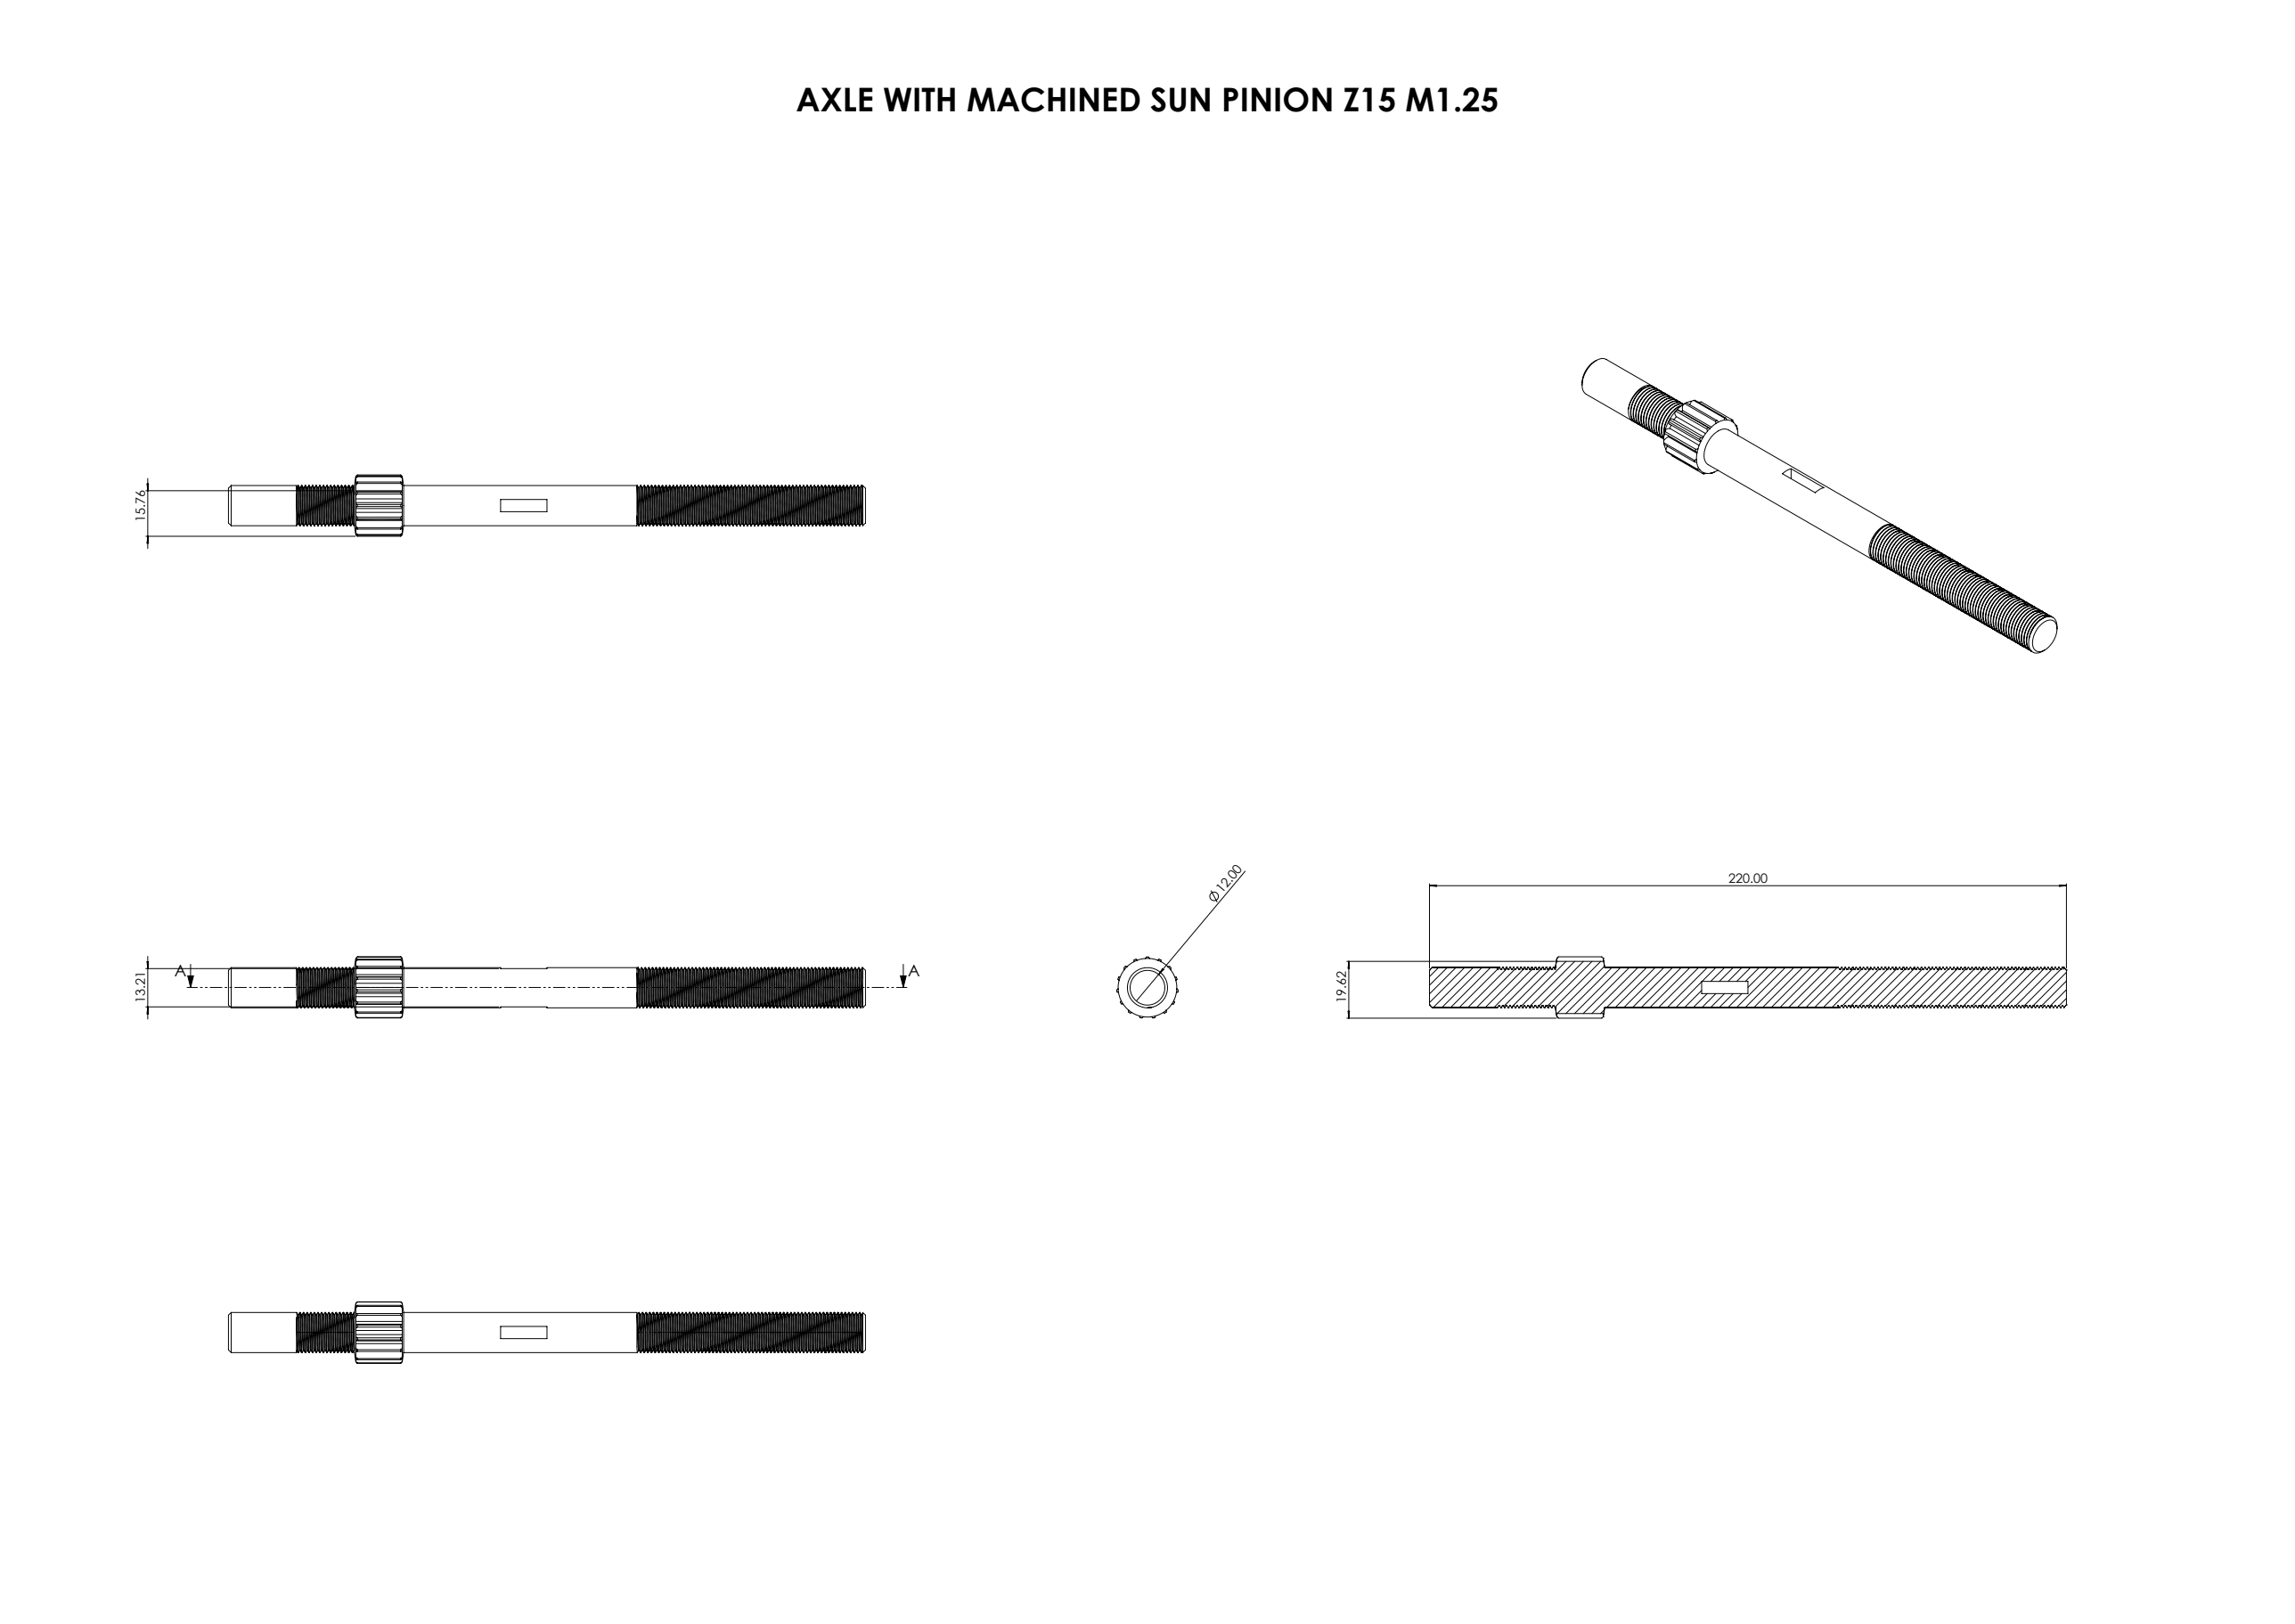
ISO-10303-21;
HEADER;
/* Generated by software containing ST-Developer
 * from STEP Tools, Inc. (www.steptools.com) 
 */

FILE_DESCRIPTION(
/* description */ (''),
/* implementation_level */ '2;1');

FILE_NAME(
/* name */ '01_Axle_with_Machined_Sun_Pinion_Z15_M1.25.step',
/* time_stamp */ '2026-10-11T13:00:10-07:00',
/* author */ (''),
/* organization */ (''),
/* preprocessor_version */ 'ST-DEVELOPER v20.2',
/* originating_system */ 'Autodesk Translation Framework v15.15.0.0',
/* authorisation */ '');

FILE_SCHEMA (('AUTOMOTIVE_DESIGN { 1 0 10303 214 3 1 1 }'));
ENDSEC;

DATA;
#10=MECHANICAL_DESIGN_GEOMETRIC_PRESENTATION_REPRESENTATION('',(#358),#65563);
#336=SHAPE_REPRESENTATION_RELATIONSHIP('SRR','None',#65614,#347);
#347=ADVANCED_BREP_SHAPE_REPRESENTATION('',(#369),#65552);
#358=STYLED_ITEM('',(#65788),#369);
#369=MANIFOLD_SOLID_BREP('Body1',#20008);
#380=CONICAL_SURFACE('',#20340,10.375,0.785398163397451);
#381=CONICAL_SURFACE('',#20343,10.375,0.785398163397451);
#382=CONICAL_SURFACE('',#20348,10.375,0.785398163397451);
#383=CONICAL_SURFACE('',#20357,10.375,0.785398163397451);
#384=CONICAL_SURFACE('',#20362,10.375,0.785398163397451);
#385=CONICAL_SURFACE('',#20371,10.375,0.785398163397451);
#386=CONICAL_SURFACE('',#20376,10.375,0.785398163397451);
#387=CONICAL_SURFACE('',#20385,10.375,0.785398163397451);
#388=CONICAL_SURFACE('',#20390,10.375,0.785398163397451);
#389=CONICAL_SURFACE('',#20399,10.375,0.785398163397451);
#390=CONICAL_SURFACE('',#20404,10.375,0.785398163397451);
#391=CONICAL_SURFACE('',#20413,10.375,0.785398163397451);
#392=CONICAL_SURFACE('',#20418,10.375,0.785398163397451);
#393=CONICAL_SURFACE('',#20427,10.375,0.785398163397451);
#394=CONICAL_SURFACE('',#20432,10.375,0.785398163397451);
#395=CONICAL_SURFACE('',#20443,10.375,0.785398163397451);
#396=CONICAL_SURFACE('',#20448,10.375,0.785398163397451);
#397=CONICAL_SURFACE('',#20457,10.375,0.785398163397451);
#398=CONICAL_SURFACE('',#20462,10.375,0.785398163397451);
#399=CONICAL_SURFACE('',#20471,10.375,0.785398163397451);
#400=CONICAL_SURFACE('',#20476,10.375,0.785398163397451);
#401=CONICAL_SURFACE('',#20485,10.375,0.785398163397451);
#402=CONICAL_SURFACE('',#20490,10.375,0.785398163397451);
#403=CONICAL_SURFACE('',#20499,10.375,0.785398163397451);
#404=CONICAL_SURFACE('',#20504,10.375,0.785398163397451);
#405=CONICAL_SURFACE('',#20513,10.375,0.785398163397451);
#406=CONICAL_SURFACE('',#20518,10.375,0.785398163397451);
#407=CONICAL_SURFACE('',#20527,10.375,0.785398163397451);
#408=CONICAL_SURFACE('',#20532,10.375,0.785398163397451);
#409=CONICAL_SURFACE('',#20541,10.375,0.785398163397451);
#410=CONICAL_SURFACE('',#20547,6.5,0.78539816339745);
#411=CONICAL_SURFACE('',#20548,8.5625,1.41214106460849);
#412=CONICAL_SURFACE('',#20549,8.5625,1.4121410646085);
#413=CONICAL_SURFACE('',#20552,6.5,0.78539816339745);
#500=(
BOUNDED_SURFACE()
B_SPLINE_SURFACE(5,1,((#42423,#42424),(#42425,#42426),(#42427,#42428),(#42429,
#42430),(#42431,#42432),(#42433,#42434),(#42435,#42436),(#42437,#42438),
(#42439,#42440),(#42441,#42442),(#42443,#42444),(#42445,#42446),(#42447,
#42448),(#42449,#42450),(#42451,#42452),(#42453,#42454),(#42455,#42456),
(#42457,#42458),(#42459,#42460),(#42461,#42462),(#42463,#42464),(#42465,
#42466),(#42467,#42468),(#42469,#42470),(#42471,#42472),(#42473,#42474),
(#42475,#42476),(#42477,#42478),(#42479,#42480),(#42481,#42482),(#42483,
#42484),(#42485,#42486),(#42487,#42488),(#42489,#42490),(#42491,#42492),
(#42493,#42494),(#42495,#42496),(#42497,#42498),(#42499,#42500),(#42501,
#42502)),.UNSPECIFIED.,.F.,.F.,.F.)
B_SPLINE_SURFACE_WITH_KNOTS((6,1,1,1,1,1,1,1,1,1,1,1,1,1,1,1,1,1,1,1,1,
1,1,1,1,1,1,1,1,1,1,1,1,1,1,6),(2,2),(-1.,-0.971428571428572,-0.942857142857143,
-0.914285714285714,-0.885714285714286,-0.857142857142857,-0.828571428571429,
-0.8,-0.771428571428572,-0.742857142857143,-0.714285714285714,-0.685714285714286,
-0.657142857142857,-0.628571428571429,-0.6,-0.571428571428572,-0.542857142857143,
-0.514285714285714,-0.485714285714286,-0.457142857142857,-0.428571428571429,
-0.4,-0.371428571428571,-0.342857142857143,-0.314285714285714,-0.285714285714286,
-0.257142857142857,-0.228571428571429,-0.2,-0.171428571428571,-0.142857142857143,
-0.114285714285714,-0.0857142857142857,-0.0571428571428571,-0.0285714285714286,
0.),(0.,1.6),.UNSPECIFIED.)
GEOMETRIC_REPRESENTATION_ITEM()
RATIONAL_B_SPLINE_SURFACE(((1.,1.),(1.,1.),(1.,1.),(1.,1.),(1.,1.),(1.,
1.),(1.,1.),(1.,1.),(1.,1.),(1.,1.),(1.,1.),(1.,1.),(1.,1.),(1.,1.),(1.,
1.),(1.,1.),(1.,1.),(1.,1.),(1.,1.),(1.,1.),(1.,1.),(1.,1.),(1.,1.),(1.,
1.),(1.,1.),(1.,1.),(1.,1.),(1.,1.),(1.,1.),(1.,1.),(1.,1.),(1.,1.),(1.,
1.),(1.,1.),(1.,1.),(1.,1.),(1.,1.),(1.,1.),(1.,1.),(1.,1.)))
REPRESENTATION_ITEM('')
SURFACE()
);
#501=(
BOUNDED_SURFACE()
B_SPLINE_SURFACE(5,1,((#42551,#42552),(#42553,#42554),(#42555,#42556),(#42557,
#42558),(#42559,#42560),(#42561,#42562),(#42563,#42564),(#42565,#42566),
(#42567,#42568),(#42569,#42570),(#42571,#42572),(#42573,#42574),(#42575,
#42576),(#42577,#42578),(#42579,#42580),(#42581,#42582),(#42583,#42584),
(#42585,#42586),(#42587,#42588),(#42589,#42590),(#42591,#42592),(#42593,
#42594),(#42595,#42596),(#42597,#42598),(#42599,#42600),(#42601,#42602),
(#42603,#42604),(#42605,#42606),(#42607,#42608),(#42609,#42610),(#42611,
#42612),(#42613,#42614),(#42615,#42616),(#42617,#42618),(#42619,#42620),
(#42621,#42622),(#42623,#42624),(#42625,#42626),(#42627,#42628),(#42629,
#42630)),.UNSPECIFIED.,.F.,.F.,.F.)
B_SPLINE_SURFACE_WITH_KNOTS((6,1,1,1,1,1,1,1,1,1,1,1,1,1,1,1,1,1,1,1,1,
1,1,1,1,1,1,1,1,1,1,1,1,1,1,6),(2,2),(-1.,-0.971428571428572,-0.942857142857143,
-0.914285714285714,-0.885714285714286,-0.857142857142857,-0.828571428571429,
-0.8,-0.771428571428572,-0.742857142857143,-0.714285714285714,-0.685714285714286,
-0.657142857142857,-0.628571428571429,-0.6,-0.571428571428572,-0.542857142857143,
-0.514285714285714,-0.485714285714286,-0.457142857142857,-0.428571428571429,
-0.4,-0.371428571428571,-0.342857142857143,-0.314285714285714,-0.285714285714286,
-0.257142857142857,-0.228571428571429,-0.2,-0.171428571428571,-0.142857142857143,
-0.114285714285714,-0.0857142857142857,-0.0571428571428571,-0.0285714285714286,
0.),(0.,1.6),.UNSPECIFIED.)
GEOMETRIC_REPRESENTATION_ITEM()
RATIONAL_B_SPLINE_SURFACE(((1.,1.),(1.,1.),(1.,1.),(1.,1.),(1.,1.),(1.,
1.),(1.,1.),(1.,1.),(1.,1.),(1.,1.),(1.,1.),(1.,1.),(1.,1.),(1.,1.),(1.,
1.),(1.,1.),(1.,1.),(1.,1.),(1.,1.),(1.,1.),(1.,1.),(1.,1.),(1.,1.),(1.,
1.),(1.,1.),(1.,1.),(1.,1.),(1.,1.),(1.,1.),(1.,1.),(1.,1.),(1.,1.),(1.,
1.),(1.,1.),(1.,1.),(1.,1.),(1.,1.),(1.,1.),(1.,1.),(1.,1.)))
REPRESENTATION_ITEM('')
SURFACE()
);
#502=(
BOUNDED_SURFACE()
B_SPLINE_SURFACE(5,1,((#42775,#42776),(#42777,#42778),(#42779,#42780),(#42781,
#42782),(#42783,#42784),(#42785,#42786),(#42787,#42788),(#42789,#42790),
(#42791,#42792),(#42793,#42794),(#42795,#42796),(#42797,#42798),(#42799,
#42800),(#42801,#42802),(#42803,#42804),(#42805,#42806),(#42807,#42808),
(#42809,#42810),(#42811,#42812),(#42813,#42814),(#42815,#42816),(#42817,
#42818),(#42819,#42820),(#42821,#42822),(#42823,#42824),(#42825,#42826),
(#42827,#42828),(#42829,#42830),(#42831,#42832),(#42833,#42834),(#42835,
#42836),(#42837,#42838),(#42839,#42840),(#42841,#42842),(#42843,#42844),
(#42845,#42846),(#42847,#42848),(#42849,#42850),(#42851,#42852),(#42853,
#42854)),.UNSPECIFIED.,.F.,.F.,.F.)
B_SPLINE_SURFACE_WITH_KNOTS((6,1,1,1,1,1,1,1,1,1,1,1,1,1,1,1,1,1,1,1,1,
1,1,1,1,1,1,1,1,1,1,1,1,1,1,6),(2,2),(-1.,-0.971428571428572,-0.942857142857143,
-0.914285714285714,-0.885714285714286,-0.857142857142857,-0.828571428571429,
-0.8,-0.771428571428572,-0.742857142857143,-0.714285714285714,-0.685714285714286,
-0.657142857142857,-0.628571428571429,-0.6,-0.571428571428572,-0.542857142857143,
-0.514285714285714,-0.485714285714286,-0.457142857142857,-0.428571428571429,
-0.4,-0.371428571428571,-0.342857142857143,-0.314285714285714,-0.285714285714286,
-0.257142857142857,-0.228571428571429,-0.2,-0.171428571428571,-0.142857142857143,
-0.114285714285714,-0.0857142857142857,-0.0571428571428571,-0.0285714285714286,
0.),(0.,1.6),.UNSPECIFIED.)
GEOMETRIC_REPRESENTATION_ITEM()
RATIONAL_B_SPLINE_SURFACE(((1.,1.),(1.,1.),(1.,1.),(1.,1.),(1.,1.),(1.,
1.),(1.,1.),(1.,1.),(1.,1.),(1.,1.),(1.,1.),(1.,1.),(1.,1.),(1.,1.),(1.,
1.),(1.,1.),(1.,1.),(1.,1.),(1.,1.),(1.,1.),(1.,1.),(1.,1.),(1.,1.),(1.,
1.),(1.,1.),(1.,1.),(1.,1.),(1.,1.),(1.,1.),(1.,1.),(1.,1.),(1.,1.),(1.,
1.),(1.,1.),(1.,1.),(1.,1.),(1.,1.),(1.,1.),(1.,1.),(1.,1.)))
REPRESENTATION_ITEM('')
SURFACE()
);
#503=(
BOUNDED_SURFACE()
B_SPLINE_SURFACE(5,1,((#42903,#42904),(#42905,#42906),(#42907,#42908),(#42909,
#42910),(#42911,#42912),(#42913,#42914),(#42915,#42916),(#42917,#42918),
(#42919,#42920),(#42921,#42922),(#42923,#42924),(#42925,#42926),(#42927,
#42928),(#42929,#42930),(#42931,#42932),(#42933,#42934),(#42935,#42936),
(#42937,#42938),(#42939,#42940),(#42941,#42942),(#42943,#42944),(#42945,
#42946),(#42947,#42948),(#42949,#42950),(#42951,#42952),(#42953,#42954),
(#42955,#42956),(#42957,#42958),(#42959,#42960),(#42961,#42962),(#42963,
#42964),(#42965,#42966),(#42967,#42968),(#42969,#42970),(#42971,#42972),
(#42973,#42974),(#42975,#42976),(#42977,#42978),(#42979,#42980),(#42981,
#42982)),.UNSPECIFIED.,.F.,.F.,.F.)
B_SPLINE_SURFACE_WITH_KNOTS((6,1,1,1,1,1,1,1,1,1,1,1,1,1,1,1,1,1,1,1,1,
1,1,1,1,1,1,1,1,1,1,1,1,1,1,6),(2,2),(-1.,-0.971428571428572,-0.942857142857143,
-0.914285714285714,-0.885714285714286,-0.857142857142857,-0.828571428571429,
-0.8,-0.771428571428572,-0.742857142857143,-0.714285714285714,-0.685714285714286,
-0.657142857142857,-0.628571428571429,-0.6,-0.571428571428572,-0.542857142857143,
-0.514285714285714,-0.485714285714286,-0.457142857142857,-0.428571428571429,
-0.4,-0.371428571428571,-0.342857142857143,-0.314285714285714,-0.285714285714286,
-0.257142857142857,-0.228571428571429,-0.2,-0.171428571428571,-0.142857142857143,
-0.114285714285714,-0.0857142857142857,-0.0571428571428571,-0.0285714285714286,
0.),(0.,1.6),.UNSPECIFIED.)
GEOMETRIC_REPRESENTATION_ITEM()
RATIONAL_B_SPLINE_SURFACE(((1.,1.),(1.,1.),(1.,1.),(1.,1.),(1.,1.),(1.,
1.),(1.,1.),(1.,1.),(1.,1.),(1.,1.),(1.,1.),(1.,1.),(1.,1.),(1.,1.),(1.,
1.),(1.,1.),(1.,1.),(1.,1.),(1.,1.),(1.,1.),(1.,1.),(1.,1.),(1.,1.),(1.,
1.),(1.,1.),(1.,1.),(1.,1.),(1.,1.),(1.,1.),(1.,1.),(1.,1.),(1.,1.),(1.,
1.),(1.,1.),(1.,1.),(1.,1.),(1.,1.),(1.,1.),(1.,1.),(1.,1.)))
REPRESENTATION_ITEM('')
SURFACE()
);
#504=(
BOUNDED_SURFACE()
B_SPLINE_SURFACE(5,1,((#43097,#43098),(#43099,#43100),(#43101,#43102),(#43103,
#43104),(#43105,#43106),(#43107,#43108),(#43109,#43110),(#43111,#43112),
(#43113,#43114),(#43115,#43116),(#43117,#43118),(#43119,#43120),(#43121,
#43122),(#43123,#43124),(#43125,#43126),(#43127,#43128),(#43129,#43130),
(#43131,#43132),(#43133,#43134),(#43135,#43136),(#43137,#43138),(#43139,
#43140),(#43141,#43142),(#43143,#43144),(#43145,#43146),(#43147,#43148),
(#43149,#43150),(#43151,#43152),(#43153,#43154),(#43155,#43156),(#43157,
#43158),(#43159,#43160),(#43161,#43162),(#43163,#43164),(#43165,#43166),
(#43167,#43168),(#43169,#43170),(#43171,#43172),(#43173,#43174),(#43175,
#43176)),.UNSPECIFIED.,.F.,.F.,.F.)
B_SPLINE_SURFACE_WITH_KNOTS((6,1,1,1,1,1,1,1,1,1,1,1,1,1,1,1,1,1,1,1,1,
1,1,1,1,1,1,1,1,1,1,1,1,1,1,6),(2,2),(-1.,-0.971428571428572,-0.942857142857143,
-0.914285714285714,-0.885714285714286,-0.857142857142857,-0.828571428571429,
-0.8,-0.771428571428572,-0.742857142857143,-0.714285714285714,-0.685714285714286,
-0.657142857142857,-0.628571428571429,-0.6,-0.571428571428572,-0.542857142857143,
-0.514285714285714,-0.485714285714286,-0.457142857142857,-0.428571428571429,
-0.4,-0.371428571428571,-0.342857142857143,-0.314285714285714,-0.285714285714286,
-0.257142857142857,-0.228571428571429,-0.2,-0.171428571428571,-0.142857142857143,
-0.114285714285714,-0.0857142857142857,-0.0571428571428571,-0.0285714285714286,
0.),(0.,1.6),.UNSPECIFIED.)
GEOMETRIC_REPRESENTATION_ITEM()
RATIONAL_B_SPLINE_SURFACE(((1.,1.),(1.,1.),(1.,1.),(1.,1.),(1.,1.),(1.,
1.),(1.,1.),(1.,1.),(1.,1.),(1.,1.),(1.,1.),(1.,1.),(1.,1.),(1.,1.),(1.,
1.),(1.,1.),(1.,1.),(1.,1.),(1.,1.),(1.,1.),(1.,1.),(1.,1.),(1.,1.),(1.,
1.),(1.,1.),(1.,1.),(1.,1.),(1.,1.),(1.,1.),(1.,1.),(1.,1.),(1.,1.),(1.,
1.),(1.,1.),(1.,1.),(1.,1.),(1.,1.),(1.,1.),(1.,1.),(1.,1.)))
REPRESENTATION_ITEM('')
SURFACE()
);
#505=(
BOUNDED_SURFACE()
B_SPLINE_SURFACE(5,1,((#43225,#43226),(#43227,#43228),(#43229,#43230),(#43231,
#43232),(#43233,#43234),(#43235,#43236),(#43237,#43238),(#43239,#43240),
(#43241,#43242),(#43243,#43244),(#43245,#43246),(#43247,#43248),(#43249,
#43250),(#43251,#43252),(#43253,#43254),(#43255,#43256),(#43257,#43258),
(#43259,#43260),(#43261,#43262),(#43263,#43264),(#43265,#43266),(#43267,
#43268),(#43269,#43270),(#43271,#43272),(#43273,#43274),(#43275,#43276),
(#43277,#43278),(#43279,#43280),(#43281,#43282),(#43283,#43284),(#43285,
#43286),(#43287,#43288),(#43289,#43290),(#43291,#43292),(#43293,#43294),
(#43295,#43296),(#43297,#43298),(#43299,#43300),(#43301,#43302),(#43303,
#43304)),.UNSPECIFIED.,.F.,.F.,.F.)
B_SPLINE_SURFACE_WITH_KNOTS((6,1,1,1,1,1,1,1,1,1,1,1,1,1,1,1,1,1,1,1,1,
1,1,1,1,1,1,1,1,1,1,1,1,1,1,6),(2,2),(-1.,-0.971428571428572,-0.942857142857143,
-0.914285714285714,-0.885714285714286,-0.857142857142857,-0.828571428571429,
-0.8,-0.771428571428572,-0.742857142857143,-0.714285714285714,-0.685714285714286,
-0.657142857142857,-0.628571428571429,-0.6,-0.571428571428572,-0.542857142857143,
-0.514285714285714,-0.485714285714286,-0.457142857142857,-0.428571428571429,
-0.4,-0.371428571428571,-0.342857142857143,-0.314285714285714,-0.285714285714286,
-0.257142857142857,-0.228571428571429,-0.2,-0.171428571428571,-0.142857142857143,
-0.114285714285714,-0.0857142857142857,-0.0571428571428571,-0.0285714285714286,
0.),(0.,1.6),.UNSPECIFIED.)
GEOMETRIC_REPRESENTATION_ITEM()
RATIONAL_B_SPLINE_SURFACE(((1.,1.),(1.,1.),(1.,1.),(1.,1.),(1.,1.),(1.,
1.),(1.,1.),(1.,1.),(1.,1.),(1.,1.),(1.,1.),(1.,1.),(1.,1.),(1.,1.),(1.,
1.),(1.,1.),(1.,1.),(1.,1.),(1.,1.),(1.,1.),(1.,1.),(1.,1.),(1.,1.),(1.,
1.),(1.,1.),(1.,1.),(1.,1.),(1.,1.),(1.,1.),(1.,1.),(1.,1.),(1.,1.),(1.,
1.),(1.,1.),(1.,1.),(1.,1.),(1.,1.),(1.,1.),(1.,1.),(1.,1.)))
REPRESENTATION_ITEM('')
SURFACE()
);
#506=(
BOUNDED_SURFACE()
B_SPLINE_SURFACE(5,1,((#43419,#43420),(#43421,#43422),(#43423,#43424),(#43425,
#43426),(#43427,#43428),(#43429,#43430),(#43431,#43432),(#43433,#43434),
(#43435,#43436),(#43437,#43438),(#43439,#43440),(#43441,#43442),(#43443,
#43444),(#43445,#43446),(#43447,#43448),(#43449,#43450),(#43451,#43452),
(#43453,#43454),(#43455,#43456),(#43457,#43458),(#43459,#43460),(#43461,
#43462),(#43463,#43464),(#43465,#43466),(#43467,#43468),(#43469,#43470),
(#43471,#43472),(#43473,#43474),(#43475,#43476),(#43477,#43478),(#43479,
#43480),(#43481,#43482),(#43483,#43484),(#43485,#43486),(#43487,#43488),
(#43489,#43490),(#43491,#43492),(#43493,#43494),(#43495,#43496),(#43497,
#43498)),.UNSPECIFIED.,.F.,.F.,.F.)
B_SPLINE_SURFACE_WITH_KNOTS((6,1,1,1,1,1,1,1,1,1,1,1,1,1,1,1,1,1,1,1,1,
1,1,1,1,1,1,1,1,1,1,1,1,1,1,6),(2,2),(-1.,-0.971428571428572,-0.942857142857143,
-0.914285714285714,-0.885714285714286,-0.857142857142857,-0.828571428571429,
-0.8,-0.771428571428572,-0.742857142857143,-0.714285714285714,-0.685714285714286,
-0.657142857142857,-0.628571428571429,-0.6,-0.571428571428572,-0.542857142857143,
-0.514285714285714,-0.485714285714286,-0.457142857142857,-0.428571428571429,
-0.4,-0.371428571428571,-0.342857142857143,-0.314285714285714,-0.285714285714286,
-0.257142857142857,-0.228571428571429,-0.2,-0.171428571428571,-0.142857142857143,
-0.114285714285714,-0.0857142857142857,-0.0571428571428571,-0.0285714285714286,
0.),(0.,1.6),.UNSPECIFIED.)
GEOMETRIC_REPRESENTATION_ITEM()
RATIONAL_B_SPLINE_SURFACE(((1.,1.),(1.,1.),(1.,1.),(1.,1.),(1.,1.),(1.,
1.),(1.,1.),(1.,1.),(1.,1.),(1.,1.),(1.,1.),(1.,1.),(1.,1.),(1.,1.),(1.,
1.),(1.,1.),(1.,1.),(1.,1.),(1.,1.),(1.,1.),(1.,1.),(1.,1.),(1.,1.),(1.,
1.),(1.,1.),(1.,1.),(1.,1.),(1.,1.),(1.,1.),(1.,1.),(1.,1.),(1.,1.),(1.,
1.),(1.,1.),(1.,1.),(1.,1.),(1.,1.),(1.,1.),(1.,1.),(1.,1.)))
REPRESENTATION_ITEM('')
SURFACE()
);
#507=(
BOUNDED_SURFACE()
B_SPLINE_SURFACE(5,1,((#43547,#43548),(#43549,#43550),(#43551,#43552),(#43553,
#43554),(#43555,#43556),(#43557,#43558),(#43559,#43560),(#43561,#43562),
(#43563,#43564),(#43565,#43566),(#43567,#43568),(#43569,#43570),(#43571,
#43572),(#43573,#43574),(#43575,#43576),(#43577,#43578),(#43579,#43580),
(#43581,#43582),(#43583,#43584),(#43585,#43586),(#43587,#43588),(#43589,
#43590),(#43591,#43592),(#43593,#43594),(#43595,#43596),(#43597,#43598),
(#43599,#43600),(#43601,#43602),(#43603,#43604),(#43605,#43606),(#43607,
#43608),(#43609,#43610),(#43611,#43612),(#43613,#43614),(#43615,#43616),
(#43617,#43618),(#43619,#43620),(#43621,#43622),(#43623,#43624),(#43625,
#43626)),.UNSPECIFIED.,.F.,.F.,.F.)
B_SPLINE_SURFACE_WITH_KNOTS((6,1,1,1,1,1,1,1,1,1,1,1,1,1,1,1,1,1,1,1,1,
1,1,1,1,1,1,1,1,1,1,1,1,1,1,6),(2,2),(-1.,-0.971428571428572,-0.942857142857143,
-0.914285714285714,-0.885714285714286,-0.857142857142857,-0.828571428571429,
-0.8,-0.771428571428572,-0.742857142857143,-0.714285714285714,-0.685714285714286,
-0.657142857142857,-0.628571428571429,-0.6,-0.571428571428572,-0.542857142857143,
-0.514285714285714,-0.485714285714286,-0.457142857142857,-0.428571428571429,
-0.4,-0.371428571428571,-0.342857142857143,-0.314285714285714,-0.285714285714286,
-0.257142857142857,-0.228571428571429,-0.2,-0.171428571428571,-0.142857142857143,
-0.114285714285714,-0.0857142857142857,-0.0571428571428571,-0.0285714285714286,
0.),(0.,1.6),.UNSPECIFIED.)
GEOMETRIC_REPRESENTATION_ITEM()
RATIONAL_B_SPLINE_SURFACE(((1.,1.),(1.,1.),(1.,1.),(1.,1.),(1.,1.),(1.,
1.),(1.,1.),(1.,1.),(1.,1.),(1.,1.),(1.,1.),(1.,1.),(1.,1.),(1.,1.),(1.,
1.),(1.,1.),(1.,1.),(1.,1.),(1.,1.),(1.,1.),(1.,1.),(1.,1.),(1.,1.),(1.,
1.),(1.,1.),(1.,1.),(1.,1.),(1.,1.),(1.,1.),(1.,1.),(1.,1.),(1.,1.),(1.,
1.),(1.,1.),(1.,1.),(1.,1.),(1.,1.),(1.,1.),(1.,1.),(1.,1.)))
REPRESENTATION_ITEM('')
SURFACE()
);
#508=(
BOUNDED_SURFACE()
B_SPLINE_SURFACE(5,1,((#43741,#43742),(#43743,#43744),(#43745,#43746),(#43747,
#43748),(#43749,#43750),(#43751,#43752),(#43753,#43754),(#43755,#43756),
(#43757,#43758),(#43759,#43760),(#43761,#43762),(#43763,#43764),(#43765,
#43766),(#43767,#43768),(#43769,#43770),(#43771,#43772),(#43773,#43774),
(#43775,#43776),(#43777,#43778),(#43779,#43780),(#43781,#43782),(#43783,
#43784),(#43785,#43786),(#43787,#43788),(#43789,#43790),(#43791,#43792),
(#43793,#43794),(#43795,#43796),(#43797,#43798),(#43799,#43800),(#43801,
#43802),(#43803,#43804),(#43805,#43806),(#43807,#43808),(#43809,#43810),
(#43811,#43812),(#43813,#43814),(#43815,#43816),(#43817,#43818),(#43819,
#43820)),.UNSPECIFIED.,.F.,.F.,.F.)
B_SPLINE_SURFACE_WITH_KNOTS((6,1,1,1,1,1,1,1,1,1,1,1,1,1,1,1,1,1,1,1,1,
1,1,1,1,1,1,1,1,1,1,1,1,1,1,6),(2,2),(-1.,-0.971428571428572,-0.942857142857143,
-0.914285714285714,-0.885714285714286,-0.857142857142857,-0.828571428571429,
-0.8,-0.771428571428572,-0.742857142857143,-0.714285714285714,-0.685714285714286,
-0.657142857142857,-0.628571428571429,-0.6,-0.571428571428572,-0.542857142857143,
-0.514285714285714,-0.485714285714286,-0.457142857142857,-0.428571428571429,
-0.4,-0.371428571428571,-0.342857142857143,-0.314285714285714,-0.285714285714286,
-0.257142857142857,-0.228571428571429,-0.2,-0.171428571428571,-0.142857142857143,
-0.114285714285714,-0.0857142857142857,-0.0571428571428571,-0.0285714285714286,
0.),(0.,1.6),.UNSPECIFIED.)
GEOMETRIC_REPRESENTATION_ITEM()
RATIONAL_B_SPLINE_SURFACE(((1.,1.),(1.,1.),(1.,1.),(1.,1.),(1.,1.),(1.,
1.),(1.,1.),(1.,1.),(1.,1.),(1.,1.),(1.,1.),(1.,1.),(1.,1.),(1.,1.),(1.,
1.),(1.,1.),(1.,1.),(1.,1.),(1.,1.),(1.,1.),(1.,1.),(1.,1.),(1.,1.),(1.,
1.),(1.,1.),(1.,1.),(1.,1.),(1.,1.),(1.,1.),(1.,1.),(1.,1.),(1.,1.),(1.,
1.),(1.,1.),(1.,1.),(1.,1.),(1.,1.),(1.,1.),(1.,1.),(1.,1.)))
REPRESENTATION_ITEM('')
SURFACE()
);
#509=(
BOUNDED_SURFACE()
B_SPLINE_SURFACE(5,1,((#43882,#43883),(#43884,#43885),(#43886,#43887),(#43888,
#43889),(#43890,#43891),(#43892,#43893),(#43894,#43895),(#43896,#43897),
(#43898,#43899),(#43900,#43901),(#43902,#43903),(#43904,#43905),(#43906,
#43907),(#43908,#43909),(#43910,#43911),(#43912,#43913),(#43914,#43915),
(#43916,#43917),(#43918,#43919),(#43920,#43921),(#43922,#43923),(#43924,
#43925),(#43926,#43927),(#43928,#43929),(#43930,#43931),(#43932,#43933),
(#43934,#43935),(#43936,#43937),(#43938,#43939),(#43940,#43941),(#43942,
#43943),(#43944,#43945),(#43946,#43947),(#43948,#43949),(#43950,#43951),
(#43952,#43953),(#43954,#43955),(#43956,#43957),(#43958,#43959),(#43960,
#43961)),.UNSPECIFIED.,.F.,.F.,.F.)
B_SPLINE_SURFACE_WITH_KNOTS((6,1,1,1,1,1,1,1,1,1,1,1,1,1,1,1,1,1,1,1,1,
1,1,1,1,1,1,1,1,1,1,1,1,1,1,6),(2,2),(-1.,-0.971428571428572,-0.942857142857143,
-0.914285714285714,-0.885714285714286,-0.857142857142857,-0.828571428571429,
-0.8,-0.771428571428572,-0.742857142857143,-0.714285714285714,-0.685714285714286,
-0.657142857142857,-0.628571428571429,-0.6,-0.571428571428572,-0.542857142857143,
-0.514285714285714,-0.485714285714286,-0.457142857142857,-0.428571428571429,
-0.4,-0.371428571428571,-0.342857142857143,-0.314285714285714,-0.285714285714286,
-0.257142857142857,-0.228571428571429,-0.2,-0.171428571428571,-0.142857142857143,
-0.114285714285714,-0.0857142857142857,-0.0571428571428571,-0.0285714285714286,
0.),(0.,1.6),.UNSPECIFIED.)
GEOMETRIC_REPRESENTATION_ITEM()
RATIONAL_B_SPLINE_SURFACE(((1.,1.),(1.,1.),(1.,1.),(1.,1.),(1.,1.),(1.,
1.),(1.,1.),(1.,1.),(1.,1.),(1.,1.),(1.,1.),(1.,1.),(1.,1.),(1.,1.),(1.,
1.),(1.,1.),(1.,1.),(1.,1.),(1.,1.),(1.,1.),(1.,1.),(1.,1.),(1.,1.),(1.,
1.),(1.,1.),(1.,1.),(1.,1.),(1.,1.),(1.,1.),(1.,1.),(1.,1.),(1.,1.),(1.,
1.),(1.,1.),(1.,1.),(1.,1.),(1.,1.),(1.,1.),(1.,1.),(1.,1.)))
REPRESENTATION_ITEM('')
SURFACE()
);
#510=(
BOUNDED_SURFACE()
B_SPLINE_SURFACE(5,1,((#44076,#44077),(#44078,#44079),(#44080,#44081),(#44082,
#44083),(#44084,#44085),(#44086,#44087),(#44088,#44089),(#44090,#44091),
(#44092,#44093),(#44094,#44095),(#44096,#44097),(#44098,#44099),(#44100,
#44101),(#44102,#44103),(#44104,#44105),(#44106,#44107),(#44108,#44109),
(#44110,#44111),(#44112,#44113),(#44114,#44115),(#44116,#44117),(#44118,
#44119),(#44120,#44121),(#44122,#44123),(#44124,#44125),(#44126,#44127),
(#44128,#44129),(#44130,#44131),(#44132,#44133),(#44134,#44135),(#44136,
#44137),(#44138,#44139),(#44140,#44141),(#44142,#44143),(#44144,#44145),
(#44146,#44147),(#44148,#44149),(#44150,#44151),(#44152,#44153),(#44154,
#44155)),.UNSPECIFIED.,.F.,.F.,.F.)
B_SPLINE_SURFACE_WITH_KNOTS((6,1,1,1,1,1,1,1,1,1,1,1,1,1,1,1,1,1,1,1,1,
1,1,1,1,1,1,1,1,1,1,1,1,1,1,6),(2,2),(-1.,-0.971428571428572,-0.942857142857143,
-0.914285714285714,-0.885714285714286,-0.857142857142857,-0.828571428571429,
-0.8,-0.771428571428572,-0.742857142857143,-0.714285714285714,-0.685714285714286,
-0.657142857142857,-0.628571428571429,-0.6,-0.571428571428572,-0.542857142857143,
-0.514285714285714,-0.485714285714286,-0.457142857142857,-0.428571428571429,
-0.4,-0.371428571428571,-0.342857142857143,-0.314285714285714,-0.285714285714286,
-0.257142857142857,-0.228571428571429,-0.2,-0.171428571428571,-0.142857142857143,
-0.114285714285714,-0.0857142857142857,-0.0571428571428571,-0.0285714285714286,
0.),(0.,1.6),.UNSPECIFIED.)
GEOMETRIC_REPRESENTATION_ITEM()
RATIONAL_B_SPLINE_SURFACE(((1.,1.),(1.,1.),(1.,1.),(1.,1.),(1.,1.),(1.,
1.),(1.,1.),(1.,1.),(1.,1.),(1.,1.),(1.,1.),(1.,1.),(1.,1.),(1.,1.),(1.,
1.),(1.,1.),(1.,1.),(1.,1.),(1.,1.),(1.,1.),(1.,1.),(1.,1.),(1.,1.),(1.,
1.),(1.,1.),(1.,1.),(1.,1.),(1.,1.),(1.,1.),(1.,1.),(1.,1.),(1.,1.),(1.,
1.),(1.,1.),(1.,1.),(1.,1.),(1.,1.),(1.,1.),(1.,1.),(1.,1.)))
REPRESENTATION_ITEM('')
SURFACE()
);
#511=(
BOUNDED_SURFACE()
B_SPLINE_SURFACE(5,1,((#44204,#44205),(#44206,#44207),(#44208,#44209),(#44210,
#44211),(#44212,#44213),(#44214,#44215),(#44216,#44217),(#44218,#44219),
(#44220,#44221),(#44222,#44223),(#44224,#44225),(#44226,#44227),(#44228,
#44229),(#44230,#44231),(#44232,#44233),(#44234,#44235),(#44236,#44237),
(#44238,#44239),(#44240,#44241),(#44242,#44243),(#44244,#44245),(#44246,
#44247),(#44248,#44249),(#44250,#44251),(#44252,#44253),(#44254,#44255),
(#44256,#44257),(#44258,#44259),(#44260,#44261),(#44262,#44263),(#44264,
#44265),(#44266,#44267),(#44268,#44269),(#44270,#44271),(#44272,#44273),
(#44274,#44275),(#44276,#44277),(#44278,#44279),(#44280,#44281),(#44282,
#44283)),.UNSPECIFIED.,.F.,.F.,.F.)
B_SPLINE_SURFACE_WITH_KNOTS((6,1,1,1,1,1,1,1,1,1,1,1,1,1,1,1,1,1,1,1,1,
1,1,1,1,1,1,1,1,1,1,1,1,1,1,6),(2,2),(-1.,-0.971428571428572,-0.942857142857143,
-0.914285714285714,-0.885714285714286,-0.857142857142857,-0.828571428571429,
-0.8,-0.771428571428572,-0.742857142857143,-0.714285714285714,-0.685714285714286,
-0.657142857142857,-0.628571428571429,-0.6,-0.571428571428572,-0.542857142857143,
-0.514285714285714,-0.485714285714286,-0.457142857142857,-0.428571428571429,
-0.4,-0.371428571428571,-0.342857142857143,-0.314285714285714,-0.285714285714286,
-0.257142857142857,-0.228571428571429,-0.2,-0.171428571428571,-0.142857142857143,
-0.114285714285714,-0.0857142857142857,-0.0571428571428571,-0.0285714285714286,
0.),(0.,1.6),.UNSPECIFIED.)
GEOMETRIC_REPRESENTATION_ITEM()
RATIONAL_B_SPLINE_SURFACE(((1.,1.),(1.,1.),(1.,1.),(1.,1.),(1.,1.),(1.,
1.),(1.,1.),(1.,1.),(1.,1.),(1.,1.),(1.,1.),(1.,1.),(1.,1.),(1.,1.),(1.,
1.),(1.,1.),(1.,1.),(1.,1.),(1.,1.),(1.,1.),(1.,1.),(1.,1.),(1.,1.),(1.,
1.),(1.,1.),(1.,1.),(1.,1.),(1.,1.),(1.,1.),(1.,1.),(1.,1.),(1.,1.),(1.,
1.),(1.,1.),(1.,1.),(1.,1.),(1.,1.),(1.,1.),(1.,1.),(1.,1.)))
REPRESENTATION_ITEM('')
SURFACE()
);
#512=(
BOUNDED_SURFACE()
B_SPLINE_SURFACE(5,1,((#44398,#44399),(#44400,#44401),(#44402,#44403),(#44404,
#44405),(#44406,#44407),(#44408,#44409),(#44410,#44411),(#44412,#44413),
(#44414,#44415),(#44416,#44417),(#44418,#44419),(#44420,#44421),(#44422,
#44423),(#44424,#44425),(#44426,#44427),(#44428,#44429),(#44430,#44431),
(#44432,#44433),(#44434,#44435),(#44436,#44437),(#44438,#44439),(#44440,
#44441),(#44442,#44443),(#44444,#44445),(#44446,#44447),(#44448,#44449),
(#44450,#44451),(#44452,#44453),(#44454,#44455),(#44456,#44457),(#44458,
#44459),(#44460,#44461),(#44462,#44463),(#44464,#44465),(#44466,#44467),
(#44468,#44469),(#44470,#44471),(#44472,#44473),(#44474,#44475),(#44476,
#44477)),.UNSPECIFIED.,.F.,.F.,.F.)
B_SPLINE_SURFACE_WITH_KNOTS((6,1,1,1,1,1,1,1,1,1,1,1,1,1,1,1,1,1,1,1,1,
1,1,1,1,1,1,1,1,1,1,1,1,1,1,6),(2,2),(-1.,-0.971428571428572,-0.942857142857143,
-0.914285714285714,-0.885714285714286,-0.857142857142857,-0.828571428571429,
-0.8,-0.771428571428572,-0.742857142857143,-0.714285714285714,-0.685714285714286,
-0.657142857142857,-0.628571428571429,-0.6,-0.571428571428572,-0.542857142857143,
-0.514285714285714,-0.485714285714286,-0.457142857142857,-0.428571428571429,
-0.4,-0.371428571428571,-0.342857142857143,-0.314285714285714,-0.285714285714286,
-0.257142857142857,-0.228571428571429,-0.2,-0.171428571428571,-0.142857142857143,
-0.114285714285714,-0.0857142857142857,-0.0571428571428571,-0.0285714285714286,
0.),(0.,1.6),.UNSPECIFIED.)
GEOMETRIC_REPRESENTATION_ITEM()
RATIONAL_B_SPLINE_SURFACE(((1.,1.),(1.,1.),(1.,1.),(1.,1.),(1.,1.),(1.,
1.),(1.,1.),(1.,1.),(1.,1.),(1.,1.),(1.,1.),(1.,1.),(1.,1.),(1.,1.),(1.,
1.),(1.,1.),(1.,1.),(1.,1.),(1.,1.),(1.,1.),(1.,1.),(1.,1.),(1.,1.),(1.,
1.),(1.,1.),(1.,1.),(1.,1.),(1.,1.),(1.,1.),(1.,1.),(1.,1.),(1.,1.),(1.,
1.),(1.,1.),(1.,1.),(1.,1.),(1.,1.),(1.,1.),(1.,1.),(1.,1.)))
REPRESENTATION_ITEM('')
SURFACE()
);
#513=(
BOUNDED_SURFACE()
B_SPLINE_SURFACE(5,1,((#44526,#44527),(#44528,#44529),(#44530,#44531),(#44532,
#44533),(#44534,#44535),(#44536,#44537),(#44538,#44539),(#44540,#44541),
(#44542,#44543),(#44544,#44545),(#44546,#44547),(#44548,#44549),(#44550,
#44551),(#44552,#44553),(#44554,#44555),(#44556,#44557),(#44558,#44559),
(#44560,#44561),(#44562,#44563),(#44564,#44565),(#44566,#44567),(#44568,
#44569),(#44570,#44571),(#44572,#44573),(#44574,#44575),(#44576,#44577),
(#44578,#44579),(#44580,#44581),(#44582,#44583),(#44584,#44585),(#44586,
#44587),(#44588,#44589),(#44590,#44591),(#44592,#44593),(#44594,#44595),
(#44596,#44597),(#44598,#44599),(#44600,#44601),(#44602,#44603),(#44604,
#44605)),.UNSPECIFIED.,.F.,.F.,.F.)
B_SPLINE_SURFACE_WITH_KNOTS((6,1,1,1,1,1,1,1,1,1,1,1,1,1,1,1,1,1,1,1,1,
1,1,1,1,1,1,1,1,1,1,1,1,1,1,6),(2,2),(-1.,-0.971428571428572,-0.942857142857143,
-0.914285714285714,-0.885714285714286,-0.857142857142857,-0.828571428571429,
-0.8,-0.771428571428572,-0.742857142857143,-0.714285714285714,-0.685714285714286,
-0.657142857142857,-0.628571428571429,-0.6,-0.571428571428572,-0.542857142857143,
-0.514285714285714,-0.485714285714286,-0.457142857142857,-0.428571428571429,
-0.4,-0.371428571428571,-0.342857142857143,-0.314285714285714,-0.285714285714286,
-0.257142857142857,-0.228571428571429,-0.2,-0.171428571428571,-0.142857142857143,
-0.114285714285714,-0.0857142857142857,-0.0571428571428571,-0.0285714285714286,
0.),(0.,1.6),.UNSPECIFIED.)
GEOMETRIC_REPRESENTATION_ITEM()
RATIONAL_B_SPLINE_SURFACE(((1.,1.),(1.,1.),(1.,1.),(1.,1.),(1.,1.),(1.,
1.),(1.,1.),(1.,1.),(1.,1.),(1.,1.),(1.,1.),(1.,1.),(1.,1.),(1.,1.),(1.,
1.),(1.,1.),(1.,1.),(1.,1.),(1.,1.),(1.,1.),(1.,1.),(1.,1.),(1.,1.),(1.,
1.),(1.,1.),(1.,1.),(1.,1.),(1.,1.),(1.,1.),(1.,1.),(1.,1.),(1.,1.),(1.,
1.),(1.,1.),(1.,1.),(1.,1.),(1.,1.),(1.,1.),(1.,1.),(1.,1.)))
REPRESENTATION_ITEM('')
SURFACE()
);
#514=(
BOUNDED_SURFACE()
B_SPLINE_SURFACE(5,1,((#44722,#44723),(#44724,#44725),(#44726,#44727),(#44728,
#44729),(#44730,#44731),(#44732,#44733),(#44734,#44735),(#44736,#44737),
(#44738,#44739),(#44740,#44741),(#44742,#44743),(#44744,#44745),(#44746,
#44747),(#44748,#44749),(#44750,#44751),(#44752,#44753),(#44754,#44755),
(#44756,#44757),(#44758,#44759),(#44760,#44761),(#44762,#44763),(#44764,
#44765),(#44766,#44767),(#44768,#44769),(#44770,#44771),(#44772,#44773),
(#44774,#44775),(#44776,#44777),(#44778,#44779),(#44780,#44781),(#44782,
#44783),(#44784,#44785),(#44786,#44787),(#44788,#44789),(#44790,#44791),
(#44792,#44793),(#44794,#44795),(#44796,#44797),(#44798,#44799),(#44800,
#44801)),.UNSPECIFIED.,.F.,.F.,.F.)
B_SPLINE_SURFACE_WITH_KNOTS((6,1,1,1,1,1,1,1,1,1,1,1,1,1,1,1,1,1,1,1,1,
1,1,1,1,1,1,1,1,1,1,1,1,1,1,6),(2,2),(-1.,-0.971428571428572,-0.942857142857143,
-0.914285714285714,-0.885714285714286,-0.857142857142857,-0.828571428571429,
-0.8,-0.771428571428572,-0.742857142857143,-0.714285714285714,-0.685714285714286,
-0.657142857142857,-0.628571428571429,-0.6,-0.571428571428572,-0.542857142857143,
-0.514285714285714,-0.485714285714286,-0.457142857142857,-0.428571428571429,
-0.4,-0.371428571428571,-0.342857142857143,-0.314285714285714,-0.285714285714286,
-0.257142857142857,-0.228571428571429,-0.2,-0.171428571428571,-0.142857142857143,
-0.114285714285714,-0.0857142857142857,-0.0571428571428571,-0.0285714285714286,
0.),(0.,1.6),.UNSPECIFIED.)
GEOMETRIC_REPRESENTATION_ITEM()
RATIONAL_B_SPLINE_SURFACE(((1.,1.),(1.,1.),(1.,1.),(1.,1.),(1.,1.),(1.,
1.),(1.,1.),(1.,1.),(1.,1.),(1.,1.),(1.,1.),(1.,1.),(1.,1.),(1.,1.),(1.,
1.),(1.,1.),(1.,1.),(1.,1.),(1.,1.),(1.,1.),(1.,1.),(1.,1.),(1.,1.),(1.,
1.),(1.,1.),(1.,1.),(1.,1.),(1.,1.),(1.,1.),(1.,1.),(1.,1.),(1.,1.),(1.,
1.),(1.,1.),(1.,1.),(1.,1.),(1.,1.),(1.,1.),(1.,1.),(1.,1.)))
REPRESENTATION_ITEM('')
SURFACE()
);
#515=(
BOUNDED_SURFACE()
B_SPLINE_SURFACE(5,1,((#44852,#44853),(#44854,#44855),(#44856,#44857),(#44858,
#44859),(#44860,#44861),(#44862,#44863),(#44864,#44865),(#44866,#44867),
(#44868,#44869),(#44870,#44871),(#44872,#44873),(#44874,#44875),(#44876,
#44877),(#44878,#44879),(#44880,#44881),(#44882,#44883),(#44884,#44885),
(#44886,#44887),(#44888,#44889),(#44890,#44891),(#44892,#44893),(#44894,
#44895),(#44896,#44897),(#44898,#44899),(#44900,#44901),(#44902,#44903),
(#44904,#44905),(#44906,#44907),(#44908,#44909),(#44910,#44911),(#44912,
#44913),(#44914,#44915),(#44916,#44917),(#44918,#44919),(#44920,#44921),
(#44922,#44923),(#44924,#44925),(#44926,#44927),(#44928,#44929),(#44930,
#44931)),.UNSPECIFIED.,.F.,.F.,.F.)
B_SPLINE_SURFACE_WITH_KNOTS((6,1,1,1,1,1,1,1,1,1,1,1,1,1,1,1,1,1,1,1,1,
1,1,1,1,1,1,1,1,1,1,1,1,1,1,6),(2,2),(-1.,-0.971428571428572,-0.942857142857143,
-0.914285714285714,-0.885714285714286,-0.857142857142857,-0.828571428571429,
-0.8,-0.771428571428572,-0.742857142857143,-0.714285714285714,-0.685714285714286,
-0.657142857142857,-0.628571428571429,-0.6,-0.571428571428572,-0.542857142857143,
-0.514285714285714,-0.485714285714286,-0.457142857142857,-0.428571428571429,
-0.4,-0.371428571428571,-0.342857142857143,-0.314285714285714,-0.285714285714286,
-0.257142857142857,-0.228571428571429,-0.2,-0.171428571428571,-0.142857142857143,
-0.114285714285714,-0.0857142857142857,-0.0571428571428571,-0.0285714285714286,
0.),(0.,1.6),.UNSPECIFIED.)
GEOMETRIC_REPRESENTATION_ITEM()
RATIONAL_B_SPLINE_SURFACE(((1.,1.),(1.,1.),(1.,1.),(1.,1.),(1.,1.),(1.,
1.),(1.,1.),(1.,1.),(1.,1.),(1.,1.),(1.,1.),(1.,1.),(1.,1.),(1.,1.),(1.,
1.),(1.,1.),(1.,1.),(1.,1.),(1.,1.),(1.,1.),(1.,1.),(1.,1.),(1.,1.),(1.,
1.),(1.,1.),(1.,1.),(1.,1.),(1.,1.),(1.,1.),(1.,1.),(1.,1.),(1.,1.),(1.,
1.),(1.,1.),(1.,1.),(1.,1.),(1.,1.),(1.,1.),(1.,1.),(1.,1.)))
REPRESENTATION_ITEM('')
SURFACE()
);
#516=(
BOUNDED_SURFACE()
B_SPLINE_SURFACE(5,1,((#45048,#45049),(#45050,#45051),(#45052,#45053),(#45054,
#45055),(#45056,#45057),(#45058,#45059),(#45060,#45061),(#45062,#45063),
(#45064,#45065),(#45066,#45067),(#45068,#45069),(#45070,#45071),(#45072,
#45073),(#45074,#45075),(#45076,#45077),(#45078,#45079),(#45080,#45081),
(#45082,#45083),(#45084,#45085),(#45086,#45087),(#45088,#45089),(#45090,
#45091),(#45092,#45093),(#45094,#45095),(#45096,#45097),(#45098,#45099),
(#45100,#45101),(#45102,#45103),(#45104,#45105),(#45106,#45107),(#45108,
#45109),(#45110,#45111),(#45112,#45113),(#45114,#45115),(#45116,#45117),
(#45118,#45119),(#45120,#45121),(#45122,#45123),(#45124,#45125),(#45126,
#45127)),.UNSPECIFIED.,.F.,.F.,.F.)
B_SPLINE_SURFACE_WITH_KNOTS((6,1,1,1,1,1,1,1,1,1,1,1,1,1,1,1,1,1,1,1,1,
1,1,1,1,1,1,1,1,1,1,1,1,1,1,6),(2,2),(-1.,-0.971428571428572,-0.942857142857143,
-0.914285714285714,-0.885714285714286,-0.857142857142857,-0.828571428571429,
-0.8,-0.771428571428572,-0.742857142857143,-0.714285714285714,-0.685714285714286,
-0.657142857142857,-0.628571428571429,-0.6,-0.571428571428572,-0.542857142857143,
-0.514285714285714,-0.485714285714286,-0.457142857142857,-0.428571428571429,
-0.4,-0.371428571428571,-0.342857142857143,-0.314285714285714,-0.285714285714286,
-0.257142857142857,-0.228571428571429,-0.2,-0.171428571428571,-0.142857142857143,
-0.114285714285714,-0.0857142857142857,-0.0571428571428571,-0.0285714285714286,
0.),(0.,1.6),.UNSPECIFIED.)
GEOMETRIC_REPRESENTATION_ITEM()
RATIONAL_B_SPLINE_SURFACE(((1.,1.),(1.,1.),(1.,1.),(1.,1.),(1.,1.),(1.,
1.),(1.,1.),(1.,1.),(1.,1.),(1.,1.),(1.,1.),(1.,1.),(1.,1.),(1.,1.),(1.,
1.),(1.,1.),(1.,1.),(1.,1.),(1.,1.),(1.,1.),(1.,1.),(1.,1.),(1.,1.),(1.,
1.),(1.,1.),(1.,1.),(1.,1.),(1.,1.),(1.,1.),(1.,1.),(1.,1.),(1.,1.),(1.,
1.),(1.,1.),(1.,1.),(1.,1.),(1.,1.),(1.,1.),(1.,1.),(1.,1.)))
REPRESENTATION_ITEM('')
SURFACE()
);
#517=(
BOUNDED_SURFACE()
B_SPLINE_SURFACE(5,1,((#45176,#45177),(#45178,#45179),(#45180,#45181),(#45182,
#45183),(#45184,#45185),(#45186,#45187),(#45188,#45189),(#45190,#45191),
(#45192,#45193),(#45194,#45195),(#45196,#45197),(#45198,#45199),(#45200,
#45201),(#45202,#45203),(#45204,#45205),(#45206,#45207),(#45208,#45209),
(#45210,#45211),(#45212,#45213),(#45214,#45215),(#45216,#45217),(#45218,
#45219),(#45220,#45221),(#45222,#45223),(#45224,#45225),(#45226,#45227),
(#45228,#45229),(#45230,#45231),(#45232,#45233),(#45234,#45235),(#45236,
#45237),(#45238,#45239),(#45240,#45241),(#45242,#45243),(#45244,#45245),
(#45246,#45247),(#45248,#45249),(#45250,#45251),(#45252,#45253),(#45254,
#45255)),.UNSPECIFIED.,.F.,.F.,.F.)
B_SPLINE_SURFACE_WITH_KNOTS((6,1,1,1,1,1,1,1,1,1,1,1,1,1,1,1,1,1,1,1,1,
1,1,1,1,1,1,1,1,1,1,1,1,1,1,6),(2,2),(-1.,-0.971428571428572,-0.942857142857143,
-0.914285714285714,-0.885714285714286,-0.857142857142857,-0.828571428571429,
-0.8,-0.771428571428572,-0.742857142857143,-0.714285714285714,-0.685714285714286,
-0.657142857142857,-0.628571428571429,-0.6,-0.571428571428572,-0.542857142857143,
-0.514285714285714,-0.485714285714286,-0.457142857142857,-0.428571428571429,
-0.4,-0.371428571428571,-0.342857142857143,-0.314285714285714,-0.285714285714286,
-0.257142857142857,-0.228571428571429,-0.2,-0.171428571428571,-0.142857142857143,
-0.114285714285714,-0.0857142857142857,-0.0571428571428571,-0.0285714285714286,
0.),(0.,1.6),.UNSPECIFIED.)
GEOMETRIC_REPRESENTATION_ITEM()
RATIONAL_B_SPLINE_SURFACE(((1.,1.),(1.,1.),(1.,1.),(1.,1.),(1.,1.),(1.,
1.),(1.,1.),(1.,1.),(1.,1.),(1.,1.),(1.,1.),(1.,1.),(1.,1.),(1.,1.),(1.,
1.),(1.,1.),(1.,1.),(1.,1.),(1.,1.),(1.,1.),(1.,1.),(1.,1.),(1.,1.),(1.,
1.),(1.,1.),(1.,1.),(1.,1.),(1.,1.),(1.,1.),(1.,1.),(1.,1.),(1.,1.),(1.,
1.),(1.,1.),(1.,1.),(1.,1.),(1.,1.),(1.,1.),(1.,1.),(1.,1.)))
REPRESENTATION_ITEM('')
SURFACE()
);
#518=(
BOUNDED_SURFACE()
B_SPLINE_SURFACE(5,1,((#45370,#45371),(#45372,#45373),(#45374,#45375),(#45376,
#45377),(#45378,#45379),(#45380,#45381),(#45382,#45383),(#45384,#45385),
(#45386,#45387),(#45388,#45389),(#45390,#45391),(#45392,#45393),(#45394,
#45395),(#45396,#45397),(#45398,#45399),(#45400,#45401),(#45402,#45403),
(#45404,#45405),(#45406,#45407),(#45408,#45409),(#45410,#45411),(#45412,
#45413),(#45414,#45415),(#45416,#45417),(#45418,#45419),(#45420,#45421),
(#45422,#45423),(#45424,#45425),(#45426,#45427),(#45428,#45429),(#45430,
#45431),(#45432,#45433),(#45434,#45435),(#45436,#45437),(#45438,#45439),
(#45440,#45441),(#45442,#45443),(#45444,#45445),(#45446,#45447),(#45448,
#45449)),.UNSPECIFIED.,.F.,.F.,.F.)
B_SPLINE_SURFACE_WITH_KNOTS((6,1,1,1,1,1,1,1,1,1,1,1,1,1,1,1,1,1,1,1,1,
1,1,1,1,1,1,1,1,1,1,1,1,1,1,6),(2,2),(-1.,-0.971428571428572,-0.942857142857143,
-0.914285714285714,-0.885714285714286,-0.857142857142857,-0.828571428571429,
-0.8,-0.771428571428572,-0.742857142857143,-0.714285714285714,-0.685714285714286,
-0.657142857142857,-0.628571428571429,-0.6,-0.571428571428572,-0.542857142857143,
-0.514285714285714,-0.485714285714286,-0.457142857142857,-0.428571428571429,
-0.4,-0.371428571428571,-0.342857142857143,-0.314285714285714,-0.285714285714286,
-0.257142857142857,-0.228571428571429,-0.2,-0.171428571428571,-0.142857142857143,
-0.114285714285714,-0.0857142857142857,-0.0571428571428571,-0.0285714285714286,
0.),(0.,1.6),.UNSPECIFIED.)
GEOMETRIC_REPRESENTATION_ITEM()
RATIONAL_B_SPLINE_SURFACE(((1.,1.),(1.,1.),(1.,1.),(1.,1.),(1.,1.),(1.,
1.),(1.,1.),(1.,1.),(1.,1.),(1.,1.),(1.,1.),(1.,1.),(1.,1.),(1.,1.),(1.,
1.),(1.,1.),(1.,1.),(1.,1.),(1.,1.),(1.,1.),(1.,1.),(1.,1.),(1.,1.),(1.,
1.),(1.,1.),(1.,1.),(1.,1.),(1.,1.),(1.,1.),(1.,1.),(1.,1.),(1.,1.),(1.,
1.),(1.,1.),(1.,1.),(1.,1.),(1.,1.),(1.,1.),(1.,1.),(1.,1.)))
REPRESENTATION_ITEM('')
SURFACE()
);
#519=(
BOUNDED_SURFACE()
B_SPLINE_SURFACE(5,1,((#45498,#45499),(#45500,#45501),(#45502,#45503),(#45504,
#45505),(#45506,#45507),(#45508,#45509),(#45510,#45511),(#45512,#45513),
(#45514,#45515),(#45516,#45517),(#45518,#45519),(#45520,#45521),(#45522,
#45523),(#45524,#45525),(#45526,#45527),(#45528,#45529),(#45530,#45531),
(#45532,#45533),(#45534,#45535),(#45536,#45537),(#45538,#45539),(#45540,
#45541),(#45542,#45543),(#45544,#45545),(#45546,#45547),(#45548,#45549),
(#45550,#45551),(#45552,#45553),(#45554,#45555),(#45556,#45557),(#45558,
#45559),(#45560,#45561),(#45562,#45563),(#45564,#45565),(#45566,#45567),
(#45568,#45569),(#45570,#45571),(#45572,#45573),(#45574,#45575),(#45576,
#45577)),.UNSPECIFIED.,.F.,.F.,.F.)
B_SPLINE_SURFACE_WITH_KNOTS((6,1,1,1,1,1,1,1,1,1,1,1,1,1,1,1,1,1,1,1,1,
1,1,1,1,1,1,1,1,1,1,1,1,1,1,6),(2,2),(-1.,-0.971428571428572,-0.942857142857143,
-0.914285714285714,-0.885714285714286,-0.857142857142857,-0.828571428571429,
-0.8,-0.771428571428572,-0.742857142857143,-0.714285714285714,-0.685714285714286,
-0.657142857142857,-0.628571428571429,-0.6,-0.571428571428572,-0.542857142857143,
-0.514285714285714,-0.485714285714286,-0.457142857142857,-0.428571428571429,
-0.4,-0.371428571428571,-0.342857142857143,-0.314285714285714,-0.285714285714286,
-0.257142857142857,-0.228571428571429,-0.2,-0.171428571428571,-0.142857142857143,
-0.114285714285714,-0.0857142857142857,-0.0571428571428571,-0.0285714285714286,
0.),(0.,1.6),.UNSPECIFIED.)
GEOMETRIC_REPRESENTATION_ITEM()
RATIONAL_B_SPLINE_SURFACE(((1.,1.),(1.,1.),(1.,1.),(1.,1.),(1.,1.),(1.,
1.),(1.,1.),(1.,1.),(1.,1.),(1.,1.),(1.,1.),(1.,1.),(1.,1.),(1.,1.),(1.,
1.),(1.,1.),(1.,1.),(1.,1.),(1.,1.),(1.,1.),(1.,1.),(1.,1.),(1.,1.),(1.,
1.),(1.,1.),(1.,1.),(1.,1.),(1.,1.),(1.,1.),(1.,1.),(1.,1.),(1.,1.),(1.,
1.),(1.,1.),(1.,1.),(1.,1.),(1.,1.),(1.,1.),(1.,1.),(1.,1.)))
REPRESENTATION_ITEM('')
SURFACE()
);
#520=(
BOUNDED_SURFACE()
B_SPLINE_SURFACE(5,1,((#45692,#45693),(#45694,#45695),(#45696,#45697),(#45698,
#45699),(#45700,#45701),(#45702,#45703),(#45704,#45705),(#45706,#45707),
(#45708,#45709),(#45710,#45711),(#45712,#45713),(#45714,#45715),(#45716,
#45717),(#45718,#45719),(#45720,#45721),(#45722,#45723),(#45724,#45725),
(#45726,#45727),(#45728,#45729),(#45730,#45731),(#45732,#45733),(#45734,
#45735),(#45736,#45737),(#45738,#45739),(#45740,#45741),(#45742,#45743),
(#45744,#45745),(#45746,#45747),(#45748,#45749),(#45750,#45751),(#45752,
#45753),(#45754,#45755),(#45756,#45757),(#45758,#45759),(#45760,#45761),
(#45762,#45763),(#45764,#45765),(#45766,#45767),(#45768,#45769),(#45770,
#45771)),.UNSPECIFIED.,.F.,.F.,.F.)
B_SPLINE_SURFACE_WITH_KNOTS((6,1,1,1,1,1,1,1,1,1,1,1,1,1,1,1,1,1,1,1,1,
1,1,1,1,1,1,1,1,1,1,1,1,1,1,6),(2,2),(-1.,-0.971428571428572,-0.942857142857143,
-0.914285714285714,-0.885714285714286,-0.857142857142857,-0.828571428571429,
-0.8,-0.771428571428572,-0.742857142857143,-0.714285714285714,-0.685714285714286,
-0.657142857142857,-0.628571428571429,-0.6,-0.571428571428572,-0.542857142857143,
-0.514285714285714,-0.485714285714286,-0.457142857142857,-0.428571428571429,
-0.4,-0.371428571428571,-0.342857142857143,-0.314285714285714,-0.285714285714286,
-0.257142857142857,-0.228571428571429,-0.2,-0.171428571428571,-0.142857142857143,
-0.114285714285714,-0.0857142857142857,-0.0571428571428571,-0.0285714285714286,
0.),(0.,1.6),.UNSPECIFIED.)
GEOMETRIC_REPRESENTATION_ITEM()
RATIONAL_B_SPLINE_SURFACE(((1.,1.),(1.,1.),(1.,1.),(1.,1.),(1.,1.),(1.,
1.),(1.,1.),(1.,1.),(1.,1.),(1.,1.),(1.,1.),(1.,1.),(1.,1.),(1.,1.),(1.,
1.),(1.,1.),(1.,1.),(1.,1.),(1.,1.),(1.,1.),(1.,1.),(1.,1.),(1.,1.),(1.,
1.),(1.,1.),(1.,1.),(1.,1.),(1.,1.),(1.,1.),(1.,1.),(1.,1.),(1.,1.),(1.,
1.),(1.,1.),(1.,1.),(1.,1.),(1.,1.),(1.,1.),(1.,1.),(1.,1.)))
REPRESENTATION_ITEM('')
SURFACE()
);
#521=(
BOUNDED_SURFACE()
B_SPLINE_SURFACE(5,1,((#45820,#45821),(#45822,#45823),(#45824,#45825),(#45826,
#45827),(#45828,#45829),(#45830,#45831),(#45832,#45833),(#45834,#45835),
(#45836,#45837),(#45838,#45839),(#45840,#45841),(#45842,#45843),(#45844,
#45845),(#45846,#45847),(#45848,#45849),(#45850,#45851),(#45852,#45853),
(#45854,#45855),(#45856,#45857),(#45858,#45859),(#45860,#45861),(#45862,
#45863),(#45864,#45865),(#45866,#45867),(#45868,#45869),(#45870,#45871),
(#45872,#45873),(#45874,#45875),(#45876,#45877),(#45878,#45879),(#45880,
#45881),(#45882,#45883),(#45884,#45885),(#45886,#45887),(#45888,#45889),
(#45890,#45891),(#45892,#45893),(#45894,#45895),(#45896,#45897),(#45898,
#45899)),.UNSPECIFIED.,.F.,.F.,.F.)
B_SPLINE_SURFACE_WITH_KNOTS((6,1,1,1,1,1,1,1,1,1,1,1,1,1,1,1,1,1,1,1,1,
1,1,1,1,1,1,1,1,1,1,1,1,1,1,6),(2,2),(-1.,-0.971428571428572,-0.942857142857143,
-0.914285714285714,-0.885714285714286,-0.857142857142857,-0.828571428571429,
-0.8,-0.771428571428572,-0.742857142857143,-0.714285714285714,-0.685714285714286,
-0.657142857142857,-0.628571428571429,-0.6,-0.571428571428572,-0.542857142857143,
-0.514285714285714,-0.485714285714286,-0.457142857142857,-0.428571428571429,
-0.4,-0.371428571428571,-0.342857142857143,-0.314285714285714,-0.285714285714286,
-0.257142857142857,-0.228571428571429,-0.2,-0.171428571428571,-0.142857142857143,
-0.114285714285714,-0.0857142857142857,-0.0571428571428571,-0.0285714285714286,
0.),(0.,1.6),.UNSPECIFIED.)
GEOMETRIC_REPRESENTATION_ITEM()
RATIONAL_B_SPLINE_SURFACE(((1.,1.),(1.,1.),(1.,1.),(1.,1.),(1.,1.),(1.,
1.),(1.,1.),(1.,1.),(1.,1.),(1.,1.),(1.,1.),(1.,1.),(1.,1.),(1.,1.),(1.,
1.),(1.,1.),(1.,1.),(1.,1.),(1.,1.),(1.,1.),(1.,1.),(1.,1.),(1.,1.),(1.,
1.),(1.,1.),(1.,1.),(1.,1.),(1.,1.),(1.,1.),(1.,1.),(1.,1.),(1.,1.),(1.,
1.),(1.,1.),(1.,1.),(1.,1.),(1.,1.),(1.,1.),(1.,1.),(1.,1.)))
REPRESENTATION_ITEM('')
SURFACE()
);
#522=(
BOUNDED_SURFACE()
B_SPLINE_SURFACE(5,1,((#46020,#46021),(#46022,#46023),(#46024,#46025),(#46026,
#46027),(#46028,#46029),(#46030,#46031),(#46032,#46033),(#46034,#46035),
(#46036,#46037),(#46038,#46039),(#46040,#46041),(#46042,#46043),(#46044,
#46045),(#46046,#46047),(#46048,#46049),(#46050,#46051),(#46052,#46053),
(#46054,#46055),(#46056,#46057),(#46058,#46059),(#46060,#46061),(#46062,
#46063),(#46064,#46065),(#46066,#46067),(#46068,#46069),(#46070,#46071),
(#46072,#46073),(#46074,#46075),(#46076,#46077),(#46078,#46079),(#46080,
#46081),(#46082,#46083),(#46084,#46085),(#46086,#46087),(#46088,#46089),
(#46090,#46091),(#46092,#46093),(#46094,#46095),(#46096,#46097),(#46098,
#46099)),.UNSPECIFIED.,.F.,.F.,.F.)
B_SPLINE_SURFACE_WITH_KNOTS((6,1,1,1,1,1,1,1,1,1,1,1,1,1,1,1,1,1,1,1,1,
1,1,1,1,1,1,1,1,1,1,1,1,1,1,6),(2,2),(-1.,-0.971428571428572,-0.942857142857143,
-0.914285714285714,-0.885714285714286,-0.857142857142857,-0.828571428571429,
-0.8,-0.771428571428572,-0.742857142857143,-0.714285714285714,-0.685714285714286,
-0.657142857142857,-0.628571428571429,-0.6,-0.571428571428572,-0.542857142857143,
-0.514285714285714,-0.485714285714286,-0.457142857142857,-0.428571428571429,
-0.4,-0.371428571428571,-0.342857142857143,-0.314285714285714,-0.285714285714286,
-0.257142857142857,-0.228571428571429,-0.2,-0.171428571428571,-0.142857142857143,
-0.114285714285714,-0.0857142857142857,-0.0571428571428571,-0.0285714285714286,
0.),(0.,1.6),.UNSPECIFIED.)
GEOMETRIC_REPRESENTATION_ITEM()
RATIONAL_B_SPLINE_SURFACE(((1.,1.),(1.,1.),(1.,1.),(1.,1.),(1.,1.),(1.,
1.),(1.,1.),(1.,1.),(1.,1.),(1.,1.),(1.,1.),(1.,1.),(1.,1.),(1.,1.),(1.,
1.),(1.,1.),(1.,1.),(1.,1.),(1.,1.),(1.,1.),(1.,1.),(1.,1.),(1.,1.),(1.,
1.),(1.,1.),(1.,1.),(1.,1.),(1.,1.),(1.,1.),(1.,1.),(1.,1.),(1.,1.),(1.,
1.),(1.,1.),(1.,1.),(1.,1.),(1.,1.),(1.,1.),(1.,1.),(1.,1.)))
REPRESENTATION_ITEM('')
SURFACE()
);
#523=(
BOUNDED_SURFACE()
B_SPLINE_SURFACE(5,1,((#46148,#46149),(#46150,#46151),(#46152,#46153),(#46154,
#46155),(#46156,#46157),(#46158,#46159),(#46160,#46161),(#46162,#46163),
(#46164,#46165),(#46166,#46167),(#46168,#46169),(#46170,#46171),(#46172,
#46173),(#46174,#46175),(#46176,#46177),(#46178,#46179),(#46180,#46181),
(#46182,#46183),(#46184,#46185),(#46186,#46187),(#46188,#46189),(#46190,
#46191),(#46192,#46193),(#46194,#46195),(#46196,#46197),(#46198,#46199),
(#46200,#46201),(#46202,#46203),(#46204,#46205),(#46206,#46207),(#46208,
#46209),(#46210,#46211),(#46212,#46213),(#46214,#46215),(#46216,#46217),
(#46218,#46219),(#46220,#46221),(#46222,#46223),(#46224,#46225),(#46226,
#46227)),.UNSPECIFIED.,.F.,.F.,.F.)
B_SPLINE_SURFACE_WITH_KNOTS((6,1,1,1,1,1,1,1,1,1,1,1,1,1,1,1,1,1,1,1,1,
1,1,1,1,1,1,1,1,1,1,1,1,1,1,6),(2,2),(-1.,-0.971428571428572,-0.942857142857143,
-0.914285714285714,-0.885714285714286,-0.857142857142857,-0.828571428571429,
-0.8,-0.771428571428572,-0.742857142857143,-0.714285714285714,-0.685714285714286,
-0.657142857142857,-0.628571428571429,-0.6,-0.571428571428572,-0.542857142857143,
-0.514285714285714,-0.485714285714286,-0.457142857142857,-0.428571428571429,
-0.4,-0.371428571428571,-0.342857142857143,-0.314285714285714,-0.285714285714286,
-0.257142857142857,-0.228571428571429,-0.2,-0.171428571428571,-0.142857142857143,
-0.114285714285714,-0.0857142857142857,-0.0571428571428571,-0.0285714285714286,
0.),(0.,1.6),.UNSPECIFIED.)
GEOMETRIC_REPRESENTATION_ITEM()
RATIONAL_B_SPLINE_SURFACE(((1.,1.),(1.,1.),(1.,1.),(1.,1.),(1.,1.),(1.,
1.),(1.,1.),(1.,1.),(1.,1.),(1.,1.),(1.,1.),(1.,1.),(1.,1.),(1.,1.),(1.,
1.),(1.,1.),(1.,1.),(1.,1.),(1.,1.),(1.,1.),(1.,1.),(1.,1.),(1.,1.),(1.,
1.),(1.,1.),(1.,1.),(1.,1.),(1.,1.),(1.,1.),(1.,1.),(1.,1.),(1.,1.),(1.,
1.),(1.,1.),(1.,1.),(1.,1.),(1.,1.),(1.,1.),(1.,1.),(1.,1.)))
REPRESENTATION_ITEM('')
SURFACE()
);
#524=(
BOUNDED_SURFACE()
B_SPLINE_SURFACE(5,1,((#46342,#46343),(#46344,#46345),(#46346,#46347),(#46348,
#46349),(#46350,#46351),(#46352,#46353),(#46354,#46355),(#46356,#46357),
(#46358,#46359),(#46360,#46361),(#46362,#46363),(#46364,#46365),(#46366,
#46367),(#46368,#46369),(#46370,#46371),(#46372,#46373),(#46374,#46375),
(#46376,#46377),(#46378,#46379),(#46380,#46381),(#46382,#46383),(#46384,
#46385),(#46386,#46387),(#46388,#46389),(#46390,#46391),(#46392,#46393),
(#46394,#46395),(#46396,#46397),(#46398,#46399),(#46400,#46401),(#46402,
#46403),(#46404,#46405),(#46406,#46407),(#46408,#46409),(#46410,#46411),
(#46412,#46413),(#46414,#46415),(#46416,#46417),(#46418,#46419),(#46420,
#46421)),.UNSPECIFIED.,.F.,.F.,.F.)
B_SPLINE_SURFACE_WITH_KNOTS((6,1,1,1,1,1,1,1,1,1,1,1,1,1,1,1,1,1,1,1,1,
1,1,1,1,1,1,1,1,1,1,1,1,1,1,6),(2,2),(-1.,-0.971428571428572,-0.942857142857143,
-0.914285714285714,-0.885714285714286,-0.857142857142857,-0.828571428571429,
-0.8,-0.771428571428572,-0.742857142857143,-0.714285714285714,-0.685714285714286,
-0.657142857142857,-0.628571428571429,-0.6,-0.571428571428572,-0.542857142857143,
-0.514285714285714,-0.485714285714286,-0.457142857142857,-0.428571428571429,
-0.4,-0.371428571428571,-0.342857142857143,-0.314285714285714,-0.285714285714286,
-0.257142857142857,-0.228571428571429,-0.2,-0.171428571428571,-0.142857142857143,
-0.114285714285714,-0.0857142857142857,-0.0571428571428571,-0.0285714285714286,
0.),(0.,1.6),.UNSPECIFIED.)
GEOMETRIC_REPRESENTATION_ITEM()
RATIONAL_B_SPLINE_SURFACE(((1.,1.),(1.,1.),(1.,1.),(1.,1.),(1.,1.),(1.,
1.),(1.,1.),(1.,1.),(1.,1.),(1.,1.),(1.,1.),(1.,1.),(1.,1.),(1.,1.),(1.,
1.),(1.,1.),(1.,1.),(1.,1.),(1.,1.),(1.,1.),(1.,1.),(1.,1.),(1.,1.),(1.,
1.),(1.,1.),(1.,1.),(1.,1.),(1.,1.),(1.,1.),(1.,1.),(1.,1.),(1.,1.),(1.,
1.),(1.,1.),(1.,1.),(1.,1.),(1.,1.),(1.,1.),(1.,1.),(1.,1.)))
REPRESENTATION_ITEM('')
SURFACE()
);
#525=(
BOUNDED_SURFACE()
B_SPLINE_SURFACE(5,1,((#46470,#46471),(#46472,#46473),(#46474,#46475),(#46476,
#46477),(#46478,#46479),(#46480,#46481),(#46482,#46483),(#46484,#46485),
(#46486,#46487),(#46488,#46489),(#46490,#46491),(#46492,#46493),(#46494,
#46495),(#46496,#46497),(#46498,#46499),(#46500,#46501),(#46502,#46503),
(#46504,#46505),(#46506,#46507),(#46508,#46509),(#46510,#46511),(#46512,
#46513),(#46514,#46515),(#46516,#46517),(#46518,#46519),(#46520,#46521),
(#46522,#46523),(#46524,#46525),(#46526,#46527),(#46528,#46529),(#46530,
#46531),(#46532,#46533),(#46534,#46535),(#46536,#46537),(#46538,#46539),
(#46540,#46541),(#46542,#46543),(#46544,#46545),(#46546,#46547),(#46548,
#46549)),.UNSPECIFIED.,.F.,.F.,.F.)
B_SPLINE_SURFACE_WITH_KNOTS((6,1,1,1,1,1,1,1,1,1,1,1,1,1,1,1,1,1,1,1,1,
1,1,1,1,1,1,1,1,1,1,1,1,1,1,6),(2,2),(-1.,-0.971428571428572,-0.942857142857143,
-0.914285714285714,-0.885714285714286,-0.857142857142857,-0.828571428571429,
-0.8,-0.771428571428572,-0.742857142857143,-0.714285714285714,-0.685714285714286,
-0.657142857142857,-0.628571428571429,-0.6,-0.571428571428572,-0.542857142857143,
-0.514285714285714,-0.485714285714286,-0.457142857142857,-0.428571428571429,
-0.4,-0.371428571428571,-0.342857142857143,-0.314285714285714,-0.285714285714286,
-0.257142857142857,-0.228571428571429,-0.2,-0.171428571428571,-0.142857142857143,
-0.114285714285714,-0.0857142857142857,-0.0571428571428571,-0.0285714285714286,
0.),(0.,1.6),.UNSPECIFIED.)
GEOMETRIC_REPRESENTATION_ITEM()
RATIONAL_B_SPLINE_SURFACE(((1.,1.),(1.,1.),(1.,1.),(1.,1.),(1.,1.),(1.,
1.),(1.,1.),(1.,1.),(1.,1.),(1.,1.),(1.,1.),(1.,1.),(1.,1.),(1.,1.),(1.,
1.),(1.,1.),(1.,1.),(1.,1.),(1.,1.),(1.,1.),(1.,1.),(1.,1.),(1.,1.),(1.,
1.),(1.,1.),(1.,1.),(1.,1.),(1.,1.),(1.,1.),(1.,1.),(1.,1.),(1.,1.),(1.,
1.),(1.,1.),(1.,1.),(1.,1.),(1.,1.),(1.,1.),(1.,1.),(1.,1.)))
REPRESENTATION_ITEM('')
SURFACE()
);
#526=(
BOUNDED_SURFACE()
B_SPLINE_SURFACE(5,1,((#46664,#46665),(#46666,#46667),(#46668,#46669),(#46670,
#46671),(#46672,#46673),(#46674,#46675),(#46676,#46677),(#46678,#46679),
(#46680,#46681),(#46682,#46683),(#46684,#46685),(#46686,#46687),(#46688,
#46689),(#46690,#46691),(#46692,#46693),(#46694,#46695),(#46696,#46697),
(#46698,#46699),(#46700,#46701),(#46702,#46703),(#46704,#46705),(#46706,
#46707),(#46708,#46709),(#46710,#46711),(#46712,#46713),(#46714,#46715),
(#46716,#46717),(#46718,#46719),(#46720,#46721),(#46722,#46723),(#46724,
#46725),(#46726,#46727),(#46728,#46729),(#46730,#46731),(#46732,#46733),
(#46734,#46735),(#46736,#46737),(#46738,#46739),(#46740,#46741),(#46742,
#46743)),.UNSPECIFIED.,.F.,.F.,.F.)
B_SPLINE_SURFACE_WITH_KNOTS((6,1,1,1,1,1,1,1,1,1,1,1,1,1,1,1,1,1,1,1,1,
1,1,1,1,1,1,1,1,1,1,1,1,1,1,6),(2,2),(-1.,-0.971428571428572,-0.942857142857143,
-0.914285714285714,-0.885714285714286,-0.857142857142857,-0.828571428571429,
-0.8,-0.771428571428572,-0.742857142857143,-0.714285714285714,-0.685714285714286,
-0.657142857142857,-0.628571428571429,-0.6,-0.571428571428572,-0.542857142857143,
-0.514285714285714,-0.485714285714286,-0.457142857142857,-0.428571428571429,
-0.4,-0.371428571428571,-0.342857142857143,-0.314285714285714,-0.285714285714286,
-0.257142857142857,-0.228571428571429,-0.2,-0.171428571428571,-0.142857142857143,
-0.114285714285714,-0.0857142857142857,-0.0571428571428571,-0.0285714285714286,
0.),(0.,1.6),.UNSPECIFIED.)
GEOMETRIC_REPRESENTATION_ITEM()
RATIONAL_B_SPLINE_SURFACE(((1.,1.),(1.,1.),(1.,1.),(1.,1.),(1.,1.),(1.,
1.),(1.,1.),(1.,1.),(1.,1.),(1.,1.),(1.,1.),(1.,1.),(1.,1.),(1.,1.),(1.,
1.),(1.,1.),(1.,1.),(1.,1.),(1.,1.),(1.,1.),(1.,1.),(1.,1.),(1.,1.),(1.,
1.),(1.,1.),(1.,1.),(1.,1.),(1.,1.),(1.,1.),(1.,1.),(1.,1.),(1.,1.),(1.,
1.),(1.,1.),(1.,1.),(1.,1.),(1.,1.),(1.,1.),(1.,1.),(1.,1.)))
REPRESENTATION_ITEM('')
SURFACE()
);
#527=(
BOUNDED_SURFACE()
B_SPLINE_SURFACE(5,1,((#46792,#46793),(#46794,#46795),(#46796,#46797),(#46798,
#46799),(#46800,#46801),(#46802,#46803),(#46804,#46805),(#46806,#46807),
(#46808,#46809),(#46810,#46811),(#46812,#46813),(#46814,#46815),(#46816,
#46817),(#46818,#46819),(#46820,#46821),(#46822,#46823),(#46824,#46825),
(#46826,#46827),(#46828,#46829),(#46830,#46831),(#46832,#46833),(#46834,
#46835),(#46836,#46837),(#46838,#46839),(#46840,#46841),(#46842,#46843),
(#46844,#46845),(#46846,#46847),(#46848,#46849),(#46850,#46851),(#46852,
#46853),(#46854,#46855),(#46856,#46857),(#46858,#46859),(#46860,#46861),
(#46862,#46863),(#46864,#46865),(#46866,#46867),(#46868,#46869),(#46870,
#46871)),.UNSPECIFIED.,.F.,.F.,.F.)
B_SPLINE_SURFACE_WITH_KNOTS((6,1,1,1,1,1,1,1,1,1,1,1,1,1,1,1,1,1,1,1,1,
1,1,1,1,1,1,1,1,1,1,1,1,1,1,6),(2,2),(-1.,-0.971428571428572,-0.942857142857143,
-0.914285714285714,-0.885714285714286,-0.857142857142857,-0.828571428571429,
-0.8,-0.771428571428572,-0.742857142857143,-0.714285714285714,-0.685714285714286,
-0.657142857142857,-0.628571428571429,-0.6,-0.571428571428572,-0.542857142857143,
-0.514285714285714,-0.485714285714286,-0.457142857142857,-0.428571428571429,
-0.4,-0.371428571428571,-0.342857142857143,-0.314285714285714,-0.285714285714286,
-0.257142857142857,-0.228571428571429,-0.2,-0.171428571428571,-0.142857142857143,
-0.114285714285714,-0.0857142857142857,-0.0571428571428571,-0.0285714285714286,
0.),(0.,1.6),.UNSPECIFIED.)
GEOMETRIC_REPRESENTATION_ITEM()
RATIONAL_B_SPLINE_SURFACE(((1.,1.),(1.,1.),(1.,1.),(1.,1.),(1.,1.),(1.,
1.),(1.,1.),(1.,1.),(1.,1.),(1.,1.),(1.,1.),(1.,1.),(1.,1.),(1.,1.),(1.,
1.),(1.,1.),(1.,1.),(1.,1.),(1.,1.),(1.,1.),(1.,1.),(1.,1.),(1.,1.),(1.,
1.),(1.,1.),(1.,1.),(1.,1.),(1.,1.),(1.,1.),(1.,1.),(1.,1.),(1.,1.),(1.,
1.),(1.,1.),(1.,1.),(1.,1.),(1.,1.),(1.,1.),(1.,1.),(1.,1.)))
REPRESENTATION_ITEM('')
SURFACE()
);
#528=(
BOUNDED_SURFACE()
B_SPLINE_SURFACE(5,1,((#46926,#46927),(#46928,#46929),(#46930,#46931),(#46932,
#46933),(#46934,#46935),(#46936,#46937),(#46938,#46939),(#46940,#46941),
(#46942,#46943),(#46944,#46945),(#46946,#46947),(#46948,#46949),(#46950,
#46951),(#46952,#46953),(#46954,#46955),(#46956,#46957),(#46958,#46959),
(#46960,#46961),(#46962,#46963),(#46964,#46965),(#46966,#46967),(#46968,
#46969),(#46970,#46971),(#46972,#46973),(#46974,#46975),(#46976,#46977),
(#46978,#46979),(#46980,#46981),(#46982,#46983),(#46984,#46985),(#46986,
#46987),(#46988,#46989),(#46990,#46991),(#46992,#46993),(#46994,#46995),
(#46996,#46997),(#46998,#46999),(#47000,#47001),(#47002,#47003),(#47004,
#47005)),.UNSPECIFIED.,.F.,.F.,.F.)
B_SPLINE_SURFACE_WITH_KNOTS((6,1,1,1,1,1,1,1,1,1,1,1,1,1,1,1,1,1,1,1,1,
1,1,1,1,1,1,1,1,1,1,1,1,1,1,6),(2,2),(-1.,-0.971428571428572,-0.942857142857143,
-0.914285714285714,-0.885714285714286,-0.857142857142857,-0.828571428571429,
-0.8,-0.771428571428572,-0.742857142857143,-0.714285714285714,-0.685714285714286,
-0.657142857142857,-0.628571428571429,-0.6,-0.571428571428572,-0.542857142857143,
-0.514285714285714,-0.485714285714286,-0.457142857142857,-0.428571428571429,
-0.4,-0.371428571428571,-0.342857142857143,-0.314285714285714,-0.285714285714286,
-0.257142857142857,-0.228571428571429,-0.2,-0.171428571428571,-0.142857142857143,
-0.114285714285714,-0.0857142857142857,-0.0571428571428571,-0.0285714285714286,
0.),(0.,1.6),.UNSPECIFIED.)
GEOMETRIC_REPRESENTATION_ITEM()
RATIONAL_B_SPLINE_SURFACE(((1.,1.),(1.,1.),(1.,1.),(1.,1.),(1.,1.),(1.,
1.),(1.,1.),(1.,1.),(1.,1.),(1.,1.),(1.,1.),(1.,1.),(1.,1.),(1.,1.),(1.,
1.),(1.,1.),(1.,1.),(1.,1.),(1.,1.),(1.,1.),(1.,1.),(1.,1.),(1.,1.),(1.,
1.),(1.,1.),(1.,1.),(1.,1.),(1.,1.),(1.,1.),(1.,1.),(1.,1.),(1.,1.),(1.,
1.),(1.,1.),(1.,1.),(1.,1.),(1.,1.),(1.,1.),(1.,1.),(1.,1.)))
REPRESENTATION_ITEM('')
SURFACE()
);
#529=(
BOUNDED_SURFACE()
B_SPLINE_SURFACE(5,1,((#47100,#47101),(#47102,#47103),(#47104,#47105),(#47106,
#47107),(#47108,#47109),(#47110,#47111),(#47112,#47113),(#47114,#47115),
(#47116,#47117),(#47118,#47119),(#47120,#47121),(#47122,#47123),(#47124,
#47125),(#47126,#47127),(#47128,#47129),(#47130,#47131),(#47132,#47133),
(#47134,#47135),(#47136,#47137),(#47138,#47139),(#47140,#47141),(#47142,
#47143),(#47144,#47145),(#47146,#47147),(#47148,#47149),(#47150,#47151),
(#47152,#47153),(#47154,#47155),(#47156,#47157),(#47158,#47159),(#47160,
#47161),(#47162,#47163),(#47164,#47165),(#47166,#47167),(#47168,#47169),
(#47170,#47171),(#47172,#47173),(#47174,#47175),(#47176,#47177),(#47178,
#47179)),.UNSPECIFIED.,.F.,.F.,.F.)
B_SPLINE_SURFACE_WITH_KNOTS((6,1,1,1,1,1,1,1,1,1,1,1,1,1,1,1,1,1,1,1,1,
1,1,1,1,1,1,1,1,1,1,1,1,1,1,6),(2,2),(-1.,-0.971428571428572,-0.942857142857143,
-0.914285714285714,-0.885714285714286,-0.857142857142857,-0.828571428571429,
-0.8,-0.771428571428572,-0.742857142857143,-0.714285714285714,-0.685714285714286,
-0.657142857142857,-0.628571428571429,-0.6,-0.571428571428572,-0.542857142857143,
-0.514285714285714,-0.485714285714286,-0.457142857142857,-0.428571428571429,
-0.4,-0.371428571428571,-0.342857142857143,-0.314285714285714,-0.285714285714286,
-0.257142857142857,-0.228571428571429,-0.2,-0.171428571428571,-0.142857142857143,
-0.114285714285714,-0.0857142857142857,-0.0571428571428571,-0.0285714285714286,
0.),(0.,1.6),.UNSPECIFIED.)
GEOMETRIC_REPRESENTATION_ITEM()
RATIONAL_B_SPLINE_SURFACE(((1.,1.),(1.,1.),(1.,1.),(1.,1.),(1.,1.),(1.,
1.),(1.,1.),(1.,1.),(1.,1.),(1.,1.),(1.,1.),(1.,1.),(1.,1.),(1.,1.),(1.,
1.),(1.,1.),(1.,1.),(1.,1.),(1.,1.),(1.,1.),(1.,1.),(1.,1.),(1.,1.),(1.,
1.),(1.,1.),(1.,1.),(1.,1.),(1.,1.),(1.,1.),(1.,1.),(1.,1.),(1.,1.),(1.,
1.),(1.,1.),(1.,1.),(1.,1.),(1.,1.),(1.,1.),(1.,1.),(1.,1.)))
REPRESENTATION_ITEM('')
SURFACE()
);
#608=(
BOUNDED_CURVE()
B_SPLINE_CURVE(5,(#42367,#42368,#42369,#42370,#42371,#42372,#42373,#42374,
#42375,#42376,#42377,#42378,#42379,#42380,#42381,#42382,#42383,#42384,#42385,
#42386,#42387,#42388,#42389,#42390,#42391,#42392,#42393,#42394,#42395),
 .UNSPECIFIED.,.F.,.F.)
B_SPLINE_CURVE_WITH_KNOTS((6,1,1,1,1,1,1,1,1,1,1,1,1,1,1,1,1,1,1,1,1,1,
1,1,6),(0.,0.0285714285714286,0.0571428571428571,0.0857142857142857,0.114285714285714,
0.142857142857143,0.171428571428571,0.2,0.228571428571429,0.257142857142857,
0.285714285714286,0.314285714285714,0.342857142857143,0.371428571428571,
0.4,0.428571428571429,0.457142857142857,0.485714285714286,0.514285714285714,
0.542857142857143,0.571428571428572,0.6,0.628571428571429,0.657142857142857,
0.667078900656917),.UNSPECIFIED.)
CURVE()
GEOMETRIC_REPRESENTATION_ITEM()
RATIONAL_B_SPLINE_CURVE((1.,1.,1.,1.,1.,1.,1.,1.,1.,1.,1.,1.,1.,1.,1.,1.,
1.,1.,1.,1.,1.,1.,1.,1.,1.,1.,1.,1.,1.))
REPRESENTATION_ITEM('')
);
#609=(
BOUNDED_CURVE()
B_SPLINE_CURVE(5,(#42398,#42399,#42400,#42401,#42402,#42403,#42404,#42405,
#42406,#42407,#42408,#42409,#42410,#42411,#42412,#42413,#42414,#42415,#42416,
#42417,#42418,#42419,#42420,#42421,#42422),.UNSPECIFIED.,.F.,.F.)
B_SPLINE_CURVE_WITH_KNOTS((6,1,1,1,1,1,1,1,1,1,1,1,1,1,1,1,1,1,1,1,6),(0.436331539942223,
0.457142857142857,0.485714285714286,0.514285714285714,0.542857142857143,
0.571428571428572,0.6,0.628571428571429,0.657142857142857,0.685714285714286,
0.714285714285714,0.742857142857143,0.771428571428572,0.8,0.828571428571429,
0.857142857142857,0.885714285714286,0.914285714285714,0.942857142857143,
0.971428571428572,1.),.UNSPECIFIED.)
CURVE()
GEOMETRIC_REPRESENTATION_ITEM()
RATIONAL_B_SPLINE_CURVE((1.,1.,1.,1.,1.,1.,1.,1.,1.,1.,1.,1.,1.,1.,1.,1.,
1.,1.,1.,1.,1.,1.,1.,1.,1.))
REPRESENTATION_ITEM('')
);
#610=(
BOUNDED_CURVE()
B_SPLINE_CURVE(5,(#42511,#42512,#42513,#42514,#42515,#42516,#42517,#42518,
#42519,#42520,#42521,#42522,#42523,#42524,#42525,#42526,#42527,#42528,#42529,
#42530,#42531,#42532,#42533,#42534,#42535),.UNSPECIFIED.,.F.,.F.)
B_SPLINE_CURVE_WITH_KNOTS((6,1,1,1,1,1,1,1,1,1,1,1,1,1,1,1,1,1,1,1,6),(-1.,
-0.971428571428572,-0.942857142857143,-0.914285714285714,-0.885714285714286,
-0.857142857142857,-0.828571428571429,-0.8,-0.771428571428572,-0.742857142857143,
-0.714285714285714,-0.685714285714286,-0.657142857142857,-0.628571428571429,
-0.6,-0.571428571428572,-0.542857142857143,-0.514285714285714,-0.485714285714286,
-0.457142857142857,-0.436331539942219),.UNSPECIFIED.)
CURVE()
GEOMETRIC_REPRESENTATION_ITEM()
RATIONAL_B_SPLINE_CURVE((1.,1.,1.,1.,1.,1.,1.,1.,1.,1.,1.,1.,1.,1.,1.,1.,
1.,1.,1.,1.,1.,1.,1.,1.,1.))
REPRESENTATION_ITEM('')
);
#611=(
BOUNDED_CURVE()
B_SPLINE_CURVE(5,(#42652,#42653,#42654,#42655,#42656,#42657,#42658,#42659,
#42660,#42661,#42662,#42663,#42664,#42665,#42666,#42667,#42668,#42669,#42670,
#42671,#42672,#42673,#42674,#42675,#42676,#42677,#42678,#42679,#42680),
 .UNSPECIFIED.,.F.,.F.)
B_SPLINE_CURVE_WITH_KNOTS((6,1,1,1,1,1,1,1,1,1,1,1,1,1,1,1,1,1,1,1,1,1,
1,1,6),(-0.667078900656922,-0.657142857142857,-0.628571428571429,-0.6,-0.571428571428572,
-0.542857142857143,-0.514285714285714,-0.485714285714286,-0.457142857142857,
-0.428571428571429,-0.4,-0.371428571428571,-0.342857142857143,-0.314285714285714,
-0.285714285714286,-0.257142857142857,-0.228571428571429,-0.2,-0.171428571428571,
-0.142857142857143,-0.114285714285714,-0.0857142857142857,-0.0571428571428571,
-0.0285714285714286,0.),.UNSPECIFIED.)
CURVE()
GEOMETRIC_REPRESENTATION_ITEM()
RATIONAL_B_SPLINE_CURVE((1.,1.,1.,1.,1.,1.,1.,1.,1.,1.,1.,1.,1.,1.,1.,1.,
1.,1.,1.,1.,1.,1.,1.,1.,1.,1.,1.,1.,1.))
REPRESENTATION_ITEM('')
);
#612=(
BOUNDED_CURVE()
B_SPLINE_CURVE(5,(#42719,#42720,#42721,#42722,#42723,#42724,#42725,#42726,
#42727,#42728,#42729,#42730,#42731,#42732,#42733,#42734,#42735,#42736,#42737,
#42738,#42739,#42740,#42741,#42742,#42743,#42744,#42745,#42746,#42747),
 .UNSPECIFIED.,.F.,.F.)
B_SPLINE_CURVE_WITH_KNOTS((6,1,1,1,1,1,1,1,1,1,1,1,1,1,1,1,1,1,1,1,1,1,
1,1,6),(0.,0.0285714285714286,0.0571428571428571,0.0857142857142857,0.114285714285714,
0.142857142857143,0.171428571428571,0.2,0.228571428571429,0.257142857142857,
0.285714285714286,0.314285714285714,0.342857142857143,0.371428571428571,
0.4,0.428571428571429,0.457142857142857,0.485714285714286,0.514285714285714,
0.542857142857143,0.571428571428572,0.6,0.628571428571429,0.657142857142857,
0.667078900656917),.UNSPECIFIED.)
CURVE()
GEOMETRIC_REPRESENTATION_ITEM()
RATIONAL_B_SPLINE_CURVE((1.,1.,1.,1.,1.,1.,1.,1.,1.,1.,1.,1.,1.,1.,1.,1.,
1.,1.,1.,1.,1.,1.,1.,1.,1.,1.,1.,1.,1.))
REPRESENTATION_ITEM('')
);
#613=(
BOUNDED_CURVE()
B_SPLINE_CURVE(5,(#42750,#42751,#42752,#42753,#42754,#42755,#42756,#42757,
#42758,#42759,#42760,#42761,#42762,#42763,#42764,#42765,#42766,#42767,#42768,
#42769,#42770,#42771,#42772,#42773,#42774),.UNSPECIFIED.,.F.,.F.)
B_SPLINE_CURVE_WITH_KNOTS((6,1,1,1,1,1,1,1,1,1,1,1,1,1,1,1,1,1,1,1,6),(0.436331539942223,
0.457142857142857,0.485714285714286,0.514285714285714,0.542857142857143,
0.571428571428572,0.6,0.628571428571429,0.657142857142857,0.685714285714286,
0.714285714285714,0.742857142857143,0.771428571428572,0.8,0.828571428571429,
0.857142857142857,0.885714285714286,0.914285714285714,0.942857142857143,
0.971428571428572,1.),.UNSPECIFIED.)
CURVE()
GEOMETRIC_REPRESENTATION_ITEM()
RATIONAL_B_SPLINE_CURVE((1.,1.,1.,1.,1.,1.,1.,1.,1.,1.,1.,1.,1.,1.,1.,1.,
1.,1.,1.,1.,1.,1.,1.,1.,1.))
REPRESENTATION_ITEM('')
);
#614=(
BOUNDED_CURVE()
B_SPLINE_CURVE(5,(#42863,#42864,#42865,#42866,#42867,#42868,#42869,#42870,
#42871,#42872,#42873,#42874,#42875,#42876,#42877,#42878,#42879,#42880,#42881,
#42882,#42883,#42884,#42885,#42886,#42887),.UNSPECIFIED.,.F.,.F.)
B_SPLINE_CURVE_WITH_KNOTS((6,1,1,1,1,1,1,1,1,1,1,1,1,1,1,1,1,1,1,1,6),(-1.,
-0.971428571428572,-0.942857142857143,-0.914285714285714,-0.885714285714286,
-0.857142857142857,-0.828571428571429,-0.8,-0.771428571428572,-0.742857142857143,
-0.714285714285714,-0.685714285714286,-0.657142857142857,-0.628571428571429,
-0.6,-0.571428571428572,-0.542857142857143,-0.514285714285714,-0.485714285714286,
-0.457142857142857,-0.436331539942219),.UNSPECIFIED.)
CURVE()
GEOMETRIC_REPRESENTATION_ITEM()
RATIONAL_B_SPLINE_CURVE((1.,1.,1.,1.,1.,1.,1.,1.,1.,1.,1.,1.,1.,1.,1.,1.,
1.,1.,1.,1.,1.,1.,1.,1.,1.))
REPRESENTATION_ITEM('')
);
#615=(
BOUNDED_CURVE()
B_SPLINE_CURVE(5,(#42983,#42984,#42985,#42986,#42987,#42988,#42989,#42990,
#42991,#42992,#42993,#42994,#42995,#42996,#42997,#42998,#42999,#43000,#43001,
#43002,#43003,#43004,#43005,#43006,#43007,#43008,#43009,#43010,#43011),
 .UNSPECIFIED.,.F.,.F.)
B_SPLINE_CURVE_WITH_KNOTS((6,1,1,1,1,1,1,1,1,1,1,1,1,1,1,1,1,1,1,1,1,1,
1,1,6),(-0.667078900656922,-0.657142857142857,-0.628571428571429,-0.6,-0.571428571428572,
-0.542857142857143,-0.514285714285714,-0.485714285714286,-0.457142857142857,
-0.428571428571429,-0.4,-0.371428571428571,-0.342857142857143,-0.314285714285714,
-0.285714285714286,-0.257142857142857,-0.228571428571429,-0.2,-0.171428571428571,
-0.142857142857143,-0.114285714285714,-0.0857142857142857,-0.0571428571428571,
-0.0285714285714286,0.),.UNSPECIFIED.)
CURVE()
GEOMETRIC_REPRESENTATION_ITEM()
RATIONAL_B_SPLINE_CURVE((1.,1.,1.,1.,1.,1.,1.,1.,1.,1.,1.,1.,1.,1.,1.,1.,
1.,1.,1.,1.,1.,1.,1.,1.,1.,1.,1.,1.,1.))
REPRESENTATION_ITEM('')
);
#616=(
BOUNDED_CURVE()
B_SPLINE_CURVE(5,(#43041,#43042,#43043,#43044,#43045,#43046,#43047,#43048,
#43049,#43050,#43051,#43052,#43053,#43054,#43055,#43056,#43057,#43058,#43059,
#43060,#43061,#43062,#43063,#43064,#43065,#43066,#43067,#43068,#43069),
 .UNSPECIFIED.,.F.,.F.)
B_SPLINE_CURVE_WITH_KNOTS((6,1,1,1,1,1,1,1,1,1,1,1,1,1,1,1,1,1,1,1,1,1,
1,1,6),(0.,0.0285714285714286,0.0571428571428571,0.0857142857142857,0.114285714285714,
0.142857142857143,0.171428571428571,0.2,0.228571428571429,0.257142857142857,
0.285714285714286,0.314285714285714,0.342857142857143,0.371428571428571,
0.4,0.428571428571429,0.457142857142857,0.485714285714286,0.514285714285714,
0.542857142857143,0.571428571428572,0.6,0.628571428571429,0.657142857142857,
0.667078900656917),.UNSPECIFIED.)
CURVE()
GEOMETRIC_REPRESENTATION_ITEM()
RATIONAL_B_SPLINE_CURVE((1.,1.,1.,1.,1.,1.,1.,1.,1.,1.,1.,1.,1.,1.,1.,1.,
1.,1.,1.,1.,1.,1.,1.,1.,1.,1.,1.,1.,1.))
REPRESENTATION_ITEM('')
);
#617=(
BOUNDED_CURVE()
B_SPLINE_CURVE(5,(#43072,#43073,#43074,#43075,#43076,#43077,#43078,#43079,
#43080,#43081,#43082,#43083,#43084,#43085,#43086,#43087,#43088,#43089,#43090,
#43091,#43092,#43093,#43094,#43095,#43096),.UNSPECIFIED.,.F.,.F.)
B_SPLINE_CURVE_WITH_KNOTS((6,1,1,1,1,1,1,1,1,1,1,1,1,1,1,1,1,1,1,1,6),(0.436331539942223,
0.457142857142857,0.485714285714286,0.514285714285714,0.542857142857143,
0.571428571428572,0.6,0.628571428571429,0.657142857142857,0.685714285714286,
0.714285714285714,0.742857142857143,0.771428571428572,0.8,0.828571428571429,
0.857142857142857,0.885714285714286,0.914285714285714,0.942857142857143,
0.971428571428572,1.),.UNSPECIFIED.)
CURVE()
GEOMETRIC_REPRESENTATION_ITEM()
RATIONAL_B_SPLINE_CURVE((1.,1.,1.,1.,1.,1.,1.,1.,1.,1.,1.,1.,1.,1.,1.,1.,
1.,1.,1.,1.,1.,1.,1.,1.,1.))
REPRESENTATION_ITEM('')
);
#618=(
BOUNDED_CURVE()
B_SPLINE_CURVE(5,(#43185,#43186,#43187,#43188,#43189,#43190,#43191,#43192,
#43193,#43194,#43195,#43196,#43197,#43198,#43199,#43200,#43201,#43202,#43203,
#43204,#43205,#43206,#43207,#43208,#43209),.UNSPECIFIED.,.F.,.F.)
B_SPLINE_CURVE_WITH_KNOTS((6,1,1,1,1,1,1,1,1,1,1,1,1,1,1,1,1,1,1,1,6),(-1.,
-0.971428571428572,-0.942857142857143,-0.914285714285714,-0.885714285714286,
-0.857142857142857,-0.828571428571429,-0.8,-0.771428571428572,-0.742857142857143,
-0.714285714285714,-0.685714285714286,-0.657142857142857,-0.628571428571429,
-0.6,-0.571428571428572,-0.542857142857143,-0.514285714285714,-0.485714285714286,
-0.457142857142857,-0.436331539942219),.UNSPECIFIED.)
CURVE()
GEOMETRIC_REPRESENTATION_ITEM()
RATIONAL_B_SPLINE_CURVE((1.,1.,1.,1.,1.,1.,1.,1.,1.,1.,1.,1.,1.,1.,1.,1.,
1.,1.,1.,1.,1.,1.,1.,1.,1.))
REPRESENTATION_ITEM('')
);
#619=(
BOUNDED_CURVE()
B_SPLINE_CURVE(5,(#43305,#43306,#43307,#43308,#43309,#43310,#43311,#43312,
#43313,#43314,#43315,#43316,#43317,#43318,#43319,#43320,#43321,#43322,#43323,
#43324,#43325,#43326,#43327,#43328,#43329,#43330,#43331,#43332,#43333),
 .UNSPECIFIED.,.F.,.F.)
B_SPLINE_CURVE_WITH_KNOTS((6,1,1,1,1,1,1,1,1,1,1,1,1,1,1,1,1,1,1,1,1,1,
1,1,6),(-0.667078900656922,-0.657142857142857,-0.628571428571429,-0.6,-0.571428571428572,
-0.542857142857143,-0.514285714285714,-0.485714285714286,-0.457142857142857,
-0.428571428571429,-0.4,-0.371428571428571,-0.342857142857143,-0.314285714285714,
-0.285714285714286,-0.257142857142857,-0.228571428571429,-0.2,-0.171428571428571,
-0.142857142857143,-0.114285714285714,-0.0857142857142857,-0.0571428571428571,
-0.0285714285714286,0.),.UNSPECIFIED.)
CURVE()
GEOMETRIC_REPRESENTATION_ITEM()
RATIONAL_B_SPLINE_CURVE((1.,1.,1.,1.,1.,1.,1.,1.,1.,1.,1.,1.,1.,1.,1.,1.,
1.,1.,1.,1.,1.,1.,1.,1.,1.,1.,1.,1.,1.))
REPRESENTATION_ITEM('')
);
#620=(
BOUNDED_CURVE()
B_SPLINE_CURVE(5,(#43363,#43364,#43365,#43366,#43367,#43368,#43369,#43370,
#43371,#43372,#43373,#43374,#43375,#43376,#43377,#43378,#43379,#43380,#43381,
#43382,#43383,#43384,#43385,#43386,#43387,#43388,#43389,#43390,#43391),
 .UNSPECIFIED.,.F.,.F.)
B_SPLINE_CURVE_WITH_KNOTS((6,1,1,1,1,1,1,1,1,1,1,1,1,1,1,1,1,1,1,1,1,1,
1,1,6),(0.,0.0285714285714286,0.0571428571428571,0.0857142857142857,0.114285714285714,
0.142857142857143,0.171428571428571,0.2,0.228571428571429,0.257142857142857,
0.285714285714286,0.314285714285714,0.342857142857143,0.371428571428571,
0.4,0.428571428571429,0.457142857142857,0.485714285714286,0.514285714285714,
0.542857142857143,0.571428571428572,0.6,0.628571428571429,0.657142857142857,
0.667078900656917),.UNSPECIFIED.)
CURVE()
GEOMETRIC_REPRESENTATION_ITEM()
RATIONAL_B_SPLINE_CURVE((1.,1.,1.,1.,1.,1.,1.,1.,1.,1.,1.,1.,1.,1.,1.,1.,
1.,1.,1.,1.,1.,1.,1.,1.,1.,1.,1.,1.,1.))
REPRESENTATION_ITEM('')
);
#621=(
BOUNDED_CURVE()
B_SPLINE_CURVE(5,(#43394,#43395,#43396,#43397,#43398,#43399,#43400,#43401,
#43402,#43403,#43404,#43405,#43406,#43407,#43408,#43409,#43410,#43411,#43412,
#43413,#43414,#43415,#43416,#43417,#43418),.UNSPECIFIED.,.F.,.F.)
B_SPLINE_CURVE_WITH_KNOTS((6,1,1,1,1,1,1,1,1,1,1,1,1,1,1,1,1,1,1,1,6),(0.436331539942223,
0.457142857142857,0.485714285714286,0.514285714285714,0.542857142857143,
0.571428571428572,0.6,0.628571428571429,0.657142857142857,0.685714285714286,
0.714285714285714,0.742857142857143,0.771428571428572,0.8,0.828571428571429,
0.857142857142857,0.885714285714286,0.914285714285714,0.942857142857143,
0.971428571428572,1.),.UNSPECIFIED.)
CURVE()
GEOMETRIC_REPRESENTATION_ITEM()
RATIONAL_B_SPLINE_CURVE((1.,1.,1.,1.,1.,1.,1.,1.,1.,1.,1.,1.,1.,1.,1.,1.,
1.,1.,1.,1.,1.,1.,1.,1.,1.))
REPRESENTATION_ITEM('')
);
#622=(
BOUNDED_CURVE()
B_SPLINE_CURVE(5,(#43507,#43508,#43509,#43510,#43511,#43512,#43513,#43514,
#43515,#43516,#43517,#43518,#43519,#43520,#43521,#43522,#43523,#43524,#43525,
#43526,#43527,#43528,#43529,#43530,#43531),.UNSPECIFIED.,.F.,.F.)
B_SPLINE_CURVE_WITH_KNOTS((6,1,1,1,1,1,1,1,1,1,1,1,1,1,1,1,1,1,1,1,6),(-1.,
-0.971428571428572,-0.942857142857143,-0.914285714285714,-0.885714285714286,
-0.857142857142857,-0.828571428571429,-0.8,-0.771428571428572,-0.742857142857143,
-0.714285714285714,-0.685714285714286,-0.657142857142857,-0.628571428571429,
-0.6,-0.571428571428572,-0.542857142857143,-0.514285714285714,-0.485714285714286,
-0.457142857142857,-0.436331539942219),.UNSPECIFIED.)
CURVE()
GEOMETRIC_REPRESENTATION_ITEM()
RATIONAL_B_SPLINE_CURVE((1.,1.,1.,1.,1.,1.,1.,1.,1.,1.,1.,1.,1.,1.,1.,1.,
1.,1.,1.,1.,1.,1.,1.,1.,1.))
REPRESENTATION_ITEM('')
);
#623=(
BOUNDED_CURVE()
B_SPLINE_CURVE(5,(#43627,#43628,#43629,#43630,#43631,#43632,#43633,#43634,
#43635,#43636,#43637,#43638,#43639,#43640,#43641,#43642,#43643,#43644,#43645,
#43646,#43647,#43648,#43649,#43650,#43651,#43652,#43653,#43654,#43655),
 .UNSPECIFIED.,.F.,.F.)
B_SPLINE_CURVE_WITH_KNOTS((6,1,1,1,1,1,1,1,1,1,1,1,1,1,1,1,1,1,1,1,1,1,
1,1,6),(-0.667078900656922,-0.657142857142857,-0.628571428571429,-0.6,-0.571428571428572,
-0.542857142857143,-0.514285714285714,-0.485714285714286,-0.457142857142857,
-0.428571428571429,-0.4,-0.371428571428571,-0.342857142857143,-0.314285714285714,
-0.285714285714286,-0.257142857142857,-0.228571428571429,-0.2,-0.171428571428571,
-0.142857142857143,-0.114285714285714,-0.0857142857142857,-0.0571428571428571,
-0.0285714285714286,0.),.UNSPECIFIED.)
CURVE()
GEOMETRIC_REPRESENTATION_ITEM()
RATIONAL_B_SPLINE_CURVE((1.,1.,1.,1.,1.,1.,1.,1.,1.,1.,1.,1.,1.,1.,1.,1.,
1.,1.,1.,1.,1.,1.,1.,1.,1.,1.,1.,1.,1.))
REPRESENTATION_ITEM('')
);
#624=(
BOUNDED_CURVE()
B_SPLINE_CURVE(5,(#43685,#43686,#43687,#43688,#43689,#43690,#43691,#43692,
#43693,#43694,#43695,#43696,#43697,#43698,#43699,#43700,#43701,#43702,#43703,
#43704,#43705,#43706,#43707,#43708,#43709,#43710,#43711,#43712,#43713),
 .UNSPECIFIED.,.F.,.F.)
B_SPLINE_CURVE_WITH_KNOTS((6,1,1,1,1,1,1,1,1,1,1,1,1,1,1,1,1,1,1,1,1,1,
1,1,6),(0.,0.0285714285714286,0.0571428571428571,0.0857142857142857,0.114285714285714,
0.142857142857143,0.171428571428571,0.2,0.228571428571429,0.257142857142857,
0.285714285714286,0.314285714285714,0.342857142857143,0.371428571428571,
0.4,0.428571428571429,0.457142857142857,0.485714285714286,0.514285714285714,
0.542857142857143,0.571428571428572,0.6,0.628571428571429,0.657142857142857,
0.667078900656917),.UNSPECIFIED.)
CURVE()
GEOMETRIC_REPRESENTATION_ITEM()
RATIONAL_B_SPLINE_CURVE((1.,1.,1.,1.,1.,1.,1.,1.,1.,1.,1.,1.,1.,1.,1.,1.,
1.,1.,1.,1.,1.,1.,1.,1.,1.,1.,1.,1.,1.))
REPRESENTATION_ITEM('')
);
#625=(
BOUNDED_CURVE()
B_SPLINE_CURVE(5,(#43716,#43717,#43718,#43719,#43720,#43721,#43722,#43723,
#43724,#43725,#43726,#43727,#43728,#43729,#43730,#43731,#43732,#43733,#43734,
#43735,#43736,#43737,#43738,#43739,#43740),.UNSPECIFIED.,.F.,.F.)
B_SPLINE_CURVE_WITH_KNOTS((6,1,1,1,1,1,1,1,1,1,1,1,1,1,1,1,1,1,1,1,6),(0.436331539942223,
0.457142857142857,0.485714285714286,0.514285714285714,0.542857142857143,
0.571428571428572,0.6,0.628571428571429,0.657142857142857,0.685714285714286,
0.714285714285714,0.742857142857143,0.771428571428572,0.8,0.828571428571429,
0.857142857142857,0.885714285714286,0.914285714285714,0.942857142857143,
0.971428571428572,1.),.UNSPECIFIED.)
CURVE()
GEOMETRIC_REPRESENTATION_ITEM()
RATIONAL_B_SPLINE_CURVE((1.,1.,1.,1.,1.,1.,1.,1.,1.,1.,1.,1.,1.,1.,1.,1.,
1.,1.,1.,1.,1.,1.,1.,1.,1.))
REPRESENTATION_ITEM('')
);
#626=(
BOUNDED_CURVE()
B_SPLINE_CURVE(5,(#43829,#43830,#43831,#43832,#43833,#43834,#43835,#43836,
#43837,#43838,#43839,#43840,#43841,#43842,#43843,#43844,#43845,#43846,#43847,
#43848,#43849,#43850,#43851,#43852,#43853),.UNSPECIFIED.,.F.,.F.)
B_SPLINE_CURVE_WITH_KNOTS((6,1,1,1,1,1,1,1,1,1,1,1,1,1,1,1,1,1,1,1,6),(-1.,
-0.971428571428572,-0.942857142857143,-0.914285714285714,-0.885714285714286,
-0.857142857142857,-0.828571428571429,-0.8,-0.771428571428572,-0.742857142857143,
-0.714285714285714,-0.685714285714286,-0.657142857142857,-0.628571428571429,
-0.6,-0.571428571428572,-0.542857142857143,-0.514285714285714,-0.485714285714286,
-0.457142857142857,-0.436331539942219),.UNSPECIFIED.)
CURVE()
GEOMETRIC_REPRESENTATION_ITEM()
RATIONAL_B_SPLINE_CURVE((1.,1.,1.,1.,1.,1.,1.,1.,1.,1.,1.,1.,1.,1.,1.,1.,
1.,1.,1.,1.,1.,1.,1.,1.,1.))
REPRESENTATION_ITEM('')
);
#627=(
BOUNDED_CURVE()
B_SPLINE_CURVE(5,(#43962,#43963,#43964,#43965,#43966,#43967,#43968,#43969,
#43970,#43971,#43972,#43973,#43974,#43975,#43976,#43977,#43978,#43979,#43980,
#43981,#43982,#43983,#43984,#43985,#43986,#43987,#43988,#43989,#43990),
 .UNSPECIFIED.,.F.,.F.)
B_SPLINE_CURVE_WITH_KNOTS((6,1,1,1,1,1,1,1,1,1,1,1,1,1,1,1,1,1,1,1,1,1,
1,1,6),(-0.667078900656922,-0.657142857142857,-0.628571428571429,-0.6,-0.571428571428572,
-0.542857142857143,-0.514285714285714,-0.485714285714286,-0.457142857142857,
-0.428571428571429,-0.4,-0.371428571428571,-0.342857142857143,-0.314285714285714,
-0.285714285714286,-0.257142857142857,-0.228571428571429,-0.2,-0.171428571428571,
-0.142857142857143,-0.114285714285714,-0.0857142857142857,-0.0571428571428571,
-0.0285714285714286,0.),.UNSPECIFIED.)
CURVE()
GEOMETRIC_REPRESENTATION_ITEM()
RATIONAL_B_SPLINE_CURVE((1.,1.,1.,1.,1.,1.,1.,1.,1.,1.,1.,1.,1.,1.,1.,1.,
1.,1.,1.,1.,1.,1.,1.,1.,1.,1.,1.,1.,1.))
REPRESENTATION_ITEM('')
);
#628=(
BOUNDED_CURVE()
B_SPLINE_CURVE(5,(#44020,#44021,#44022,#44023,#44024,#44025,#44026,#44027,
#44028,#44029,#44030,#44031,#44032,#44033,#44034,#44035,#44036,#44037,#44038,
#44039,#44040,#44041,#44042,#44043,#44044,#44045,#44046,#44047,#44048),
 .UNSPECIFIED.,.F.,.F.)
B_SPLINE_CURVE_WITH_KNOTS((6,1,1,1,1,1,1,1,1,1,1,1,1,1,1,1,1,1,1,1,1,1,
1,1,6),(0.,0.0285714285714286,0.0571428571428571,0.0857142857142857,0.114285714285714,
0.142857142857143,0.171428571428571,0.2,0.228571428571429,0.257142857142857,
0.285714285714286,0.314285714285714,0.342857142857143,0.371428571428571,
0.4,0.428571428571429,0.457142857142857,0.485714285714286,0.514285714285714,
0.542857142857143,0.571428571428572,0.6,0.628571428571429,0.657142857142857,
0.667078900656916),.UNSPECIFIED.)
CURVE()
GEOMETRIC_REPRESENTATION_ITEM()
RATIONAL_B_SPLINE_CURVE((1.,1.,1.,1.,1.,1.,1.,1.,1.,1.,1.,1.,1.,1.,1.,1.,
1.,1.,1.,1.,1.,1.,1.,1.,1.,1.,1.,1.,1.))
REPRESENTATION_ITEM('')
);
#629=(
BOUNDED_CURVE()
B_SPLINE_CURVE(5,(#44051,#44052,#44053,#44054,#44055,#44056,#44057,#44058,
#44059,#44060,#44061,#44062,#44063,#44064,#44065,#44066,#44067,#44068,#44069,
#44070,#44071,#44072,#44073,#44074,#44075),.UNSPECIFIED.,.F.,.F.)
B_SPLINE_CURVE_WITH_KNOTS((6,1,1,1,1,1,1,1,1,1,1,1,1,1,1,1,1,1,1,1,6),(0.436331539942223,
0.457142857142857,0.485714285714286,0.514285714285714,0.542857142857143,
0.571428571428572,0.6,0.628571428571429,0.657142857142857,0.685714285714286,
0.714285714285714,0.742857142857143,0.771428571428572,0.8,0.828571428571429,
0.857142857142857,0.885714285714286,0.914285714285714,0.942857142857143,
0.971428571428572,1.),.UNSPECIFIED.)
CURVE()
GEOMETRIC_REPRESENTATION_ITEM()
RATIONAL_B_SPLINE_CURVE((1.,1.,1.,1.,1.,1.,1.,1.,1.,1.,1.,1.,1.,1.,1.,1.,
1.,1.,1.,1.,1.,1.,1.,1.,1.))
REPRESENTATION_ITEM('')
);
#630=(
BOUNDED_CURVE()
B_SPLINE_CURVE(5,(#44164,#44165,#44166,#44167,#44168,#44169,#44170,#44171,
#44172,#44173,#44174,#44175,#44176,#44177,#44178,#44179,#44180,#44181,#44182,
#44183,#44184,#44185,#44186,#44187,#44188),.UNSPECIFIED.,.F.,.F.)
B_SPLINE_CURVE_WITH_KNOTS((6,1,1,1,1,1,1,1,1,1,1,1,1,1,1,1,1,1,1,1,6),(-1.,
-0.971428571428572,-0.942857142857143,-0.914285714285714,-0.885714285714286,
-0.857142857142857,-0.828571428571429,-0.8,-0.771428571428572,-0.742857142857143,
-0.714285714285714,-0.685714285714286,-0.657142857142857,-0.628571428571429,
-0.6,-0.571428571428572,-0.542857142857143,-0.514285714285714,-0.485714285714286,
-0.457142857142857,-0.436331539942219),.UNSPECIFIED.)
CURVE()
GEOMETRIC_REPRESENTATION_ITEM()
RATIONAL_B_SPLINE_CURVE((1.,1.,1.,1.,1.,1.,1.,1.,1.,1.,1.,1.,1.,1.,1.,1.,
1.,1.,1.,1.,1.,1.,1.,1.,1.))
REPRESENTATION_ITEM('')
);
#631=(
BOUNDED_CURVE()
B_SPLINE_CURVE(5,(#44284,#44285,#44286,#44287,#44288,#44289,#44290,#44291,
#44292,#44293,#44294,#44295,#44296,#44297,#44298,#44299,#44300,#44301,#44302,
#44303,#44304,#44305,#44306,#44307,#44308,#44309,#44310,#44311,#44312),
 .UNSPECIFIED.,.F.,.F.)
B_SPLINE_CURVE_WITH_KNOTS((6,1,1,1,1,1,1,1,1,1,1,1,1,1,1,1,1,1,1,1,1,1,
1,1,6),(-0.667078900656921,-0.657142857142857,-0.628571428571429,-0.6,-0.571428571428572,
-0.542857142857143,-0.514285714285714,-0.485714285714286,-0.457142857142857,
-0.428571428571429,-0.4,-0.371428571428571,-0.342857142857143,-0.314285714285714,
-0.285714285714286,-0.257142857142857,-0.228571428571429,-0.2,-0.171428571428571,
-0.142857142857143,-0.114285714285714,-0.0857142857142857,-0.0571428571428571,
-0.0285714285714286,0.),.UNSPECIFIED.)
CURVE()
GEOMETRIC_REPRESENTATION_ITEM()
RATIONAL_B_SPLINE_CURVE((1.,1.,1.,1.,1.,1.,1.,1.,1.,1.,1.,1.,1.,1.,1.,1.,
1.,1.,1.,1.,1.,1.,1.,1.,1.,1.,1.,1.,1.))
REPRESENTATION_ITEM('')
);
#632=(
BOUNDED_CURVE()
B_SPLINE_CURVE(5,(#44342,#44343,#44344,#44345,#44346,#44347,#44348,#44349,
#44350,#44351,#44352,#44353,#44354,#44355,#44356,#44357,#44358,#44359,#44360,
#44361,#44362,#44363,#44364,#44365,#44366,#44367,#44368,#44369,#44370),
 .UNSPECIFIED.,.F.,.F.)
B_SPLINE_CURVE_WITH_KNOTS((6,1,1,1,1,1,1,1,1,1,1,1,1,1,1,1,1,1,1,1,1,1,
1,1,6),(0.,0.0285714285714286,0.0571428571428571,0.0857142857142857,0.114285714285714,
0.142857142857143,0.171428571428571,0.2,0.228571428571429,0.257142857142857,
0.285714285714286,0.314285714285714,0.342857142857143,0.371428571428571,
0.4,0.428571428571429,0.457142857142857,0.485714285714286,0.514285714285714,
0.542857142857143,0.571428571428572,0.6,0.628571428571429,0.657142857142857,
0.667078900656917),.UNSPECIFIED.)
CURVE()
GEOMETRIC_REPRESENTATION_ITEM()
RATIONAL_B_SPLINE_CURVE((1.,1.,1.,1.,1.,1.,1.,1.,1.,1.,1.,1.,1.,1.,1.,1.,
1.,1.,1.,1.,1.,1.,1.,1.,1.,1.,1.,1.,1.))
REPRESENTATION_ITEM('')
);
#633=(
BOUNDED_CURVE()
B_SPLINE_CURVE(5,(#44373,#44374,#44375,#44376,#44377,#44378,#44379,#44380,
#44381,#44382,#44383,#44384,#44385,#44386,#44387,#44388,#44389,#44390,#44391,
#44392,#44393,#44394,#44395,#44396,#44397),.UNSPECIFIED.,.F.,.F.)
B_SPLINE_CURVE_WITH_KNOTS((6,1,1,1,1,1,1,1,1,1,1,1,1,1,1,1,1,1,1,1,6),(0.436331539942223,
0.457142857142857,0.485714285714286,0.514285714285714,0.542857142857143,
0.571428571428572,0.6,0.628571428571429,0.657142857142857,0.685714285714286,
0.714285714285714,0.742857142857143,0.771428571428572,0.8,0.828571428571429,
0.857142857142857,0.885714285714286,0.914285714285714,0.942857142857143,
0.971428571428572,1.),.UNSPECIFIED.)
CURVE()
GEOMETRIC_REPRESENTATION_ITEM()
RATIONAL_B_SPLINE_CURVE((1.,1.,1.,1.,1.,1.,1.,1.,1.,1.,1.,1.,1.,1.,1.,1.,
1.,1.,1.,1.,1.,1.,1.,1.,1.))
REPRESENTATION_ITEM('')
);
#634=(
BOUNDED_CURVE()
B_SPLINE_CURVE(5,(#44486,#44487,#44488,#44489,#44490,#44491,#44492,#44493,
#44494,#44495,#44496,#44497,#44498,#44499,#44500,#44501,#44502,#44503,#44504,
#44505,#44506,#44507,#44508,#44509,#44510),.UNSPECIFIED.,.F.,.F.)
B_SPLINE_CURVE_WITH_KNOTS((6,1,1,1,1,1,1,1,1,1,1,1,1,1,1,1,1,1,1,1,6),(-1.,
-0.971428571428572,-0.942857142857143,-0.914285714285714,-0.885714285714286,
-0.857142857142857,-0.828571428571429,-0.8,-0.771428571428572,-0.742857142857143,
-0.714285714285714,-0.685714285714286,-0.657142857142857,-0.628571428571429,
-0.6,-0.571428571428572,-0.542857142857143,-0.514285714285714,-0.485714285714286,
-0.457142857142857,-0.436331539942219),.UNSPECIFIED.)
CURVE()
GEOMETRIC_REPRESENTATION_ITEM()
RATIONAL_B_SPLINE_CURVE((1.,1.,1.,1.,1.,1.,1.,1.,1.,1.,1.,1.,1.,1.,1.,1.,
1.,1.,1.,1.,1.,1.,1.,1.,1.))
REPRESENTATION_ITEM('')
);
#635=(
BOUNDED_CURVE()
B_SPLINE_CURVE(5,(#44606,#44607,#44608,#44609,#44610,#44611,#44612,#44613,
#44614,#44615,#44616,#44617,#44618,#44619,#44620,#44621,#44622,#44623,#44624,
#44625,#44626,#44627,#44628,#44629,#44630,#44631,#44632,#44633,#44634),
 .UNSPECIFIED.,.F.,.F.)
B_SPLINE_CURVE_WITH_KNOTS((6,1,1,1,1,1,1,1,1,1,1,1,1,1,1,1,1,1,1,1,1,1,
1,1,6),(-0.667078900656922,-0.657142857142857,-0.628571428571429,-0.6,-0.571428571428572,
-0.542857142857143,-0.514285714285714,-0.485714285714286,-0.457142857142857,
-0.428571428571429,-0.4,-0.371428571428571,-0.342857142857143,-0.314285714285714,
-0.285714285714286,-0.257142857142857,-0.228571428571429,-0.2,-0.171428571428571,
-0.142857142857143,-0.114285714285714,-0.0857142857142857,-0.0571428571428571,
-0.0285714285714286,0.),.UNSPECIFIED.)
CURVE()
GEOMETRIC_REPRESENTATION_ITEM()
RATIONAL_B_SPLINE_CURVE((1.,1.,1.,1.,1.,1.,1.,1.,1.,1.,1.,1.,1.,1.,1.,1.,
1.,1.,1.,1.,1.,1.,1.,1.,1.,1.,1.,1.,1.))
REPRESENTATION_ITEM('')
);
#636=(
BOUNDED_CURVE()
B_SPLINE_CURVE(5,(#44666,#44667,#44668,#44669,#44670,#44671,#44672,#44673,
#44674,#44675,#44676,#44677,#44678,#44679,#44680,#44681,#44682,#44683,#44684,
#44685,#44686,#44687,#44688,#44689,#44690,#44691,#44692,#44693,#44694),
 .UNSPECIFIED.,.F.,.F.)
B_SPLINE_CURVE_WITH_KNOTS((6,1,1,1,1,1,1,1,1,1,1,1,1,1,1,1,1,1,1,1,1,1,
1,1,6),(0.,0.0285714285714286,0.0571428571428571,0.0857142857142857,0.114285714285714,
0.142857142857143,0.171428571428571,0.2,0.228571428571429,0.257142857142857,
0.285714285714286,0.314285714285714,0.342857142857143,0.371428571428571,
0.4,0.428571428571429,0.457142857142857,0.485714285714286,0.514285714285714,
0.542857142857143,0.571428571428572,0.6,0.628571428571429,0.657142857142857,
0.667078900656917),.UNSPECIFIED.)
CURVE()
GEOMETRIC_REPRESENTATION_ITEM()
RATIONAL_B_SPLINE_CURVE((1.,1.,1.,1.,1.,1.,1.,1.,1.,1.,1.,1.,1.,1.,1.,1.,
1.,1.,1.,1.,1.,1.,1.,1.,1.,1.,1.,1.,1.))
REPRESENTATION_ITEM('')
);
#637=(
BOUNDED_CURVE()
B_SPLINE_CURVE(5,(#44697,#44698,#44699,#44700,#44701,#44702,#44703,#44704,
#44705,#44706,#44707,#44708,#44709,#44710,#44711,#44712,#44713,#44714,#44715,
#44716,#44717,#44718,#44719,#44720,#44721),.UNSPECIFIED.,.F.,.F.)
B_SPLINE_CURVE_WITH_KNOTS((6,1,1,1,1,1,1,1,1,1,1,1,1,1,1,1,1,1,1,1,6),(0.436331539942224,
0.457142857142857,0.485714285714286,0.514285714285714,0.542857142857143,
0.571428571428572,0.6,0.628571428571429,0.657142857142857,0.685714285714286,
0.714285714285714,0.742857142857143,0.771428571428572,0.8,0.828571428571429,
0.857142857142857,0.885714285714286,0.914285714285714,0.942857142857143,
0.971428571428572,1.),.UNSPECIFIED.)
CURVE()
GEOMETRIC_REPRESENTATION_ITEM()
RATIONAL_B_SPLINE_CURVE((1.,1.,1.,1.,1.,1.,1.,1.,1.,1.,1.,1.,1.,1.,1.,1.,
1.,1.,1.,1.,1.,1.,1.,1.,1.))
REPRESENTATION_ITEM('')
);
#638=(
BOUNDED_CURVE()
B_SPLINE_CURVE(5,(#44812,#44813,#44814,#44815,#44816,#44817,#44818,#44819,
#44820,#44821,#44822,#44823,#44824,#44825,#44826,#44827,#44828,#44829,#44830,
#44831,#44832,#44833,#44834,#44835,#44836),.UNSPECIFIED.,.F.,.F.)
B_SPLINE_CURVE_WITH_KNOTS((6,1,1,1,1,1,1,1,1,1,1,1,1,1,1,1,1,1,1,1,6),(-1.,
-0.971428571428572,-0.942857142857143,-0.914285714285714,-0.885714285714286,
-0.857142857142857,-0.828571428571429,-0.8,-0.771428571428572,-0.742857142857143,
-0.714285714285714,-0.685714285714286,-0.657142857142857,-0.628571428571429,
-0.6,-0.571428571428572,-0.542857142857143,-0.514285714285714,-0.485714285714286,
-0.457142857142857,-0.43633153994222),.UNSPECIFIED.)
CURVE()
GEOMETRIC_REPRESENTATION_ITEM()
RATIONAL_B_SPLINE_CURVE((1.,1.,1.,1.,1.,1.,1.,1.,1.,1.,1.,1.,1.,1.,1.,1.,
1.,1.,1.,1.,1.,1.,1.,1.,1.))
REPRESENTATION_ITEM('')
);
#639=(
BOUNDED_CURVE()
B_SPLINE_CURVE(5,(#44932,#44933,#44934,#44935,#44936,#44937,#44938,#44939,
#44940,#44941,#44942,#44943,#44944,#44945,#44946,#44947,#44948,#44949,#44950,
#44951,#44952,#44953,#44954,#44955,#44956,#44957,#44958,#44959,#44960),
 .UNSPECIFIED.,.F.,.F.)
B_SPLINE_CURVE_WITH_KNOTS((6,1,1,1,1,1,1,1,1,1,1,1,1,1,1,1,1,1,1,1,1,1,
1,1,6),(-0.667078900656922,-0.657142857142857,-0.628571428571429,-0.6,-0.571428571428572,
-0.542857142857143,-0.514285714285714,-0.485714285714286,-0.457142857142857,
-0.428571428571429,-0.4,-0.371428571428571,-0.342857142857143,-0.314285714285714,
-0.285714285714286,-0.257142857142857,-0.228571428571429,-0.2,-0.171428571428571,
-0.142857142857143,-0.114285714285714,-0.0857142857142857,-0.0571428571428571,
-0.0285714285714286,0.),.UNSPECIFIED.)
CURVE()
GEOMETRIC_REPRESENTATION_ITEM()
RATIONAL_B_SPLINE_CURVE((1.,1.,1.,1.,1.,1.,1.,1.,1.,1.,1.,1.,1.,1.,1.,1.,
1.,1.,1.,1.,1.,1.,1.,1.,1.,1.,1.,1.,1.))
REPRESENTATION_ITEM('')
);
#640=(
BOUNDED_CURVE()
B_SPLINE_CURVE(5,(#44992,#44993,#44994,#44995,#44996,#44997,#44998,#44999,
#45000,#45001,#45002,#45003,#45004,#45005,#45006,#45007,#45008,#45009,#45010,
#45011,#45012,#45013,#45014,#45015,#45016,#45017,#45018,#45019,#45020),
 .UNSPECIFIED.,.F.,.F.)
B_SPLINE_CURVE_WITH_KNOTS((6,1,1,1,1,1,1,1,1,1,1,1,1,1,1,1,1,1,1,1,1,1,
1,1,6),(0.,0.0285714285714286,0.0571428571428571,0.0857142857142857,0.114285714285714,
0.142857142857143,0.171428571428571,0.2,0.228571428571429,0.257142857142857,
0.285714285714286,0.314285714285714,0.342857142857143,0.371428571428571,
0.4,0.428571428571429,0.457142857142857,0.485714285714286,0.514285714285714,
0.542857142857143,0.571428571428572,0.6,0.628571428571429,0.657142857142857,
0.667078900656917),.UNSPECIFIED.)
CURVE()
GEOMETRIC_REPRESENTATION_ITEM()
RATIONAL_B_SPLINE_CURVE((1.,1.,1.,1.,1.,1.,1.,1.,1.,1.,1.,1.,1.,1.,1.,1.,
1.,1.,1.,1.,1.,1.,1.,1.,1.,1.,1.,1.,1.))
REPRESENTATION_ITEM('')
);
#641=(
BOUNDED_CURVE()
B_SPLINE_CURVE(5,(#45023,#45024,#45025,#45026,#45027,#45028,#45029,#45030,
#45031,#45032,#45033,#45034,#45035,#45036,#45037,#45038,#45039,#45040,#45041,
#45042,#45043,#45044,#45045,#45046,#45047),.UNSPECIFIED.,.F.,.F.)
B_SPLINE_CURVE_WITH_KNOTS((6,1,1,1,1,1,1,1,1,1,1,1,1,1,1,1,1,1,1,1,6),(0.436331539942223,
0.457142857142857,0.485714285714286,0.514285714285714,0.542857142857143,
0.571428571428572,0.6,0.628571428571429,0.657142857142857,0.685714285714286,
0.714285714285714,0.742857142857143,0.771428571428572,0.8,0.828571428571429,
0.857142857142857,0.885714285714286,0.914285714285714,0.942857142857143,
0.971428571428572,1.),.UNSPECIFIED.)
CURVE()
GEOMETRIC_REPRESENTATION_ITEM()
RATIONAL_B_SPLINE_CURVE((1.,1.,1.,1.,1.,1.,1.,1.,1.,1.,1.,1.,1.,1.,1.,1.,
1.,1.,1.,1.,1.,1.,1.,1.,1.))
REPRESENTATION_ITEM('')
);
#642=(
BOUNDED_CURVE()
B_SPLINE_CURVE(5,(#45136,#45137,#45138,#45139,#45140,#45141,#45142,#45143,
#45144,#45145,#45146,#45147,#45148,#45149,#45150,#45151,#45152,#45153,#45154,
#45155,#45156,#45157,#45158,#45159,#45160),.UNSPECIFIED.,.F.,.F.)
B_SPLINE_CURVE_WITH_KNOTS((6,1,1,1,1,1,1,1,1,1,1,1,1,1,1,1,1,1,1,1,6),(-1.,
-0.971428571428572,-0.942857142857143,-0.914285714285714,-0.885714285714286,
-0.857142857142857,-0.828571428571429,-0.8,-0.771428571428572,-0.742857142857143,
-0.714285714285714,-0.685714285714286,-0.657142857142857,-0.628571428571429,
-0.6,-0.571428571428572,-0.542857142857143,-0.514285714285714,-0.485714285714286,
-0.457142857142857,-0.436331539942219),.UNSPECIFIED.)
CURVE()
GEOMETRIC_REPRESENTATION_ITEM()
RATIONAL_B_SPLINE_CURVE((1.,1.,1.,1.,1.,1.,1.,1.,1.,1.,1.,1.,1.,1.,1.,1.,
1.,1.,1.,1.,1.,1.,1.,1.,1.))
REPRESENTATION_ITEM('')
);
#643=(
BOUNDED_CURVE()
B_SPLINE_CURVE(5,(#45256,#45257,#45258,#45259,#45260,#45261,#45262,#45263,
#45264,#45265,#45266,#45267,#45268,#45269,#45270,#45271,#45272,#45273,#45274,
#45275,#45276,#45277,#45278,#45279,#45280,#45281,#45282,#45283,#45284),
 .UNSPECIFIED.,.F.,.F.)
B_SPLINE_CURVE_WITH_KNOTS((6,1,1,1,1,1,1,1,1,1,1,1,1,1,1,1,1,1,1,1,1,1,
1,1,6),(-0.667078900656922,-0.657142857142857,-0.628571428571429,-0.6,-0.571428571428572,
-0.542857142857143,-0.514285714285714,-0.485714285714286,-0.457142857142857,
-0.428571428571429,-0.4,-0.371428571428571,-0.342857142857143,-0.314285714285714,
-0.285714285714286,-0.257142857142857,-0.228571428571429,-0.2,-0.171428571428571,
-0.142857142857143,-0.114285714285714,-0.0857142857142857,-0.0571428571428571,
-0.0285714285714286,0.),.UNSPECIFIED.)
CURVE()
GEOMETRIC_REPRESENTATION_ITEM()
RATIONAL_B_SPLINE_CURVE((1.,1.,1.,1.,1.,1.,1.,1.,1.,1.,1.,1.,1.,1.,1.,1.,
1.,1.,1.,1.,1.,1.,1.,1.,1.,1.,1.,1.,1.))
REPRESENTATION_ITEM('')
);
#644=(
BOUNDED_CURVE()
B_SPLINE_CURVE(5,(#45314,#45315,#45316,#45317,#45318,#45319,#45320,#45321,
#45322,#45323,#45324,#45325,#45326,#45327,#45328,#45329,#45330,#45331,#45332,
#45333,#45334,#45335,#45336,#45337,#45338,#45339,#45340,#45341,#45342),
 .UNSPECIFIED.,.F.,.F.)
B_SPLINE_CURVE_WITH_KNOTS((6,1,1,1,1,1,1,1,1,1,1,1,1,1,1,1,1,1,1,1,1,1,
1,1,6),(0.,0.0285714285714286,0.0571428571428571,0.0857142857142857,0.114285714285714,
0.142857142857143,0.171428571428571,0.2,0.228571428571429,0.257142857142857,
0.285714285714286,0.314285714285714,0.342857142857143,0.371428571428571,
0.4,0.428571428571429,0.457142857142857,0.485714285714286,0.514285714285714,
0.542857142857143,0.571428571428572,0.6,0.628571428571429,0.657142857142857,
0.667078900656917),.UNSPECIFIED.)
CURVE()
GEOMETRIC_REPRESENTATION_ITEM()
RATIONAL_B_SPLINE_CURVE((1.,1.,1.,1.,1.,1.,1.,1.,1.,1.,1.,1.,1.,1.,1.,1.,
1.,1.,1.,1.,1.,1.,1.,1.,1.,1.,1.,1.,1.))
REPRESENTATION_ITEM('')
);
#645=(
BOUNDED_CURVE()
B_SPLINE_CURVE(5,(#45345,#45346,#45347,#45348,#45349,#45350,#45351,#45352,
#45353,#45354,#45355,#45356,#45357,#45358,#45359,#45360,#45361,#45362,#45363,
#45364,#45365,#45366,#45367,#45368,#45369),.UNSPECIFIED.,.F.,.F.)
B_SPLINE_CURVE_WITH_KNOTS((6,1,1,1,1,1,1,1,1,1,1,1,1,1,1,1,1,1,1,1,6),(0.436331539942223,
0.457142857142857,0.485714285714286,0.514285714285714,0.542857142857143,
0.571428571428572,0.6,0.628571428571429,0.657142857142857,0.685714285714286,
0.714285714285714,0.742857142857143,0.771428571428572,0.8,0.828571428571429,
0.857142857142857,0.885714285714286,0.914285714285714,0.942857142857143,
0.971428571428572,1.),.UNSPECIFIED.)
CURVE()
GEOMETRIC_REPRESENTATION_ITEM()
RATIONAL_B_SPLINE_CURVE((1.,1.,1.,1.,1.,1.,1.,1.,1.,1.,1.,1.,1.,1.,1.,1.,
1.,1.,1.,1.,1.,1.,1.,1.,1.))
REPRESENTATION_ITEM('')
);
#646=(
BOUNDED_CURVE()
B_SPLINE_CURVE(5,(#45458,#45459,#45460,#45461,#45462,#45463,#45464,#45465,
#45466,#45467,#45468,#45469,#45470,#45471,#45472,#45473,#45474,#45475,#45476,
#45477,#45478,#45479,#45480,#45481,#45482),.UNSPECIFIED.,.F.,.F.)
B_SPLINE_CURVE_WITH_KNOTS((6,1,1,1,1,1,1,1,1,1,1,1,1,1,1,1,1,1,1,1,6),(-1.,
-0.971428571428572,-0.942857142857143,-0.914285714285714,-0.885714285714286,
-0.857142857142857,-0.828571428571429,-0.8,-0.771428571428572,-0.742857142857143,
-0.714285714285714,-0.685714285714286,-0.657142857142857,-0.628571428571429,
-0.6,-0.571428571428572,-0.542857142857143,-0.514285714285714,-0.485714285714286,
-0.457142857142857,-0.436331539942219),.UNSPECIFIED.)
CURVE()
GEOMETRIC_REPRESENTATION_ITEM()
RATIONAL_B_SPLINE_CURVE((1.,1.,1.,1.,1.,1.,1.,1.,1.,1.,1.,1.,1.,1.,1.,1.,
1.,1.,1.,1.,1.,1.,1.,1.,1.))
REPRESENTATION_ITEM('')
);
#647=(
BOUNDED_CURVE()
B_SPLINE_CURVE(5,(#45578,#45579,#45580,#45581,#45582,#45583,#45584,#45585,
#45586,#45587,#45588,#45589,#45590,#45591,#45592,#45593,#45594,#45595,#45596,
#45597,#45598,#45599,#45600,#45601,#45602,#45603,#45604,#45605,#45606),
 .UNSPECIFIED.,.F.,.F.)
B_SPLINE_CURVE_WITH_KNOTS((6,1,1,1,1,1,1,1,1,1,1,1,1,1,1,1,1,1,1,1,1,1,
1,1,6),(-0.667078900656922,-0.657142857142857,-0.628571428571429,-0.6,-0.571428571428572,
-0.542857142857143,-0.514285714285714,-0.485714285714286,-0.457142857142857,
-0.428571428571429,-0.4,-0.371428571428571,-0.342857142857143,-0.314285714285714,
-0.285714285714286,-0.257142857142857,-0.228571428571429,-0.2,-0.171428571428571,
-0.142857142857143,-0.114285714285714,-0.0857142857142857,-0.0571428571428571,
-0.0285714285714286,0.),.UNSPECIFIED.)
CURVE()
GEOMETRIC_REPRESENTATION_ITEM()
RATIONAL_B_SPLINE_CURVE((1.,1.,1.,1.,1.,1.,1.,1.,1.,1.,1.,1.,1.,1.,1.,1.,
1.,1.,1.,1.,1.,1.,1.,1.,1.,1.,1.,1.,1.))
REPRESENTATION_ITEM('')
);
#648=(
BOUNDED_CURVE()
B_SPLINE_CURVE(5,(#45636,#45637,#45638,#45639,#45640,#45641,#45642,#45643,
#45644,#45645,#45646,#45647,#45648,#45649,#45650,#45651,#45652,#45653,#45654,
#45655,#45656,#45657,#45658,#45659,#45660,#45661,#45662,#45663,#45664),
 .UNSPECIFIED.,.F.,.F.)
B_SPLINE_CURVE_WITH_KNOTS((6,1,1,1,1,1,1,1,1,1,1,1,1,1,1,1,1,1,1,1,1,1,
1,1,6),(0.,0.0285714285714286,0.0571428571428571,0.0857142857142857,0.114285714285714,
0.142857142857143,0.171428571428571,0.2,0.228571428571429,0.257142857142857,
0.285714285714286,0.314285714285714,0.342857142857143,0.371428571428571,
0.4,0.428571428571429,0.457142857142857,0.485714285714286,0.514285714285714,
0.542857142857143,0.571428571428572,0.6,0.628571428571429,0.657142857142857,
0.667078900656917),.UNSPECIFIED.)
CURVE()
GEOMETRIC_REPRESENTATION_ITEM()
RATIONAL_B_SPLINE_CURVE((1.,1.,1.,1.,1.,1.,1.,1.,1.,1.,1.,1.,1.,1.,1.,1.,
1.,1.,1.,1.,1.,1.,1.,1.,1.,1.,1.,1.,1.))
REPRESENTATION_ITEM('')
);
#649=(
BOUNDED_CURVE()
B_SPLINE_CURVE(5,(#45667,#45668,#45669,#45670,#45671,#45672,#45673,#45674,
#45675,#45676,#45677,#45678,#45679,#45680,#45681,#45682,#45683,#45684,#45685,
#45686,#45687,#45688,#45689,#45690,#45691),.UNSPECIFIED.,.F.,.F.)
B_SPLINE_CURVE_WITH_KNOTS((6,1,1,1,1,1,1,1,1,1,1,1,1,1,1,1,1,1,1,1,6),(0.436331539942223,
0.457142857142857,0.485714285714286,0.514285714285714,0.542857142857143,
0.571428571428572,0.6,0.628571428571429,0.657142857142857,0.685714285714286,
0.714285714285714,0.742857142857143,0.771428571428572,0.8,0.828571428571429,
0.857142857142857,0.885714285714286,0.914285714285714,0.942857142857143,
0.971428571428572,1.),.UNSPECIFIED.)
CURVE()
GEOMETRIC_REPRESENTATION_ITEM()
RATIONAL_B_SPLINE_CURVE((1.,1.,1.,1.,1.,1.,1.,1.,1.,1.,1.,1.,1.,1.,1.,1.,
1.,1.,1.,1.,1.,1.,1.,1.,1.))
REPRESENTATION_ITEM('')
);
#650=(
BOUNDED_CURVE()
B_SPLINE_CURVE(5,(#45780,#45781,#45782,#45783,#45784,#45785,#45786,#45787,
#45788,#45789,#45790,#45791,#45792,#45793,#45794,#45795,#45796,#45797,#45798,
#45799,#45800,#45801,#45802,#45803,#45804),.UNSPECIFIED.,.F.,.F.)
B_SPLINE_CURVE_WITH_KNOTS((6,1,1,1,1,1,1,1,1,1,1,1,1,1,1,1,1,1,1,1,6),(-1.,
-0.971428571428572,-0.942857142857143,-0.914285714285714,-0.885714285714286,
-0.857142857142857,-0.828571428571429,-0.8,-0.771428571428572,-0.742857142857143,
-0.714285714285714,-0.685714285714286,-0.657142857142857,-0.628571428571429,
-0.6,-0.571428571428572,-0.542857142857143,-0.514285714285714,-0.485714285714286,
-0.457142857142857,-0.436331539942219),.UNSPECIFIED.)
CURVE()
GEOMETRIC_REPRESENTATION_ITEM()
RATIONAL_B_SPLINE_CURVE((1.,1.,1.,1.,1.,1.,1.,1.,1.,1.,1.,1.,1.,1.,1.,1.,
1.,1.,1.,1.,1.,1.,1.,1.,1.))
REPRESENTATION_ITEM('')
);
#651=(
BOUNDED_CURVE()
B_SPLINE_CURVE(5,(#45900,#45901,#45902,#45903,#45904,#45905,#45906,#45907,
#45908,#45909,#45910,#45911,#45912,#45913,#45914,#45915,#45916,#45917,#45918,
#45919,#45920,#45921,#45922,#45923,#45924,#45925,#45926,#45927,#45928),
 .UNSPECIFIED.,.F.,.F.)
B_SPLINE_CURVE_WITH_KNOTS((6,1,1,1,1,1,1,1,1,1,1,1,1,1,1,1,1,1,1,1,1,1,
1,1,6),(-0.667078900656922,-0.657142857142857,-0.628571428571429,-0.6,-0.571428571428572,
-0.542857142857143,-0.514285714285714,-0.485714285714286,-0.457142857142857,
-0.428571428571429,-0.4,-0.371428571428571,-0.342857142857143,-0.314285714285714,
-0.285714285714286,-0.257142857142857,-0.228571428571429,-0.2,-0.171428571428571,
-0.142857142857143,-0.114285714285714,-0.0857142857142857,-0.0571428571428571,
-0.0285714285714286,0.),.UNSPECIFIED.)
CURVE()
GEOMETRIC_REPRESENTATION_ITEM()
RATIONAL_B_SPLINE_CURVE((1.,1.,1.,1.,1.,1.,1.,1.,1.,1.,1.,1.,1.,1.,1.,1.,
1.,1.,1.,1.,1.,1.,1.,1.,1.,1.,1.,1.,1.))
REPRESENTATION_ITEM('')
);
#652=(
BOUNDED_CURVE()
B_SPLINE_CURVE(5,(#45964,#45965,#45966,#45967,#45968,#45969,#45970,#45971,
#45972,#45973,#45974,#45975,#45976,#45977,#45978,#45979,#45980,#45981,#45982,
#45983,#45984,#45985,#45986,#45987,#45988,#45989,#45990,#45991,#45992),
 .UNSPECIFIED.,.F.,.F.)
B_SPLINE_CURVE_WITH_KNOTS((6,1,1,1,1,1,1,1,1,1,1,1,1,1,1,1,1,1,1,1,1,1,
1,1,6),(0.,0.0285714285714286,0.0571428571428571,0.0857142857142857,0.114285714285714,
0.142857142857143,0.171428571428571,0.2,0.228571428571429,0.257142857142857,
0.285714285714286,0.314285714285714,0.342857142857143,0.371428571428571,
0.4,0.428571428571429,0.457142857142857,0.485714285714286,0.514285714285714,
0.542857142857143,0.571428571428572,0.6,0.628571428571429,0.657142857142857,
0.667078900656916),.UNSPECIFIED.)
CURVE()
GEOMETRIC_REPRESENTATION_ITEM()
RATIONAL_B_SPLINE_CURVE((1.,1.,1.,1.,1.,1.,1.,1.,1.,1.,1.,1.,1.,1.,1.,1.,
1.,1.,1.,1.,1.,1.,1.,1.,1.,1.,1.,1.,1.))
REPRESENTATION_ITEM('')
);
#653=(
BOUNDED_CURVE()
B_SPLINE_CURVE(5,(#45995,#45996,#45997,#45998,#45999,#46000,#46001,#46002,
#46003,#46004,#46005,#46006,#46007,#46008,#46009,#46010,#46011,#46012,#46013,
#46014,#46015,#46016,#46017,#46018,#46019),.UNSPECIFIED.,.F.,.F.)
B_SPLINE_CURVE_WITH_KNOTS((6,1,1,1,1,1,1,1,1,1,1,1,1,1,1,1,1,1,1,1,6),(0.436331539942224,
0.457142857142857,0.485714285714286,0.514285714285714,0.542857142857143,
0.571428571428572,0.6,0.628571428571429,0.657142857142857,0.685714285714286,
0.714285714285714,0.742857142857143,0.771428571428572,0.8,0.828571428571429,
0.857142857142857,0.885714285714286,0.914285714285714,0.942857142857143,
0.971428571428572,1.),.UNSPECIFIED.)
CURVE()
GEOMETRIC_REPRESENTATION_ITEM()
RATIONAL_B_SPLINE_CURVE((1.,1.,1.,1.,1.,1.,1.,1.,1.,1.,1.,1.,1.,1.,1.,1.,
1.,1.,1.,1.,1.,1.,1.,1.,1.))
REPRESENTATION_ITEM('')
);
#654=(
BOUNDED_CURVE()
B_SPLINE_CURVE(5,(#46108,#46109,#46110,#46111,#46112,#46113,#46114,#46115,
#46116,#46117,#46118,#46119,#46120,#46121,#46122,#46123,#46124,#46125,#46126,
#46127,#46128,#46129,#46130,#46131,#46132),.UNSPECIFIED.,.F.,.F.)
B_SPLINE_CURVE_WITH_KNOTS((6,1,1,1,1,1,1,1,1,1,1,1,1,1,1,1,1,1,1,1,6),(-1.,
-0.971428571428572,-0.942857142857143,-0.914285714285714,-0.885714285714286,
-0.857142857142857,-0.828571428571429,-0.8,-0.771428571428572,-0.742857142857143,
-0.714285714285714,-0.685714285714286,-0.657142857142857,-0.628571428571429,
-0.6,-0.571428571428572,-0.542857142857143,-0.514285714285714,-0.485714285714286,
-0.457142857142857,-0.43633153994222),.UNSPECIFIED.)
CURVE()
GEOMETRIC_REPRESENTATION_ITEM()
RATIONAL_B_SPLINE_CURVE((1.,1.,1.,1.,1.,1.,1.,1.,1.,1.,1.,1.,1.,1.,1.,1.,
1.,1.,1.,1.,1.,1.,1.,1.,1.))
REPRESENTATION_ITEM('')
);
#655=(
BOUNDED_CURVE()
B_SPLINE_CURVE(5,(#46228,#46229,#46230,#46231,#46232,#46233,#46234,#46235,
#46236,#46237,#46238,#46239,#46240,#46241,#46242,#46243,#46244,#46245,#46246,
#46247,#46248,#46249,#46250,#46251,#46252,#46253,#46254,#46255,#46256),
 .UNSPECIFIED.,.F.,.F.)
B_SPLINE_CURVE_WITH_KNOTS((6,1,1,1,1,1,1,1,1,1,1,1,1,1,1,1,1,1,1,1,1,1,
1,1,6),(-0.667078900656921,-0.657142857142857,-0.628571428571429,-0.6,-0.571428571428572,
-0.542857142857143,-0.514285714285714,-0.485714285714286,-0.457142857142857,
-0.428571428571429,-0.4,-0.371428571428571,-0.342857142857143,-0.314285714285714,
-0.285714285714286,-0.257142857142857,-0.228571428571429,-0.2,-0.171428571428571,
-0.142857142857143,-0.114285714285714,-0.0857142857142857,-0.0571428571428571,
-0.0285714285714286,0.),.UNSPECIFIED.)
CURVE()
GEOMETRIC_REPRESENTATION_ITEM()
RATIONAL_B_SPLINE_CURVE((1.,1.,1.,1.,1.,1.,1.,1.,1.,1.,1.,1.,1.,1.,1.,1.,
1.,1.,1.,1.,1.,1.,1.,1.,1.,1.,1.,1.,1.))
REPRESENTATION_ITEM('')
);
#656=(
BOUNDED_CURVE()
B_SPLINE_CURVE(5,(#46286,#46287,#46288,#46289,#46290,#46291,#46292,#46293,
#46294,#46295,#46296,#46297,#46298,#46299,#46300,#46301,#46302,#46303,#46304,
#46305,#46306,#46307,#46308,#46309,#46310,#46311,#46312,#46313,#46314),
 .UNSPECIFIED.,.F.,.F.)
B_SPLINE_CURVE_WITH_KNOTS((6,1,1,1,1,1,1,1,1,1,1,1,1,1,1,1,1,1,1,1,1,1,
1,1,6),(0.,0.0285714285714286,0.0571428571428571,0.0857142857142857,0.114285714285714,
0.142857142857143,0.171428571428571,0.2,0.228571428571429,0.257142857142857,
0.285714285714286,0.314285714285714,0.342857142857143,0.371428571428571,
0.4,0.428571428571429,0.457142857142857,0.485714285714286,0.514285714285714,
0.542857142857143,0.571428571428572,0.6,0.628571428571429,0.657142857142857,
0.667078900656917),.UNSPECIFIED.)
CURVE()
GEOMETRIC_REPRESENTATION_ITEM()
RATIONAL_B_SPLINE_CURVE((1.,1.,1.,1.,1.,1.,1.,1.,1.,1.,1.,1.,1.,1.,1.,1.,
1.,1.,1.,1.,1.,1.,1.,1.,1.,1.,1.,1.,1.))
REPRESENTATION_ITEM('')
);
#657=(
BOUNDED_CURVE()
B_SPLINE_CURVE(5,(#46317,#46318,#46319,#46320,#46321,#46322,#46323,#46324,
#46325,#46326,#46327,#46328,#46329,#46330,#46331,#46332,#46333,#46334,#46335,
#46336,#46337,#46338,#46339,#46340,#46341),.UNSPECIFIED.,.F.,.F.)
B_SPLINE_CURVE_WITH_KNOTS((6,1,1,1,1,1,1,1,1,1,1,1,1,1,1,1,1,1,1,1,6),(0.436331539942224,
0.457142857142857,0.485714285714286,0.514285714285714,0.542857142857143,
0.571428571428572,0.6,0.628571428571429,0.657142857142857,0.685714285714286,
0.714285714285714,0.742857142857143,0.771428571428572,0.8,0.828571428571429,
0.857142857142857,0.885714285714286,0.914285714285714,0.942857142857143,
0.971428571428572,1.),.UNSPECIFIED.)
CURVE()
GEOMETRIC_REPRESENTATION_ITEM()
RATIONAL_B_SPLINE_CURVE((1.,1.,1.,1.,1.,1.,1.,1.,1.,1.,1.,1.,1.,1.,1.,1.,
1.,1.,1.,1.,1.,1.,1.,1.,1.))
REPRESENTATION_ITEM('')
);
#658=(
BOUNDED_CURVE()
B_SPLINE_CURVE(5,(#46430,#46431,#46432,#46433,#46434,#46435,#46436,#46437,
#46438,#46439,#46440,#46441,#46442,#46443,#46444,#46445,#46446,#46447,#46448,
#46449,#46450,#46451,#46452,#46453,#46454),.UNSPECIFIED.,.F.,.F.)
B_SPLINE_CURVE_WITH_KNOTS((6,1,1,1,1,1,1,1,1,1,1,1,1,1,1,1,1,1,1,1,6),(-1.,
-0.971428571428572,-0.942857142857143,-0.914285714285714,-0.885714285714286,
-0.857142857142857,-0.828571428571429,-0.8,-0.771428571428572,-0.742857142857143,
-0.714285714285714,-0.685714285714286,-0.657142857142857,-0.628571428571429,
-0.6,-0.571428571428572,-0.542857142857143,-0.514285714285714,-0.485714285714286,
-0.457142857142857,-0.43633153994222),.UNSPECIFIED.)
CURVE()
GEOMETRIC_REPRESENTATION_ITEM()
RATIONAL_B_SPLINE_CURVE((1.,1.,1.,1.,1.,1.,1.,1.,1.,1.,1.,1.,1.,1.,1.,1.,
1.,1.,1.,1.,1.,1.,1.,1.,1.))
REPRESENTATION_ITEM('')
);
#659=(
BOUNDED_CURVE()
B_SPLINE_CURVE(5,(#46550,#46551,#46552,#46553,#46554,#46555,#46556,#46557,
#46558,#46559,#46560,#46561,#46562,#46563,#46564,#46565,#46566,#46567,#46568,
#46569,#46570,#46571,#46572,#46573,#46574,#46575,#46576,#46577,#46578),
 .UNSPECIFIED.,.F.,.F.)
B_SPLINE_CURVE_WITH_KNOTS((6,1,1,1,1,1,1,1,1,1,1,1,1,1,1,1,1,1,1,1,1,1,
1,1,6),(-0.667078900656921,-0.657142857142857,-0.628571428571429,-0.6,-0.571428571428572,
-0.542857142857143,-0.514285714285714,-0.485714285714286,-0.457142857142857,
-0.428571428571429,-0.4,-0.371428571428571,-0.342857142857143,-0.314285714285714,
-0.285714285714286,-0.257142857142857,-0.228571428571429,-0.2,-0.171428571428571,
-0.142857142857143,-0.114285714285714,-0.0857142857142857,-0.0571428571428571,
-0.0285714285714286,0.),.UNSPECIFIED.)
CURVE()
GEOMETRIC_REPRESENTATION_ITEM()
RATIONAL_B_SPLINE_CURVE((1.,1.,1.,1.,1.,1.,1.,1.,1.,1.,1.,1.,1.,1.,1.,1.,
1.,1.,1.,1.,1.,1.,1.,1.,1.,1.,1.,1.,1.))
REPRESENTATION_ITEM('')
);
#660=(
BOUNDED_CURVE()
B_SPLINE_CURVE(5,(#46608,#46609,#46610,#46611,#46612,#46613,#46614,#46615,
#46616,#46617,#46618,#46619,#46620,#46621,#46622,#46623,#46624,#46625,#46626,
#46627,#46628,#46629,#46630,#46631,#46632,#46633,#46634,#46635,#46636),
 .UNSPECIFIED.,.F.,.F.)
B_SPLINE_CURVE_WITH_KNOTS((6,1,1,1,1,1,1,1,1,1,1,1,1,1,1,1,1,1,1,1,1,1,
1,1,6),(0.,0.0285714285714286,0.0571428571428571,0.0857142857142857,0.114285714285714,
0.142857142857143,0.171428571428571,0.2,0.228571428571429,0.257142857142857,
0.285714285714286,0.314285714285714,0.342857142857143,0.371428571428571,
0.4,0.428571428571429,0.457142857142857,0.485714285714286,0.514285714285714,
0.542857142857143,0.571428571428572,0.6,0.628571428571429,0.657142857142857,
0.667078900656917),.UNSPECIFIED.)
CURVE()
GEOMETRIC_REPRESENTATION_ITEM()
RATIONAL_B_SPLINE_CURVE((1.,1.,1.,1.,1.,1.,1.,1.,1.,1.,1.,1.,1.,1.,1.,1.,
1.,1.,1.,1.,1.,1.,1.,1.,1.,1.,1.,1.,1.))
REPRESENTATION_ITEM('')
);
#661=(
BOUNDED_CURVE()
B_SPLINE_CURVE(5,(#46639,#46640,#46641,#46642,#46643,#46644,#46645,#46646,
#46647,#46648,#46649,#46650,#46651,#46652,#46653,#46654,#46655,#46656,#46657,
#46658,#46659,#46660,#46661,#46662,#46663),.UNSPECIFIED.,.F.,.F.)
B_SPLINE_CURVE_WITH_KNOTS((6,1,1,1,1,1,1,1,1,1,1,1,1,1,1,1,1,1,1,1,6),(0.436331539942223,
0.457142857142857,0.485714285714286,0.514285714285714,0.542857142857143,
0.571428571428572,0.6,0.628571428571429,0.657142857142857,0.685714285714286,
0.714285714285714,0.742857142857143,0.771428571428572,0.8,0.828571428571429,
0.857142857142857,0.885714285714286,0.914285714285714,0.942857142857143,
0.971428571428572,1.),.UNSPECIFIED.)
CURVE()
GEOMETRIC_REPRESENTATION_ITEM()
RATIONAL_B_SPLINE_CURVE((1.,1.,1.,1.,1.,1.,1.,1.,1.,1.,1.,1.,1.,1.,1.,1.,
1.,1.,1.,1.,1.,1.,1.,1.,1.))
REPRESENTATION_ITEM('')
);
#662=(
BOUNDED_CURVE()
B_SPLINE_CURVE(5,(#46752,#46753,#46754,#46755,#46756,#46757,#46758,#46759,
#46760,#46761,#46762,#46763,#46764,#46765,#46766,#46767,#46768,#46769,#46770,
#46771,#46772,#46773,#46774,#46775,#46776),.UNSPECIFIED.,.F.,.F.)
B_SPLINE_CURVE_WITH_KNOTS((6,1,1,1,1,1,1,1,1,1,1,1,1,1,1,1,1,1,1,1,6),(-1.,
-0.971428571428572,-0.942857142857143,-0.914285714285714,-0.885714285714286,
-0.857142857142857,-0.828571428571429,-0.8,-0.771428571428572,-0.742857142857143,
-0.714285714285714,-0.685714285714286,-0.657142857142857,-0.628571428571429,
-0.6,-0.571428571428572,-0.542857142857143,-0.514285714285714,-0.485714285714286,
-0.457142857142857,-0.436331539942219),.UNSPECIFIED.)
CURVE()
GEOMETRIC_REPRESENTATION_ITEM()
RATIONAL_B_SPLINE_CURVE((1.,1.,1.,1.,1.,1.,1.,1.,1.,1.,1.,1.,1.,1.,1.,1.,
1.,1.,1.,1.,1.,1.,1.,1.,1.))
REPRESENTATION_ITEM('')
);
#663=(
BOUNDED_CURVE()
B_SPLINE_CURVE(5,(#46872,#46873,#46874,#46875,#46876,#46877,#46878,#46879,
#46880,#46881,#46882,#46883,#46884,#46885,#46886,#46887,#46888,#46889,#46890,
#46891,#46892,#46893,#46894,#46895,#46896,#46897,#46898,#46899,#46900),
 .UNSPECIFIED.,.F.,.F.)
B_SPLINE_CURVE_WITH_KNOTS((6,1,1,1,1,1,1,1,1,1,1,1,1,1,1,1,1,1,1,1,1,1,
1,1,6),(-0.667078900656922,-0.657142857142857,-0.628571428571429,-0.6,-0.571428571428572,
-0.542857142857143,-0.514285714285714,-0.485714285714286,-0.457142857142857,
-0.428571428571429,-0.4,-0.371428571428571,-0.342857142857143,-0.314285714285714,
-0.285714285714286,-0.257142857142857,-0.228571428571429,-0.2,-0.171428571428571,
-0.142857142857143,-0.114285714285714,-0.0857142857142857,-0.0571428571428571,
-0.0285714285714286,0.),.UNSPECIFIED.)
CURVE()
GEOMETRIC_REPRESENTATION_ITEM()
RATIONAL_B_SPLINE_CURVE((1.,1.,1.,1.,1.,1.,1.,1.,1.,1.,1.,1.,1.,1.,1.,1.,
1.,1.,1.,1.,1.,1.,1.,1.,1.,1.,1.,1.,1.))
REPRESENTATION_ITEM('')
);
#664=(
BOUNDED_CURVE()
B_SPLINE_CURVE(5,(#47007,#47008,#47009,#47010,#47011,#47012,#47013,#47014,
#47015,#47016,#47017,#47018,#47019,#47020,#47021,#47022,#47023,#47024,#47025,
#47026,#47027,#47028,#47029,#47030,#47031,#47032,#47033,#47034,#47035),
 .UNSPECIFIED.,.F.,.F.)
B_SPLINE_CURVE_WITH_KNOTS((6,1,1,1,1,1,1,1,1,1,1,1,1,1,1,1,1,1,1,1,1,1,
1,1,6),(-0.667078900656922,-0.657142857142857,-0.628571428571429,-0.6,-0.571428571428572,
-0.542857142857143,-0.514285714285714,-0.485714285714286,-0.457142857142857,
-0.428571428571429,-0.4,-0.371428571428571,-0.342857142857143,-0.314285714285714,
-0.285714285714286,-0.257142857142857,-0.228571428571429,-0.2,-0.171428571428571,
-0.142857142857143,-0.114285714285714,-0.0857142857142857,-0.0571428571428571,
-0.0285714285714286,0.),.UNSPECIFIED.)
CURVE()
GEOMETRIC_REPRESENTATION_ITEM()
RATIONAL_B_SPLINE_CURVE((1.,1.,1.,1.,1.,1.,1.,1.,1.,1.,1.,1.,1.,1.,1.,1.,
1.,1.,1.,1.,1.,1.,1.,1.,1.,1.,1.,1.,1.))
REPRESENTATION_ITEM('')
);
#665=(
BOUNDED_CURVE()
B_SPLINE_CURVE(5,(#47038,#47039,#47040,#47041,#47042,#47043,#47044,#47045,
#47046,#47047,#47048,#47049,#47050,#47051,#47052,#47053,#47054,#47055,#47056,
#47057,#47058,#47059,#47060,#47061,#47062,#47063,#47064,#47065,#47066),
 .UNSPECIFIED.,.F.,.F.)
B_SPLINE_CURVE_WITH_KNOTS((6,1,1,1,1,1,1,1,1,1,1,1,1,1,1,1,1,1,1,1,1,1,
1,1,6),(0.,0.0285714285714286,0.0571428571428571,0.0857142857142857,0.114285714285714,
0.142857142857143,0.171428571428571,0.2,0.228571428571429,0.257142857142857,
0.285714285714286,0.314285714285714,0.342857142857143,0.371428571428571,
0.4,0.428571428571429,0.457142857142857,0.485714285714286,0.514285714285714,
0.542857142857143,0.571428571428572,0.6,0.628571428571429,0.657142857142857,
0.667078900656918),.UNSPECIFIED.)
CURVE()
GEOMETRIC_REPRESENTATION_ITEM()
RATIONAL_B_SPLINE_CURVE((1.,1.,1.,1.,1.,1.,1.,1.,1.,1.,1.,1.,1.,1.,1.,1.,
1.,1.,1.,1.,1.,1.,1.,1.,1.,1.,1.,1.,1.))
REPRESENTATION_ITEM('')
);
#666=(
BOUNDED_CURVE()
B_SPLINE_CURVE(5,(#47071,#47072,#47073,#47074,#47075,#47076,#47077,#47078,
#47079,#47080,#47081,#47082,#47083,#47084,#47085,#47086,#47087,#47088,#47089,
#47090,#47091,#47092,#47093,#47094,#47095),.UNSPECIFIED.,.F.,.F.)
B_SPLINE_CURVE_WITH_KNOTS((6,1,1,1,1,1,1,1,1,1,1,1,1,1,1,1,1,1,1,1,6),(0.436331539942222,
0.457142857142857,0.485714285714286,0.514285714285714,0.542857142857143,
0.571428571428572,0.6,0.628571428571429,0.657142857142857,0.685714285714286,
0.714285714285714,0.742857142857143,0.771428571428572,0.8,0.828571428571429,
0.857142857142857,0.885714285714286,0.914285714285714,0.942857142857143,
0.971428571428572,1.),.UNSPECIFIED.)
CURVE()
GEOMETRIC_REPRESENTATION_ITEM()
RATIONAL_B_SPLINE_CURVE((1.,1.,1.,1.,1.,1.,1.,1.,1.,1.,1.,1.,1.,1.,1.,1.,
1.,1.,1.,1.,1.,1.,1.,1.,1.))
REPRESENTATION_ITEM('')
);
#667=(
BOUNDED_CURVE()
B_SPLINE_CURVE(5,(#47192,#47193,#47194,#47195,#47196,#47197,#47198,#47199,
#47200,#47201,#47202,#47203,#47204,#47205,#47206,#47207,#47208,#47209,#47210,
#47211,#47212,#47213,#47214,#47215,#47216),.UNSPECIFIED.,.F.,.F.)
B_SPLINE_CURVE_WITH_KNOTS((6,1,1,1,1,1,1,1,1,1,1,1,1,1,1,1,1,1,1,1,6),(-1.,
-0.971428571428572,-0.942857142857143,-0.914285714285714,-0.885714285714286,
-0.857142857142857,-0.828571428571429,-0.8,-0.771428571428572,-0.742857142857143,
-0.714285714285714,-0.685714285714286,-0.657142857142857,-0.628571428571429,
-0.6,-0.571428571428572,-0.542857142857143,-0.514285714285714,-0.485714285714286,
-0.457142857142857,-0.436331539942219),.UNSPECIFIED.)
CURVE()
GEOMETRIC_REPRESENTATION_ITEM()
RATIONAL_B_SPLINE_CURVE((1.,1.,1.,1.,1.,1.,1.,1.,1.,1.,1.,1.,1.,1.,1.,1.,
1.,1.,1.,1.,1.,1.,1.,1.,1.))
REPRESENTATION_ITEM('')
);
#834=B_SPLINE_SURFACE_WITH_KNOTS('',3,3,((#35741,#35742,#35743,#35744,#35745,
#35746,#35747,#35748,#35749,#35750,#35751,#35752,#35753,#35754,#35755,#35756,
#35757,#35758,#35759,#35760,#35761,#35762,#35763,#35764,#35765,#35766,#35767,
#35768,#35769,#35770,#35771,#35772,#35773,#35774,#35775,#35776,#35777,#35778,
#35779,#35780,#35781,#35782,#35783,#35784,#35785,#35786,#35787,#35788,#35789,
#35790,#35791,#35792,#35793,#35794,#35795,#35796,#35797,#35798,#35799,#35800,
#35801,#35802,#35803,#35804,#35805,#35806,#35807,#35808,#35809,#35810,#35811,
#35812,#35813,#35814,#35815,#35816,#35817,#35818,#35819,#35820,#35821,#35822,
#35823,#35824,#35825,#35826,#35827,#35828,#35829,#35830,#35831,#35832,#35833,
#35834,#35835,#35836,#35837,#35838,#35839,#35840,#35841,#35842,#35843,#35844,
#35845,#35846,#35847,#35848,#35849,#35850,#35851,#35852,#35853,#35854,#35855,
#35856,#35857,#35858,#35859,#35860,#35861,#35862,#35863,#35864,#35865,#35866,
#35867,#35868,#35869,#35870,#35871,#35872,#35873,#35874,#35875,#35876,#35877,
#35878,#35879,#35880,#35881,#35882,#35883,#35884,#35885,#35886,#35887,#35888,
#35889,#35890,#35891,#35892,#35893,#35894,#35895,#35896,#35897,#35898,#35899,
#35900,#35901,#35902,#35903,#35904,#35905,#35906,#35907,#35908,#35909,#35910,
#35911,#35912,#35913,#35914,#35915,#35916,#35917,#35918,#35919,#35920,#35921,
#35922,#35923,#35924,#35925,#35926,#35927,#35928,#35929,#35930,#35931,#35932,
#35933,#35934,#35935,#35936,#35937,#35938,#35939,#35940,#35941,#35942,#35943,
#35944,#35945,#35946,#35947,#35948,#35949,#35950,#35951,#35952,#35953,#35954,
#35955,#35956,#35957,#35958,#35959,#35960,#35961,#35962,#35963,#35964,#35965,
#35966,#35967,#35968,#35969,#35970,#35971,#35972,#35973,#35974,#35975,#35976,
#35977,#35978,#35979,#35980,#35981,#35982,#35983,#35984,#35985,#35986,#35987,
#35988,#35989,#35990,#35991,#35992,#35993,#35994,#35995,#35996,#35997,#35998,
#35999,#36000,#36001,#36002,#36003,#36004,#36005,#36006,#36007,#36008,#36009,
#36010,#36011,#36012,#36013,#36014,#36015,#36016,#36017,#36018,#36019,#36020,
#36021,#36022,#36023,#36024,#36025,#36026,#36027,#36028,#36029,#36030,#36031,
#36032,#36033,#36034,#36035,#36036,#36037,#36038,#36039,#36040,#36041,#36042,
#36043,#36044,#36045,#36046,#36047,#36048,#36049,#36050,#36051,#36052,#36053,
#36054,#36055,#36056,#36057,#36058,#36059,#36060,#36061,#36062,#36063,#36064,
#36065,#36066,#36067,#36068,#36069,#36070,#36071,#36072,#36073,#36074,#36075,
#36076,#36077,#36078,#36079,#36080,#36081,#36082,#36083,#36084,#36085,#36086,
#36087,#36088,#36089,#36090,#36091,#36092,#36093,#36094,#36095,#36096,#36097,
#36098,#36099,#36100,#36101,#36102,#36103,#36104,#36105,#36106,#36107,#36108,
#36109,#36110,#36111,#36112,#36113,#36114,#36115,#36116,#36117,#36118,#36119,
#36120,#36121,#36122,#36123,#36124,#36125,#36126,#36127,#36128,#36129,#36130,
#36131,#36132,#36133,#36134,#36135,#36136,#36137,#36138,#36139,#36140,#36141,
#36142,#36143,#36144,#36145,#36146,#36147,#36148,#36149,#36150,#36151,#36152,
#36153,#36154,#36155,#36156,#36157,#36158,#36159,#36160,#36161,#36162,#36163,
#36164,#36165,#36166,#36167,#36168,#36169,#36170,#36171,#36172,#36173,#36174,
#36175,#36176,#36177,#36178,#36179,#36180,#36181,#36182,#36183,#36184,#36185,
#36186,#36187,#36188,#36189,#36190,#36191,#36192,#36193,#36194,#36195,#36196,
#36197,#36198,#36199,#36200,#36201,#36202,#36203,#36204,#36205,#36206,#36207,
#36208,#36209,#36210,#36211,#36212,#36213,#36214,#36215,#36216,#36217,#36218,
#36219,#36220,#36221,#36222,#36223,#36224,#36225,#36226,#36227,#36228,#36229,
#36230,#36231,#36232,#36233,#36234,#36235,#36236,#36237,#36238,#36239,#36240,
#36241,#36242,#36243,#36244,#36245,#36246,#36247,#36248,#36249,#36250,#36251,
#36252,#36253),(#36254,#36255,#36256,#36257,#36258,#36259,#36260,#36261,
#36262,#36263,#36264,#36265,#36266,#36267,#36268,#36269,#36270,#36271,#36272,
#36273,#36274,#36275,#36276,#36277,#36278,#36279,#36280,#36281,#36282,#36283,
#36284,#36285,#36286,#36287,#36288,#36289,#36290,#36291,#36292,#36293,#36294,
#36295,#36296,#36297,#36298,#36299,#36300,#36301,#36302,#36303,#36304,#36305,
#36306,#36307,#36308,#36309,#36310,#36311,#36312,#36313,#36314,#36315,#36316,
#36317,#36318,#36319,#36320,#36321,#36322,#36323,#36324,#36325,#36326,#36327,
#36328,#36329,#36330,#36331,#36332,#36333,#36334,#36335,#36336,#36337,#36338,
#36339,#36340,#36341,#36342,#36343,#36344,#36345,#36346,#36347,#36348,#36349,
#36350,#36351,#36352,#36353,#36354,#36355,#36356,#36357,#36358,#36359,#36360,
#36361,#36362,#36363,#36364,#36365,#36366,#36367,#36368,#36369,#36370,#36371,
#36372,#36373,#36374,#36375,#36376,#36377,#36378,#36379,#36380,#36381,#36382,
#36383,#36384,#36385,#36386,#36387,#36388,#36389,#36390,#36391,#36392,#36393,
#36394,#36395,#36396,#36397,#36398,#36399,#36400,#36401,#36402,#36403,#36404,
#36405,#36406,#36407,#36408,#36409,#36410,#36411,#36412,#36413,#36414,#36415,
#36416,#36417,#36418,#36419,#36420,#36421,#36422,#36423,#36424,#36425,#36426,
#36427,#36428,#36429,#36430,#36431,#36432,#36433,#36434,#36435,#36436,#36437,
#36438,#36439,#36440,#36441,#36442,#36443,#36444,#36445,#36446,#36447,#36448,
#36449,#36450,#36451,#36452,#36453,#36454,#36455,#36456,#36457,#36458,#36459,
#36460,#36461,#36462,#36463,#36464,#36465,#36466,#36467,#36468,#36469,#36470,
#36471,#36472,#36473,#36474,#36475,#36476,#36477,#36478,#36479,#36480,#36481,
#36482,#36483,#36484,#36485,#36486,#36487,#36488,#36489,#36490,#36491,#36492,
#36493,#36494,#36495,#36496,#36497,#36498,#36499,#36500,#36501,#36502,#36503,
#36504,#36505,#36506,#36507,#36508,#36509,#36510,#36511,#36512,#36513,#36514,
#36515,#36516,#36517,#36518,#36519,#36520,#36521,#36522,#36523,#36524,#36525,
#36526,#36527,#36528,#36529,#36530,#36531,#36532,#36533,#36534,#36535,#36536,
#36537,#36538,#36539,#36540,#36541,#36542,#36543,#36544,#36545,#36546,#36547,
#36548,#36549,#36550,#36551,#36552,#36553,#36554,#36555,#36556,#36557,#36558,
#36559,#36560,#36561,#36562,#36563,#36564,#36565,#36566,#36567,#36568,#36569,
#36570,#36571,#36572,#36573,#36574,#36575,#36576,#36577,#36578,#36579,#36580,
#36581,#36582,#36583,#36584,#36585,#36586,#36587,#36588,#36589,#36590,#36591,
#36592,#36593,#36594,#36595,#36596,#36597,#36598,#36599,#36600,#36601,#36602,
#36603,#36604,#36605,#36606,#36607,#36608,#36609,#36610,#36611,#36612,#36613,
#36614,#36615,#36616,#36617,#36618,#36619,#36620,#36621,#36622,#36623,#36624,
#36625,#36626,#36627,#36628,#36629,#36630,#36631,#36632,#36633,#36634,#36635,
#36636,#36637,#36638,#36639,#36640,#36641,#36642,#36643,#36644,#36645,#36646,
#36647,#36648,#36649,#36650,#36651,#36652,#36653,#36654,#36655,#36656,#36657,
#36658,#36659,#36660,#36661,#36662,#36663,#36664,#36665,#36666,#36667,#36668,
#36669,#36670,#36671,#36672,#36673,#36674,#36675,#36676,#36677,#36678,#36679,
#36680,#36681,#36682,#36683,#36684,#36685,#36686,#36687,#36688,#36689,#36690,
#36691,#36692,#36693,#36694,#36695,#36696,#36697,#36698,#36699,#36700,#36701,
#36702,#36703,#36704,#36705,#36706,#36707,#36708,#36709,#36710,#36711,#36712,
#36713,#36714,#36715,#36716,#36717,#36718,#36719,#36720,#36721,#36722,#36723,
#36724,#36725,#36726,#36727,#36728,#36729,#36730,#36731,#36732,#36733,#36734,
#36735,#36736,#36737,#36738,#36739,#36740,#36741,#36742,#36743,#36744,#36745,
#36746,#36747,#36748,#36749,#36750,#36751,#36752,#36753,#36754,#36755,#36756,
#36757,#36758,#36759,#36760,#36761,#36762,#36763,#36764,#36765,#36766),
(#36767,#36768,#36769,#36770,#36771,#36772,#36773,#36774,#36775,#36776,
#36777,#36778,#36779,#36780,#36781,#36782,#36783,#36784,#36785,#36786,#36787,
#36788,#36789,#36790,#36791,#36792,#36793,#36794,#36795,#36796,#36797,#36798,
#36799,#36800,#36801,#36802,#36803,#36804,#36805,#36806,#36807,#36808,#36809,
#36810,#36811,#36812,#36813,#36814,#36815,#36816,#36817,#36818,#36819,#36820,
#36821,#36822,#36823,#36824,#36825,#36826,#36827,#36828,#36829,#36830,#36831,
#36832,#36833,#36834,#36835,#36836,#36837,#36838,#36839,#36840,#36841,#36842,
#36843,#36844,#36845,#36846,#36847,#36848,#36849,#36850,#36851,#36852,#36853,
#36854,#36855,#36856,#36857,#36858,#36859,#36860,#36861,#36862,#36863,#36864,
#36865,#36866,#36867,#36868,#36869,#36870,#36871,#36872,#36873,#36874,#36875,
#36876,#36877,#36878,#36879,#36880,#36881,#36882,#36883,#36884,#36885,#36886,
#36887,#36888,#36889,#36890,#36891,#36892,#36893,#36894,#36895,#36896,#36897,
#36898,#36899,#36900,#36901,#36902,#36903,#36904,#36905,#36906,#36907,#36908,
#36909,#36910,#36911,#36912,#36913,#36914,#36915,#36916,#36917,#36918,#36919,
#36920,#36921,#36922,#36923,#36924,#36925,#36926,#36927,#36928,#36929,#36930,
#36931,#36932,#36933,#36934,#36935,#36936,#36937,#36938,#36939,#36940,#36941,
#36942,#36943,#36944,#36945,#36946,#36947,#36948,#36949,#36950,#36951,#36952,
#36953,#36954,#36955,#36956,#36957,#36958,#36959,#36960,#36961,#36962,#36963,
#36964,#36965,#36966,#36967,#36968,#36969,#36970,#36971,#36972,#36973,#36974,
#36975,#36976,#36977,#36978,#36979,#36980,#36981,#36982,#36983,#36984,#36985,
#36986,#36987,#36988,#36989,#36990,#36991,#36992,#36993,#36994,#36995,#36996,
#36997,#36998,#36999,#37000,#37001,#37002,#37003,#37004,#37005,#37006,#37007,
#37008,#37009,#37010,#37011,#37012,#37013,#37014,#37015,#37016,#37017,#37018,
#37019,#37020,#37021,#37022,#37023,#37024,#37025,#37026,#37027,#37028,#37029,
#37030,#37031,#37032,#37033,#37034,#37035,#37036,#37037,#37038,#37039,#37040,
#37041,#37042,#37043,#37044,#37045,#37046,#37047,#37048,#37049,#37050,#37051,
#37052,#37053,#37054,#37055,#37056,#37057,#37058,#37059,#37060,#37061,#37062,
#37063,#37064,#37065,#37066,#37067,#37068,#37069,#37070,#37071,#37072,#37073,
#37074,#37075,#37076,#37077,#37078,#37079,#37080,#37081,#37082,#37083,#37084,
#37085,#37086,#37087,#37088,#37089,#37090,#37091,#37092,#37093,#37094,#37095,
#37096,#37097,#37098,#37099,#37100,#37101,#37102,#37103,#37104,#37105,#37106,
#37107,#37108,#37109,#37110,#37111,#37112,#37113,#37114,#37115,#37116,#37117,
#37118,#37119,#37120,#37121,#37122,#37123,#37124,#37125,#37126,#37127,#37128,
#37129,#37130,#37131,#37132,#37133,#37134,#37135,#37136,#37137,#37138,#37139,
#37140,#37141,#37142,#37143,#37144,#37145,#37146,#37147,#37148,#37149,#37150,
#37151,#37152,#37153,#37154,#37155,#37156,#37157,#37158,#37159,#37160,#37161,
#37162,#37163,#37164,#37165,#37166,#37167,#37168,#37169,#37170,#37171,#37172,
#37173,#37174,#37175,#37176,#37177,#37178,#37179,#37180,#37181,#37182,#37183,
#37184,#37185,#37186,#37187,#37188,#37189,#37190,#37191,#37192,#37193,#37194,
#37195,#37196,#37197,#37198,#37199,#37200,#37201,#37202,#37203,#37204,#37205,
#37206,#37207,#37208,#37209,#37210,#37211,#37212,#37213,#37214,#37215,#37216,
#37217,#37218,#37219,#37220,#37221,#37222,#37223,#37224,#37225,#37226,#37227,
#37228,#37229,#37230,#37231,#37232,#37233,#37234,#37235,#37236,#37237,#37238,
#37239,#37240,#37241,#37242,#37243,#37244,#37245,#37246,#37247,#37248,#37249,
#37250,#37251,#37252,#37253,#37254,#37255,#37256,#37257,#37258,#37259,#37260,
#37261,#37262,#37263,#37264,#37265,#37266,#37267,#37268,#37269,#37270,#37271,
#37272,#37273,#37274,#37275,#37276,#37277,#37278,#37279),(#37280,#37281,
#37282,#37283,#37284,#37285,#37286,#37287,#37288,#37289,#37290,#37291,#37292,
#37293,#37294,#37295,#37296,#37297,#37298,#37299,#37300,#37301,#37302,#37303,
#37304,#37305,#37306,#37307,#37308,#37309,#37310,#37311,#37312,#37313,#37314,
#37315,#37316,#37317,#37318,#37319,#37320,#37321,#37322,#37323,#37324,#37325,
#37326,#37327,#37328,#37329,#37330,#37331,#37332,#37333,#37334,#37335,#37336,
#37337,#37338,#37339,#37340,#37341,#37342,#37343,#37344,#37345,#37346,#37347,
#37348,#37349,#37350,#37351,#37352,#37353,#37354,#37355,#37356,#37357,#37358,
#37359,#37360,#37361,#37362,#37363,#37364,#37365,#37366,#37367,#37368,#37369,
#37370,#37371,#37372,#37373,#37374,#37375,#37376,#37377,#37378,#37379,#37380,
#37381,#37382,#37383,#37384,#37385,#37386,#37387,#37388,#37389,#37390,#37391,
#37392,#37393,#37394,#37395,#37396,#37397,#37398,#37399,#37400,#37401,#37402,
#37403,#37404,#37405,#37406,#37407,#37408,#37409,#37410,#37411,#37412,#37413,
#37414,#37415,#37416,#37417,#37418,#37419,#37420,#37421,#37422,#37423,#37424,
#37425,#37426,#37427,#37428,#37429,#37430,#37431,#37432,#37433,#37434,#37435,
#37436,#37437,#37438,#37439,#37440,#37441,#37442,#37443,#37444,#37445,#37446,
#37447,#37448,#37449,#37450,#37451,#37452,#37453,#37454,#37455,#37456,#37457,
#37458,#37459,#37460,#37461,#37462,#37463,#37464,#37465,#37466,#37467,#37468,
#37469,#37470,#37471,#37472,#37473,#37474,#37475,#37476,#37477,#37478,#37479,
#37480,#37481,#37482,#37483,#37484,#37485,#37486,#37487,#37488,#37489,#37490,
#37491,#37492,#37493,#37494,#37495,#37496,#37497,#37498,#37499,#37500,#37501,
#37502,#37503,#37504,#37505,#37506,#37507,#37508,#37509,#37510,#37511,#37512,
#37513,#37514,#37515,#37516,#37517,#37518,#37519,#37520,#37521,#37522,#37523,
#37524,#37525,#37526,#37527,#37528,#37529,#37530,#37531,#37532,#37533,#37534,
#37535,#37536,#37537,#37538,#37539,#37540,#37541,#37542,#37543,#37544,#37545,
#37546,#37547,#37548,#37549,#37550,#37551,#37552,#37553,#37554,#37555,#37556,
#37557,#37558,#37559,#37560,#37561,#37562,#37563,#37564,#37565,#37566,#37567,
#37568,#37569,#37570,#37571,#37572,#37573,#37574,#37575,#37576,#37577,#37578,
#37579,#37580,#37581,#37582,#37583,#37584,#37585,#37586,#37587,#37588,#37589,
#37590,#37591,#37592,#37593,#37594,#37595,#37596,#37597,#37598,#37599,#37600,
#37601,#37602,#37603,#37604,#37605,#37606,#37607,#37608,#37609,#37610,#37611,
#37612,#37613,#37614,#37615,#37616,#37617,#37618,#37619,#37620,#37621,#37622,
#37623,#37624,#37625,#37626,#37627,#37628,#37629,#37630,#37631,#37632,#37633,
#37634,#37635,#37636,#37637,#37638,#37639,#37640,#37641,#37642,#37643,#37644,
#37645,#37646,#37647,#37648,#37649,#37650,#37651,#37652,#37653,#37654,#37655,
#37656,#37657,#37658,#37659,#37660,#37661,#37662,#37663,#37664,#37665,#37666,
#37667,#37668,#37669,#37670,#37671,#37672,#37673,#37674,#37675,#37676,#37677,
#37678,#37679,#37680,#37681,#37682,#37683,#37684,#37685,#37686,#37687,#37688,
#37689,#37690,#37691,#37692,#37693,#37694,#37695,#37696,#37697,#37698,#37699,
#37700,#37701,#37702,#37703,#37704,#37705,#37706,#37707,#37708,#37709,#37710,
#37711,#37712,#37713,#37714,#37715,#37716,#37717,#37718,#37719,#37720,#37721,
#37722,#37723,#37724,#37725,#37726,#37727,#37728,#37729,#37730,#37731,#37732,
#37733,#37734,#37735,#37736,#37737,#37738,#37739,#37740,#37741,#37742,#37743,
#37744,#37745,#37746,#37747,#37748,#37749,#37750,#37751,#37752,#37753,#37754,
#37755,#37756,#37757,#37758,#37759,#37760,#37761,#37762,#37763,#37764,#37765,
#37766,#37767,#37768,#37769,#37770,#37771,#37772,#37773,#37774,#37775,#37776,
#37777,#37778,#37779,#37780,#37781,#37782,#37783,#37784,#37785,#37786,#37787,
#37788,#37789,#37790,#37791,#37792)),.UNSPECIFIED.,.F.,.F.,.F.,(4,4),(4,
1,1,1,1,1,1,1,1,1,1,1,1,1,1,1,1,1,1,1,1,1,1,1,1,1,1,1,1,1,1,1,1,1,1,1,1,
1,1,1,1,1,1,1,1,1,1,1,1,1,1,1,1,1,1,1,1,1,1,1,1,1,1,1,1,1,1,1,1,1,1,1,1,
1,1,1,1,1,1,1,1,1,1,1,1,1,1,1,1,1,1,1,1,1,1,1,1,1,1,1,1,1,1,1,1,1,1,1,1,
1,1,1,1,1,1,1,1,1,1,1,1,1,1,1,1,1,1,1,1,1,1,1,1,1,1,1,1,1,1,1,1,1,1,1,1,
1,1,1,1,1,1,1,1,1,1,1,1,1,1,1,1,1,1,1,1,1,1,1,1,1,1,1,1,1,1,1,1,1,1,1,1,
1,1,1,1,1,1,1,1,1,1,1,1,1,1,1,1,1,1,1,1,1,1,1,1,1,1,1,1,1,1,1,1,1,1,1,1,
1,1,1,1,1,1,1,1,1,1,1,1,1,1,1,1,1,1,1,1,1,1,1,1,1,1,1,1,1,1,1,1,1,1,1,1,
1,1,1,1,1,1,1,1,1,1,1,1,1,1,1,1,1,1,1,1,1,1,1,1,1,1,1,1,1,1,1,1,1,1,1,1,
1,1,1,1,1,1,1,1,1,1,1,1,1,1,1,1,1,1,1,1,1,1,1,1,1,1,1,1,1,1,1,1,1,1,1,1,
1,1,1,1,1,1,1,1,1,1,1,1,1,1,1,1,1,1,1,1,1,1,1,1,1,1,1,1,1,1,1,1,1,1,1,1,
1,1,1,1,1,1,1,1,1,1,1,1,1,1,1,1,1,1,1,1,1,1,1,1,1,1,1,1,1,1,1,1,1,1,1,1,
1,1,1,1,1,1,1,1,1,1,1,1,1,1,1,1,1,1,1,1,1,1,1,1,1,1,1,1,1,1,1,1,1,1,1,1,
1,1,1,1,1,1,1,1,1,1,1,1,1,1,1,1,1,1,1,1,1,1,1,1,1,1,1,1,1,1,1,1,1,1,1,1,
1,1,1,1,1,1,1,1,1,1,1,1,1,1,1,1,1,1,1,1,1,1,1,1,1,1,1,1,1,1,1,1,1,1,1,1,
1,1,1,1,1,4),(0.,0.082416750926819),(11.1008888355104,11.5998029140446,
12.0987169925787,12.5976310711128,13.096545149647,14.0943733067152,15.0922014637835,
16.0900296208517,16.5889436993859,17.08785777792,17.5867718564541,18.0856859349882,
19.0835140920565,20.0813422491248,21.079170406193,22.0769985632613,23.0748267203295,
23.5737407988637,24.0726548773978,24.5715689559319,25.070483034466,26.0683111915343,
27.0661393486026,28.0639675056708,29.0617956627391,30.0596238198073,30.5585378983415,
31.0574519768756,31.5563660554097,32.0552801339438,33.0531082910121,34.0509364480804,
35.0487646051486,36.0465927622169,37.0444209192851,37.5433349978193,38.0422490763534,
38.5411631548875,39.0400772334217,40.0379053904899,41.0357335475582,42.0335617046264,
43.0313898616947,44.0292180187629,44.5281320972971,45.0270461758312,45.5259602543653,
46.0248743328995,47.0227024899677,48.020530647036,49.0183588041042,50.0161869611725,
51.0140151182407,51.5129291967749,52.011843275309,52.5107573538431,53.0096714323773,
54.0074995894455,55.0053277465138,56.003155903582,57.0009840606503,57.9988122177186,
58.4977262962527,58.9966403747868,59.4955544533209,59.9944685318551,60.9922966889233,
61.9901248459916,62.9879530030598,63.9857811601281,64.9836093171964,65.4825233957305,
65.9814374742646,66.4803515527987,66.9792656313329,67.9770937884011,68.9749219454694,
69.9727501025376,70.9705782596059,71.9684064166742,72.4673204952083,72.9662345737424,
73.4651486522765,73.9640627308107,74.9618908878789,75.9597190449472,76.9575472020154,
77.9553753590837,78.953203516152,79.4521175946861,79.9510316732202,80.4499457517543,
80.9488598302885,81.9466879873567,82.944516144425,83.9423443014932,84.9401724585615,
85.9380006156298,86.4369146941639,86.935828772698,87.4347428512321,87.9336569297663,
88.9314850868345,89.9293132439028,90.927141400971,91.9249695580393,92.9227977151076,
93.4217117936417,93.9206258721758,94.4195399507099,94.9184540292441,95.9162821863123,
96.9141103433806,97.9119385004489,98.9097666575171,99.9075948145854,100.406508893119,
100.905422971654,101.404337050188,101.903251128722,102.90107928579,103.898907442858,
104.896735599927,105.894563756995,106.892391914063,107.391305992597,107.890220071131,
108.389134149666,108.8880482282,109.885876385268,110.883704542336,111.881532699404,
112.879360856473,113.877189013541,114.376103092075,114.875017170609,115.373931249143,
115.872845327677,116.870673484746,117.868501641814,118.866329798882,119.864157955951,
120.861986113019,121.360900191553,121.859814270087,122.358728348621,122.857642427155,
123.855470584224,124.853298741292,125.85112689836,126.848955055428,127.846783212497,
128.345697291031,128.844611369565,129.343525448099,129.842439526633,130.840267683701,
131.83809584077,132.835923997838,133.833752154906,134.831580311974,135.330494390509,
135.829408469043,136.328322547577,136.827236626111,137.825064783179,138.822892940247,
139.820721097316,140.818549254384,141.816377411452,142.315291489986,142.81420556852,
143.313119647055,143.812033725589,144.809861882657,145.807690039725,146.805518196793,
147.803346353862,148.80117451093,149.300088589464,149.799002667998,150.297916746532,
150.796830825067,151.794658982135,152.792487139203,153.790315296271,154.78814345334,
155.785971610408,156.284885688942,156.783799767476,157.28271384601,157.781627924544,
158.779456081613,159.777284238681,160.775112395749,161.772940552817,162.770768709886,
163.26968278842,163.768596866954,164.267510945488,164.766425024022,165.76425318109,
166.762081338159,167.759909495227,168.757737652295,169.755565809363,170.254479887898,
170.753393966432,171.252308044966,171.7512221235,172.749050280568,173.746878437636,
174.744706594705,175.742534751773,176.740362908841,177.239276987375,177.738191065909,
178.237105144444,178.736019222978,179.733847380046,180.731675537114,181.729503694182,
182.727331851251,183.725160008319,184.224074086853,184.722988165387,185.221902243921,
185.720816322456,186.718644479524,187.716472636592,188.71430079366,189.712128950729,
190.709957107797,191.208871186331,191.707785264865,192.206699343399,192.705613421933,
193.703441579002,194.70126973607,195.699097893138,196.696926050206,197.694754207275,
198.193668285809,198.692582364343,199.191496442877,199.690410521411,200.688238678479,
201.686066835548,202.683894992616,203.681723149684,204.679551306752,205.178465385287,
205.677379463821,206.176293542355,206.675207620889,207.673035777957,208.670863935025,
209.668692092094,210.666520249162,211.66434840623,212.662176563298,213.161090641833,
213.660004720367,214.657832877435,215.655661034503,216.653489191572,217.152403270106,
217.65131734864,218.150231427174,218.649145505708,219.646973662776,220.644801819845,
221.642629976913,222.640458133981,223.638286291049,224.137200369583,224.636114448118,
225.135028526652,225.633942605186,226.631770762254,227.629598919322,228.627427076391,
229.625255233459,230.623083390527,231.121997469061,231.620911547595,232.11982562613,
232.618739704664,233.616567861732,234.6143960188,235.612224175868,236.610052332937,
237.607880490005,238.106794568539,238.605708647073,239.104622725607,239.603536804141,
240.60136496121,241.599193118278,242.597021275346,243.594849432414,244.592677589483,
245.091591668017,245.590505746551,246.089419825085,246.588333903619,247.586162060688,
248.583990217756,249.581818374824,250.579646531892,251.577474688961,252.076388767495,
252.575302846029,253.074216924563,253.573131003097,254.570959160165,255.568787317234,
256.566615474302,257.56444363137,258.562271788438,259.061185866972,259.560099945507,
260.059014024041,260.557928102575,261.555756259643,262.553584416711,263.55141257378,
264.549240730848,265.547068887916,266.04598296645,266.544897044984,267.043811123519,
267.542725202053,268.540553359121,269.538381516189,270.536209673257,271.534037830326,
272.531865987394,273.030780065928,273.529694144462,274.028608222996,274.52752230153,
275.525350458599,276.523178615667,277.521006772735,278.518834929803,279.516663086872,
280.015577165406,280.51449124394,281.013405322474,281.512319401008,282.510147558077,
283.507975715145,284.505803872213,285.503632029281,286.50146018635,287.000374264884,
287.499288343418,287.998202421952,288.497116500486,289.494944657554,290.492772814623,
291.490600971691,292.488429128759,293.486257285827,293.985171364361,294.484085442896,
294.98299952143,295.481913599964,296.479741757032,297.4775699141,298.475398071169,
299.473226228237,300.471054385305,300.969968463839,301.468882542373,301.967796620908,
302.466710699442,303.46453885651,304.462367013578,305.460195170646,306.458023327715,
307.455851484783,307.954765563317,308.453679641851,308.952593720385,309.451507798919,
310.449335955988,311.447164113056,312.444992270124,313.442820427192,314.440648584261,
314.939562662795,315.438476741329,315.937390819863,316.436304898397,317.434133055466,
318.431961212534,319.429789369602,320.42761752667,321.425445683739,321.924359762273,
322.423273840807,322.922187919341,323.421101997875,324.418930154943,325.416758312012,
326.41458646908,327.412414626148,328.410242783216,328.90915686175,329.408070940285,
329.906985018819,330.405899097353,331.403727254421,332.401555411489,333.399383568558,
334.397211725626,335.395039882694,335.893953961228,336.392868039762,336.891782118297,
337.390696196831,338.388524353899,339.386352510967,340.384180668035,341.382008825104,
342.379836982172,342.878751060706,343.37766513924,343.876579217774,344.375493296308,
345.373321453377,346.371149610445,347.368977767513,348.366805924582,349.36463408165,
349.863548160184,350.362462238718,350.861376317252,351.360290395786,352.358118552855,
353.355946709923,354.353774866991,355.351603024059,356.349431181128,356.848345259662,
357.347259338196,357.84617341673,358.345087495264,359.342915652332,360.340743809401,
361.338571966469,362.336400123537,363.334228280605,363.83314235914,364.332056437674,
364.830970516208,365.329884594742,366.32771275181,367.325540908878,368.323369065947,
369.321197223015,370.319025380083,370.817939458617,371.316853537151,371.815767615686,
372.31468169422,373.312509851288,374.310338008356,375.308166165424,376.305994322493,
377.303822479561,377.802736558095,378.301650636629,378.800564715163,379.299478793698,
380.297306950766,381.295135107834,382.292963264902,383.290791421971,384.288619579039,
384.787533657573,385.286447736107,385.785361814641,386.284275893175,387.282104050244,
388.279932207312,389.27776036438,390.275588521448,391.273416678517,391.772330757051,
392.271244835585,392.770158914119,393.269072992653,394.266901149721,395.26472930679,
396.262557463858,397.260385620926,398.258213777994,398.757127856529,399.256041935063,
399.754956013597,400.253870092131,401.251698249199,402.249526406267,403.247354563336,
403.74626864187,404.245182720404,404.744096798938,405.243010877472),
 .UNSPECIFIED.);
#835=B_SPLINE_SURFACE_WITH_KNOTS('',3,3,((#38059,#38060,#38061,#38062,#38063,
#38064,#38065,#38066,#38067,#38068,#38069,#38070,#38071,#38072,#38073,#38074,
#38075,#38076,#38077,#38078,#38079,#38080,#38081,#38082,#38083,#38084,#38085,
#38086,#38087,#38088,#38089,#38090,#38091,#38092,#38093,#38094,#38095,#38096,
#38097,#38098,#38099,#38100,#38101,#38102,#38103,#38104,#38105,#38106,#38107,
#38108,#38109,#38110,#38111,#38112,#38113,#38114,#38115,#38116,#38117,#38118,
#38119,#38120,#38121,#38122,#38123,#38124,#38125,#38126,#38127,#38128,#38129,
#38130,#38131,#38132,#38133,#38134,#38135,#38136,#38137,#38138,#38139,#38140,
#38141,#38142,#38143,#38144,#38145,#38146,#38147,#38148,#38149,#38150,#38151,
#38152,#38153,#38154,#38155,#38156,#38157,#38158,#38159,#38160,#38161,#38162,
#38163,#38164,#38165,#38166,#38167,#38168,#38169,#38170,#38171,#38172,#38173,
#38174,#38175,#38176,#38177,#38178,#38179,#38180,#38181,#38182,#38183,#38184,
#38185,#38186,#38187,#38188,#38189,#38190,#38191,#38192,#38193,#38194,#38195,
#38196,#38197,#38198,#38199,#38200,#38201,#38202,#38203,#38204,#38205,#38206,
#38207,#38208,#38209,#38210,#38211,#38212,#38213,#38214,#38215,#38216,#38217,
#38218,#38219,#38220,#38221,#38222,#38223,#38224,#38225,#38226,#38227,#38228,
#38229,#38230,#38231,#38232,#38233,#38234,#38235,#38236,#38237,#38238,#38239,
#38240,#38241,#38242,#38243,#38244,#38245,#38246,#38247,#38248,#38249,#38250,
#38251,#38252,#38253,#38254,#38255,#38256,#38257,#38258,#38259,#38260,#38261,
#38262,#38263,#38264,#38265,#38266,#38267,#38268,#38269,#38270,#38271,#38272,
#38273,#38274,#38275,#38276,#38277,#38278,#38279,#38280,#38281,#38282,#38283,
#38284,#38285,#38286,#38287,#38288,#38289,#38290,#38291,#38292,#38293,#38294,
#38295,#38296,#38297,#38298,#38299,#38300,#38301,#38302,#38303,#38304,#38305,
#38306,#38307,#38308,#38309,#38310,#38311,#38312,#38313,#38314,#38315,#38316,
#38317,#38318,#38319,#38320,#38321,#38322,#38323,#38324,#38325,#38326,#38327,
#38328,#38329,#38330,#38331,#38332,#38333,#38334,#38335,#38336,#38337,#38338,
#38339,#38340,#38341,#38342,#38343,#38344,#38345,#38346,#38347,#38348,#38349,
#38350,#38351,#38352,#38353,#38354,#38355,#38356,#38357,#38358,#38359,#38360,
#38361,#38362,#38363,#38364,#38365,#38366,#38367,#38368,#38369,#38370,#38371,
#38372,#38373,#38374,#38375,#38376,#38377,#38378,#38379,#38380,#38381,#38382,
#38383,#38384,#38385,#38386,#38387,#38388,#38389,#38390,#38391,#38392,#38393,
#38394,#38395,#38396,#38397,#38398,#38399,#38400,#38401,#38402,#38403,#38404,
#38405,#38406,#38407,#38408,#38409,#38410,#38411,#38412,#38413,#38414,#38415,
#38416,#38417,#38418,#38419,#38420,#38421,#38422,#38423,#38424,#38425,#38426,
#38427,#38428,#38429,#38430,#38431,#38432,#38433,#38434,#38435,#38436,#38437,
#38438,#38439,#38440,#38441,#38442,#38443,#38444,#38445,#38446,#38447,#38448,
#38449,#38450,#38451,#38452,#38453,#38454,#38455,#38456,#38457,#38458,#38459,
#38460,#38461,#38462,#38463,#38464,#38465,#38466,#38467,#38468,#38469,#38470,
#38471,#38472,#38473,#38474,#38475,#38476,#38477,#38478,#38479,#38480,#38481,
#38482,#38483,#38484,#38485,#38486,#38487,#38488,#38489,#38490,#38491,#38492,
#38493,#38494,#38495,#38496,#38497,#38498,#38499,#38500,#38501,#38502,#38503,
#38504,#38505,#38506,#38507,#38508,#38509,#38510,#38511,#38512,#38513,#38514,
#38515,#38516,#38517,#38518,#38519,#38520,#38521,#38522,#38523,#38524,#38525,
#38526,#38527,#38528,#38529,#38530,#38531,#38532,#38533,#38534,#38535,#38536,
#38537,#38538,#38539,#38540,#38541,#38542,#38543,#38544,#38545,#38546,#38547,
#38548,#38549,#38550,#38551,#38552,#38553,#38554,#38555,#38556,#38557,#38558,
#38559,#38560,#38561,#38562,#38563,#38564,#38565,#38566,#38567,#38568,#38569,
#38570,#38571),(#38572,#38573,#38574,#38575,#38576,#38577,#38578,#38579,
#38580,#38581,#38582,#38583,#38584,#38585,#38586,#38587,#38588,#38589,#38590,
#38591,#38592,#38593,#38594,#38595,#38596,#38597,#38598,#38599,#38600,#38601,
#38602,#38603,#38604,#38605,#38606,#38607,#38608,#38609,#38610,#38611,#38612,
#38613,#38614,#38615,#38616,#38617,#38618,#38619,#38620,#38621,#38622,#38623,
#38624,#38625,#38626,#38627,#38628,#38629,#38630,#38631,#38632,#38633,#38634,
#38635,#38636,#38637,#38638,#38639,#38640,#38641,#38642,#38643,#38644,#38645,
#38646,#38647,#38648,#38649,#38650,#38651,#38652,#38653,#38654,#38655,#38656,
#38657,#38658,#38659,#38660,#38661,#38662,#38663,#38664,#38665,#38666,#38667,
#38668,#38669,#38670,#38671,#38672,#38673,#38674,#38675,#38676,#38677,#38678,
#38679,#38680,#38681,#38682,#38683,#38684,#38685,#38686,#38687,#38688,#38689,
#38690,#38691,#38692,#38693,#38694,#38695,#38696,#38697,#38698,#38699,#38700,
#38701,#38702,#38703,#38704,#38705,#38706,#38707,#38708,#38709,#38710,#38711,
#38712,#38713,#38714,#38715,#38716,#38717,#38718,#38719,#38720,#38721,#38722,
#38723,#38724,#38725,#38726,#38727,#38728,#38729,#38730,#38731,#38732,#38733,
#38734,#38735,#38736,#38737,#38738,#38739,#38740,#38741,#38742,#38743,#38744,
#38745,#38746,#38747,#38748,#38749,#38750,#38751,#38752,#38753,#38754,#38755,
#38756,#38757,#38758,#38759,#38760,#38761,#38762,#38763,#38764,#38765,#38766,
#38767,#38768,#38769,#38770,#38771,#38772,#38773,#38774,#38775,#38776,#38777,
#38778,#38779,#38780,#38781,#38782,#38783,#38784,#38785,#38786,#38787,#38788,
#38789,#38790,#38791,#38792,#38793,#38794,#38795,#38796,#38797,#38798,#38799,
#38800,#38801,#38802,#38803,#38804,#38805,#38806,#38807,#38808,#38809,#38810,
#38811,#38812,#38813,#38814,#38815,#38816,#38817,#38818,#38819,#38820,#38821,
#38822,#38823,#38824,#38825,#38826,#38827,#38828,#38829,#38830,#38831,#38832,
#38833,#38834,#38835,#38836,#38837,#38838,#38839,#38840,#38841,#38842,#38843,
#38844,#38845,#38846,#38847,#38848,#38849,#38850,#38851,#38852,#38853,#38854,
#38855,#38856,#38857,#38858,#38859,#38860,#38861,#38862,#38863,#38864,#38865,
#38866,#38867,#38868,#38869,#38870,#38871,#38872,#38873,#38874,#38875,#38876,
#38877,#38878,#38879,#38880,#38881,#38882,#38883,#38884,#38885,#38886,#38887,
#38888,#38889,#38890,#38891,#38892,#38893,#38894,#38895,#38896,#38897,#38898,
#38899,#38900,#38901,#38902,#38903,#38904,#38905,#38906,#38907,#38908,#38909,
#38910,#38911,#38912,#38913,#38914,#38915,#38916,#38917,#38918,#38919,#38920,
#38921,#38922,#38923,#38924,#38925,#38926,#38927,#38928,#38929,#38930,#38931,
#38932,#38933,#38934,#38935,#38936,#38937,#38938,#38939,#38940,#38941,#38942,
#38943,#38944,#38945,#38946,#38947,#38948,#38949,#38950,#38951,#38952,#38953,
#38954,#38955,#38956,#38957,#38958,#38959,#38960,#38961,#38962,#38963,#38964,
#38965,#38966,#38967,#38968,#38969,#38970,#38971,#38972,#38973,#38974,#38975,
#38976,#38977,#38978,#38979,#38980,#38981,#38982,#38983,#38984,#38985,#38986,
#38987,#38988,#38989,#38990,#38991,#38992,#38993,#38994,#38995,#38996,#38997,
#38998,#38999,#39000,#39001,#39002,#39003,#39004,#39005,#39006,#39007,#39008,
#39009,#39010,#39011,#39012,#39013,#39014,#39015,#39016,#39017,#39018,#39019,
#39020,#39021,#39022,#39023,#39024,#39025,#39026,#39027,#39028,#39029,#39030,
#39031,#39032,#39033,#39034,#39035,#39036,#39037,#39038,#39039,#39040,#39041,
#39042,#39043,#39044,#39045,#39046,#39047,#39048,#39049,#39050,#39051,#39052,
#39053,#39054,#39055,#39056,#39057,#39058,#39059,#39060,#39061,#39062,#39063,
#39064,#39065,#39066,#39067,#39068,#39069,#39070,#39071,#39072,#39073,#39074,
#39075,#39076,#39077,#39078,#39079,#39080,#39081,#39082,#39083,#39084),
(#39085,#39086,#39087,#39088,#39089,#39090,#39091,#39092,#39093,#39094,
#39095,#39096,#39097,#39098,#39099,#39100,#39101,#39102,#39103,#39104,#39105,
#39106,#39107,#39108,#39109,#39110,#39111,#39112,#39113,#39114,#39115,#39116,
#39117,#39118,#39119,#39120,#39121,#39122,#39123,#39124,#39125,#39126,#39127,
#39128,#39129,#39130,#39131,#39132,#39133,#39134,#39135,#39136,#39137,#39138,
#39139,#39140,#39141,#39142,#39143,#39144,#39145,#39146,#39147,#39148,#39149,
#39150,#39151,#39152,#39153,#39154,#39155,#39156,#39157,#39158,#39159,#39160,
#39161,#39162,#39163,#39164,#39165,#39166,#39167,#39168,#39169,#39170,#39171,
#39172,#39173,#39174,#39175,#39176,#39177,#39178,#39179,#39180,#39181,#39182,
#39183,#39184,#39185,#39186,#39187,#39188,#39189,#39190,#39191,#39192,#39193,
#39194,#39195,#39196,#39197,#39198,#39199,#39200,#39201,#39202,#39203,#39204,
#39205,#39206,#39207,#39208,#39209,#39210,#39211,#39212,#39213,#39214,#39215,
#39216,#39217,#39218,#39219,#39220,#39221,#39222,#39223,#39224,#39225,#39226,
#39227,#39228,#39229,#39230,#39231,#39232,#39233,#39234,#39235,#39236,#39237,
#39238,#39239,#39240,#39241,#39242,#39243,#39244,#39245,#39246,#39247,#39248,
#39249,#39250,#39251,#39252,#39253,#39254,#39255,#39256,#39257,#39258,#39259,
#39260,#39261,#39262,#39263,#39264,#39265,#39266,#39267,#39268,#39269,#39270,
#39271,#39272,#39273,#39274,#39275,#39276,#39277,#39278,#39279,#39280,#39281,
#39282,#39283,#39284,#39285,#39286,#39287,#39288,#39289,#39290,#39291,#39292,
#39293,#39294,#39295,#39296,#39297,#39298,#39299,#39300,#39301,#39302,#39303,
#39304,#39305,#39306,#39307,#39308,#39309,#39310,#39311,#39312,#39313,#39314,
#39315,#39316,#39317,#39318,#39319,#39320,#39321,#39322,#39323,#39324,#39325,
#39326,#39327,#39328,#39329,#39330,#39331,#39332,#39333,#39334,#39335,#39336,
#39337,#39338,#39339,#39340,#39341,#39342,#39343,#39344,#39345,#39346,#39347,
#39348,#39349,#39350,#39351,#39352,#39353,#39354,#39355,#39356,#39357,#39358,
#39359,#39360,#39361,#39362,#39363,#39364,#39365,#39366,#39367,#39368,#39369,
#39370,#39371,#39372,#39373,#39374,#39375,#39376,#39377,#39378,#39379,#39380,
#39381,#39382,#39383,#39384,#39385,#39386,#39387,#39388,#39389,#39390,#39391,
#39392,#39393,#39394,#39395,#39396,#39397,#39398,#39399,#39400,#39401,#39402,
#39403,#39404,#39405,#39406,#39407,#39408,#39409,#39410,#39411,#39412,#39413,
#39414,#39415,#39416,#39417,#39418,#39419,#39420,#39421,#39422,#39423,#39424,
#39425,#39426,#39427,#39428,#39429,#39430,#39431,#39432,#39433,#39434,#39435,
#39436,#39437,#39438,#39439,#39440,#39441,#39442,#39443,#39444,#39445,#39446,
#39447,#39448,#39449,#39450,#39451,#39452,#39453,#39454,#39455,#39456,#39457,
#39458,#39459,#39460,#39461,#39462,#39463,#39464,#39465,#39466,#39467,#39468,
#39469,#39470,#39471,#39472,#39473,#39474,#39475,#39476,#39477,#39478,#39479,
#39480,#39481,#39482,#39483,#39484,#39485,#39486,#39487,#39488,#39489,#39490,
#39491,#39492,#39493,#39494,#39495,#39496,#39497,#39498,#39499,#39500,#39501,
#39502,#39503,#39504,#39505,#39506,#39507,#39508,#39509,#39510,#39511,#39512,
#39513,#39514,#39515,#39516,#39517,#39518,#39519,#39520,#39521,#39522,#39523,
#39524,#39525,#39526,#39527,#39528,#39529,#39530,#39531,#39532,#39533,#39534,
#39535,#39536,#39537,#39538,#39539,#39540,#39541,#39542,#39543,#39544,#39545,
#39546,#39547,#39548,#39549,#39550,#39551,#39552,#39553,#39554,#39555,#39556,
#39557,#39558,#39559,#39560,#39561,#39562,#39563,#39564,#39565,#39566,#39567,
#39568,#39569,#39570,#39571,#39572,#39573,#39574,#39575,#39576,#39577,#39578,
#39579,#39580,#39581,#39582,#39583,#39584,#39585,#39586,#39587,#39588,#39589,
#39590,#39591,#39592,#39593,#39594,#39595,#39596,#39597),(#39598,#39599,
#39600,#39601,#39602,#39603,#39604,#39605,#39606,#39607,#39608,#39609,#39610,
#39611,#39612,#39613,#39614,#39615,#39616,#39617,#39618,#39619,#39620,#39621,
#39622,#39623,#39624,#39625,#39626,#39627,#39628,#39629,#39630,#39631,#39632,
#39633,#39634,#39635,#39636,#39637,#39638,#39639,#39640,#39641,#39642,#39643,
#39644,#39645,#39646,#39647,#39648,#39649,#39650,#39651,#39652,#39653,#39654,
#39655,#39656,#39657,#39658,#39659,#39660,#39661,#39662,#39663,#39664,#39665,
#39666,#39667,#39668,#39669,#39670,#39671,#39672,#39673,#39674,#39675,#39676,
#39677,#39678,#39679,#39680,#39681,#39682,#39683,#39684,#39685,#39686,#39687,
#39688,#39689,#39690,#39691,#39692,#39693,#39694,#39695,#39696,#39697,#39698,
#39699,#39700,#39701,#39702,#39703,#39704,#39705,#39706,#39707,#39708,#39709,
#39710,#39711,#39712,#39713,#39714,#39715,#39716,#39717,#39718,#39719,#39720,
#39721,#39722,#39723,#39724,#39725,#39726,#39727,#39728,#39729,#39730,#39731,
#39732,#39733,#39734,#39735,#39736,#39737,#39738,#39739,#39740,#39741,#39742,
#39743,#39744,#39745,#39746,#39747,#39748,#39749,#39750,#39751,#39752,#39753,
#39754,#39755,#39756,#39757,#39758,#39759,#39760,#39761,#39762,#39763,#39764,
#39765,#39766,#39767,#39768,#39769,#39770,#39771,#39772,#39773,#39774,#39775,
#39776,#39777,#39778,#39779,#39780,#39781,#39782,#39783,#39784,#39785,#39786,
#39787,#39788,#39789,#39790,#39791,#39792,#39793,#39794,#39795,#39796,#39797,
#39798,#39799,#39800,#39801,#39802,#39803,#39804,#39805,#39806,#39807,#39808,
#39809,#39810,#39811,#39812,#39813,#39814,#39815,#39816,#39817,#39818,#39819,
#39820,#39821,#39822,#39823,#39824,#39825,#39826,#39827,#39828,#39829,#39830,
#39831,#39832,#39833,#39834,#39835,#39836,#39837,#39838,#39839,#39840,#39841,
#39842,#39843,#39844,#39845,#39846,#39847,#39848,#39849,#39850,#39851,#39852,
#39853,#39854,#39855,#39856,#39857,#39858,#39859,#39860,#39861,#39862,#39863,
#39864,#39865,#39866,#39867,#39868,#39869,#39870,#39871,#39872,#39873,#39874,
#39875,#39876,#39877,#39878,#39879,#39880,#39881,#39882,#39883,#39884,#39885,
#39886,#39887,#39888,#39889,#39890,#39891,#39892,#39893,#39894,#39895,#39896,
#39897,#39898,#39899,#39900,#39901,#39902,#39903,#39904,#39905,#39906,#39907,
#39908,#39909,#39910,#39911,#39912,#39913,#39914,#39915,#39916,#39917,#39918,
#39919,#39920,#39921,#39922,#39923,#39924,#39925,#39926,#39927,#39928,#39929,
#39930,#39931,#39932,#39933,#39934,#39935,#39936,#39937,#39938,#39939,#39940,
#39941,#39942,#39943,#39944,#39945,#39946,#39947,#39948,#39949,#39950,#39951,
#39952,#39953,#39954,#39955,#39956,#39957,#39958,#39959,#39960,#39961,#39962,
#39963,#39964,#39965,#39966,#39967,#39968,#39969,#39970,#39971,#39972,#39973,
#39974,#39975,#39976,#39977,#39978,#39979,#39980,#39981,#39982,#39983,#39984,
#39985,#39986,#39987,#39988,#39989,#39990,#39991,#39992,#39993,#39994,#39995,
#39996,#39997,#39998,#39999,#40000,#40001,#40002,#40003,#40004,#40005,#40006,
#40007,#40008,#40009,#40010,#40011,#40012,#40013,#40014,#40015,#40016,#40017,
#40018,#40019,#40020,#40021,#40022,#40023,#40024,#40025,#40026,#40027,#40028,
#40029,#40030,#40031,#40032,#40033,#40034,#40035,#40036,#40037,#40038,#40039,
#40040,#40041,#40042,#40043,#40044,#40045,#40046,#40047,#40048,#40049,#40050,
#40051,#40052,#40053,#40054,#40055,#40056,#40057,#40058,#40059,#40060,#40061,
#40062,#40063,#40064,#40065,#40066,#40067,#40068,#40069,#40070,#40071,#40072,
#40073,#40074,#40075,#40076,#40077,#40078,#40079,#40080,#40081,#40082,#40083,
#40084,#40085,#40086,#40087,#40088,#40089,#40090,#40091,#40092,#40093,#40094,
#40095,#40096,#40097,#40098,#40099,#40100,#40101,#40102,#40103,#40104,#40105,
#40106,#40107,#40108,#40109,#40110)),.UNSPECIFIED.,.F.,.F.,.F.,(4,4),(4,
1,1,1,1,1,1,1,1,1,1,1,1,1,1,1,1,1,1,1,1,1,1,1,1,1,1,1,1,1,1,1,1,1,1,1,1,
1,1,1,1,1,1,1,1,1,1,1,1,1,1,1,1,1,1,1,1,1,1,1,1,1,1,1,1,1,1,1,1,1,1,1,1,
1,1,1,1,1,1,1,1,1,1,1,1,1,1,1,1,1,1,1,1,1,1,1,1,1,1,1,1,1,1,1,1,1,1,1,1,
1,1,1,1,1,1,1,1,1,1,1,1,1,1,1,1,1,1,1,1,1,1,1,1,1,1,1,1,1,1,1,1,1,1,1,1,
1,1,1,1,1,1,1,1,1,1,1,1,1,1,1,1,1,1,1,1,1,1,1,1,1,1,1,1,1,1,1,1,1,1,1,1,
1,1,1,1,1,1,1,1,1,1,1,1,1,1,1,1,1,1,1,1,1,1,1,1,1,1,1,1,1,1,1,1,1,1,1,1,
1,1,1,1,1,1,1,1,1,1,1,1,1,1,1,1,1,1,1,1,1,1,1,1,1,1,1,1,1,1,1,1,1,1,1,1,
1,1,1,1,1,1,1,1,1,1,1,1,1,1,1,1,1,1,1,1,1,1,1,1,1,1,1,1,1,1,1,1,1,1,1,1,
1,1,1,1,1,1,1,1,1,1,1,1,1,1,1,1,1,1,1,1,1,1,1,1,1,1,1,1,1,1,1,1,1,1,1,1,
1,1,1,1,1,1,1,1,1,1,1,1,1,1,1,1,1,1,1,1,1,1,1,1,1,1,1,1,1,1,1,1,1,1,1,1,
1,1,1,1,1,1,1,1,1,1,1,1,1,1,1,1,1,1,1,1,1,1,1,1,1,1,1,1,1,1,1,1,1,1,1,1,
1,1,1,1,1,1,1,1,1,1,1,1,1,1,1,1,1,1,1,1,1,1,1,1,1,1,1,1,1,1,1,1,1,1,1,1,
1,1,1,1,1,1,1,1,1,1,1,1,1,1,1,1,1,1,1,1,1,1,1,1,1,1,1,1,1,1,1,1,1,1,1,1,
1,1,1,1,1,1,1,1,1,1,1,1,1,1,1,1,1,1,1,1,1,1,1,1,1,1,1,1,1,1,1,1,1,1,1,1,
1,1,1,1,1,4),(0.,0.082416750926819),(14.4112373819487,14.9101514604828,
15.4090655390169,15.9079796175511,16.4068936960852,17.4047218531535,18.4025500102217,
19.40037816729,19.8992922458241,20.3982063243582,20.8971204028924,21.3960344814265,
22.3938626384947,23.391690795563,24.3895189526313,25.3873471096995,26.3851752667678,
26.8840893453019,27.383003423836,27.8819175023702,28.3808315809043,29.3786597379725,
30.3764878950408,31.3743160521091,32.3721442091773,33.3699723662456,33.8688864447797,
34.3678005233138,34.866714601848,35.3656286803821,36.3634568374504,37.3612849945186,
38.3591131515869,39.3569413086551,40.3547694657234,40.8536835442575,41.3525976227916,
41.8515117013258,42.3504257798599,43.3482539369282,44.3460820939964,45.3439102510647,
46.3417384081329,47.3395665652012,47.8384806437353,48.3373947222694,48.8363088008036,
49.3352228793377,50.333051036406,51.3308791934742,52.3287073505425,53.3265355076107,
54.324363664679,54.8232777432131,55.3221918217472,55.8211059002814,56.3200199788155,
57.3178481358838,58.315676292952,59.3135044500203,60.3113326070885,61.3091607641568,
61.8080748426909,62.306988921225,62.8059029997592,63.3048170782933,64.3026452353616,
65.3004733924298,66.2983015494981,67.2961297065663,68.2939578636346,68.7928719421687,
69.2917860207028,69.790700099237,70.2896141777711,71.2874423348394,72.2852704919076,
73.2830986489759,74.2809268060441,75.2787549631124,75.7776690416465,76.2765831201806,
76.7754971987148,77.2744112772489,78.2722394343172,79.2700675913854,80.2678957484537,
81.2657239055219,82.2635520625902,82.7624661411243,83.2613802196584,83.7602942981926,
84.2592083767267,85.257036533795,86.2548646908632,87.2526928479315,88.2505210049997,
89.248349162068,89.7472632406021,90.2461773191363,90.7450913976704,91.2440054762045,
92.2418336332728,93.239661790341,94.2374899474093,95.2353181044775,96.2331462615458,
96.7320603400799,97.2309744186141,97.7298884971482,98.2288025756823,99.2266307327506,
100.224458889819,101.222287046887,102.220115203955,103.217943361024,103.716857439558,
104.215771518092,104.714685596626,105.21359967516,106.211427832228,107.209255989297,
108.207084146365,109.204912303433,110.202740460501,110.701654539036,111.20056861757,
111.699482696104,112.198396774638,113.196224931706,114.194053088774,115.191881245843,
116.189709402911,117.187537559979,117.686451638513,118.185365717047,118.684279795582,
119.183193874116,120.181022031184,121.178850188252,122.17667834532,123.174506502389,
124.172334659457,124.671248737991,125.170162816525,125.669076895059,126.167990973594,
127.165819130662,128.16364728773,129.161475444798,130.159303601867,131.157131758935,
131.656045837469,132.154959916003,132.653873994537,133.152788073071,134.15061623014,
135.148444387208,136.146272544276,137.144100701344,138.141928858413,138.640842936947,
139.139757015481,139.638671094015,140.137585172549,141.135413329617,142.133241486686,
143.131069643754,144.128897800822,145.12672595789,145.625640036425,146.124554114959,
146.623468193493,147.122382272027,148.120210429095,149.118038586163,150.115866743232,
151.1136949003,152.111523057368,152.610437135902,153.109351214436,153.608265292971,
154.107179371505,155.105007528573,156.102835685641,157.100663842709,158.098491999778,
159.096320156846,159.59523423538,160.094148313914,160.593062392448,161.091976470983,
162.089804628051,163.087632785119,164.085460942187,165.083289099256,166.081117256324,
166.580031334858,167.078945413392,167.577859491926,168.07677357046,169.074601727529,
170.072429884597,171.070258041665,172.068086198733,173.065914355802,173.564828434336,
174.06374251287,174.562656591404,175.061570669938,176.059398827006,177.057226984075,
178.055055141143,179.052883298211,180.050711455279,180.549625533814,181.048539612348,
181.547453690882,182.046367769416,183.044195926484,184.042024083552,185.039852240621,
186.037680397689,187.035508554757,187.534422633291,188.033336711825,188.53225079036,
189.031164868894,190.028993025962,191.02682118303,192.024649340099,193.022477497167,
194.020305654235,194.519219732769,195.018133811303,195.517047889837,196.015961968372,
197.01379012544,198.011618282508,199.009446439576,200.007274596645,201.005102753713,
201.504016832247,202.002930910781,202.501844989315,203.000759067849,203.998587224918,
204.996415381986,205.994243539054,206.992071696122,207.989899853191,208.488813931725,
208.987728010259,209.486642088793,209.985556167327,210.983384324395,211.981212481464,
212.979040638532,213.9768687956,214.974696952668,215.972525109737,216.471439188271,
216.970353266805,217.968181423873,218.966009580941,219.96383773801,220.462751816544,
220.961665895078,221.460579973612,221.959494052146,222.957322209214,223.955150366283,
224.952978523351,225.950806680419,226.948634837488,227.447548916022,227.946462994556,
228.44537707309,228.944291151624,229.942119308692,230.939947465761,231.937775622829,
232.935603779897,233.933431936965,234.432346015499,234.931260094034,235.430174172568,
235.929088251102,236.92691640817,237.924744565238,238.922572722307,239.920400879375,
240.918229036443,241.417143114977,241.916057193511,242.414971272045,242.91388535058,
243.911713507648,244.909541664716,245.907369821784,246.905197978853,247.903026135921,
248.401940214455,248.900854292989,249.399768371523,249.898682450057,250.896510607126,
251.894338764194,252.892166921262,253.88999507833,254.887823235399,255.386737313933,
255.885651392467,256.384565471001,256.883479549535,257.881307706603,258.879135863672,
259.87696402074,260.874792177808,261.872620334877,262.371534413411,262.870448491945,
263.369362570479,263.868276649013,264.866104806081,265.86393296315,266.861761120218,
267.859589277286,268.857417434354,269.356331512888,269.855245591423,270.354159669957,
270.853073748491,271.850901905559,272.848730062627,273.846558219696,274.844386376764,
275.842214533832,276.341128612366,276.8400426909,277.338956769435,277.837870847969,
278.835699005037,279.833527162105,280.831355319173,281.829183476242,282.82701163331,
283.325925711844,283.824839790378,284.323753868912,284.822667947446,285.820496104515,
286.818324261583,287.816152418651,288.813980575719,289.811808732788,290.310722811322,
290.809636889856,291.30855096839,291.807465046924,292.805293203993,293.803121361061,
294.800949518129,295.798777675197,296.796605832266,297.2955199108,297.794433989334,
298.293348067868,298.792262146402,299.79009030347,300.787918460539,301.785746617607,
302.783574774675,303.781402931743,304.280317010277,304.779231088812,305.278145167346,
305.77705924588,306.774887402948,307.772715560016,308.770543717085,309.768371874153,
310.766200031221,311.265114109755,311.764028188289,312.262942266824,312.761856345358,
313.759684502426,314.757512659494,315.755340816562,316.753168973631,317.750997130699,
318.249911209233,318.748825287767,319.247739366301,319.746653444835,320.744481601904,
321.742309758972,322.74013791604,323.737966073108,324.735794230177,325.234708308711,
325.733622387245,326.232536465779,326.731450544313,327.729278701381,328.72710685845,
329.724935015518,330.722763172586,331.720591329655,332.219505408189,332.718419486723,
333.217333565257,333.716247643791,334.714075800859,335.711903957928,336.709732114996,
337.707560272064,338.705388429132,339.204302507666,339.703216586201,340.202130664735,
340.701044743269,341.698872900337,342.696701057405,343.694529214474,344.692357371542,
345.69018552861,346.189099607144,346.688013685678,347.186927764213,347.685841842747,
348.683669999815,349.681498156883,350.679326313951,351.67715447102,352.674982628088,
353.173896706622,353.672810785156,354.17172486369,354.670638942224,355.668467099293,
356.666295256361,357.664123413429,358.661951570497,359.659779727566,360.1586938061,
360.657607884634,361.156521963168,361.655436041702,362.653264198771,363.651092355839,
364.648920512907,365.646748669975,366.644576827044,367.143490905578,367.642404984112,
368.141319062646,368.64023314118,369.638061298248,370.635889455317,371.633717612385,
372.631545769453,373.629373926521,374.128288005055,374.62720208359,375.126116162124,
375.625030240658,376.622858397726,377.620686554794,378.618514711863,379.616342868931,
380.614171025999,381.113085104533,381.611999183067,382.110913261602,382.609827340136,
383.607655497204,384.605483654272,385.60331181134,386.601139968409,387.598968125477,
388.097882204011,388.596796282545,389.095710361079,389.594624439613,390.592452596682,
391.59028075375,392.588108910818,393.585937067887,394.583765224955,395.082679303489,
395.581593382023,396.080507460557,396.579421539091,397.57724969616,398.575077853228,
399.572906010296,400.570734167364,401.568562324433,402.067476402967,402.566390481501,
403.065304560035,403.564218638569,404.562046795637,405.559874952706,406.557703109774,
407.056617188308,407.555531266842,408.054445345376,408.55335942391),
 .UNSPECIFIED.);
#836=B_SPLINE_SURFACE_WITH_KNOTS('',3,3,((#40363,#40364,#40365,#40366,#40367,
#40368,#40369,#40370,#40371,#40372,#40373,#40374,#40375,#40376,#40377,#40378,
#40379,#40380,#40381,#40382,#40383,#40384,#40385,#40386,#40387,#40388,#40389,
#40390,#40391,#40392,#40393,#40394,#40395,#40396,#40397,#40398,#40399,#40400,
#40401,#40402,#40403,#40404,#40405,#40406,#40407,#40408,#40409,#40410,#40411,
#40412,#40413,#40414,#40415,#40416,#40417,#40418,#40419,#40420,#40421,#40422,
#40423,#40424,#40425,#40426,#40427,#40428,#40429,#40430,#40431,#40432,#40433,
#40434,#40435,#40436,#40437,#40438,#40439,#40440,#40441,#40442,#40443,#40444,
#40445,#40446,#40447,#40448,#40449,#40450,#40451,#40452,#40453,#40454,#40455,
#40456,#40457,#40458,#40459,#40460,#40461,#40462,#40463,#40464,#40465,#40466,
#40467,#40468,#40469,#40470,#40471,#40472,#40473,#40474,#40475,#40476,#40477,
#40478,#40479,#40480,#40481,#40482,#40483,#40484,#40485,#40486,#40487,#40488,
#40489,#40490,#40491,#40492,#40493,#40494,#40495,#40496,#40497,#40498,#40499,
#40500,#40501,#40502,#40503,#40504,#40505,#40506,#40507,#40508,#40509,#40510,
#40511,#40512,#40513,#40514,#40515,#40516,#40517,#40518,#40519,#40520,#40521,
#40522,#40523,#40524,#40525,#40526,#40527,#40528,#40529,#40530,#40531,#40532,
#40533,#40534,#40535,#40536,#40537,#40538,#40539,#40540,#40541,#40542,#40543,
#40544,#40545,#40546,#40547,#40548,#40549,#40550,#40551,#40552,#40553,#40554,
#40555,#40556,#40557,#40558,#40559,#40560,#40561,#40562,#40563,#40564,#40565,
#40566,#40567,#40568,#40569,#40570,#40571),(#40572,#40573,#40574,#40575,
#40576,#40577,#40578,#40579,#40580,#40581,#40582,#40583,#40584,#40585,#40586,
#40587,#40588,#40589,#40590,#40591,#40592,#40593,#40594,#40595,#40596,#40597,
#40598,#40599,#40600,#40601,#40602,#40603,#40604,#40605,#40606,#40607,#40608,
#40609,#40610,#40611,#40612,#40613,#40614,#40615,#40616,#40617,#40618,#40619,
#40620,#40621,#40622,#40623,#40624,#40625,#40626,#40627,#40628,#40629,#40630,
#40631,#40632,#40633,#40634,#40635,#40636,#40637,#40638,#40639,#40640,#40641,
#40642,#40643,#40644,#40645,#40646,#40647,#40648,#40649,#40650,#40651,#40652,
#40653,#40654,#40655,#40656,#40657,#40658,#40659,#40660,#40661,#40662,#40663,
#40664,#40665,#40666,#40667,#40668,#40669,#40670,#40671,#40672,#40673,#40674,
#40675,#40676,#40677,#40678,#40679,#40680,#40681,#40682,#40683,#40684,#40685,
#40686,#40687,#40688,#40689,#40690,#40691,#40692,#40693,#40694,#40695,#40696,
#40697,#40698,#40699,#40700,#40701,#40702,#40703,#40704,#40705,#40706,#40707,
#40708,#40709,#40710,#40711,#40712,#40713,#40714,#40715,#40716,#40717,#40718,
#40719,#40720,#40721,#40722,#40723,#40724,#40725,#40726,#40727,#40728,#40729,
#40730,#40731,#40732,#40733,#40734,#40735,#40736,#40737,#40738,#40739,#40740,
#40741,#40742,#40743,#40744,#40745,#40746,#40747,#40748,#40749,#40750,#40751,
#40752,#40753,#40754,#40755,#40756,#40757,#40758,#40759,#40760,#40761,#40762,
#40763,#40764,#40765,#40766,#40767,#40768,#40769,#40770,#40771,#40772,#40773,
#40774,#40775,#40776,#40777,#40778,#40779,#40780),(#40781,#40782,#40783,
#40784,#40785,#40786,#40787,#40788,#40789,#40790,#40791,#40792,#40793,#40794,
#40795,#40796,#40797,#40798,#40799,#40800,#40801,#40802,#40803,#40804,#40805,
#40806,#40807,#40808,#40809,#40810,#40811,#40812,#40813,#40814,#40815,#40816,
#40817,#40818,#40819,#40820,#40821,#40822,#40823,#40824,#40825,#40826,#40827,
#40828,#40829,#40830,#40831,#40832,#40833,#40834,#40835,#40836,#40837,#40838,
#40839,#40840,#40841,#40842,#40843,#40844,#40845,#40846,#40847,#40848,#40849,
#40850,#40851,#40852,#40853,#40854,#40855,#40856,#40857,#40858,#40859,#40860,
#40861,#40862,#40863,#40864,#40865,#40866,#40867,#40868,#40869,#40870,#40871,
#40872,#40873,#40874,#40875,#40876,#40877,#40878,#40879,#40880,#40881,#40882,
#40883,#40884,#40885,#40886,#40887,#40888,#40889,#40890,#40891,#40892,#40893,
#40894,#40895,#40896,#40897,#40898,#40899,#40900,#40901,#40902,#40903,#40904,
#40905,#40906,#40907,#40908,#40909,#40910,#40911,#40912,#40913,#40914,#40915,
#40916,#40917,#40918,#40919,#40920,#40921,#40922,#40923,#40924,#40925,#40926,
#40927,#40928,#40929,#40930,#40931,#40932,#40933,#40934,#40935,#40936,#40937,
#40938,#40939,#40940,#40941,#40942,#40943,#40944,#40945,#40946,#40947,#40948,
#40949,#40950,#40951,#40952,#40953,#40954,#40955,#40956,#40957,#40958,#40959,
#40960,#40961,#40962,#40963,#40964,#40965,#40966,#40967,#40968,#40969,#40970,
#40971,#40972,#40973,#40974,#40975,#40976,#40977,#40978,#40979,#40980,#40981,
#40982,#40983,#40984,#40985,#40986,#40987,#40988,#40989),(#40990,#40991,
#40992,#40993,#40994,#40995,#40996,#40997,#40998,#40999,#41000,#41001,#41002,
#41003,#41004,#41005,#41006,#41007,#41008,#41009,#41010,#41011,#41012,#41013,
#41014,#41015,#41016,#41017,#41018,#41019,#41020,#41021,#41022,#41023,#41024,
#41025,#41026,#41027,#41028,#41029,#41030,#41031,#41032,#41033,#41034,#41035,
#41036,#41037,#41038,#41039,#41040,#41041,#41042,#41043,#41044,#41045,#41046,
#41047,#41048,#41049,#41050,#41051,#41052,#41053,#41054,#41055,#41056,#41057,
#41058,#41059,#41060,#41061,#41062,#41063,#41064,#41065,#41066,#41067,#41068,
#41069,#41070,#41071,#41072,#41073,#41074,#41075,#41076,#41077,#41078,#41079,
#41080,#41081,#41082,#41083,#41084,#41085,#41086,#41087,#41088,#41089,#41090,
#41091,#41092,#41093,#41094,#41095,#41096,#41097,#41098,#41099,#41100,#41101,
#41102,#41103,#41104,#41105,#41106,#41107,#41108,#41109,#41110,#41111,#41112,
#41113,#41114,#41115,#41116,#41117,#41118,#41119,#41120,#41121,#41122,#41123,
#41124,#41125,#41126,#41127,#41128,#41129,#41130,#41131,#41132,#41133,#41134,
#41135,#41136,#41137,#41138,#41139,#41140,#41141,#41142,#41143,#41144,#41145,
#41146,#41147,#41148,#41149,#41150,#41151,#41152,#41153,#41154,#41155,#41156,
#41157,#41158,#41159,#41160,#41161,#41162,#41163,#41164,#41165,#41166,#41167,
#41168,#41169,#41170,#41171,#41172,#41173,#41174,#41175,#41176,#41177,#41178,
#41179,#41180,#41181,#41182,#41183,#41184,#41185,#41186,#41187,#41188,#41189,
#41190,#41191,#41192,#41193,#41194,#41195,#41196,#41197,#41198)),
 .UNSPECIFIED.,.F.,.F.,.F.,(4,4),(4,1,1,1,1,1,1,1,1,1,1,1,1,1,1,1,1,1,1,
1,1,1,1,1,1,1,1,1,1,1,1,1,1,1,1,1,1,1,1,1,1,1,1,1,1,1,1,1,1,1,1,1,1,1,1,
1,1,1,1,1,1,1,1,1,1,1,1,1,1,1,1,1,1,1,1,1,1,1,1,1,1,1,1,1,1,1,1,1,1,1,1,
1,1,1,1,1,1,1,1,1,1,1,1,1,1,1,1,1,1,1,1,1,1,1,1,1,1,1,1,1,1,1,1,1,1,1,1,
1,1,1,1,1,1,1,1,1,1,1,1,1,1,1,1,1,1,1,1,1,1,1,1,1,1,1,1,1,1,1,1,1,1,1,1,
1,1,1,1,1,1,1,1,1,1,1,1,1,1,1,1,1,1,1,1,1,1,1,1,1,1,1,1,1,1,1,1,1,1,1,1,
1,1,1,1,1,1,1,4),(0.,0.0824167509268187),(8.58761471263784,9.08568424559332,
9.58375377854879,10.0818233115043,10.5798928444598,11.0779623774152,11.5760319103707,
12.0741014433262,12.5721709762817,13.0702405092372,13.5683100421926,14.0663795751481,
14.5644491081036,15.0625186410591,15.5605881740146,16.05865770697,16.5567272399255,
17.054796772881,17.5528663058365,18.0509358387919,18.5490053717474,19.0470749047029,
19.5451444376584,20.0432139706139,20.5412835035693,21.0393530365248,21.5374225694803,
22.0354921024358,22.5335616353913,23.0316311683467,23.5297007013022,24.0277702342577,
24.5258397672132,25.0239093001687,25.5219788331241,26.0200483660796,26.5181178990351,
27.0161874319906,27.5142569649461,28.0123264979015,28.510396030857,29.0084655638125,
29.506535096768,30.0046046297235,30.5026741626789,31.0007436956344,31.4988132285899,
31.9968827615454,32.4949522945009,32.9930218274563,33.4910913604118,33.9891608933673,
34.4872304263228,34.9852999592783,35.4833694922337,35.9814390251892,36.4795085581447,
36.9775780911002,37.4756476240557,37.9737171570111,38.4717866899666,38.9698562229221,
39.4679257558776,39.9659952888331,40.4640648217885,40.962134354744,41.4602038876995,
41.958273420655,42.4563429536105,42.9544124865659,43.4524820195214,43.9505515524769,
44.4486210854324,44.9466906183878,45.4447601513433,45.9428296842988,46.4408992172543,
46.9389687502098,47.4370382831653,47.9351078161207,48.4331773490762,48.9312468820317,
49.4293164149872,49.9273859479427,50.4254554808981,50.9235250138536,51.4215945468091,
51.9196640797646,52.41773361272,52.9158031456755,53.413872678631,53.9119422115865,
54.410011744542,54.9080812774974,55.4061508104529,55.9042203434084,56.4022898763639,
56.9003594093194,57.3984289422748,57.8964984752303,58.3945680081858,58.8926375411413,
59.3907070740968,59.8887766070523,60.3868461400077,60.8849156729632,61.3829852059187,
61.8810547388742,62.3791242718296,62.8771938047851,63.3752633377406,63.8733328706961,
64.3714024036516,64.869471936607,65.3675414695625,65.865611002518,66.3636805354735,
66.861750068429,67.3598196013844,67.8578891343399,68.3559586672954,68.8540282002509,
69.3520977332063,69.8501672661618,70.3482367991173,70.8463063320728,71.3443758650283,
71.8424453979838,72.3405149309392,72.8385844638947,73.3366539968502,73.8347235298057,
74.3327930627611,74.8308625957166,75.3289321286721,75.8270016616276,76.3250711945831,
76.8231407275385,77.321210260494,77.8192797934495,78.317349326405,78.8154188593605,
79.3134883923159,79.8115579252714,80.3096274582269,80.8076969911824,81.3057665241379,
81.8038360570933,82.3019055900488,82.7999751230043,83.2980446559598,83.7961141889153,
84.2941837218707,84.7922532548262,85.2903227877817,85.7883923207372,86.2864618536927,
86.7845313866481,87.2826009196036,87.7806704525591,88.2787399855146,88.7768095184701,
89.2748790514255,89.772948584381,90.2710181173365,90.769087650292,91.2671571832475,
91.7652267162029,92.2632962491584,92.7613657821139,93.2594353150694,93.7575048480249,
94.2555743809803,94.7536439139358,95.2517134468913,95.7497829798468,96.2478525128023,
96.7459220457577,97.2439915787132,97.7420611116687,98.2401306446242,98.7382001775796,
99.2362697105351,99.7343392434906,100.232408776446,100.730478309402,101.228547842357,
101.726617375313,102.224686908268,102.722756441223,103.220825974179,103.718895507134,
104.21696504009,104.715034573045,105.213104106001,105.711173638956,106.209243171912,
106.707312704867,107.205382237823,107.703451770778,108.201521303734,108.699590836689,
109.197660369645,109.6957299026,110.193799435556,110.691868968511,111.189938501467),
 .UNSPECIFIED.);
#837=B_SPLINE_SURFACE_WITH_KNOTS('',3,3,((#41493,#41494,#41495,#41496,#41497,
#41498,#41499,#41500,#41501,#41502,#41503,#41504,#41505,#41506,#41507,#41508,
#41509,#41510,#41511,#41512,#41513,#41514,#41515,#41516,#41517,#41518,#41519,
#41520,#41521,#41522,#41523,#41524,#41525,#41526,#41527,#41528,#41529,#41530,
#41531,#41532,#41533,#41534,#41535,#41536,#41537,#41538,#41539,#41540,#41541,
#41542,#41543,#41544,#41545,#41546,#41547,#41548,#41549,#41550,#41551,#41552,
#41553,#41554,#41555,#41556,#41557,#41558,#41559,#41560,#41561,#41562,#41563,
#41564,#41565,#41566,#41567,#41568,#41569,#41570,#41571,#41572,#41573,#41574,
#41575,#41576,#41577,#41578,#41579,#41580,#41581,#41582,#41583,#41584,#41585,
#41586,#41587,#41588,#41589,#41590,#41591,#41592,#41593,#41594,#41595,#41596,
#41597,#41598,#41599,#41600,#41601,#41602,#41603,#41604,#41605,#41606,#41607,
#41608,#41609,#41610,#41611,#41612,#41613,#41614,#41615,#41616,#41617,#41618,
#41619,#41620,#41621,#41622,#41623,#41624,#41625,#41626,#41627,#41628,#41629,
#41630,#41631,#41632,#41633,#41634,#41635,#41636,#41637,#41638,#41639,#41640,
#41641,#41642,#41643,#41644,#41645,#41646,#41647,#41648,#41649,#41650,#41651,
#41652,#41653,#41654,#41655,#41656,#41657,#41658,#41659,#41660,#41661,#41662,
#41663,#41664,#41665,#41666,#41667,#41668,#41669,#41670,#41671,#41672,#41673,
#41674,#41675,#41676,#41677,#41678,#41679,#41680,#41681,#41682,#41683,#41684,
#41685,#41686,#41687,#41688,#41689,#41690,#41691,#41692,#41693,#41694,#41695,
#41696,#41697,#41698,#41699,#41700,#41701),(#41702,#41703,#41704,#41705,
#41706,#41707,#41708,#41709,#41710,#41711,#41712,#41713,#41714,#41715,#41716,
#41717,#41718,#41719,#41720,#41721,#41722,#41723,#41724,#41725,#41726,#41727,
#41728,#41729,#41730,#41731,#41732,#41733,#41734,#41735,#41736,#41737,#41738,
#41739,#41740,#41741,#41742,#41743,#41744,#41745,#41746,#41747,#41748,#41749,
#41750,#41751,#41752,#41753,#41754,#41755,#41756,#41757,#41758,#41759,#41760,
#41761,#41762,#41763,#41764,#41765,#41766,#41767,#41768,#41769,#41770,#41771,
#41772,#41773,#41774,#41775,#41776,#41777,#41778,#41779,#41780,#41781,#41782,
#41783,#41784,#41785,#41786,#41787,#41788,#41789,#41790,#41791,#41792,#41793,
#41794,#41795,#41796,#41797,#41798,#41799,#41800,#41801,#41802,#41803,#41804,
#41805,#41806,#41807,#41808,#41809,#41810,#41811,#41812,#41813,#41814,#41815,
#41816,#41817,#41818,#41819,#41820,#41821,#41822,#41823,#41824,#41825,#41826,
#41827,#41828,#41829,#41830,#41831,#41832,#41833,#41834,#41835,#41836,#41837,
#41838,#41839,#41840,#41841,#41842,#41843,#41844,#41845,#41846,#41847,#41848,
#41849,#41850,#41851,#41852,#41853,#41854,#41855,#41856,#41857,#41858,#41859,
#41860,#41861,#41862,#41863,#41864,#41865,#41866,#41867,#41868,#41869,#41870,
#41871,#41872,#41873,#41874,#41875,#41876,#41877,#41878,#41879,#41880,#41881,
#41882,#41883,#41884,#41885,#41886,#41887,#41888,#41889,#41890,#41891,#41892,
#41893,#41894,#41895,#41896,#41897,#41898,#41899,#41900,#41901,#41902,#41903,
#41904,#41905,#41906,#41907,#41908,#41909,#41910),(#41911,#41912,#41913,
#41914,#41915,#41916,#41917,#41918,#41919,#41920,#41921,#41922,#41923,#41924,
#41925,#41926,#41927,#41928,#41929,#41930,#41931,#41932,#41933,#41934,#41935,
#41936,#41937,#41938,#41939,#41940,#41941,#41942,#41943,#41944,#41945,#41946,
#41947,#41948,#41949,#41950,#41951,#41952,#41953,#41954,#41955,#41956,#41957,
#41958,#41959,#41960,#41961,#41962,#41963,#41964,#41965,#41966,#41967,#41968,
#41969,#41970,#41971,#41972,#41973,#41974,#41975,#41976,#41977,#41978,#41979,
#41980,#41981,#41982,#41983,#41984,#41985,#41986,#41987,#41988,#41989,#41990,
#41991,#41992,#41993,#41994,#41995,#41996,#41997,#41998,#41999,#42000,#42001,
#42002,#42003,#42004,#42005,#42006,#42007,#42008,#42009,#42010,#42011,#42012,
#42013,#42014,#42015,#42016,#42017,#42018,#42019,#42020,#42021,#42022,#42023,
#42024,#42025,#42026,#42027,#42028,#42029,#42030,#42031,#42032,#42033,#42034,
#42035,#42036,#42037,#42038,#42039,#42040,#42041,#42042,#42043,#42044,#42045,
#42046,#42047,#42048,#42049,#42050,#42051,#42052,#42053,#42054,#42055,#42056,
#42057,#42058,#42059,#42060,#42061,#42062,#42063,#42064,#42065,#42066,#42067,
#42068,#42069,#42070,#42071,#42072,#42073,#42074,#42075,#42076,#42077,#42078,
#42079,#42080,#42081,#42082,#42083,#42084,#42085,#42086,#42087,#42088,#42089,
#42090,#42091,#42092,#42093,#42094,#42095,#42096,#42097,#42098,#42099,#42100,
#42101,#42102,#42103,#42104,#42105,#42106,#42107,#42108,#42109,#42110,#42111,
#42112,#42113,#42114,#42115,#42116,#42117,#42118,#42119),(#42120,#42121,
#42122,#42123,#42124,#42125,#42126,#42127,#42128,#42129,#42130,#42131,#42132,
#42133,#42134,#42135,#42136,#42137,#42138,#42139,#42140,#42141,#42142,#42143,
#42144,#42145,#42146,#42147,#42148,#42149,#42150,#42151,#42152,#42153,#42154,
#42155,#42156,#42157,#42158,#42159,#42160,#42161,#42162,#42163,#42164,#42165,
#42166,#42167,#42168,#42169,#42170,#42171,#42172,#42173,#42174,#42175,#42176,
#42177,#42178,#42179,#42180,#42181,#42182,#42183,#42184,#42185,#42186,#42187,
#42188,#42189,#42190,#42191,#42192,#42193,#42194,#42195,#42196,#42197,#42198,
#42199,#42200,#42201,#42202,#42203,#42204,#42205,#42206,#42207,#42208,#42209,
#42210,#42211,#42212,#42213,#42214,#42215,#42216,#42217,#42218,#42219,#42220,
#42221,#42222,#42223,#42224,#42225,#42226,#42227,#42228,#42229,#42230,#42231,
#42232,#42233,#42234,#42235,#42236,#42237,#42238,#42239,#42240,#42241,#42242,
#42243,#42244,#42245,#42246,#42247,#42248,#42249,#42250,#42251,#42252,#42253,
#42254,#42255,#42256,#42257,#42258,#42259,#42260,#42261,#42262,#42263,#42264,
#42265,#42266,#42267,#42268,#42269,#42270,#42271,#42272,#42273,#42274,#42275,
#42276,#42277,#42278,#42279,#42280,#42281,#42282,#42283,#42284,#42285,#42286,
#42287,#42288,#42289,#42290,#42291,#42292,#42293,#42294,#42295,#42296,#42297,
#42298,#42299,#42300,#42301,#42302,#42303,#42304,#42305,#42306,#42307,#42308,
#42309,#42310,#42311,#42312,#42313,#42314,#42315,#42316,#42317,#42318,#42319,
#42320,#42321,#42322,#42323,#42324,#42325,#42326,#42327,#42328)),
 .UNSPECIFIED.,.F.,.F.,.F.,(4,4),(4,1,1,1,1,1,1,1,1,1,1,1,1,1,1,1,1,1,1,
1,1,1,1,1,1,1,1,1,1,1,1,1,1,1,1,1,1,1,1,1,1,1,1,1,1,1,1,1,1,1,1,1,1,1,1,
1,1,1,1,1,1,1,1,1,1,1,1,1,1,1,1,1,1,1,1,1,1,1,1,1,1,1,1,1,1,1,1,1,1,1,1,
1,1,1,1,1,1,1,1,1,1,1,1,1,1,1,1,1,1,1,1,1,1,1,1,1,1,1,1,1,1,1,1,1,1,1,1,
1,1,1,1,1,1,1,1,1,1,1,1,1,1,1,1,1,1,1,1,1,1,1,1,1,1,1,1,1,1,1,1,1,1,1,1,
1,1,1,1,1,1,1,1,1,1,1,1,1,1,1,1,1,1,1,1,1,1,1,1,1,1,1,1,1,1,1,1,1,1,1,1,
1,1,1,1,1,1,1,4),(0.,0.0824167509268187),(11.897963259076,12.3960327920314,
12.8941023249869,13.3921718579424,13.8902413908979,14.3883109238534,14.8863804568088,
15.3844499897643,15.8825195227198,16.3805890556753,16.8786585886308,17.3767281215862,
17.8747976545417,18.3728671874972,18.8709367204527,19.3690062534082,19.8670757863636,
20.3651453193191,20.8632148522746,21.3612843852301,21.8593539181856,22.357423451141,
22.8554929840965,23.353562517052,23.8516320500075,24.349701582963,24.8477711159184,
25.3458406488739,25.8439101818294,26.3419797147849,26.8400492477403,27.3381187806958,
27.8361883136513,28.3342578466068,28.8323273795623,29.3303969125177,29.8284664454732,
30.3265359784287,30.8246055113842,31.3226750443397,31.8207445772951,32.3188141102506,
32.8168836432061,33.3149531761616,33.8130227091171,34.3110922420725,34.809161775028,
35.3072313079835,35.805300840939,36.3033703738945,36.8014399068499,37.2995094398054,
37.7975789727609,38.2956485057164,38.7937180386719,39.2917875716273,39.7898571045828,
40.2879266375383,40.7859961704938,41.2840657034493,41.7821352364047,42.2802047693602,
42.7782743023157,43.2763438352712,43.7744133682266,44.2724829011821,44.7705524341376,
45.2686219670931,45.7666915000486,46.264761033004,46.7628305659595,47.260900098915,
47.7589696318705,48.257039164826,48.7551086977815,49.2531782307369,49.7512477636924,
50.2493172966479,50.7473868296034,51.2454563625588,51.7435258955143,52.2415954284698,
52.7396649614253,53.2377344943808,53.7358040273362,54.2338735602917,54.7319430932472,
55.2300126262027,55.7280821591582,56.2261516921136,56.7242212250691,57.2222907580246,
57.7203602909801,58.2184298239356,58.716499356891,59.2145688898465,59.712638422802,
60.2107079557575,60.708777488713,61.2068470216684,61.7049165546239,62.2029860875794,
62.7010556205349,63.1991251534903,63.6971946864458,64.1952642194013,64.6933337523568,
65.1914032853123,65.6894728182677,66.1875423512232,66.6856118841787,67.1836814171342,
67.6817509500897,68.1798204830451,68.6778900160006,69.1759595489561,69.6740290819116,
70.1720986148671,70.6701681478225,71.168237680778,71.6663072137335,72.164376746689,
72.6624462796445,73.1605158125999,73.6585853455554,74.1566548785109,74.6547244114664,
75.1527939444219,75.6508634773773,76.1489330103328,76.6470025432883,77.1450720762438,
77.6431416091993,78.1412111421547,78.6392806751102,79.1373502080657,79.6354197410212,
80.1334892739767,80.6315588069321,81.1296283398876,81.6276978728431,82.1257674057986,
82.6238369387541,83.1219064717095,83.619976004665,84.1180455376205,84.616115070576,
85.1141846035315,85.6122541364869,86.1103236694424,86.6083932023979,87.1064627353534,
87.6045322683088,88.1026018012643,88.6006713342198,89.0987408671753,89.5968104001308,
90.0948799330862,90.5929494660417,91.0910189989972,91.5890885319527,92.0871580649082,
92.5852275978636,93.0832971308191,93.5813666637746,94.0794361967301,94.5775057296856,
95.0755752626411,95.5736447955965,96.071714328552,96.5697838615075,97.067853394463,
97.5659229274184,98.0639924603739,98.5620619933294,99.0601315262849,99.5582010592404,
100.056270592196,100.554340125151,101.052409658107,101.550479191062,102.048548724018,
102.546618256973,103.044687789929,103.542757322884,104.04082685584,104.538896388795,
105.036965921751,105.535035454706,106.033104987662,106.531174520617,107.029244053573,
107.527313586528,108.025383119484,108.523452652439,109.021522185394,109.51959171835,
110.017661251305,110.515730784261,111.013800317216,111.511869850172,112.009939383127,
112.508008916083,113.006078449038,113.504147981994,114.002217514949,114.500287047905),
 .UNSPECIFIED.);
#853=PLANE('',#20315);
#854=PLANE('',#20316);
#855=PLANE('',#20317);
#856=PLANE('',#20318);
#857=PLANE('',#20319);
#858=PLANE('',#20322);
#859=PLANE('',#20325);
#860=PLANE('',#20328);
#861=PLANE('',#20333);
#862=PLANE('',#20338);
#863=PLANE('',#20350);
#864=PLANE('',#20355);
#865=PLANE('',#20364);
#866=PLANE('',#20369);
#867=PLANE('',#20378);
#868=PLANE('',#20383);
#869=PLANE('',#20392);
#870=PLANE('',#20397);
#871=PLANE('',#20406);
#872=PLANE('',#20411);
#873=PLANE('',#20420);
#874=PLANE('',#20425);
#875=PLANE('',#20434);
#876=PLANE('',#20440);
#877=PLANE('',#20450);
#878=PLANE('',#20455);
#879=PLANE('',#20464);
#880=PLANE('',#20469);
#881=PLANE('',#20478);
#882=PLANE('',#20483);
#883=PLANE('',#20492);
#884=PLANE('',#20497);
#885=PLANE('',#20506);
#886=PLANE('',#20511);
#887=PLANE('',#20520);
#888=PLANE('',#20525);
#889=PLANE('',#20534);
#890=PLANE('',#20539);
#891=PLANE('',#20545);
#892=PLANE('',#20554);
#1082=FACE_BOUND('',#2313,.T.);
#1126=FACE_OUTER_BOUND('',#2312,.T.);
#1127=FACE_OUTER_BOUND('',#2314,.T.);
#1128=FACE_OUTER_BOUND('',#2315,.T.);
#1129=FACE_OUTER_BOUND('',#2316,.T.);
#1130=FACE_OUTER_BOUND('',#2317,.T.);
#1131=FACE_OUTER_BOUND('',#2318,.T.);
#1132=FACE_OUTER_BOUND('',#2319,.T.);
#1133=FACE_OUTER_BOUND('',#2320,.T.);
#1134=FACE_OUTER_BOUND('',#2321,.T.);
#1135=FACE_OUTER_BOUND('',#2322,.T.);
#1136=FACE_OUTER_BOUND('',#2323,.T.);
#1137=FACE_OUTER_BOUND('',#2324,.T.);
#1138=FACE_OUTER_BOUND('',#2325,.T.);
#1139=FACE_OUTER_BOUND('',#2326,.T.);
#1140=FACE_OUTER_BOUND('',#2327,.T.);
#1141=FACE_OUTER_BOUND('',#2328,.T.);
#1142=FACE_OUTER_BOUND('',#2329,.T.);
#1143=FACE_OUTER_BOUND('',#2330,.T.);
#1144=FACE_OUTER_BOUND('',#2331,.T.);
#1145=FACE_OUTER_BOUND('',#2332,.T.);
#1146=FACE_OUTER_BOUND('',#2333,.T.);
#1147=FACE_OUTER_BOUND('',#2334,.T.);
#1148=FACE_OUTER_BOUND('',#2335,.T.);
#1149=FACE_OUTER_BOUND('',#2336,.T.);
#1150=FACE_OUTER_BOUND('',#2337,.T.);
#1151=FACE_OUTER_BOUND('',#2338,.T.);
#1152=FACE_OUTER_BOUND('',#2339,.T.);
#1153=FACE_OUTER_BOUND('',#2340,.T.);
#1154=FACE_OUTER_BOUND('',#2341,.T.);
#1155=FACE_OUTER_BOUND('',#2342,.T.);
#1156=FACE_OUTER_BOUND('',#2343,.T.);
#1157=FACE_OUTER_BOUND('',#2344,.T.);
#1158=FACE_OUTER_BOUND('',#2345,.T.);
#1159=FACE_OUTER_BOUND('',#2346,.T.);
#1160=FACE_OUTER_BOUND('',#2347,.T.);
#1161=FACE_OUTER_BOUND('',#2348,.T.);
#1162=FACE_OUTER_BOUND('',#2349,.T.);
#1163=FACE_OUTER_BOUND('',#2350,.T.);
#1164=FACE_OUTER_BOUND('',#2351,.T.);
#1165=FACE_OUTER_BOUND('',#2352,.T.);
#1166=FACE_OUTER_BOUND('',#2353,.T.);
#1167=FACE_OUTER_BOUND('',#2354,.T.);
#1168=FACE_OUTER_BOUND('',#2355,.T.);
#1169=FACE_OUTER_BOUND('',#2356,.T.);
#1170=FACE_OUTER_BOUND('',#2357,.T.);
#1171=FACE_OUTER_BOUND('',#2358,.T.);
#1172=FACE_OUTER_BOUND('',#2359,.T.);
#1173=FACE_OUTER_BOUND('',#2360,.T.);
#1174=FACE_OUTER_BOUND('',#2361,.T.);
#1175=FACE_OUTER_BOUND('',#2362,.T.);
#1176=FACE_OUTER_BOUND('',#2363,.T.);
#1177=FACE_OUTER_BOUND('',#2364,.T.);
#1178=FACE_OUTER_BOUND('',#2365,.T.);
#1179=FACE_OUTER_BOUND('',#2366,.T.);
#1180=FACE_OUTER_BOUND('',#2367,.T.);
#1181=FACE_OUTER_BOUND('',#2368,.T.);
#1182=FACE_OUTER_BOUND('',#2369,.T.);
#1183=FACE_OUTER_BOUND('',#2370,.T.);
#1184=FACE_OUTER_BOUND('',#2371,.T.);
#1185=FACE_OUTER_BOUND('',#2372,.T.);
#1186=FACE_OUTER_BOUND('',#2373,.T.);
#1187=FACE_OUTER_BOUND('',#2374,.T.);
#1188=FACE_OUTER_BOUND('',#2375,.T.);
#1189=FACE_OUTER_BOUND('',#2376,.T.);
#1190=FACE_OUTER_BOUND('',#2377,.T.);
#1191=FACE_OUTER_BOUND('',#2378,.T.);
#1192=FACE_OUTER_BOUND('',#2379,.T.);
#1193=FACE_OUTER_BOUND('',#2380,.T.);
#1194=FACE_OUTER_BOUND('',#2381,.T.);
#1195=FACE_OUTER_BOUND('',#2382,.T.);
#1196=FACE_OUTER_BOUND('',#2383,.T.);
#1197=FACE_OUTER_BOUND('',#2384,.T.);
#1198=FACE_OUTER_BOUND('',#2385,.T.);
#1199=FACE_OUTER_BOUND('',#2386,.T.);
#1200=FACE_OUTER_BOUND('',#2387,.T.);
#1201=FACE_OUTER_BOUND('',#2388,.T.);
#1202=FACE_OUTER_BOUND('',#2389,.T.);
#1203=FACE_OUTER_BOUND('',#2390,.T.);
#1204=FACE_OUTER_BOUND('',#2391,.T.);
#1205=FACE_OUTER_BOUND('',#2392,.T.);
#1206=FACE_OUTER_BOUND('',#2393,.T.);
#1207=FACE_OUTER_BOUND('',#2394,.T.);
#1208=FACE_OUTER_BOUND('',#2395,.T.);
#1209=FACE_OUTER_BOUND('',#2396,.T.);
#1210=FACE_OUTER_BOUND('',#2397,.T.);
#1211=FACE_OUTER_BOUND('',#2398,.T.);
#1212=FACE_OUTER_BOUND('',#2399,.T.);
#1213=FACE_OUTER_BOUND('',#2400,.T.);
#1214=FACE_OUTER_BOUND('',#2401,.T.);
#1215=FACE_OUTER_BOUND('',#2402,.T.);
#1216=FACE_OUTER_BOUND('',#2403,.T.);
#1217=FACE_OUTER_BOUND('',#2404,.T.);
#1218=FACE_OUTER_BOUND('',#2405,.T.);
#1219=FACE_OUTER_BOUND('',#2406,.T.);
#1220=FACE_OUTER_BOUND('',#2407,.T.);
#1221=FACE_OUTER_BOUND('',#2408,.T.);
#1222=FACE_OUTER_BOUND('',#2409,.T.);
#1223=FACE_OUTER_BOUND('',#2410,.T.);
#1224=FACE_OUTER_BOUND('',#2411,.T.);
#1225=FACE_OUTER_BOUND('',#2412,.T.);
#1226=FACE_OUTER_BOUND('',#2413,.T.);
#1227=FACE_OUTER_BOUND('',#2414,.T.);
#1228=FACE_OUTER_BOUND('',#2415,.T.);
#1229=FACE_OUTER_BOUND('',#2416,.T.);
#1230=FACE_OUTER_BOUND('',#2417,.T.);
#1231=FACE_OUTER_BOUND('',#2418,.T.);
#1232=FACE_OUTER_BOUND('',#2419,.T.);
#1233=FACE_OUTER_BOUND('',#2420,.T.);
#1234=FACE_OUTER_BOUND('',#2421,.T.);
#1235=FACE_OUTER_BOUND('',#2422,.T.);
#1236=FACE_OUTER_BOUND('',#2423,.T.);
#1237=FACE_OUTER_BOUND('',#2424,.T.);
#1238=FACE_OUTER_BOUND('',#2425,.T.);
#1239=FACE_OUTER_BOUND('',#2426,.T.);
#1240=FACE_OUTER_BOUND('',#2427,.T.);
#1241=FACE_OUTER_BOUND('',#2428,.T.);
#1242=FACE_OUTER_BOUND('',#2429,.T.);
#1243=FACE_OUTER_BOUND('',#2430,.T.);
#1244=FACE_OUTER_BOUND('',#2431,.T.);
#1245=FACE_OUTER_BOUND('',#2432,.T.);
#1246=FACE_OUTER_BOUND('',#2433,.T.);
#1247=FACE_OUTER_BOUND('',#2434,.T.);
#1248=FACE_OUTER_BOUND('',#2435,.T.);
#1249=FACE_OUTER_BOUND('',#2436,.T.);
#1250=FACE_OUTER_BOUND('',#2437,.T.);
#1251=FACE_OUTER_BOUND('',#2438,.T.);
#1252=FACE_OUTER_BOUND('',#2439,.T.);
#1253=FACE_OUTER_BOUND('',#2440,.T.);
#1254=FACE_OUTER_BOUND('',#2441,.T.);
#1255=FACE_OUTER_BOUND('',#2442,.T.);
#1256=FACE_OUTER_BOUND('',#2443,.T.);
#1257=FACE_OUTER_BOUND('',#2444,.T.);
#1258=FACE_OUTER_BOUND('',#2445,.T.);
#1259=FACE_OUTER_BOUND('',#2446,.T.);
#1260=FACE_OUTER_BOUND('',#2447,.T.);
#1261=FACE_OUTER_BOUND('',#2448,.T.);
#1262=FACE_OUTER_BOUND('',#2449,.T.);
#1263=FACE_OUTER_BOUND('',#2450,.T.);
#1264=FACE_OUTER_BOUND('',#2451,.T.);
#1265=FACE_OUTER_BOUND('',#2452,.T.);
#1266=FACE_OUTER_BOUND('',#2453,.T.);
#1267=FACE_OUTER_BOUND('',#2454,.T.);
#1268=FACE_OUTER_BOUND('',#2455,.T.);
#1269=FACE_OUTER_BOUND('',#2456,.T.);
#1270=FACE_OUTER_BOUND('',#2457,.T.);
#1271=FACE_OUTER_BOUND('',#2458,.T.);
#1272=FACE_OUTER_BOUND('',#2459,.T.);
#1273=FACE_OUTER_BOUND('',#2460,.T.);
#1274=FACE_OUTER_BOUND('',#2461,.T.);
#1275=FACE_OUTER_BOUND('',#2462,.T.);
#1276=FACE_OUTER_BOUND('',#2463,.T.);
#1277=FACE_OUTER_BOUND('',#2464,.T.);
#1278=FACE_OUTER_BOUND('',#2465,.T.);
#1279=FACE_OUTER_BOUND('',#2466,.T.);
#1280=FACE_OUTER_BOUND('',#2467,.T.);
#1281=FACE_OUTER_BOUND('',#2468,.T.);
#1282=FACE_OUTER_BOUND('',#2469,.T.);
#1283=FACE_OUTER_BOUND('',#2470,.T.);
#1284=FACE_OUTER_BOUND('',#2471,.T.);
#1285=FACE_OUTER_BOUND('',#2472,.T.);
#1286=FACE_OUTER_BOUND('',#2473,.T.);
#1287=FACE_OUTER_BOUND('',#2474,.T.);
#1288=FACE_OUTER_BOUND('',#2475,.T.);
#1289=FACE_OUTER_BOUND('',#2476,.T.);
#1290=FACE_OUTER_BOUND('',#2477,.T.);
#1291=FACE_OUTER_BOUND('',#2478,.T.);
#1292=FACE_OUTER_BOUND('',#2479,.T.);
#1293=FACE_OUTER_BOUND('',#2480,.T.);
#1294=FACE_OUTER_BOUND('',#2481,.T.);
#1295=FACE_OUTER_BOUND('',#2482,.T.);
#1296=FACE_OUTER_BOUND('',#2483,.T.);
#1297=FACE_OUTER_BOUND('',#2484,.T.);
#1298=FACE_OUTER_BOUND('',#2485,.T.);
#1299=FACE_OUTER_BOUND('',#2486,.T.);
#1300=FACE_OUTER_BOUND('',#2487,.T.);
#1301=FACE_OUTER_BOUND('',#2488,.T.);
#1302=FACE_OUTER_BOUND('',#2489,.T.);
#1303=FACE_OUTER_BOUND('',#2490,.T.);
#1304=FACE_OUTER_BOUND('',#2491,.T.);
#1305=FACE_OUTER_BOUND('',#2492,.T.);
#1306=FACE_OUTER_BOUND('',#2493,.T.);
#1307=FACE_OUTER_BOUND('',#2494,.T.);
#1308=FACE_OUTER_BOUND('',#2495,.T.);
#1309=FACE_OUTER_BOUND('',#2496,.T.);
#1310=FACE_OUTER_BOUND('',#2497,.T.);
#1311=FACE_OUTER_BOUND('',#2498,.T.);
#1312=FACE_OUTER_BOUND('',#2499,.T.);
#1313=FACE_OUTER_BOUND('',#2500,.T.);
#1314=FACE_OUTER_BOUND('',#2501,.T.);
#1315=FACE_OUTER_BOUND('',#2502,.T.);
#1316=FACE_OUTER_BOUND('',#2503,.T.);
#1317=FACE_OUTER_BOUND('',#2504,.T.);
#1318=FACE_OUTER_BOUND('',#2505,.T.);
#1319=FACE_OUTER_BOUND('',#2506,.T.);
#1320=FACE_OUTER_BOUND('',#2507,.T.);
#1321=FACE_OUTER_BOUND('',#2508,.T.);
#1322=FACE_OUTER_BOUND('',#2509,.T.);
#1323=FACE_OUTER_BOUND('',#2510,.T.);
#1324=FACE_OUTER_BOUND('',#2511,.T.);
#1325=FACE_OUTER_BOUND('',#2512,.T.);
#1326=FACE_OUTER_BOUND('',#2513,.T.);
#1327=FACE_OUTER_BOUND('',#2514,.T.);
#1328=FACE_OUTER_BOUND('',#2515,.T.);
#1329=FACE_OUTER_BOUND('',#2516,.T.);
#1330=FACE_OUTER_BOUND('',#2517,.T.);
#1331=FACE_OUTER_BOUND('',#2518,.T.);
#1332=FACE_OUTER_BOUND('',#2519,.T.);
#1333=FACE_OUTER_BOUND('',#2520,.T.);
#1334=FACE_OUTER_BOUND('',#2521,.T.);
#1335=FACE_OUTER_BOUND('',#2522,.T.);
#1336=FACE_OUTER_BOUND('',#2523,.T.);
#1337=FACE_OUTER_BOUND('',#2524,.T.);
#1338=FACE_OUTER_BOUND('',#2525,.T.);
#1339=FACE_OUTER_BOUND('',#2526,.T.);
#1340=FACE_OUTER_BOUND('',#2527,.T.);
#1341=FACE_OUTER_BOUND('',#2528,.T.);
#1342=FACE_OUTER_BOUND('',#2529,.T.);
#1343=FACE_OUTER_BOUND('',#2530,.T.);
#1344=FACE_OUTER_BOUND('',#2531,.T.);
#1345=FACE_OUTER_BOUND('',#2532,.T.);
#1346=FACE_OUTER_BOUND('',#2533,.T.);
#1347=FACE_OUTER_BOUND('',#2534,.T.);
#1348=FACE_OUTER_BOUND('',#2535,.T.);
#1349=FACE_OUTER_BOUND('',#2536,.T.);
#1350=FACE_OUTER_BOUND('',#2537,.T.);
#1351=FACE_OUTER_BOUND('',#2538,.T.);
#1352=FACE_OUTER_BOUND('',#2539,.T.);
#1353=FACE_OUTER_BOUND('',#2540,.T.);
#1354=FACE_OUTER_BOUND('',#2541,.T.);
#1355=FACE_OUTER_BOUND('',#2542,.T.);
#1356=FACE_OUTER_BOUND('',#2543,.T.);
#1357=FACE_OUTER_BOUND('',#2544,.T.);
#1358=FACE_OUTER_BOUND('',#2545,.T.);
#1359=FACE_OUTER_BOUND('',#2546,.T.);
#1360=FACE_OUTER_BOUND('',#2547,.T.);
#1361=FACE_OUTER_BOUND('',#2548,.T.);
#1362=FACE_OUTER_BOUND('',#2549,.T.);
#1363=FACE_OUTER_BOUND('',#2550,.T.);
#1364=FACE_OUTER_BOUND('',#2551,.T.);
#1365=FACE_OUTER_BOUND('',#2552,.T.);
#1366=FACE_OUTER_BOUND('',#2553,.T.);
#1367=FACE_OUTER_BOUND('',#2554,.T.);
#1368=FACE_OUTER_BOUND('',#2555,.T.);
#1369=FACE_OUTER_BOUND('',#2556,.T.);
#1370=FACE_OUTER_BOUND('',#2557,.T.);
#1371=FACE_OUTER_BOUND('',#2558,.T.);
#1372=FACE_OUTER_BOUND('',#2559,.T.);
#1373=FACE_OUTER_BOUND('',#2560,.T.);
#1374=FACE_OUTER_BOUND('',#2561,.T.);
#1375=FACE_OUTER_BOUND('',#2562,.T.);
#1376=FACE_OUTER_BOUND('',#2563,.T.);
#1377=FACE_OUTER_BOUND('',#2564,.T.);
#1378=FACE_OUTER_BOUND('',#2565,.T.);
#1379=FACE_OUTER_BOUND('',#2566,.T.);
#1380=FACE_OUTER_BOUND('',#2567,.T.);
#1381=FACE_OUTER_BOUND('',#2568,.T.);
#1382=FACE_OUTER_BOUND('',#2569,.T.);
#1383=FACE_OUTER_BOUND('',#2570,.T.);
#1384=FACE_OUTER_BOUND('',#2571,.T.);
#1385=FACE_OUTER_BOUND('',#2572,.T.);
#1386=FACE_OUTER_BOUND('',#2573,.T.);
#1387=FACE_OUTER_BOUND('',#2574,.T.);
#1388=FACE_OUTER_BOUND('',#2575,.T.);
#1389=FACE_OUTER_BOUND('',#2576,.T.);
#1390=FACE_OUTER_BOUND('',#2577,.T.);
#1391=FACE_OUTER_BOUND('',#2578,.T.);
#1392=FACE_OUTER_BOUND('',#2579,.T.);
#1393=FACE_OUTER_BOUND('',#2580,.T.);
#1394=FACE_OUTER_BOUND('',#2581,.T.);
#1395=FACE_OUTER_BOUND('',#2582,.T.);
#1396=FACE_OUTER_BOUND('',#2583,.T.);
#1397=FACE_OUTER_BOUND('',#2584,.T.);
#1398=FACE_OUTER_BOUND('',#2585,.T.);
#1399=FACE_OUTER_BOUND('',#2586,.T.);
#1400=FACE_OUTER_BOUND('',#2587,.T.);
#1401=FACE_OUTER_BOUND('',#2588,.T.);
#1402=FACE_OUTER_BOUND('',#2589,.T.);
#1403=FACE_OUTER_BOUND('',#2590,.T.);
#1404=FACE_OUTER_BOUND('',#2591,.T.);
#1405=FACE_OUTER_BOUND('',#2592,.T.);
#1406=FACE_OUTER_BOUND('',#2593,.T.);
#1407=FACE_OUTER_BOUND('',#2594,.T.);
#1408=FACE_OUTER_BOUND('',#2595,.T.);
#1409=FACE_OUTER_BOUND('',#2596,.T.);
#1410=FACE_OUTER_BOUND('',#2597,.T.);
#1411=FACE_OUTER_BOUND('',#2598,.T.);
#1412=FACE_OUTER_BOUND('',#2599,.T.);
#1413=FACE_OUTER_BOUND('',#2600,.T.);
#1414=FACE_OUTER_BOUND('',#2601,.T.);
#1415=FACE_OUTER_BOUND('',#2602,.T.);
#1416=FACE_OUTER_BOUND('',#2603,.T.);
#1417=FACE_OUTER_BOUND('',#2604,.T.);
#1418=FACE_OUTER_BOUND('',#2605,.T.);
#1419=FACE_OUTER_BOUND('',#2606,.T.);
#1420=FACE_OUTER_BOUND('',#2607,.T.);
#1421=FACE_OUTER_BOUND('',#2608,.T.);
#1422=FACE_OUTER_BOUND('',#2609,.T.);
#1423=FACE_OUTER_BOUND('',#2610,.T.);
#1424=FACE_OUTER_BOUND('',#2611,.T.);
#2312=EDGE_LOOP('',(#12188,#12189,#12190,#12191,#12192,#12193,#12194,#12195,
#12196,#12197,#12198,#12199,#12200,#12201,#12202,#12203));
#2313=EDGE_LOOP('',(#12204,#12205,#12206,#12207));
#2314=EDGE_LOOP('',(#12208,#12209,#12210,#12211));
#2315=EDGE_LOOP('',(#12212,#12213,#12214,#12215));
#2316=EDGE_LOOP('',(#12216,#12217,#12218,#12219));
#2317=EDGE_LOOP('',(#12220,#12221,#12222,#12223));
#2318=EDGE_LOOP('',(#12224,#12225,#12226,#12227));
#2319=EDGE_LOOP('',(#12228,#12229,#12230,#12231));
#2320=EDGE_LOOP('',(#12232,#12233,#12234,#12235));
#2321=EDGE_LOOP('',(#12236,#12237,#12238,#12239));
#2322=EDGE_LOOP('',(#12240,#12241,#12242,#12243));
#2323=EDGE_LOOP('',(#12244,#12245,#12246,#12247));
#2324=EDGE_LOOP('',(#12248,#12249,#12250,#12251));
#2325=EDGE_LOOP('',(#12252,#12253,#12254,#12255));
#2326=EDGE_LOOP('',(#12256,#12257,#12258,#12259));
#2327=EDGE_LOOP('',(#12260,#12261,#12262,#12263));
#2328=EDGE_LOOP('',(#12264,#12265,#12266,#12267));
#2329=EDGE_LOOP('',(#12268,#12269,#12270,#12271));
#2330=EDGE_LOOP('',(#12272,#12273,#12274,#12275));
#2331=EDGE_LOOP('',(#12276,#12277,#12278,#12279));
#2332=EDGE_LOOP('',(#12280,#12281,#12282,#12283));
#2333=EDGE_LOOP('',(#12284,#12285,#12286,#12287));
#2334=EDGE_LOOP('',(#12288,#12289,#12290,#12291));
#2335=EDGE_LOOP('',(#12292,#12293,#12294,#12295));
#2336=EDGE_LOOP('',(#12296,#12297,#12298,#12299));
#2337=EDGE_LOOP('',(#12300,#12301,#12302,#12303));
#2338=EDGE_LOOP('',(#12304,#12305,#12306,#12307));
#2339=EDGE_LOOP('',(#12308,#12309,#12310,#12311));
#2340=EDGE_LOOP('',(#12312,#12313,#12314,#12315));
#2341=EDGE_LOOP('',(#12316,#12317,#12318,#12319));
#2342=EDGE_LOOP('',(#12320,#12321,#12322,#12323));
#2343=EDGE_LOOP('',(#12324,#12325,#12326,#12327));
#2344=EDGE_LOOP('',(#12328,#12329,#12330,#12331));
#2345=EDGE_LOOP('',(#12332,#12333,#12334,#12335));
#2346=EDGE_LOOP('',(#12336,#12337,#12338,#12339));
#2347=EDGE_LOOP('',(#12340,#12341,#12342,#12343));
#2348=EDGE_LOOP('',(#12344,#12345,#12346,#12347));
#2349=EDGE_LOOP('',(#12348,#12349,#12350,#12351));
#2350=EDGE_LOOP('',(#12352,#12353,#12354,#12355));
#2351=EDGE_LOOP('',(#12356,#12357,#12358,#12359));
#2352=EDGE_LOOP('',(#12360,#12361,#12362,#12363));
#2353=EDGE_LOOP('',(#12364,#12365,#12366,#12367));
#2354=EDGE_LOOP('',(#12368,#12369,#12370,#12371));
#2355=EDGE_LOOP('',(#12372,#12373,#12374,#12375));
#2356=EDGE_LOOP('',(#12376,#12377,#12378,#12379));
#2357=EDGE_LOOP('',(#12380,#12381,#12382,#12383));
#2358=EDGE_LOOP('',(#12384,#12385,#12386,#12387));
#2359=EDGE_LOOP('',(#12388,#12389,#12390,#12391));
#2360=EDGE_LOOP('',(#12392,#12393,#12394,#12395));
#2361=EDGE_LOOP('',(#12396,#12397,#12398,#12399));
#2362=EDGE_LOOP('',(#12400,#12401,#12402,#12403));
#2363=EDGE_LOOP('',(#12404,#12405,#12406,#12407));
#2364=EDGE_LOOP('',(#12408,#12409,#12410,#12411));
#2365=EDGE_LOOP('',(#12412,#12413,#12414,#12415));
#2366=EDGE_LOOP('',(#12416,#12417,#12418,#12419));
#2367=EDGE_LOOP('',(#12420,#12421,#12422,#12423));
#2368=EDGE_LOOP('',(#12424,#12425,#12426,#12427));
#2369=EDGE_LOOP('',(#12428,#12429,#12430,#12431));
#2370=EDGE_LOOP('',(#12432,#12433,#12434,#12435));
#2371=EDGE_LOOP('',(#12436,#12437,#12438,#12439));
#2372=EDGE_LOOP('',(#12440,#12441,#12442,#12443));
#2373=EDGE_LOOP('',(#12444,#12445,#12446,#12447));
#2374=EDGE_LOOP('',(#12448,#12449,#12450,#12451));
#2375=EDGE_LOOP('',(#12452,#12453,#12454,#12455,#12456,#12457,#12458,#12459));
#2376=EDGE_LOOP('',(#12460,#12461,#12462,#12463));
#2377=EDGE_LOOP('',(#12464,#12465,#12466,#12467));
#2378=EDGE_LOOP('',(#12468,#12469,#12470,#12471));
#2379=EDGE_LOOP('',(#12472,#12473,#12474,#12475));
#2380=EDGE_LOOP('',(#12476,#12477,#12478,#12479));
#2381=EDGE_LOOP('',(#12480,#12481,#12482,#12483));
#2382=EDGE_LOOP('',(#12484,#12485,#12486,#12487));
#2383=EDGE_LOOP('',(#12488,#12489,#12490,#12491));
#2384=EDGE_LOOP('',(#12492,#12493,#12494,#12495));
#2385=EDGE_LOOP('',(#12496,#12497,#12498,#12499));
#2386=EDGE_LOOP('',(#12500,#12501,#12502,#12503));
#2387=EDGE_LOOP('',(#12504,#12505,#12506,#12507));
#2388=EDGE_LOOP('',(#12508,#12509,#12510,#12511));
#2389=EDGE_LOOP('',(#12512,#12513,#12514,#12515));
#2390=EDGE_LOOP('',(#12516,#12517,#12518,#12519));
#2391=EDGE_LOOP('',(#12520,#12521,#12522,#12523));
#2392=EDGE_LOOP('',(#12524,#12525,#12526,#12527));
#2393=EDGE_LOOP('',(#12528,#12529,#12530,#12531));
#2394=EDGE_LOOP('',(#12532,#12533,#12534,#12535));
#2395=EDGE_LOOP('',(#12536,#12537,#12538,#12539));
#2396=EDGE_LOOP('',(#12540,#12541,#12542,#12543));
#2397=EDGE_LOOP('',(#12544,#12545,#12546,#12547));
#2398=EDGE_LOOP('',(#12548,#12549,#12550,#12551));
#2399=EDGE_LOOP('',(#12552,#12553,#12554,#12555));
#2400=EDGE_LOOP('',(#12556,#12557,#12558,#12559));
#2401=EDGE_LOOP('',(#12560,#12561,#12562,#12563));
#2402=EDGE_LOOP('',(#12564,#12565,#12566,#12567));
#2403=EDGE_LOOP('',(#12568,#12569,#12570,#12571));
#2404=EDGE_LOOP('',(#12572,#12573,#12574,#12575));
#2405=EDGE_LOOP('',(#12576,#12577,#12578,#12579));
#2406=EDGE_LOOP('',(#12580,#12581,#12582,#12583));
#2407=EDGE_LOOP('',(#12584,#12585,#12586));
#2408=EDGE_LOOP('',(#12587,#12588,#12589,#12590,#12591));
#2409=EDGE_LOOP('',(#12592,#12593,#12594,#12595));
#2410=EDGE_LOOP('',(#12596,#12597,#12598,#12599));
#2411=EDGE_LOOP('',(#12600,#12601,#12602,#12603));
#2412=EDGE_LOOP('',(#12604,#12605,#12606,#12607));
#2413=EDGE_LOOP('',(#12608,#12609,#12610,#12611));
#2414=EDGE_LOOP('',(#12612,#12613,#12614,#12615));
#2415=EDGE_LOOP('',(#12616,#12617,#12618,#12619));
#2416=EDGE_LOOP('',(#12620,#12621,#12622,#12623));
#2417=EDGE_LOOP('',(#12624,#12625,#12626,#12627));
#2418=EDGE_LOOP('',(#12628,#12629,#12630,#12631));
#2419=EDGE_LOOP('',(#12632,#12633,#12634,#12635));
#2420=EDGE_LOOP('',(#12636,#12637,#12638,#12639));
#2421=EDGE_LOOP('',(#12640,#12641,#12642,#12643));
#2422=EDGE_LOOP('',(#12644,#12645,#12646,#12647));
#2423=EDGE_LOOP('',(#12648,#12649,#12650,#12651));
#2424=EDGE_LOOP('',(#12652,#12653,#12654,#12655));
#2425=EDGE_LOOP('',(#12656,#12657,#12658,#12659));
#2426=EDGE_LOOP('',(#12660,#12661,#12662,#12663));
#2427=EDGE_LOOP('',(#12664,#12665,#12666,#12667));
#2428=EDGE_LOOP('',(#12668,#12669,#12670,#12671));
#2429=EDGE_LOOP('',(#12672,#12673,#12674,#12675));
#2430=EDGE_LOOP('',(#12676,#12677,#12678,#12679));
#2431=EDGE_LOOP('',(#12680,#12681,#12682,#12683));
#2432=EDGE_LOOP('',(#12684,#12685,#12686,#12687));
#2433=EDGE_LOOP('',(#12688,#12689,#12690,#12691));
#2434=EDGE_LOOP('',(#12692,#12693,#12694,#12695));
#2435=EDGE_LOOP('',(#12696,#12697,#12698,#12699));
#2436=EDGE_LOOP('',(#12700,#12701,#12702,#12703));
#2437=EDGE_LOOP('',(#12704,#12705,#12706,#12707));
#2438=EDGE_LOOP('',(#12708,#12709,#12710,#12711));
#2439=EDGE_LOOP('',(#12712,#12713,#12714,#12715));
#2440=EDGE_LOOP('',(#12716,#12717,#12718,#12719));
#2441=EDGE_LOOP('',(#12720,#12721,#12722,#12723));
#2442=EDGE_LOOP('',(#12724,#12725,#12726,#12727));
#2443=EDGE_LOOP('',(#12728,#12729,#12730,#12731));
#2444=EDGE_LOOP('',(#12732,#12733,#12734,#12735));
#2445=EDGE_LOOP('',(#12736,#12737,#12738,#12739));
#2446=EDGE_LOOP('',(#12740,#12741,#12742,#12743));
#2447=EDGE_LOOP('',(#12744,#12745,#12746,#12747));
#2448=EDGE_LOOP('',(#12748,#12749,#12750,#12751));
#2449=EDGE_LOOP('',(#12752,#12753,#12754,#12755));
#2450=EDGE_LOOP('',(#12756,#12757,#12758,#12759));
#2451=EDGE_LOOP('',(#12760,#12761,#12762,#12763));
#2452=EDGE_LOOP('',(#12764,#12765,#12766,#12767));
#2453=EDGE_LOOP('',(#12768,#12769,#12770,#12771));
#2454=EDGE_LOOP('',(#12772,#12773,#12774,#12775));
#2455=EDGE_LOOP('',(#12776,#12777,#12778,#12779));
#2456=EDGE_LOOP('',(#12780,#12781,#12782,#12783));
#2457=EDGE_LOOP('',(#12784,#12785,#12786,#12787));
#2458=EDGE_LOOP('',(#12788,#12789,#12790,#12791));
#2459=EDGE_LOOP('',(#12792,#12793,#12794,#12795));
#2460=EDGE_LOOP('',(#12796,#12797,#12798,#12799));
#2461=EDGE_LOOP('',(#12800,#12801,#12802,#12803));
#2462=EDGE_LOOP('',(#12804,#12805,#12806,#12807));
#2463=EDGE_LOOP('',(#12808,#12809,#12810,#12811));
#2464=EDGE_LOOP('',(#12812,#12813,#12814,#12815));
#2465=EDGE_LOOP('',(#12816,#12817,#12818,#12819));
#2466=EDGE_LOOP('',(#12820,#12821,#12822,#12823));
#2467=EDGE_LOOP('',(#12824,#12825,#12826,#12827));
#2468=EDGE_LOOP('',(#12828,#12829,#12830,#12831));
#2469=EDGE_LOOP('',(#12832,#12833,#12834,#12835));
#2470=EDGE_LOOP('',(#12836,#12837,#12838,#12839));
#2471=EDGE_LOOP('',(#12840,#12841,#12842,#12843,#12844));
#2472=EDGE_LOOP('',(#12845,#12846,#12847,#12848));
#2473=EDGE_LOOP('',(#12849,#12850,#12851,#12852,#12853));
#2474=EDGE_LOOP('',(#12854,#12855,#12856,#12857,#12858,#12859));
#2475=EDGE_LOOP('',(#12860,#12861,#12862,#12863,#12864,#12865,#12866,#12867,
#12868,#12869,#12870,#12871,#12872,#12873,#12874,#12875,#12876,#12877,#12878,
#12879,#12880,#12881,#12882,#12883,#12884,#12885,#12886,#12887,#12888,#12889,
#12890,#12891,#12892,#12893,#12894,#12895,#12896,#12897,#12898,#12899,#12900,
#12901,#12902,#12903,#12904,#12905,#12906,#12907,#12908,#12909,#12910,#12911,
#12912,#12913,#12914,#12915,#12916,#12917,#12918,#12919,#12920,#12921,#12922,
#12923,#12924,#12925,#12926,#12927,#12928,#12929,#12930,#12931,#12932,#12933,
#12934,#12935,#12936,#12937,#12938,#12939,#12940,#12941,#12942,#12943,#12944,
#12945,#12946,#12947,#12948,#12949,#12950,#12951,#12952,#12953,#12954,#12955,
#12956,#12957,#12958,#12959,#12960,#12961,#12962,#12963,#12964,#12965,#12966,
#12967,#12968,#12969,#12970,#12971,#12972,#12973,#12974,#12975,#12976,#12977,
#12978,#12979,#12980,#12981,#12982,#12983,#12984,#12985,#12986,#12987));
#2476=EDGE_LOOP('',(#12988,#12989,#12990,#12991,#12992));
#2477=EDGE_LOOP('',(#12993,#12994,#12995,#12996));
#2478=EDGE_LOOP('',(#12997,#12998,#12999,#13000,#13001,#13002,#13003,#13004,
#13005,#13006,#13007,#13008,#13009,#13010,#13011,#13012,#13013,#13014,#13015,
#13016,#13017,#13018,#13019,#13020,#13021,#13022,#13023,#13024,#13025,#13026,
#13027,#13028,#13029,#13030,#13031,#13032,#13033,#13034,#13035,#13036,#13037,
#13038,#13039,#13040,#13041,#13042,#13043,#13044,#13045,#13046,#13047,#13048,
#13049,#13050,#13051,#13052,#13053,#13054,#13055,#13056,#13057,#13058,#13059,
#13060,#13061,#13062,#13063,#13064,#13065,#13066,#13067,#13068,#13069,#13070,
#13071,#13072,#13073,#13074,#13075,#13076,#13077,#13078,#13079,#13080,#13081,
#13082,#13083,#13084,#13085,#13086,#13087,#13088,#13089,#13090,#13091,#13092,
#13093,#13094,#13095,#13096,#13097,#13098,#13099,#13100,#13101,#13102,#13103,
#13104,#13105,#13106,#13107,#13108,#13109,#13110,#13111,#13112,#13113,#13114,
#13115,#13116,#13117,#13118,#13119,#13120,#13121,#13122,#13123,#13124,#13125));
#2479=EDGE_LOOP('',(#13126,#13127,#13128,#13129,#13130));
#2480=EDGE_LOOP('',(#13131,#13132,#13133,#13134,#13135,#13136,#13137,#13138,
#13139,#13140,#13141,#13142,#13143,#13144,#13145,#13146,#13147,#13148,#13149,
#13150,#13151,#13152,#13153,#13154,#13155,#13156,#13157,#13158,#13159,#13160,
#13161,#13162,#13163,#13164,#13165,#13166));
#2481=EDGE_LOOP('',(#13167,#13168,#13169,#13170,#13171));
#2482=EDGE_LOOP('',(#13172,#13173,#13174,#13175));
#2483=EDGE_LOOP('',(#13176,#13177,#13178,#13179,#13180,#13181,#13182,#13183,
#13184,#13185,#13186,#13187,#13188,#13189,#13190,#13191,#13192,#13193,#13194,
#13195,#13196,#13197,#13198,#13199,#13200,#13201,#13202,#13203,#13204,#13205,
#13206,#13207,#13208,#13209,#13210,#13211));
#2484=EDGE_LOOP('',(#13212,#13213,#13214,#13215));
#2485=EDGE_LOOP('',(#13216,#13217,#13218,#13219));
#2486=EDGE_LOOP('',(#13220,#13221,#13222,#13223,#13224,#13225));
#2487=EDGE_LOOP('',(#13226,#13227,#13228,#13229));
#2488=EDGE_LOOP('',(#13230,#13231,#13232,#13233,#13234,#13235));
#2489=EDGE_LOOP('',(#13236,#13237,#13238,#13239));
#2490=EDGE_LOOP('',(#13240,#13241,#13242,#13243));
#2491=EDGE_LOOP('',(#13244,#13245,#13246,#13247));
#2492=EDGE_LOOP('',(#13248,#13249,#13250,#13251));
#2493=EDGE_LOOP('',(#13252,#13253,#13254,#13255));
#2494=EDGE_LOOP('',(#13256,#13257,#13258,#13259));
#2495=EDGE_LOOP('',(#13260,#13261,#13262,#13263,#13264,#13265));
#2496=EDGE_LOOP('',(#13266,#13267,#13268,#13269));
#2497=EDGE_LOOP('',(#13270,#13271,#13272,#13273,#13274,#13275));
#2498=EDGE_LOOP('',(#13276,#13277,#13278,#13279));
#2499=EDGE_LOOP('',(#13280,#13281,#13282,#13283));
#2500=EDGE_LOOP('',(#13284,#13285,#13286,#13287));
#2501=EDGE_LOOP('',(#13288,#13289,#13290,#13291));
#2502=EDGE_LOOP('',(#13292,#13293,#13294,#13295));
#2503=EDGE_LOOP('',(#13296,#13297,#13298,#13299,#13300,#13301));
#2504=EDGE_LOOP('',(#13302,#13303,#13304,#13305));
#2505=EDGE_LOOP('',(#13306,#13307,#13308,#13309,#13310,#13311));
#2506=EDGE_LOOP('',(#13312,#13313,#13314,#13315));
#2507=EDGE_LOOP('',(#13316,#13317,#13318,#13319));
#2508=EDGE_LOOP('',(#13320,#13321,#13322,#13323));
#2509=EDGE_LOOP('',(#13324,#13325,#13326,#13327));
#2510=EDGE_LOOP('',(#13328,#13329,#13330,#13331));
#2511=EDGE_LOOP('',(#13332,#13333,#13334,#13335,#13336,#13337));
#2512=EDGE_LOOP('',(#13338,#13339,#13340,#13341));
#2513=EDGE_LOOP('',(#13342,#13343,#13344,#13345,#13346,#13347));
#2514=EDGE_LOOP('',(#13348,#13349,#13350,#13351));
#2515=EDGE_LOOP('',(#13352,#13353,#13354,#13355));
#2516=EDGE_LOOP('',(#13356,#13357,#13358,#13359));
#2517=EDGE_LOOP('',(#13360,#13361,#13362,#13363));
#2518=EDGE_LOOP('',(#13364,#13365,#13366,#13367));
#2519=EDGE_LOOP('',(#13368,#13369,#13370,#13371,#13372,#13373));
#2520=EDGE_LOOP('',(#13374,#13375,#13376,#13377));
#2521=EDGE_LOOP('',(#13378,#13379,#13380,#13381,#13382,#13383));
#2522=EDGE_LOOP('',(#13384,#13385,#13386,#13387));
#2523=EDGE_LOOP('',(#13388,#13389,#13390,#13391));
#2524=EDGE_LOOP('',(#13392,#13393,#13394,#13395));
#2525=EDGE_LOOP('',(#13396,#13397,#13398,#13399));
#2526=EDGE_LOOP('',(#13400,#13401,#13402,#13403));
#2527=EDGE_LOOP('',(#13404,#13405,#13406,#13407,#13408,#13409));
#2528=EDGE_LOOP('',(#13410,#13411,#13412,#13413));
#2529=EDGE_LOOP('',(#13414,#13415,#13416,#13417,#13418,#13419));
#2530=EDGE_LOOP('',(#13420,#13421,#13422,#13423));
#2531=EDGE_LOOP('',(#13424,#13425,#13426,#13427));
#2532=EDGE_LOOP('',(#13428,#13429,#13430,#13431));
#2533=EDGE_LOOP('',(#13432,#13433,#13434,#13435));
#2534=EDGE_LOOP('',(#13436,#13437,#13438,#13439));
#2535=EDGE_LOOP('',(#13440,#13441,#13442,#13443,#13444,#13445));
#2536=EDGE_LOOP('',(#13446,#13447,#13448,#13449));
#2537=EDGE_LOOP('',(#13450,#13451,#13452,#13453,#13454,#13455));
#2538=EDGE_LOOP('',(#13456,#13457,#13458,#13459));
#2539=EDGE_LOOP('',(#13460,#13461,#13462,#13463));
#2540=EDGE_LOOP('',(#13464,#13465,#13466,#13467));
#2541=EDGE_LOOP('',(#13468,#13469,#13470,#13471));
#2542=EDGE_LOOP('',(#13472,#13473,#13474,#13475,#13476));
#2543=EDGE_LOOP('',(#13477,#13478,#13479,#13480,#13481,#13482));
#2544=EDGE_LOOP('',(#13483,#13484,#13485,#13486));
#2545=EDGE_LOOP('',(#13487,#13488,#13489,#13490,#13491,#13492));
#2546=EDGE_LOOP('',(#13493,#13494,#13495,#13496,#13497));
#2547=EDGE_LOOP('',(#13498,#13499,#13500,#13501));
#2548=EDGE_LOOP('',(#13502,#13503,#13504,#13505));
#2549=EDGE_LOOP('',(#13506,#13507,#13508,#13509));
#2550=EDGE_LOOP('',(#13510,#13511,#13512,#13513));
#2551=EDGE_LOOP('',(#13514,#13515,#13516,#13517,#13518,#13519));
#2552=EDGE_LOOP('',(#13520,#13521,#13522,#13523));
#2553=EDGE_LOOP('',(#13524,#13525,#13526,#13527,#13528,#13529));
#2554=EDGE_LOOP('',(#13530,#13531,#13532,#13533));
#2555=EDGE_LOOP('',(#13534,#13535,#13536,#13537));
#2556=EDGE_LOOP('',(#13538,#13539,#13540,#13541));
#2557=EDGE_LOOP('',(#13542,#13543,#13544,#13545));
#2558=EDGE_LOOP('',(#13546,#13547,#13548,#13549));
#2559=EDGE_LOOP('',(#13550,#13551,#13552,#13553,#13554,#13555));
#2560=EDGE_LOOP('',(#13556,#13557,#13558,#13559));
#2561=EDGE_LOOP('',(#13560,#13561,#13562,#13563,#13564,#13565));
#2562=EDGE_LOOP('',(#13566,#13567,#13568,#13569));
#2563=EDGE_LOOP('',(#13570,#13571,#13572,#13573));
#2564=EDGE_LOOP('',(#13574,#13575,#13576,#13577));
#2565=EDGE_LOOP('',(#13578,#13579,#13580,#13581));
#2566=EDGE_LOOP('',(#13582,#13583,#13584,#13585));
#2567=EDGE_LOOP('',(#13586,#13587,#13588,#13589,#13590,#13591));
#2568=EDGE_LOOP('',(#13592,#13593,#13594,#13595));
#2569=EDGE_LOOP('',(#13596,#13597,#13598,#13599,#13600,#13601));
#2570=EDGE_LOOP('',(#13602,#13603,#13604,#13605));
#2571=EDGE_LOOP('',(#13606,#13607,#13608,#13609));
#2572=EDGE_LOOP('',(#13610,#13611,#13612,#13613));
#2573=EDGE_LOOP('',(#13614,#13615,#13616,#13617));
#2574=EDGE_LOOP('',(#13618,#13619,#13620,#13621));
#2575=EDGE_LOOP('',(#13622,#13623,#13624,#13625,#13626,#13627));
#2576=EDGE_LOOP('',(#13628,#13629,#13630,#13631));
#2577=EDGE_LOOP('',(#13632,#13633,#13634,#13635,#13636,#13637));
#2578=EDGE_LOOP('',(#13638,#13639,#13640,#13641));
#2579=EDGE_LOOP('',(#13642,#13643,#13644,#13645));
#2580=EDGE_LOOP('',(#13646,#13647,#13648,#13649));
#2581=EDGE_LOOP('',(#13650,#13651,#13652,#13653));
#2582=EDGE_LOOP('',(#13654,#13655,#13656,#13657));
#2583=EDGE_LOOP('',(#13658,#13659,#13660,#13661,#13662,#13663));
#2584=EDGE_LOOP('',(#13664,#13665,#13666,#13667));
#2585=EDGE_LOOP('',(#13668,#13669,#13670,#13671,#13672,#13673));
#2586=EDGE_LOOP('',(#13674,#13675,#13676,#13677));
#2587=EDGE_LOOP('',(#13678,#13679,#13680,#13681));
#2588=EDGE_LOOP('',(#13682,#13683,#13684,#13685));
#2589=EDGE_LOOP('',(#13686,#13687,#13688,#13689));
#2590=EDGE_LOOP('',(#13690,#13691,#13692,#13693));
#2591=EDGE_LOOP('',(#13694,#13695,#13696,#13697,#13698,#13699));
#2592=EDGE_LOOP('',(#13700,#13701,#13702,#13703));
#2593=EDGE_LOOP('',(#13704,#13705,#13706,#13707,#13708,#13709));
#2594=EDGE_LOOP('',(#13710,#13711,#13712,#13713));
#2595=EDGE_LOOP('',(#13714,#13715,#13716,#13717));
#2596=EDGE_LOOP('',(#13718,#13719,#13720,#13721));
#2597=EDGE_LOOP('',(#13722,#13723,#13724,#13725));
#2598=EDGE_LOOP('',(#13726,#13727,#13728,#13729,#13730,#13731));
#2599=EDGE_LOOP('',(#13732,#13733,#13734,#13735));
#2600=EDGE_LOOP('',(#13736,#13737,#13738,#13739));
#2601=EDGE_LOOP('',(#13740,#13741,#13742,#13743,#13744,#13745));
#2602=EDGE_LOOP('',(#13746,#13747,#13748,#13749));
#2603=EDGE_LOOP('',(#13750,#13751,#13752,#13753));
#2604=EDGE_LOOP('',(#13754,#13755,#13756,#13757));
#2605=EDGE_LOOP('',(#13758));
#2606=EDGE_LOOP('',(#13759,#13760,#13761,#13762));
#2607=EDGE_LOOP('',(#13763,#13764,#13765,#13766,#13767,#13768,#13769,#13770,
#13771,#13772,#13773,#13774,#13775,#13776,#13777,#13778,#13779,#13780,#13781,
#13782,#13783,#13784,#13785,#13786,#13787,#13788,#13789,#13790,#13791,#13792,
#13793,#13794,#13795,#13796,#13797,#13798));
#2608=EDGE_LOOP('',(#13799,#13800,#13801,#13802,#13803,#13804,#13805,#13806,
#13807,#13808,#13809,#13810,#13811,#13812,#13813,#13814,#13815,#13816,#13817,
#13818,#13819,#13820,#13821,#13822,#13823,#13824,#13825,#13826,#13827,#13828,
#13829,#13830,#13831,#13832));
#2609=EDGE_LOOP('',(#13833,#13834,#13835,#13836));
#2610=EDGE_LOOP('',(#13837,#13838,#13839,#13840,#13841,#13842));
#2611=EDGE_LOOP('',(#13843));
#3542=CIRCLE('',#20144,6.933);
#3543=CIRCLE('',#20145,6.933);
#3544=CIRCLE('',#20146,6.933);
#3545=CIRCLE('',#20147,6.933);
#3546=CIRCLE('',#20148,6.933);
#3547=CIRCLE('',#20149,6.933);
#3548=CIRCLE('',#20150,6.933);
#3549=CIRCLE('',#20151,6.933);
#3550=CIRCLE('',#20152,6.933);
#3551=CIRCLE('',#20215,6.933);
#3552=CIRCLE('',#20216,6.933);
#3553=CIRCLE('',#20217,6.933);
#3554=CIRCLE('',#20234,6.21925);
#3555=CIRCLE('',#20251,6.21925);
#3556=CIRCLE('',#20253,6.21925);
#3557=CIRCLE('',#20320,6.933);
#3558=CIRCLE('',#20321,6.933);
#3559=CIRCLE('',#20323,6.21925);
#3560=CIRCLE('',#20326,6.933);
#3561=CIRCLE('',#20327,6.933);
#3562=CIRCLE('',#20329,6.21925);
#3563=CIRCLE('',#20332,6.933);
#3564=CIRCLE('',#20334,10.125);
#3565=CIRCLE('',#20335,7.8125);
#3566=CIRCLE('',#20337,7.8125);
#3567=CIRCLE('',#20339,10.125);
#3568=CIRCLE('',#20341,10.625);
#3569=CIRCLE('',#20342,10.125);
#3570=CIRCLE('',#20344,10.125);
#3571=CIRCLE('',#20345,10.625);
#3572=CIRCLE('',#20347,10.625);
#3573=CIRCLE('',#20349,10.125);
#3574=CIRCLE('',#20351,10.125);
#3575=CIRCLE('',#20352,7.8125);
#3576=CIRCLE('',#20354,7.8125);
#3577=CIRCLE('',#20356,10.125);
#3578=CIRCLE('',#20358,10.625);
#3579=CIRCLE('',#20359,10.125);
#3580=CIRCLE('',#20361,10.625);
#3581=CIRCLE('',#20363,10.125);
#3582=CIRCLE('',#20365,10.125);
#3583=CIRCLE('',#20366,7.8125);
#3584=CIRCLE('',#20368,7.8125);
#3585=CIRCLE('',#20370,10.125);
#3586=CIRCLE('',#20372,10.625);
#3587=CIRCLE('',#20373,10.125);
#3588=CIRCLE('',#20375,10.625);
#3589=CIRCLE('',#20377,10.125);
#3590=CIRCLE('',#20379,10.125);
#3591=CIRCLE('',#20380,7.8125);
#3592=CIRCLE('',#20382,7.8125);
#3593=CIRCLE('',#20384,10.125);
#3594=CIRCLE('',#20386,10.625);
#3595=CIRCLE('',#20387,10.125);
#3596=CIRCLE('',#20389,10.625);
#3597=CIRCLE('',#20391,10.125);
#3598=CIRCLE('',#20393,10.125);
#3599=CIRCLE('',#20394,7.8125);
#3600=CIRCLE('',#20396,7.8125);
#3601=CIRCLE('',#20398,10.125);
#3602=CIRCLE('',#20400,10.625);
#3603=CIRCLE('',#20401,10.125);
#3604=CIRCLE('',#20403,10.625);
#3605=CIRCLE('',#20405,10.125);
#3606=CIRCLE('',#20407,10.125);
#3607=CIRCLE('',#20408,7.8125);
#3608=CIRCLE('',#20410,7.8125);
#3609=CIRCLE('',#20412,10.125);
#3610=CIRCLE('',#20414,10.625);
#3611=CIRCLE('',#20415,10.125);
#3612=CIRCLE('',#20417,10.625);
#3613=CIRCLE('',#20419,10.125);
#3614=CIRCLE('',#20421,10.125);
#3615=CIRCLE('',#20422,7.8125);
#3616=CIRCLE('',#20424,7.8125);
#3617=CIRCLE('',#20426,10.125);
#3618=CIRCLE('',#20428,10.625);
#3619=CIRCLE('',#20429,10.125);
#3620=CIRCLE('',#20431,10.625);
#3621=CIRCLE('',#20433,10.125);
#3622=CIRCLE('',#20435,10.125);
#3623=CIRCLE('',#20436,10.125);
#3624=CIRCLE('',#20437,7.8125);
#3625=CIRCLE('',#20439,7.8125);
#3626=CIRCLE('',#20441,10.125);
#3627=CIRCLE('',#20442,10.125);
#3628=CIRCLE('',#20444,10.625);
#3629=CIRCLE('',#20445,10.125);
#3630=CIRCLE('',#20447,10.625);
#3631=CIRCLE('',#20449,10.125);
#3632=CIRCLE('',#20451,10.125);
#3633=CIRCLE('',#20452,7.8125);
#3634=CIRCLE('',#20454,7.8125);
#3635=CIRCLE('',#20456,10.125);
#3636=CIRCLE('',#20458,10.625);
#3637=CIRCLE('',#20459,10.125);
#3638=CIRCLE('',#20461,10.625);
#3639=CIRCLE('',#20463,10.125);
#3640=CIRCLE('',#20465,10.125);
#3641=CIRCLE('',#20466,7.8125);
#3642=CIRCLE('',#20468,7.8125);
#3643=CIRCLE('',#20470,10.125);
#3644=CIRCLE('',#20472,10.625);
#3645=CIRCLE('',#20473,10.125);
#3646=CIRCLE('',#20475,10.625);
#3647=CIRCLE('',#20477,10.125);
#3648=CIRCLE('',#20479,10.125);
#3649=CIRCLE('',#20480,7.8125);
#3650=CIRCLE('',#20482,7.8125);
#3651=CIRCLE('',#20484,10.125);
#3652=CIRCLE('',#20486,10.625);
#3653=CIRCLE('',#20487,10.125);
#3654=CIRCLE('',#20489,10.625);
#3655=CIRCLE('',#20491,10.125);
#3656=CIRCLE('',#20493,10.125);
#3657=CIRCLE('',#20494,7.8125);
#3658=CIRCLE('',#20496,7.8125);
#3659=CIRCLE('',#20498,10.125);
#3660=CIRCLE('',#20500,10.625);
#3661=CIRCLE('',#20501,10.125);
#3662=CIRCLE('',#20503,10.625);
#3663=CIRCLE('',#20505,10.125);
#3664=CIRCLE('',#20507,10.125);
#3665=CIRCLE('',#20508,7.8125);
#3666=CIRCLE('',#20510,7.8125);
#3667=CIRCLE('',#20512,10.125);
#3668=CIRCLE('',#20514,10.625);
#3669=CIRCLE('',#20515,10.125);
#3670=CIRCLE('',#20517,10.625);
#3671=CIRCLE('',#20519,10.125);
#3672=CIRCLE('',#20521,10.125);
#3673=CIRCLE('',#20522,7.8125);
#3674=CIRCLE('',#20524,7.8125);
#3675=CIRCLE('',#20526,10.125);
#3676=CIRCLE('',#20528,10.625);
#3677=CIRCLE('',#20529,10.125);
#3678=CIRCLE('',#20531,10.625);
#3679=CIRCLE('',#20533,10.125);
#3680=CIRCLE('',#20535,10.125);
#3681=CIRCLE('',#20536,7.8125);
#3682=CIRCLE('',#20538,7.8125);
#3683=CIRCLE('',#20540,10.125);
#3684=CIRCLE('',#20542,10.625);
#3685=CIRCLE('',#20543,10.125);
#3686=CIRCLE('',#20546,6.);
#3687=CIRCLE('',#20551,6.933);
#3688=CIRCLE('',#20553,6.);
#4669=B_SPLINE_CURVE_WITH_KNOTS('',3,(#27826,#27827,#27828,#27829,#27830,
#27831,#27832,#27833,#27834,#27835,#27836,#27837,#27838,#27839,#27840,#27841,
#27842,#27843,#27844,#27845,#27846,#27847,#27848,#27849,#27850),
 .UNSPECIFIED.,.F.,.F.,(4,3,3,3,3,3,3,3,4),(-7.57991119318069,-6.9847970994778,
-6.48588302094367,-5.98696894240955,-5.48805486387542,-4.98914078534129,
-3.99131262827303,-2.99348447120477,-2.07135887395547),.UNSPECIFIED.);
#4670=B_SPLINE_CURVE_WITH_KNOTS('',3,(#27871,#27872,#27873,#27874,#27875,
#27876,#27877,#27878,#27879,#27880,#27881,#27882,#27883,#27884,#27885,#27886,
#27887,#27888,#27889,#27890,#27891,#27892),.UNSPECIFIED.,.F.,.F.,(4,3,3,
3,3,3,3,4),(0.,0.498914078534124,0.99782815706825,1.49674223560237,1.9956563141365,
2.99348447120475,3.991312628273,4.60707443244022),.UNSPECIFIED.);
#4671=B_SPLINE_CURVE_WITH_KNOTS('',3,(#27905,#27906,#27907,#27908,#27909,
#27910,#27911,#27912,#27913,#27914,#27915,#27916,#27917,#27918,#27919,#27920,
#27921,#27922,#27923,#27924,#27925,#27926,#27927,#27928,#27929,#27930,#27931,
#27932),.UNSPECIFIED.,.F.,.F.,(4,3,3,3,3,3,3,3,3,4),(-13.8630965003603,
-13.4706801204215,-12.9717660418873,-12.4728519633532,-11.9739378848191,
-10.9761097277508,-9.97828157068257,-8.98045341361432,-7.98262525654606,
-7.57991119318069),.UNSPECIFIED.);
#4672=B_SPLINE_CURVE_WITH_KNOTS('',3,(#27933,#27934,#27935,#27936,#27937,
#27938,#27939,#27940,#27941,#27942,#27943,#27944,#27945,#27946,#27947,#27948,
#27949,#27950,#27951,#27952,#27953,#27954,#27955,#27956,#27957,#27958,#27959,
#27960),.UNSPECIFIED.,.F.,.F.,(4,3,3,3,3,3,3,3,3,4),(4.60707443244022,4.98914078534126,
5.48805486387539,5.98696894240953,6.48588302094366,6.9847970994778,7.98262525654606,
8.98045341361433,9.9782815706826,10.8902597396198),.UNSPECIFIED.);
#4673=B_SPLINE_CURVE_WITH_KNOTS('',3,(#27965,#27966,#27967,#27968,#27969,
#27970,#27971,#27972,#27973,#27974,#27975,#27976,#27977,#27978,#27979,#27980,
#27981,#27982,#27983,#27984,#27985,#27986,#27987,#27988,#27989),
 .UNSPECIFIED.,.F.,.F.,(4,3,3,3,3,3,3,3,4),(-20.1462818075399,-19.2833612722667,
-18.4204407369935,-17.5575202017204,-16.6945996664472,-15.831679131174,
-14.9687585959009,-14.1058380606277,-13.8630965003603),.UNSPECIFIED.);
#4674=B_SPLINE_CURVE_WITH_KNOTS('',3,(#27990,#27991,#27992,#27993,#27994,
#27995,#27996,#27997,#27998,#27999,#28000,#28001,#28002,#28003,#28004,#28005,
#28006,#28007,#28008,#28009,#28010,#28011,#28012,#28013,#28014,#28015,#28016,
#28017,#28018,#28019,#28020),.UNSPECIFIED.,.F.,.F.,(4,3,3,3,3,3,3,3,3,3,
4),(10.8902597396198,10.9761097277509,11.9739378848191,12.4728519633533,
12.9717660418874,13.4706801204215,13.9695941989556,14.9674223560239,15.9652505130921,
16.9630786701604,17.1734450467994),.UNSPECIFIED.);
#4675=B_SPLINE_CURVE_WITH_KNOTS('',3,(#28025,#28026,#28027,#28028,#28029,
#28030,#28031,#28032,#28033,#28034,#28035,#28036,#28037,#28038,#28039,#28040,
#28041,#28042,#28043,#28044,#28045,#28046,#28047,#28048,#28049),
 .UNSPECIFIED.,.F.,.F.,(4,3,3,3,3,3,3,3,4),(-26.4294671147194,-25.9435320837747,
-24.9457039267064,-23.9478757696382,-22.9500476125699,-21.9522194555017,
-20.9543912984334,-20.4554772198993,-20.1462818075399),.UNSPECIFIED.);
#4676=B_SPLINE_CURVE_WITH_KNOTS('',3,(#28050,#28051,#28052,#28053,#28054,
#28055,#28056,#28057,#28058,#28059,#28060,#28061,#28062,#28063,#28064,#28065,
#28066,#28067,#28068,#28069,#28070,#28071,#28072,#28073,#28074,#28075,#28076,
#28077),.UNSPECIFIED.,.F.,.F.,(4,3,3,3,3,3,3,3,3,4),(17.1734450467994,17.9609068272287,
18.9587349842969,19.457649062831,19.9565631413651,20.4554772198993,20.9543912984334,
21.9522194555017,22.9500476125699,23.456630353979),.UNSPECIFIED.);
#4677=B_SPLINE_CURVE_WITH_KNOTS('',3,(#28082,#28083,#28084,#28085,#28086,
#28087,#28088,#28089,#28090,#28091,#28092,#28093,#28094,#28095,#28096,#28097,
#28098,#28099,#28100,#28101,#28102,#28103,#28104,#28105,#28106,#28107,#28108,
#28109),.UNSPECIFIED.,.F.,.F.,(4,3,3,3,3,3,3,3,3,4),(-32.712652421899,-31.9305010261842,
-30.932672869116,-29.9348447120477,-28.9370165549795,-27.9391883979112,
-27.4402743193771,-26.9413602408429,-26.4424461623088,-26.4294671147194),
 .UNSPECIFIED.);
#4678=B_SPLINE_CURVE_WITH_KNOTS('',3,(#28110,#28111,#28112,#28113,#28114,
#28115,#28116,#28117,#28118,#28119,#28120,#28121,#28122,#28123,#28124,#28125,
#28126,#28127,#28128,#28129,#28130,#28131,#28132,#28133,#28134,#28135,#28136,
#28137),.UNSPECIFIED.,.F.,.F.,(4,3,3,3,3,3,3,3,3,4),(23.456630353979,23.9478757696382,
24.9457039267064,25.9435320837747,26.4424461623088,26.941360240843,27.4402743193771,
27.9391883979112,28.9370165549795,29.7398156611586),.UNSPECIFIED.);
#4679=B_SPLINE_CURVE_WITH_KNOTS('',3,(#28142,#28143,#28144,#28145,#28146,
#28147,#28148,#28149,#28150,#28151,#28152,#28153,#28154,#28155,#28156,#28157,
#28158,#28159,#28160,#28161,#28162,#28163,#28164,#28165,#28166),
 .UNSPECIFIED.,.F.,.F.,(4,3,3,3,3,3,3,3,4),(-38.9958377290786,-38.1329171938055,
-37.2699966585323,-36.4070761232591,-35.544155587986,-34.6812350527128,
-33.8183145174396,-32.9553939821665,-32.712652421899),.UNSPECIFIED.);
#4680=B_SPLINE_CURVE_WITH_KNOTS('',3,(#28167,#28168,#28169,#28170,#28171,
#28172,#28173,#28174,#28175,#28176,#28177,#28178,#28179,#28180,#28181,#28182,
#28183,#28184,#28185,#28186,#28187,#28188,#28189,#28190,#28191,#28192,#28193,
#28194,#28195,#28196,#28197),.UNSPECIFIED.,.F.,.F.,(4,3,3,3,3,3,3,3,3,3,
4),(29.7398156611586,29.9348447120478,30.932672869116,31.9305010261843,
32.9283291832525,33.4272432617867,33.9261573403208,34.4250714188549,34.923985497389,
35.9218136544573,36.0230009683381),.UNSPECIFIED.);
#4681=B_SPLINE_CURVE_WITH_KNOTS('',3,(#28202,#28203,#28204,#28205,#28206,
#28207,#28208,#28209,#28210,#28211,#28212,#28213,#28214,#28215,#28216,#28217,
#28218,#28219,#28220,#28221,#28222,#28223,#28224,#28225,#28226,#28227,#28228,
#28229),.UNSPECIFIED.,.F.,.F.,(4,3,3,3,3,3,3,3,3,4),(-45.2790230362582,
-44.9022670680716,-43.9044389110033,-42.9066107539351,-41.9087825968668,
-41.4098685183327,-40.9109544397985,-40.4120403612644,-39.9131262827303,
-38.9958377290786),.UNSPECIFIED.);
#4682=B_SPLINE_CURVE_WITH_KNOTS('',3,(#28230,#28231,#28232,#28233,#28234,
#28235,#28236,#28237,#28238,#28239,#28240,#28241,#28242,#28243,#28244,#28245,
#28246,#28247,#28248,#28249,#28250,#28251,#28252,#28253,#28254,#28255,#28256,
#28257),.UNSPECIFIED.,.F.,.F.,(4,3,3,3,3,3,3,3,3,4),(36.0230009683381,36.9196418115256,
37.9174699685938,38.915298125662,39.9131262827303,40.4120403612644,40.9109544397986,
41.4098685183327,41.9087825968668,42.3061862755177),.UNSPECIFIED.);
#4683=B_SPLINE_CURVE_WITH_KNOTS('',3,(#28262,#28263,#28264,#28265,#28266,
#28267,#28268,#28269,#28270,#28271,#28272,#28273,#28274,#28275,#28276,#28277,
#28278,#28279,#28280,#28281,#28282,#28283,#28284,#28285,#28286,#28287,#28288,
#28289),.UNSPECIFIED.,.F.,.F.,(4,3,3,3,3,3,3,3,3,4),(-51.5622083434378,
-50.8892360104811,-49.8914078534129,-48.8935796963446,-48.3946656178105,
-47.8957515392764,-47.3968374607422,-46.8979233822081,-45.9000952251398,
-45.2790230362582),.UNSPECIFIED.);
#4684=B_SPLINE_CURVE_WITH_KNOTS('',3,(#28290,#28291,#28292,#28293,#28294,
#28295,#28296,#28297,#28298,#28299,#28300,#28301,#28302,#28303,#28304,#28305,
#28306,#28307,#28308,#28309,#28310,#28311,#28312,#28313,#28314),
 .UNSPECIFIED.,.F.,.F.,(4,3,3,3,3,3,3,3,4),(42.3061862755177,43.1691068107909,
44.0320273460641,44.8949478813372,45.7578684166104,46.6207889518835,47.4837094871567,
48.3466300224299,48.5893715826973),.UNSPECIFIED.);
#4685=B_SPLINE_CURVE_WITH_KNOTS('',3,(#28319,#28320,#28321,#28322,#28323,
#28324,#28325,#28326,#28327,#28328,#28329,#28330,#28331,#28332,#28333,#28334,
#28335,#28336,#28337,#28338,#28339,#28340,#28341,#28342,#28343,#28344,#28345,
#28346),.UNSPECIFIED.,.F.,.F.,(4,3,3,3,3,3,3,3,3,4),(-57.8453936506174,
-56.8762049528907,-55.8783767958224,-55.3794627172883,-54.8805486387542,
-54.38163456022,-53.8827204816859,-52.8848923246177,-51.8870641675494,-51.5622083434378),
 .UNSPECIFIED.);
#4686=B_SPLINE_CURVE_WITH_KNOTS('',3,(#28347,#28348,#28349,#28350,#28351,
#28352,#28353,#28354,#28355,#28356,#28357,#28358,#28359,#28360,#28361,#28362,
#28363,#28364,#28365,#28366,#28367,#28368,#28369,#28370,#28371),
 .UNSPECIFIED.,.F.,.F.,(4,3,3,3,3,3,3,3,4),(48.5893715826973,48.8935796963447,
49.8914078534129,50.8892360104811,51.8870641675494,52.8848923246177,53.8827204816859,
54.38163456022,54.8725568898769),.UNSPECIFIED.);
#4687=B_SPLINE_CURVE_WITH_KNOTS('',3,(#28376,#28377,#28378,#28379,#28380,
#28381,#28382,#28383,#28384,#28385,#28386,#28387,#28388,#28389,#28390,#28391,
#28392,#28393,#28394,#28395,#28396,#28397,#28398,#28399,#28400,#28401,#28402,
#28403,#28404,#28405,#28406),.UNSPECIFIED.,.F.,.F.,(4,3,3,3,3,3,3,3,3,3,
4),(-64.128578957797,-63.8610020523685,-62.8631738953002,-62.3642598167661,
-61.865345738232,-61.3664316596978,-60.8675175811637,-59.8696894240954,
-58.8718612670272,-57.8740331099589,-57.8453936506174),.UNSPECIFIED.);
#4688=B_SPLINE_CURVE_WITH_KNOTS('',3,(#28407,#28408,#28409,#28410,#28411,
#28412,#28413,#28414,#28415,#28416,#28417,#28418,#28419,#28420,#28421,#28422,
#28423,#28424,#28425,#28426,#28427,#28428,#28429,#28430,#28431,#28432,#28433,
#28434),.UNSPECIFIED.,.F.,.F.,(4,3,3,3,3,3,3,3,3,4),(54.8725568898769,54.8805486387541,
55.3794627172883,55.8783767958224,56.8762049528906,57.8740331099589,58.8718612670272,
59.8696894240955,60.8675175811637,61.1557421970565),.UNSPECIFIED.);
#4689=B_SPLINE_CURVE_WITH_KNOTS('',3,(#28439,#28440,#28441,#28442,#28443,
#28444,#28445,#28446,#28447,#28448,#28449,#28450,#28451,#28452,#28453,#28454,
#28455,#28456,#28457,#28458,#28459,#28460,#28461,#28462,#28463),
 .UNSPECIFIED.,.F.,.F.,(4,3,3,3,3,3,3,3,4),(-70.4117642649766,-69.5488437297034,
-68.6859231944302,-67.823002659157,-66.9600821238839,-66.0971615886107,
-65.2342410533375,-64.3713205180643,-64.128578957797),.UNSPECIFIED.);
#4690=B_SPLINE_CURVE_WITH_KNOTS('',3,(#28464,#28465,#28466,#28467,#28468,
#28469,#28470,#28471,#28472,#28473,#28474,#28475,#28476,#28477,#28478,#28479,
#28480,#28481,#28482,#28483,#28484,#28485,#28486,#28487,#28488),
 .UNSPECIFIED.,.F.,.F.,(4,3,3,3,3,3,3,3,4),(61.1557421970565,62.0186627323297,
62.8815832676029,63.7445038028761,64.6074243381492,65.4703448734224,66.3332654086956,
67.1961859439688,67.4389275042361),.UNSPECIFIED.);
#4691=B_SPLINE_CURVE_WITH_KNOTS('',3,(#28493,#28494,#28495,#28496,#28497,
#28498,#28499,#28500,#28501,#28502,#28503,#28504,#28505,#28506,#28507,#28508,
#28509,#28510,#28511,#28512,#28513,#28514,#28515,#28516,#28517,#28518,#28519,
#28520),.UNSPECIFIED.,.F.,.F.,(4,3,3,3,3,3,3,3,3,4),(-76.6949495721561,
-76.3338540157217,-75.8349399371876,-75.3360258586534,-74.8371117801193,
-73.8392836230511,-72.8414554659828,-71.8436273089145,-70.8457991518463,
-70.4117642649766),.UNSPECIFIED.);
#4692=B_SPLINE_CURVE_WITH_KNOTS('',3,(#28521,#28522,#28523,#28524,#28525,
#28526,#28527,#28528,#28529,#28530,#28531,#28532,#28533,#28534,#28535,#28536,
#28537,#28538,#28539,#28540,#28541,#28542,#28543,#28544,#28545,#28546,#28547,
#28548),.UNSPECIFIED.,.F.,.F.,(4,3,3,3,3,3,3,3,3,4),(67.4389275042361,67.8523146806415,
68.3512287591757,68.8501428377098,69.3490569162439,69.847970994778,70.8457991518463,
71.8436273089145,72.8414554659828,73.7221128114157),.UNSPECIFIED.);
#4693=B_SPLINE_CURVE_WITH_KNOTS('',3,(#28553,#28554,#28555,#28556,#28557,
#28558,#28559,#28560,#28561,#28562,#28563,#28564,#28565,#28566,#28567,#28568,
#28569,#28570,#28571,#28572,#28573,#28574,#28575,#28576,#28577),
 .UNSPECIFIED.,.F.,.F.,(4,3,3,3,3,3,3,3,4),(-82.9781348793357,-82.1152143440626,
-81.2522938087894,-80.3893732735162,-79.526452738243,-78.6635322029699,
-77.8006116676967,-76.9376911324235,-76.6949495721561),.UNSPECIFIED.);
#4694=B_SPLINE_CURVE_WITH_KNOTS('',3,(#28578,#28579,#28580,#28581,#28582,
#28583,#28584,#28585,#28586,#28587,#28588,#28589,#28590,#28591,#28592,#28593,
#28594,#28595,#28596,#28597,#28598,#28599,#28600,#28601,#28602,#28603,#28604,
#28605,#28606,#28607,#28608),.UNSPECIFIED.,.F.,.F.,(4,3,3,3,3,3,3,3,3,3,
4),(73.7221128114157,73.839283623051,74.8371117801193,75.3360258586534,
75.8349399371876,76.3338540157217,76.8327680942558,77.8305962513241,78.8284244083924,
79.8262525654606,80.0052981185953),.UNSPECIFIED.);
#4695=B_SPLINE_CURVE_WITH_KNOTS('',3,(#28613,#28614,#28615,#28616,#28617,
#28618,#28619,#28620,#28621,#28622,#28623,#28624,#28625,#28626,#28627,#28628,
#28629,#28630,#28631,#28632,#28633,#28634,#28635,#28636,#28637),
 .UNSPECIFIED.,.F.,.F.,(4,3,3,3,3,3,3,3,4),(-89.2613201865154,-88.8067059790749,
-87.8088778220067,-86.8110496649384,-85.8132215078701,-84.8153933508019,
-83.8175651937336,-83.3186511151995,-82.9781348793357),.UNSPECIFIED.);
#4696=B_SPLINE_CURVE_WITH_KNOTS('',3,(#28638,#28639,#28640,#28641,#28642,
#28643,#28644,#28645,#28646,#28647,#28648,#28649,#28650,#28651,#28652,#28653,
#28654,#28655,#28656,#28657,#28658,#28659,#28660,#28661,#28662,#28663,#28664,
#28665),.UNSPECIFIED.,.F.,.F.,(4,3,3,3,3,3,3,3,3,4),(80.0052981185953,80.8240807225289,
81.8219088795971,82.3208229581313,82.8197370366654,83.3186511151995,83.8175651937337,
84.8153933508019,85.8132215078702,86.2884834257749),.UNSPECIFIED.);
#4697=B_SPLINE_CURVE_WITH_KNOTS('',3,(#28670,#28671,#28672,#28673,#28674,
#28675,#28676,#28677,#28678,#28679,#28680,#28681,#28682,#28683,#28684,#28685,
#28686,#28687,#28688,#28689,#28690,#28691,#28692,#28693,#28694),
 .UNSPECIFIED.,.F.,.F.,(4,3,3,3,3,3,3,3,4),(-95.544505493695,-94.6815849584218,
-93.8186644231486,-92.9557438878754,-92.0928233526023,-91.2299028173291,
-90.3669822820559,-89.5040617467827,-89.2613201865154),.UNSPECIFIED.);
#4698=B_SPLINE_CURVE_WITH_KNOTS('',3,(#28695,#28696,#28697,#28698,#28699,
#28700,#28701,#28702,#28703,#28704,#28705,#28706,#28707,#28708,#28709,#28710,
#28711,#28712,#28713,#28714,#28715,#28716,#28717,#28718,#28719,#28720,#28721,
#28722),.UNSPECIFIED.,.F.,.F.,(4,3,3,3,3,3,3,3,3,4),(86.2884834257749,86.8110496649385,
87.8088778220067,88.8067059790749,89.3056200576091,89.8045341361432,90.3034482146773,
90.8023622932114,91.8001904502797,92.5716687329545),.UNSPECIFIED.);
#4699=B_SPLINE_CURVE_WITH_KNOTS('',3,(#28727,#28728,#28729,#28730,#28731,
#28732,#28733,#28734,#28735,#28736,#28737,#28738,#28739,#28740,#28741,#28742,
#28743,#28744,#28745,#28746,#28747,#28748,#28749,#28750,#28751,#28752,#28753,
#28754,#28755,#28756,#28757),.UNSPECIFIED.,.F.,.F.,(4,3,3,3,3,3,3,3,3,3,
4),(-101.827690800875,-101.778472020962,-100.780643863894,-99.7828157068258,
-98.7849875497575,-97.7871593926892,-97.2882453141551,-96.789331235621,
-96.2904171570868,-95.7915030785527,-95.544505493695),.UNSPECIFIED.);
#4700=B_SPLINE_CURVE_WITH_KNOTS('',3,(#28758,#28759,#28760,#28761,#28762,
#28763,#28764,#28765,#28766,#28767,#28768,#28769,#28770,#28771,#28772,#28773,
#28774,#28775,#28776,#28777,#28778,#28779,#28780,#28781,#28782,#28783,#28784,
#28785,#28786,#28787,#28788),.UNSPECIFIED.,.F.,.F.,(4,3,3,3,3,3,3,3,3,3,
4),(92.5716687329545,92.798018607348,93.7958467644162,94.7936749214845,
95.7915030785527,96.2904171570868,96.7893312356209,97.2882453141551,97.7871593926892,
98.7849875497574,98.8548540401341),.UNSPECIFIED.);
#4701=B_SPLINE_CURVE_WITH_KNOTS('',3,(#28793,#28794,#28795,#28796,#28797,
#28798,#28799,#28800,#28801,#28802,#28803,#28804,#28805,#28806,#28807,#28808,
#28809,#28810,#28811,#28812,#28813,#28814,#28815,#28816,#28817,#28818,#28819,
#28820),.UNSPECIFIED.,.F.,.F.,(4,3,3,3,3,3,3,3,3,4),(-108.110876108054,
-107.765440963372,-106.767612806304,-105.769784649235,-104.771956492167,
-104.273042413633,-103.774128335099,-103.275214256565,-102.776300178031,
-101.827690800875),.UNSPECIFIED.);
#4702=B_SPLINE_CURVE_WITH_KNOTS('',3,(#28821,#28822,#28823,#28824,#28825,
#28826,#28827,#28828,#28829,#28830,#28831,#28832,#28833,#28834,#28835,#28836,
#28837,#28838,#28839,#28840,#28841,#28842,#28843,#28844,#28845,#28846,#28847,
#28848),.UNSPECIFIED.,.F.,.F.,(4,3,3,3,3,3,3,3,3,4),(98.8548540401341,99.7828157068257,
100.780643863894,101.778472020962,102.776300178031,103.275214256565,103.774128335099,
104.273042413633,104.771956492167,105.138039347314),.UNSPECIFIED.);
#4703=B_SPLINE_CURVE_WITH_KNOTS('',3,(#28853,#28854,#28855,#28856,#28857,
#28858,#28859,#28860,#28861,#28862,#28863,#28864,#28865,#28866,#28867,#28868,
#28869,#28870,#28871,#28872,#28873,#28874,#28875,#28876,#28877,#28878,#28879,
#28880),.UNSPECIFIED.,.F.,.F.,(4,3,3,3,3,3,3,3,3,4),(-114.394061415234,
-113.752409905781,-112.754581748713,-111.756753591645,-111.257839513111,
-110.758925434577,-110.260011356042,-109.761097277508,-108.76326912044,
-108.110876108054),.UNSPECIFIED.);
#4704=B_SPLINE_CURVE_WITH_KNOTS('',3,(#28881,#28882,#28883,#28884,#28885,
#28886,#28887,#28888,#28889,#28890,#28891,#28892,#28893,#28894,#28895,#28896,
#28897,#28898,#28899,#28900,#28901,#28902,#28903,#28904,#28905),
 .UNSPECIFIED.,.F.,.F.,(4,3,3,3,3,3,3,3,4),(105.138039347314,106.000959882587,
106.86388041786,107.726800953133,108.589721488406,109.45264202368,110.315562558953,
111.178483094226,111.421224654493),.UNSPECIFIED.);
#4705=B_SPLINE_CURVE_WITH_KNOTS('',3,(#28910,#28911,#28912,#28913,#28914,
#28915,#28916,#28917,#28918,#28919,#28920,#28921,#28922,#28923,#28924,#28925,
#28926,#28927,#28928,#28929,#28930,#28931,#28932,#28933,#28934,#28935,#28936,
#28937),.UNSPECIFIED.,.F.,.F.,(4,3,3,3,3,3,3,3,3,4),(-120.677246722413,
-119.739378848191,-118.741550691123,-118.242636612589,-117.743722534054,
-117.24480845552,-116.745894376986,-115.748066219918,-114.75023806285,-114.394061415234),
 .UNSPECIFIED.);
#4706=B_SPLINE_CURVE_WITH_KNOTS('',3,(#28938,#28939,#28940,#28941,#28942,
#28943,#28944,#28945,#28946,#28947,#28948,#28949,#28950,#28951,#28952,#28953,
#28954,#28955,#28956,#28957,#28958,#28959,#28960,#28961,#28962),
 .UNSPECIFIED.,.F.,.F.,(4,3,3,3,3,3,3,3,4),(111.421224654493,111.756753591645,
112.754581748713,113.752409905781,114.75023806285,115.748066219918,116.745894376986,
117.24480845552,117.704409961673),.UNSPECIFIED.);
#4707=B_SPLINE_CURVE_WITH_KNOTS('',3,(#28967,#28968,#28969,#28970,#28971,
#28972,#28973,#28974,#28975,#28976,#28977,#28978,#28979,#28980,#28981,#28982,
#28983,#28984,#28985,#28986,#28987,#28988,#28989,#28990,#28991,#28992,#28993,
#28994,#28995,#28996,#28997),.UNSPECIFIED.,.F.,.F.,(4,3,3,3,3,3,3,3,3,3,
4),(-126.960432029593,-126.724175947669,-125.7263477906,-125.227433712066,
-124.728519633532,-124.229605554998,-123.730691476464,-122.732863319396,
-121.735035162327,-120.737207005259,-120.677246722413),.UNSPECIFIED.);
#4708=B_SPLINE_CURVE_WITH_KNOTS('',3,(#28998,#28999,#29000,#29001,#29002,
#29003,#29004,#29005,#29006,#29007,#29008,#29009,#29010,#29011,#29012,#29013,
#29014,#29015,#29016,#29017,#29018,#29019,#29020,#29021,#29022,#29023,#29024,
#29025),.UNSPECIFIED.,.F.,.F.,(4,3,3,3,3,3,3,3,3,4),(117.704409961673,117.743722534054,
118.242636612588,118.741550691123,119.739378848191,120.737207005259,121.735035162327,
122.732863319396,123.730691476464,123.987595268852),.UNSPECIFIED.);
#4709=B_SPLINE_CURVE_WITH_KNOTS('',3,(#29030,#29031,#29032,#29033,#29034,
#29035,#29036,#29037,#29038,#29039,#29040,#29041,#29042,#29043,#29044,#29045,
#29046,#29047,#29048,#29049,#29050,#29051,#29052,#29053,#29054),
 .UNSPECIFIED.,.F.,.F.,(4,3,3,3,3,3,3,3,4),(-133.243617336773,-132.380696801499,
-131.517776266226,-130.654855730953,-129.79193519568,-128.929014660407,
-128.066094125133,-127.20317358986,-126.960432029593),.UNSPECIFIED.);
#4710=B_SPLINE_CURVE_WITH_KNOTS('',3,(#29055,#29056,#29057,#29058,#29059,
#29060,#29061,#29062,#29063,#29064,#29065,#29066,#29067,#29068,#29069,#29070,
#29071,#29072,#29073,#29074,#29075,#29076,#29077,#29078,#29079),
 .UNSPECIFIED.,.F.,.F.,(4,3,3,3,3,3,3,3,4),(123.987595268852,124.850515804126,
125.713436339399,126.576356874672,127.439277409945,128.302197945218,129.165118480492,
130.028039015765,130.270780576032),.UNSPECIFIED.);
#4711=B_SPLINE_CURVE_WITH_KNOTS('',3,(#29084,#29085,#29086,#29087,#29088,
#29089,#29090,#29091,#29092,#29093,#29094,#29095,#29096,#29097,#29098,#29099,
#29100,#29101,#29102,#29103,#29104,#29105,#29106,#29107,#29108),
 .UNSPECIFIED.,.F.,.F.,(4,3,3,3,3,3,3,3,4),(-139.526802643952,-138.663882108679,
-137.800961573406,-136.938041038132,-136.075120502859,-135.212199967586,
-134.349279432313,-133.48635889704,-133.243617336773),.UNSPECIFIED.);
#4712=B_SPLINE_CURVE_WITH_KNOTS('',3,(#29109,#29110,#29111,#29112,#29113,
#29114,#29115,#29116,#29117,#29118,#29119,#29120,#29121,#29122,#29123,#29124,
#29125,#29126,#29127,#29128,#29129,#29130,#29131,#29132,#29133,#29134,#29135,
#29136),.UNSPECIFIED.,.F.,.F.,(4,3,3,3,3,3,3,3,3,4),(130.270780576032,130.715488575942,
131.214402654476,131.71331673301,132.212230811544,132.711144890078,133.708973047147,
134.706801204215,135.704629361283,136.553965883212),.UNSPECIFIED.);
#4713=B_SPLINE_CURVE_WITH_KNOTS('',3,(#29141,#29142,#29143,#29144,#29145,
#29146,#29147,#29148,#29149,#29150,#29151,#29152,#29153,#29154,#29155,#29156,
#29157,#29158,#29159,#29160,#29161,#29162,#29163,#29164,#29165),
 .UNSPECIFIED.,.F.,.F.,(4,3,3,3,3,3,3,3,4),(-145.809987951132,-144.947067415858,
-144.084146880585,-143.221226345312,-142.358305810039,-141.495385274766,
-140.632464739492,-139.769544204219,-139.526802643952),.UNSPECIFIED.);
#4714=B_SPLINE_CURVE_WITH_KNOTS('',3,(#29166,#29167,#29168,#29169,#29170,
#29171,#29172,#29173,#29174,#29175,#29176,#29177,#29178,#29179,#29180,#29181,
#29182,#29183,#29184,#29185,#29186,#29187,#29188,#29189,#29190,#29191,#29192,
#29193,#29194,#29195,#29196),.UNSPECIFIED.,.F.,.F.,(4,3,3,3,3,3,3,3,3,3,
4),(136.553965883212,136.702457518351,137.70028567542,138.199199753954,
138.698113832488,139.197027911022,139.695941989556,140.693770146624,141.691598303693,
142.689426460761,142.837151190391),.UNSPECIFIED.);
#4715=B_SPLINE_CURVE_WITH_KNOTS('',3,(#29201,#29202,#29203,#29204,#29205,
#29206,#29207,#29208,#29209,#29210,#29211,#29212,#29213,#29214,#29215,#29216,
#29217,#29218,#29219,#29220,#29221,#29222,#29223,#29224,#29225),
 .UNSPECIFIED.,.F.,.F.,(4,3,3,3,3,3,3,3,4),(-152.093173258311,-151.669879874375,
-150.672051717307,-149.674223560239,-148.67639540317,-147.678567246102,
-146.680739089034,-146.1818250105,-145.809987951132),.UNSPECIFIED.);
#4716=B_SPLINE_CURVE_WITH_KNOTS('',3,(#29226,#29227,#29228,#29229,#29230,
#29231,#29232,#29233,#29234,#29235,#29236,#29237,#29238,#29239,#29240,#29241,
#29242,#29243,#29244,#29245,#29246,#29247,#29248,#29249,#29250,#29251,#29252,
#29253),.UNSPECIFIED.,.F.,.F.,(4,3,3,3,3,3,3,3,3,4),(142.837151190391,143.687254617829,
144.685082774897,145.183996853431,145.682910931966,146.1818250105,146.680739089034,
147.678567246102,148.67639540317,149.120336497571),.UNSPECIFIED.);
#4717=B_SPLINE_CURVE_WITH_KNOTS('',3,(#29258,#29259,#29260,#29261,#29262,
#29263,#29264,#29265,#29266,#29267,#29268,#29269,#29270,#29271,#29272,#29273,
#29274,#29275,#29276,#29277,#29278,#29279,#29280,#29281,#29282),
 .UNSPECIFIED.,.F.,.F.,(4,3,3,3,3,3,3,3,4),(-158.376358565491,-157.513438030218,
-156.650517494944,-155.787596959671,-154.924676424398,-154.061755889125,
-153.198835353852,-152.335914818578,-152.093173258311),.UNSPECIFIED.);
#4718=B_SPLINE_CURVE_WITH_KNOTS('',3,(#29283,#29284,#29285,#29286,#29287,
#29288,#29289,#29290,#29291,#29292,#29293,#29294,#29295,#29296,#29297,#29298,
#29299,#29300,#29301,#29302,#29303,#29304,#29305,#29306,#29307,#29308,#29309,
#29310),.UNSPECIFIED.,.F.,.F.,(4,3,3,3,3,3,3,3,3,4),(149.120336497571,149.674223560239,
150.672051717307,151.669879874375,152.168793952909,152.667708031443,153.166622109978,
153.665536188512,154.66336434558,155.40352180475),.UNSPECIFIED.);
#4719=B_SPLINE_CURVE_WITH_KNOTS('',3,(#29315,#29316,#29317,#29318,#29319,
#29320,#29321,#29322,#29323,#29324,#29325,#29326,#29327,#29328,#29329,#29330,
#29331,#29332,#29333,#29334,#29335,#29336,#29337,#29338,#29339,#29340,#29341,
#29342,#29343,#29344,#29345),.UNSPECIFIED.,.F.,.F.,(4,3,3,3,3,3,3,3,3,3,
4),(-164.65954387267,-164.641645916262,-163.643817759194,-162.645989602126,
-161.648161445058,-160.650333287989,-160.151419209455,-159.652505130921,
-159.153591052387,-158.654676973853,-158.376358565491),.UNSPECIFIED.);
#4720=B_SPLINE_CURVE_WITH_KNOTS('',3,(#29346,#29347,#29348,#29349,#29350,
#29351,#29352,#29353,#29354,#29355,#29356,#29357,#29358,#29359,#29360,#29361,
#29362,#29363,#29364,#29365,#29366,#29367,#29368,#29369,#29370,#29371,#29372,
#29373,#29374,#29375,#29376),.UNSPECIFIED.,.F.,.F.,(4,3,3,3,3,3,3,3,3,3,
4),(155.40352180475,155.661192502648,156.659020659716,157.656848816785,
158.654676973853,159.153591052387,159.652505130921,160.151419209455,160.650333287989,
161.648161445058,161.68670711193),.UNSPECIFIED.);
#4721=B_SPLINE_CURVE_WITH_KNOTS('',3,(#29381,#29382,#29383,#29384,#29385,
#29386,#29387,#29388,#29389,#29390,#29391,#29392,#29393,#29394,#29395,#29396,
#29397,#29398,#29399,#29400,#29401,#29402,#29403,#29404,#29405,#29406,#29407,
#29408),.UNSPECIFIED.,.F.,.F.,(4,3,3,3,3,3,3,3,3,4),(-170.94272917985,-170.628614858672,
-169.630786701604,-168.632958544536,-167.635130387467,-167.136216308933,
-166.637302230399,-166.138388151865,-165.639474073331,-164.65954387267),
 .UNSPECIFIED.);
#4722=B_SPLINE_CURVE_WITH_KNOTS('',3,(#29409,#29410,#29411,#29412,#29413,
#29414,#29415,#29416,#29417,#29418,#29419,#29420,#29421,#29422,#29423,#29424,
#29425,#29426,#29427,#29428,#29429,#29430,#29431,#29432,#29433,#29434,#29435,
#29436),.UNSPECIFIED.,.F.,.F.,(4,3,3,3,3,3,3,3,3,4),(161.68670711193,162.645989602126,
163.643817759194,164.641645916263,165.639474073331,166.138388151865,166.637302230399,
167.136216308933,167.635130387467,167.969892419109),.UNSPECIFIED.);
#4723=B_SPLINE_CURVE_WITH_KNOTS('',3,(#29441,#29442,#29443,#29444,#29445,
#29446,#29447,#29448,#29449,#29450,#29451,#29452,#29453,#29454,#29455,#29456,
#29457,#29458,#29459,#29460,#29461,#29462,#29463,#29464,#29465,#29466,#29467,
#29468),.UNSPECIFIED.,.F.,.F.,(4,3,3,3,3,3,3,3,3,4),(-177.225914487029,
-176.615583801082,-175.617755644013,-174.619927486945,-174.121013408411,
-173.622099329877,-173.123185251343,-172.624271172809,-171.62644301574,
-170.94272917985),.UNSPECIFIED.);
#4724=B_SPLINE_CURVE_WITH_KNOTS('',3,(#29469,#29470,#29471,#29472,#29473,
#29474,#29475,#29476,#29477,#29478,#29479,#29480,#29481,#29482,#29483,#29484,
#29485,#29486,#29487,#29488,#29489,#29490,#29491,#29492,#29493),
 .UNSPECIFIED.,.F.,.F.,(4,3,3,3,3,3,3,3,4),(167.969892419109,168.832812954383,
169.695733489656,170.558654024929,171.421574560202,172.284495095475,173.147415630748,
174.010336166022,174.253077726289),.UNSPECIFIED.);
#4725=B_SPLINE_CURVE_WITH_KNOTS('',3,(#29498,#29499,#29500,#29501,#29502,
#29503,#29504,#29505,#29506,#29507,#29508,#29509,#29510,#29511,#29512,#29513,
#29514,#29515,#29516,#29517,#29518,#29519,#29520,#29521,#29522,#29523,#29524,
#29525),.UNSPECIFIED.,.F.,.F.,(4,3,3,3,3,3,3,3,3,4),(-183.509099794209,
-182.602552743491,-181.604724586423,-181.105810507889,-180.606896429355,
-180.10798235082,-179.609068272286,-178.611240115218,-177.61341195815,-177.225914487029),
 .UNSPECIFIED.);
#4726=B_SPLINE_CURVE_WITH_KNOTS('',3,(#29526,#29527,#29528,#29529,#29530,
#29531,#29532,#29533,#29534,#29535,#29536,#29537,#29538,#29539,#29540,#29541,
#29542,#29543,#29544,#29545,#29546,#29547,#29548,#29549,#29550),
 .UNSPECIFIED.,.F.,.F.,(4,3,3,3,3,3,3,3,4),(174.253077726289,174.619927486945,
175.617755644013,176.615583801082,177.61341195815,178.611240115218,179.609068272286,
180.107982350821,180.536263033469),.UNSPECIFIED.);
#4727=B_SPLINE_CURVE_WITH_KNOTS('',3,(#29555,#29556,#29557,#29558,#29559,
#29560,#29561,#29562,#29563,#29564,#29565,#29566,#29567,#29568,#29569,#29570,
#29571,#29572,#29573,#29574,#29575,#29576,#29577,#29578,#29579,#29580,#29581,
#29582,#29583,#29584,#29585),.UNSPECIFIED.,.F.,.F.,(4,3,3,3,3,3,3,3,3,3,
4),(-189.792285101389,-189.587349842969,-188.589521685901,-188.090607607367,
-187.591693528832,-187.092779450298,-186.593865371764,-185.596037214696,
-184.598209057628,-183.600380900559,-183.509099794209),.UNSPECIFIED.);
#4728=B_SPLINE_CURVE_WITH_KNOTS('',3,(#29586,#29587,#29588,#29589,#29590,
#29591,#29592,#29593,#29594,#29595,#29596,#29597,#29598,#29599,#29600,#29601,
#29602,#29603,#29604,#29605,#29606,#29607,#29608,#29609,#29610),
 .UNSPECIFIED.,.F.,.F.,(4,3,3,3,3,3,3,3,4),(180.536263033469,181.399183568742,
182.262104104015,183.125024639288,183.987945174561,184.850865709834,185.713786245107,
186.576706780381,186.819448340648),.UNSPECIFIED.);
#4729=B_SPLINE_CURVE_WITH_KNOTS('',3,(#29615,#29616,#29617,#29618,#29619,
#29620,#29621,#29622,#29623,#29624,#29625,#29626,#29627,#29628,#29629,#29630,
#29631,#29632,#29633,#29634,#29635,#29636,#29637,#29638,#29639),
 .UNSPECIFIED.,.F.,.F.,(4,3,3,3,3,3,3,3,4),(-196.075470408568,-195.212549873295,
-194.349629338022,-193.486708802749,-192.623788267476,-191.760867732202,
-190.897947196929,-190.035026661656,-189.792285101389),.UNSPECIFIED.);
#4730=B_SPLINE_CURVE_WITH_KNOTS('',3,(#29640,#29641,#29642,#29643,#29644,
#29645,#29646,#29647,#29648,#29649,#29650,#29651,#29652,#29653,#29654,#29655,
#29656,#29657,#29658,#29659,#29660,#29661,#29662,#29663,#29664),
 .UNSPECIFIED.,.F.,.F.,(4,3,3,3,3,3,3,3,4),(186.819448340648,187.682368875921,
188.545289411195,189.408209946468,190.271130481741,191.134051017014,191.996971552287,
192.859892087561,193.102633647828),.UNSPECIFIED.);
#4731=B_SPLINE_CURVE_WITH_KNOTS('',3,(#29669,#29670,#29671,#29672,#29673,
#29674,#29675,#29676,#29677,#29678,#29679,#29680,#29681,#29682,#29683,#29684,
#29685,#29686,#29687,#29688,#29689,#29690,#29691,#29692,#29693),
 .UNSPECIFIED.,.F.,.F.,(4,3,3,3,3,3,3,3,4),(-202.358655715748,-202.060201806322,
-201.561287727788,-200.56345957072,-199.565631413651,-198.567803256583,
-197.569975099515,-196.572146942447,-196.075470408568),.UNSPECIFIED.);
#4732=B_SPLINE_CURVE_WITH_KNOTS('',3,(#29694,#29695,#29696,#29697,#29698,
#29699,#29700,#29701,#29702,#29703,#29704,#29705,#29706,#29707,#29708,#29709,
#29710,#29711,#29712,#29713,#29714,#29715,#29716,#29717,#29718,#29719,#29720,
#29721),.UNSPECIFIED.,.F.,.F.,(4,3,3,3,3,3,3,3,3,4),(193.102633647828,193.578662471242,
194.077576549776,194.57649062831,195.075404706844,195.574318785378,196.572146942447,
197.569975099515,198.567803256583,199.385818955007),.UNSPECIFIED.);
#4733=B_SPLINE_CURVE_WITH_KNOTS('',3,(#29726,#29727,#29728,#29729,#29730,
#29731,#29732,#29733,#29734,#29735,#29736,#29737,#29738,#29739,#29740,#29741,
#29742,#29743,#29744,#29745,#29746,#29747,#29748,#29749,#29750,#29751,#29752,
#29753,#29754,#29755,#29756),.UNSPECIFIED.,.F.,.F.,(4,3,3,3,3,3,3,3,3,3,
4),(-208.641841022927,-208.546084827266,-207.548256670198,-207.049342591663,
-206.550428513129,-206.051514434595,-205.552600356061,-204.554772198993,
-203.556944041925,-202.559115884856,-202.358655715748),.UNSPECIFIED.);
#4734=B_SPLINE_CURVE_WITH_KNOTS('',3,(#29757,#29758,#29759,#29760,#29761,
#29762,#29763,#29764,#29765,#29766,#29767,#29768,#29769,#29770,#29771,#29772,
#29773,#29774,#29775,#29776,#29777,#29778,#29779,#29780,#29781,#29782,#29783,
#29784),.UNSPECIFIED.,.F.,.F.,(4,3,3,3,3,3,3,3,3,4),(199.385818955007,199.565631413652,
200.56345957072,201.561287727788,202.060201806322,202.559115884856,203.556944041925,
204.554772198993,205.552600356061,205.669004262187),.UNSPECIFIED.);
#4735=B_SPLINE_CURVE_WITH_KNOTS('',3,(#29789,#29790,#29791,#29792,#29793,
#29794,#29795,#29796,#29797,#29798,#29799,#29800,#29801,#29802,#29803,#29804,
#29805,#29806,#29807,#29808,#29809,#29810,#29811,#29812,#29813,#29814,#29815,
#29816),.UNSPECIFIED.,.F.,.F.,(4,3,3,3,3,3,3,3,3,4),(-214.925026330107,
-214.533053769675,-214.034139691141,-213.535225612607,-213.036311534073,
-212.537397455539,-211.539569298471,-210.541741141402,-209.543912984334,
-208.641841022927),.UNSPECIFIED.);
#4736=B_SPLINE_CURVE_WITH_KNOTS('',3,(#29817,#29818,#29819,#29820,#29821,
#29822,#29823,#29824,#29825,#29826,#29827,#29828,#29829,#29830,#29831,#29832,
#29833,#29834,#29835,#29836,#29837,#29838,#29839,#29840,#29841,#29842,#29843,
#29844),.UNSPECIFIED.,.F.,.F.,(4,3,3,3,3,3,3,3,3,4),(205.669004262187,206.051514434595,
206.550428513129,207.049342591663,207.548256670198,208.546084827266,209.543912984334,
210.541741141402,211.539569298471,211.952189569366),.UNSPECIFIED.);
#4737=B_SPLINE_CURVE_WITH_KNOTS('',3,(#29849,#29850,#29851,#29852,#29853,
#29854,#29855,#29856,#29857,#29858,#29859,#29860,#29861,#29862,#29863,#29864,
#29865,#29866,#29867,#29868,#29869,#29870,#29871,#29872,#29873),
 .UNSPECIFIED.,.F.,.F.,(4,3,3,3,3,3,3,3,4),(-221.208211637286,-220.345291102013,
-219.48237056674,-218.619450031467,-217.756529496194,-216.893608960921,
-216.030688425647,-215.167767890374,-214.925026330107),.UNSPECIFIED.);
#4738=B_SPLINE_CURVE_WITH_KNOTS('',3,(#29874,#29875,#29876,#29877,#29878,
#29879,#29880,#29881,#29882,#29883,#29884,#29885,#29886,#29887,#29888,#29889,
#29890,#29891,#29892,#29893,#29894,#29895,#29896,#29897,#29898),
 .UNSPECIFIED.,.F.,.F.,(4,3,3,3,3,3,3,3,4),(211.952189569366,212.81511010464,
213.678030639913,214.540951175186,215.403871710459,216.266792245732,217.129712781005,
217.992633316278,218.235374876546),.UNSPECIFIED.);
#4739=B_SPLINE_CURVE_WITH_KNOTS('',3,(#29903,#29904,#29905,#29906,#29907,
#29908,#29909,#29910,#29911,#29912,#29913,#29914,#29915,#29916,#29917,#29918,
#29919,#29920,#29921,#29922,#29923,#29924,#29925,#29926,#29927),
 .UNSPECIFIED.,.F.,.F.,(4,3,3,3,3,3,3,3,4),(-227.491396944466,-227.005905733029,
-226.506991654494,-225.509163497426,-224.511335340358,-223.51350718329,
-222.515679026221,-221.517850869153,-221.208211637286),.UNSPECIFIED.);
#4740=B_SPLINE_CURVE_WITH_KNOTS('',3,(#29928,#29929,#29930,#29931,#29932,
#29933,#29934,#29935,#29936,#29937,#29938,#29939,#29940,#29941,#29942,#29943,
#29944,#29945,#29946,#29947,#29948,#29949,#29950,#29951,#29952,#29953,#29954,
#29955,#29956,#29957,#29958),.UNSPECIFIED.,.F.,.F.,(4,3,3,3,3,3,3,3,3,3,
4),(218.235374876546,218.524366397948,219.522194555017,220.021108633551,
220.520022712085,221.018936790619,221.517850869153,222.515679026221,223.51350718329,
224.511335340358,224.518560183726),.UNSPECIFIED.);
#4741=B_SPLINE_CURVE_WITH_KNOTS('',3,(#29963,#29964,#29965,#29966,#29967,
#29968,#29969,#29970,#29971,#29972,#29973,#29974,#29975,#29976,#29977,#29978,
#29979,#29980,#29981,#29982,#29983,#29984,#29985,#29986,#29987,#29988,#29989,
#29990),.UNSPECIFIED.,.F.,.F.,(4,3,3,3,3,3,3,3,3,4),(-233.774582251646,
-233.491788753972,-232.493960596904,-231.496132439836,-230.498304282767,
-229.500476125699,-228.502647968631,-228.003733890097,-227.504819811563,
-227.491396944466),.UNSPECIFIED.);
#4742=B_SPLINE_CURVE_WITH_KNOTS('',3,(#29991,#29992,#29993,#29994,#29995,
#29996,#29997,#29998,#29999,#30000,#30001,#30002,#30003,#30004,#30005,#30006,
#30007,#30008,#30009,#30010,#30011,#30012,#30013,#30014,#30015,#30016,#30017,
#30018),.UNSPECIFIED.,.F.,.F.,(4,3,3,3,3,3,3,3,3,4),(224.518560183726,225.509163497426,
226.506991654494,227.005905733029,227.504819811563,228.003733890097,228.502647968631,
229.500476125699,230.498304282767,230.801745490905),.UNSPECIFIED.);
#4743=B_SPLINE_CURVE_WITH_KNOTS('',3,(#30023,#30024,#30025,#30026,#30027,
#30028,#30029,#30030,#30031,#30032,#30033,#30034,#30035,#30036,#30037,#30038,
#30039,#30040,#30041,#30042,#30043,#30044,#30045,#30046,#30047),
 .UNSPECIFIED.,.F.,.F.,(4,3,3,3,3,3,3,3,4),(-240.057767558825,-239.194847023552,
-238.331926488279,-237.469005953006,-236.606085417733,-235.74316488246,
-234.880244347186,-234.017323811913,-233.774582251646),.UNSPECIFIED.);
#4744=B_SPLINE_CURVE_WITH_KNOTS('',3,(#30048,#30049,#30050,#30051,#30052,
#30053,#30054,#30055,#30056,#30057,#30058,#30059,#30060,#30061,#30062,#30063,
#30064,#30065,#30066,#30067,#30068,#30069,#30070,#30071,#30072,#30073,#30074,
#30075),.UNSPECIFIED.,.F.,.F.,(4,3,3,3,3,3,3,3,3,4),(230.801745490905,231.496132439836,
232.493960596904,233.491788753972,233.990702832506,234.489616911041,234.988530989575,
235.487445068109,236.485273225177,237.084930798085),.UNSPECIFIED.);
#4745=B_SPLINE_CURVE_WITH_KNOTS('',3,(#30080,#30081,#30082,#30083,#30084,
#30085,#30086,#30087,#30088,#30089,#30090,#30091,#30092,#30093,#30094,#30095,
#30096,#30097,#30098,#30099,#30100,#30101,#30102,#30103,#30104,#30105,#30106,
#30107),.UNSPECIFIED.,.F.,.F.,(4,3,3,3,3,3,3,3,3,4),(-246.340952866005,
-245.465726638791,-244.467898481723,-243.470070324655,-242.472242167587,
-241.973328089052,-241.474414010518,-240.975499931984,-240.47658585345,
-240.057767558825),.UNSPECIFIED.);
#4746=B_SPLINE_CURVE_WITH_KNOTS('',3,(#30108,#30109,#30110,#30111,#30112,
#30113,#30114,#30115,#30116,#30117,#30118,#30119,#30120,#30121,#30122,#30123,
#30124,#30125,#30126,#30127,#30128,#30129,#30130,#30131,#30132,#30133,#30134,
#30135),.UNSPECIFIED.,.F.,.F.,(4,3,3,3,3,3,3,3,3,4),(237.084930798085,237.483101382245,
238.480929539314,239.478757696382,240.47658585345,240.975499931984,241.474414010518,
241.973328089053,242.472242167587,243.368116105264),.UNSPECIFIED.);
#4747=B_SPLINE_CURVE_WITH_KNOTS('',3,(#30140,#30141,#30142,#30143,#30144,
#30145,#30146,#30147,#30148,#30149,#30150,#30151,#30152,#30153,#30154,#30155,
#30156,#30157,#30158,#30159,#30160,#30161,#30162,#30163,#30164,#30165,#30166,
#30167,#30168,#30169,#30170),.UNSPECIFIED.,.F.,.F.,(4,3,3,3,3,3,3,3,3,3,
4),(-252.624138173184,-252.450523738269,-251.452695581201,-250.454867424133,
-249.457039267064,-248.95812518853,-248.459211109996,-247.960297031462,
-247.461382952928,-246.46355479586,-246.340952866005),.UNSPECIFIED.);
#4748=B_SPLINE_CURVE_WITH_KNOTS('',3,(#30171,#30172,#30173,#30174,#30175,
#30176,#30177,#30178,#30179,#30180,#30181,#30182,#30183,#30184,#30185,#30186,
#30187,#30188,#30189,#30190,#30191,#30192,#30193,#30194,#30195),
 .UNSPECIFIED.,.F.,.F.,(4,3,3,3,3,3,3,3,4),(243.368116105264,244.231036640537,
245.093957175811,245.956877711084,246.819798246357,247.68271878163,248.545639316903,
249.408559852176,249.651301412444),.UNSPECIFIED.);
#4749=B_SPLINE_CURVE_WITH_KNOTS('',3,(#30200,#30201,#30202,#30203,#30204,
#30205,#30206,#30207,#30208,#30209,#30210,#30211,#30212,#30213,#30214,#30215,
#30216,#30217,#30218,#30219,#30220,#30221,#30222,#30223,#30224,#30225,#30226,
#30227),.UNSPECIFIED.,.F.,.F.,(4,3,3,3,3,3,3,3,3,4),(-258.907323480364,
-258.437492680679,-257.43966452361,-256.441836366542,-255.942922288008,
-255.444008209474,-254.94509413094,-254.446180052406,-253.448351895337,
-252.624138173184),.UNSPECIFIED.);
#4750=B_SPLINE_CURVE_WITH_KNOTS('',3,(#30228,#30229,#30230,#30231,#30232,
#30233,#30234,#30235,#30236,#30237,#30238,#30239,#30240,#30241,#30242,#30243,
#30244,#30245,#30246,#30247,#30248,#30249,#30250,#30251,#30252),
 .UNSPECIFIED.,.F.,.F.,(4,3,3,3,3,3,3,3,4),(249.651301412444,250.454867424133,
251.452695581201,252.450523738269,253.448351895337,254.446180052406,254.94509413094,
255.444008209474,255.934486719623),.UNSPECIFIED.);
#4751=B_SPLINE_CURVE_WITH_KNOTS('',3,(#30257,#30258,#30259,#30260,#30261,
#30262,#30263,#30264,#30265,#30266,#30267,#30268,#30269,#30270,#30271,#30272,
#30273,#30274,#30275,#30276,#30277,#30278,#30279,#30280,#30281,#30282,#30283,
#30284),.UNSPECIFIED.,.F.,.F.,(4,3,3,3,3,3,3,3,3,4),(-265.190508787543,
-264.424461623088,-263.42663346602,-262.927719387486,-262.428805308952,
-261.929891230418,-261.430977151883,-260.433148994815,-259.435320837747,
-258.907323480364),.UNSPECIFIED.);
#4752=B_SPLINE_CURVE_WITH_KNOTS('',3,(#30285,#30286,#30287,#30288,#30289,
#30290,#30291,#30292,#30293,#30294,#30295,#30296,#30297,#30298,#30299,#30300,
#30301,#30302,#30303,#30304,#30305,#30306,#30307,#30308,#30309,#30310,#30311,
#30312),.UNSPECIFIED.,.F.,.F.,(4,3,3,3,3,3,3,3,3,4),(255.934486719623,255.942922288008,
256.441836366542,257.43966452361,258.437492680679,259.435320837747,260.433148994815,
261.430977151884,261.929891230418,262.217672026803),.UNSPECIFIED.);
#4753=B_SPLINE_CURVE_WITH_KNOTS('',3,(#30317,#30318,#30319,#30320,#30321,
#30322,#30323,#30324,#30325,#30326,#30327,#30328,#30329,#30330,#30331,#30332,
#30333,#30334,#30335,#30336,#30337,#30338,#30339,#30340,#30341,#30342,#30343,
#30344,#30345,#30346,#30347),.UNSPECIFIED.,.F.,.F.,(4,3,3,3,3,3,3,3,3,3,
4),(-271.473694094723,-271.409258722566,-270.411430565498,-269.912516486964,
-269.413602408429,-268.914688329895,-268.415774251361,-267.417946094293,
-266.420117937225,-265.422289780157,-265.190508787543),.UNSPECIFIED.);
#4754=B_SPLINE_CURVE_WITH_KNOTS('',3,(#30348,#30349,#30350,#30351,#30352,
#30353,#30354,#30355,#30356,#30357,#30358,#30359,#30360,#30361,#30362,#30363,
#30364,#30365,#30366,#30367,#30368,#30369,#30370,#30371,#30372),
 .UNSPECIFIED.,.F.,.F.,(4,3,3,3,3,3,3,3,4),(262.217672026803,263.080592562076,
263.943513097349,264.806433632622,265.669354167895,266.532274703169,267.395195238442,
268.258115773715,268.500857333982),.UNSPECIFIED.);
#4755=B_SPLINE_CURVE_WITH_KNOTS('',3,(#30377,#30378,#30379,#30380,#30381,
#30382,#30383,#30384,#30385,#30386,#30387,#30388,#30389,#30390,#30391,#30392,
#30393,#30394,#30395,#30396,#30397,#30398,#30399,#30400,#30401,#30402,#30403,
#30404),.UNSPECIFIED.,.F.,.F.,(4,3,3,3,3,3,3,3,3,4),(-277.756879401903,
-277.396227664976,-276.897313586441,-276.398399507907,-275.899485429373,
-275.400571350839,-274.402743193771,-273.404915036703,-272.407086879634,
-271.473694094723),.UNSPECIFIED.);
#4756=B_SPLINE_CURVE_WITH_KNOTS('',3,(#30405,#30406,#30407,#30408,#30409,
#30410,#30411,#30412,#30413,#30414,#30415,#30416,#30417,#30418,#30419,#30420,
#30421,#30422,#30423,#30424,#30425,#30426,#30427,#30428,#30429,#30430,#30431,
#30432),.UNSPECIFIED.,.F.,.F.,(4,3,3,3,3,3,3,3,3,4),(268.500857333982,268.914688329895,
269.41360240843,269.912516486964,270.411430565498,271.409258722566,272.407086879634,
273.404915036703,274.402743193771,274.784042641162),.UNSPECIFIED.);
#4757=B_SPLINE_CURVE_WITH_KNOTS('',3,(#30437,#30438,#30439,#30440,#30441,
#30442,#30443,#30444,#30445,#30446,#30447,#30448,#30449,#30450,#30451,#30452,
#30453,#30454,#30455,#30456,#30457,#30458,#30459,#30460,#30461),
 .UNSPECIFIED.,.F.,.F.,(4,3,3,3,3,3,3,3,4),(-284.040064709082,-283.177144173809,
-282.314223638536,-281.451303103262,-280.588382567989,-279.725462032716,
-278.862541497443,-277.99962096217,-277.756879401903),.UNSPECIFIED.);
#4758=B_SPLINE_CURVE_WITH_KNOTS('',3,(#30462,#30463,#30464,#30465,#30466,
#30467,#30468,#30469,#30470,#30471,#30472,#30473,#30474,#30475,#30476,#30477,
#30478,#30479,#30480,#30481,#30482,#30483,#30484,#30485,#30486),
 .UNSPECIFIED.,.F.,.F.,(4,3,3,3,3,3,3,3,4),(274.784042641162,275.646963176435,
276.509883711708,277.372804246982,278.235724782255,279.098645317528,279.961565852801,
280.824486388074,281.067227948342),.UNSPECIFIED.);
#4759=B_SPLINE_CURVE_WITH_KNOTS('',3,(#30491,#30492,#30493,#30494,#30495,
#30496,#30497,#30498,#30499,#30500,#30501,#30502,#30503,#30504,#30505,#30506,
#30507,#30508,#30509,#30510,#30511,#30512,#30513,#30514,#30515),
 .UNSPECIFIED.,.F.,.F.,(4,3,3,3,3,3,3,3,4),(-290.323250016262,-289.869079628329,
-289.370165549795,-288.372337392726,-287.374509235658,-286.37668107859,
-285.378852921522,-284.381024764453,-284.040064709082),.UNSPECIFIED.);
#4760=B_SPLINE_CURVE_WITH_KNOTS('',3,(#30516,#30517,#30518,#30519,#30520,
#30521,#30522,#30523,#30524,#30525,#30526,#30527,#30528,#30529,#30530,#30531,
#30532,#30533,#30534,#30535,#30536,#30537,#30538,#30539,#30540,#30541,#30542,
#30543),.UNSPECIFIED.,.F.,.F.,(4,3,3,3,3,3,3,3,3,4),(281.067227948342,281.387540293249,
282.385368450317,282.884282528851,283.383196607385,283.882110685919,284.381024764453,
285.378852921522,286.37668107859,287.350413255521),.UNSPECIFIED.);
#4761=B_SPLINE_CURVE_WITH_KNOTS('',3,(#30548,#30549,#30550,#30551,#30552,
#30553,#30554,#30555,#30556,#30557,#30558,#30559,#30560,#30561,#30562,#30563,
#30564,#30565,#30566,#30567,#30568,#30569,#30570,#30571,#30572,#30573,#30574,
#30575),.UNSPECIFIED.,.F.,.F.,(4,3,3,3,3,3,3,3,3,4),(-296.606435323441,
-296.354962649272,-295.357134492204,-294.359306335136,-293.361478178068,
-292.363650020999,-291.365821863931,-290.866907785397,-290.367993706863,
-290.323250016262),.UNSPECIFIED.);
#4762=B_SPLINE_CURVE_WITH_KNOTS('',3,(#30576,#30577,#30578,#30579,#30580,
#30581,#30582,#30583,#30584,#30585,#30586,#30587,#30588,#30589,#30590,#30591,
#30592,#30593,#30594,#30595,#30596,#30597,#30598,#30599,#30600,#30601,#30602,
#30603,#30604,#30605,#30606),.UNSPECIFIED.,.F.,.F.,(4,3,3,3,3,3,3,3,3,3,
4),(287.350413255521,287.374509235658,288.372337392726,289.370165549795,
289.869079628329,290.367993706863,290.866907785397,291.365821863931,292.363650021,
293.361478178068,293.633598562701),.UNSPECIFIED.);
#4763=B_SPLINE_CURVE_WITH_KNOTS('',3,(#30611,#30612,#30613,#30614,#30615,
#30616,#30617,#30618,#30619,#30620,#30621,#30622,#30623,#30624,#30625,#30626,
#30627,#30628,#30629,#30630,#30631,#30632,#30633,#30634,#30635),
 .UNSPECIFIED.,.F.,.F.,(4,3,3,3,3,3,3,3,4),(-302.889620630621,-302.026700095348,
-301.163779560074,-300.300859024801,-299.437938489528,-298.575017954255,
-297.712097418982,-296.849176883708,-296.606435323441),.UNSPECIFIED.);
#4764=B_SPLINE_CURVE_WITH_KNOTS('',3,(#30636,#30637,#30638,#30639,#30640,
#30641,#30642,#30643,#30644,#30645,#30646,#30647,#30648,#30649,#30650,#30651,
#30652,#30653,#30654,#30655,#30656,#30657,#30658,#30659,#30660,#30661,#30662,
#30663),.UNSPECIFIED.,.F.,.F.,(4,3,3,3,3,3,3,3,3,4),(293.633598562701,294.359306335136,
295.357134492204,296.354962649273,296.853876727807,297.352790806341,297.851704884875,
298.350618963409,299.348447120477,299.91678386988),.UNSPECIFIED.);
#4765=B_SPLINE_CURVE_WITH_KNOTS('',3,(#30668,#30669,#30670,#30671,#30672,
#30673,#30674,#30675,#30676,#30677,#30678,#30679,#30680,#30681,#30682,#30683,
#30684,#30685,#30686,#30687,#30688,#30689,#30690,#30691,#30692,#30693,#30694,
#30695),.UNSPECIFIED.,.F.,.F.,(4,3,3,3,3,3,3,3,3,4),(-309.1728059378,-308.328900534092,
-307.331072377023,-306.333244219955,-305.335416062887,-304.836501984353,
-304.337587905819,-303.838673827284,-303.33975974875,-302.889620630621),
 .UNSPECIFIED.);
#4766=B_SPLINE_CURVE_WITH_KNOTS('',3,(#30696,#30697,#30698,#30699,#30700,
#30701,#30702,#30703,#30704,#30705,#30706,#30707,#30708,#30709,#30710,#30711,
#30712,#30713,#30714,#30715,#30716,#30717,#30718,#30719,#30720,#30721,#30722,
#30723),.UNSPECIFIED.,.F.,.F.,(4,3,3,3,3,3,3,3,3,4),(299.91678386988,300.346275277546,
301.344103434614,302.341931591682,303.33975974875,303.838673827284,304.337587905819,
304.836501984353,305.335416062887,306.19996917706),.UNSPECIFIED.);
#4767=B_SPLINE_CURVE_WITH_KNOTS('',3,(#30728,#30729,#30730,#30731,#30732,
#30733,#30734,#30735,#30736,#30737,#30738,#30739,#30740,#30741,#30742,#30743,
#30744,#30745,#30746,#30747,#30748,#30749,#30750,#30751,#30752,#30753,#30754,
#30755,#30756,#30757,#30758),.UNSPECIFIED.,.F.,.F.,(4,3,3,3,3,3,3,3,3,3,
4),(-315.45599124498,-315.313697633569,-314.315869476501,-313.318041319433,
-312.320213162365,-311.82129908383,-311.322385005296,-310.823470926762,
-310.324556848228,-309.32672869116,-309.1728059378),.UNSPECIFIED.);
#4768=B_SPLINE_CURVE_WITH_KNOTS('',3,(#30759,#30760,#30761,#30762,#30763,
#30764,#30765,#30766,#30767,#30768,#30769,#30770,#30771,#30772,#30773,#30774,
#30775,#30776,#30777,#30778,#30779,#30780,#30781,#30782,#30783),
 .UNSPECIFIED.,.F.,.F.,(4,3,3,3,3,3,3,3,4),(306.19996917706,307.062889712333,
307.925810247606,308.788730782879,309.651651318153,310.514571853426,311.377492388699,
312.240412923972,312.483154484239),.UNSPECIFIED.);
#4769=B_SPLINE_CURVE_WITH_KNOTS('',3,(#30788,#30789,#30790,#30791,#30792,
#30793,#30794,#30795,#30796,#30797,#30798,#30799,#30800,#30801,#30802,#30803,
#30804,#30805,#30806,#30807,#30808,#30809,#30810,#30811,#30812,#30813,#30814,
#30815),.UNSPECIFIED.,.F.,.F.,(4,3,3,3,3,3,3,3,3,4),(-321.739176552159,
-321.300666575979,-320.302838418911,-319.305010261842,-318.806096183308,
-318.307182104774,-317.80826802624,-317.309353947706,-316.311525790638,
-315.45599124498),.UNSPECIFIED.);
#4770=B_SPLINE_CURVE_WITH_KNOTS('',3,(#30816,#30817,#30818,#30819,#30820,
#30821,#30822,#30823,#30824,#30825,#30826,#30827,#30828,#30829,#30830,#30831,
#30832,#30833,#30834,#30835,#30836,#30837,#30838,#30839,#30840),
 .UNSPECIFIED.,.F.,.F.,(4,3,3,3,3,3,3,3,4),(312.483154484239,313.318041319433,
314.315869476501,315.313697633569,316.311525790638,317.309353947706,317.80826802624,
318.307182104774,318.766339791419),.UNSPECIFIED.);
#4771=B_SPLINE_CURVE_WITH_KNOTS('',3,(#30845,#30846,#30847,#30848,#30849,
#30850,#30851,#30852,#30853,#30854,#30855,#30856,#30857,#30858,#30859,#30860,
#30861,#30862,#30863,#30864,#30865,#30866,#30867,#30868,#30869,#30870,#30871,
#30872),.UNSPECIFIED.,.F.,.F.,(4,3,3,3,3,3,3,3,3,4),(-328.022361859339,
-327.287635518388,-326.28980736132,-325.790893282786,-325.291979204252,
-324.793065125718,-324.294151047184,-323.296322890115,-322.298494733047,
-321.739176552159),.UNSPECIFIED.);
#4772=B_SPLINE_CURVE_WITH_KNOTS('',3,(#30873,#30874,#30875,#30876,#30877,
#30878,#30879,#30880,#30881,#30882,#30883,#30884,#30885,#30886,#30887,#30888,
#30889,#30890,#30891,#30892,#30893,#30894,#30895,#30896,#30897,#30898,#30899,
#30900),.UNSPECIFIED.,.F.,.F.,(4,3,3,3,3,3,3,3,3,4),(318.766339791419,318.806096183308,
319.305010261842,320.302838418911,321.300666575979,322.298494733047,323.296322890116,
324.294151047184,324.793065125718,325.049525098599),.UNSPECIFIED.);
#4773=B_SPLINE_CURVE_WITH_KNOTS('',3,(#30905,#30906,#30907,#30908,#30909,
#30910,#30911,#30912,#30913,#30914,#30915,#30916,#30917,#30918,#30919,#30920,
#30921,#30922,#30923,#30924,#30925,#30926,#30927,#30928,#30929,#30930,#30931,
#30932,#30933,#30934,#30935),.UNSPECIFIED.,.F.,.F.,(4,3,3,3,3,3,3,3,3,3,
4),(-334.305547166519,-334.272432617866,-333.274604460798,-332.775690382264,
-332.27677630373,-331.777862225196,-331.278948146661,-330.281119989593,
-329.283291832525,-328.285463675457,-328.022361859339),.UNSPECIFIED.);
#4774=B_SPLINE_CURVE_WITH_KNOTS('',3,(#30936,#30937,#30938,#30939,#30940,
#30941,#30942,#30943,#30944,#30945,#30946,#30947,#30948,#30949,#30950,#30951,
#30952,#30953,#30954,#30955,#30956,#30957,#30958,#30959,#30960,#30961,#30962,
#30963),.UNSPECIFIED.,.F.,.F.,(4,3,3,3,3,3,3,3,3,4),(325.049525098599,325.291979204252,
325.790893282786,326.28980736132,327.287635518389,328.285463675457,329.283291832525,
330.281119989593,331.278948146662,331.332710405778),.UNSPECIFIED.);
#4775=B_SPLINE_CURVE_WITH_KNOTS('',3,(#30968,#30969,#30970,#30971,#30972,
#30973,#30974,#30975,#30976,#30977,#30978,#30979,#30980,#30981,#30982,#30983,
#30984,#30985,#30986,#30987,#30988,#30989,#30990,#30991,#30992,#30993,#30994,
#30995),.UNSPECIFIED.,.F.,.F.,(4,3,3,3,3,3,3,3,3,4),(-340.588732473698,
-340.259401560276,-339.760487481742,-339.261573403207,-338.762659324673,
-338.263745246139,-337.265917089071,-336.268088932003,-335.270260774934,
-334.305547166519),.UNSPECIFIED.);
#4776=B_SPLINE_CURVE_WITH_KNOTS('',3,(#30996,#30997,#30998,#30999,#31000,
#31001,#31002,#31003,#31004,#31005,#31006,#31007,#31008,#31009,#31010,#31011,
#31012,#31013,#31014,#31015,#31016,#31017,#31018,#31019,#31020,#31021,#31022,
#31023),.UNSPECIFIED.,.F.,.F.,(4,3,3,3,3,3,3,3,3,4),(331.332710405778,331.777862225196,
332.27677630373,332.775690382264,333.274604460798,334.272432617866,335.270260774935,
336.268088932003,337.265917089071,337.615895712958),.UNSPECIFIED.);
#4777=B_SPLINE_CURVE_WITH_KNOTS('',3,(#31028,#31029,#31030,#31031,#31032,
#31033,#31034,#31035,#31036,#31037,#31038,#31039,#31040,#31041,#31042,#31043,
#31044,#31045,#31046,#31047,#31048,#31049,#31050,#31051,#31052),
 .UNSPECIFIED.,.F.,.F.,(4,3,3,3,3,3,3,3,4),(-346.871917780878,-346.008997245604,
-345.146076710331,-344.283156175058,-343.420235639785,-342.557315104512,
-341.694394569239,-340.831474033966,-340.588732473698),.UNSPECIFIED.);
#4778=B_SPLINE_CURVE_WITH_KNOTS('',3,(#31053,#31054,#31055,#31056,#31057,
#31058,#31059,#31060,#31061,#31062,#31063,#31064,#31065,#31066,#31067,#31068,
#31069,#31070,#31071,#31072,#31073,#31074,#31075,#31076,#31077),
 .UNSPECIFIED.,.F.,.F.,(4,3,3,3,3,3,3,3,4),(337.615895712958,338.478816248231,
339.341736783504,340.204657318777,341.06757785405,341.930498389324,342.793418924597,
343.65633945987,343.899081020137),.UNSPECIFIED.);
#4779=B_SPLINE_CURVE_WITH_KNOTS('',3,(#31082,#31083,#31084,#31085,#31086,
#31087,#31088,#31089,#31090,#31091,#31092,#31093,#31094,#31095,#31096,#31097,
#31098,#31099,#31100,#31101,#31102,#31103,#31104,#31105,#31106),
 .UNSPECIFIED.,.F.,.F.,(4,3,3,3,3,3,3,3,4),(-353.155103088057,-352.732253523629,
-352.233339445095,-351.235511288027,-350.237683130958,-349.23985497389,
-348.242026816822,-347.244198659754,-346.871917780878),.UNSPECIFIED.);
#4780=B_SPLINE_CURVE_WITH_KNOTS('',3,(#31107,#31108,#31109,#31110,#31111,
#31112,#31113,#31114,#31115,#31116,#31117,#31118,#31119,#31120,#31121,#31122,
#31123,#31124,#31125,#31126,#31127,#31128,#31129,#31130,#31131,#31132,#31133,
#31134),.UNSPECIFIED.,.F.,.F.,(4,3,3,3,3,3,3,3,3,4),(343.899081020137,344.250714188549,
345.248542345617,345.747456424151,346.246370502685,346.74528458122,347.244198659754,
348.242026816822,349.23985497389,350.182266327317),.UNSPECIFIED.);
#4781=B_SPLINE_CURVE_WITH_KNOTS('',3,(#31139,#31140,#31141,#31142,#31143,
#31144,#31145,#31146,#31147,#31148,#31149,#31150,#31151,#31152,#31153,#31154,
#31155,#31156,#31157,#31158,#31159,#31160,#31161,#31162,#31163),
 .UNSPECIFIED.,.F.,.F.,(4,3,3,3,3,3,3,3,4),(-359.438288395237,-358.575367859964,
-357.712447324691,-356.849526789417,-355.986606254144,-355.123685718871,
-354.260765183598,-353.397844648325,-353.155103088057),.UNSPECIFIED.);
#4782=B_SPLINE_CURVE_WITH_KNOTS('',3,(#31164,#31165,#31166,#31167,#31168,
#31169,#31170,#31171,#31172,#31173,#31174,#31175,#31176,#31177,#31178,#31179,
#31180,#31181,#31182,#31183,#31184,#31185,#31186,#31187,#31188,#31189,#31190,
#31191,#31192,#31193,#31194),.UNSPECIFIED.,.F.,.F.,(4,3,3,3,3,3,3,3,3,3,
4),(350.182266327317,350.237683130958,351.235511288027,352.233339445095,
352.732253523629,353.231167602163,353.730081680697,354.228995759231,355.2268239163,
356.224652073368,356.465451634496),.UNSPECIFIED.);
#4783=B_SPLINE_CURVE_WITH_KNOTS('',3,(#31199,#31200,#31201,#31202,#31203,
#31204,#31205,#31206,#31207,#31208,#31209,#31210,#31211,#31212,#31213,#31214,
#31215,#31216,#31217,#31218,#31219,#31220,#31221,#31222,#31223),
 .UNSPECIFIED.,.F.,.F.,(4,3,3,3,3,3,3,3,4),(-365.721473702416,-364.858553167143,
-363.99563263187,-363.132712096597,-362.269791561324,-361.406871026051,
-360.543950490778,-359.681029955504,-359.438288395237),.UNSPECIFIED.);
#4784=B_SPLINE_CURVE_WITH_KNOTS('',3,(#31224,#31225,#31226,#31227,#31228,
#31229,#31230,#31231,#31232,#31233,#31234,#31235,#31236,#31237,#31238,#31239,
#31240,#31241,#31242,#31243,#31244,#31245,#31246,#31247,#31248,#31249,#31250,
#31251),.UNSPECIFIED.,.F.,.F.,(4,3,3,3,3,3,3,3,3,4),(356.465451634496,357.222480230436,
358.220308387505,359.218136544573,359.717050623107,360.215964701641,360.714878780175,
361.213792858709,362.211621015778,362.748636941676),.UNSPECIFIED.);
#4785=B_SPLINE_CURVE_WITH_KNOTS('',3,(#31256,#31257,#31258,#31259,#31260,
#31261,#31262,#31263,#31264,#31265,#31266,#31267,#31268,#31269,#31270,#31271,
#31272,#31273,#31274,#31275,#31276,#31277,#31278,#31279,#31280),
 .UNSPECIFIED.,.F.,.F.,(4,3,3,3,3,3,3,3,4),(-372.004659009596,-371.141738474323,
-370.278817939049,-369.415897403776,-368.552976868503,-367.69005633323,
-366.827135797956,-365.964215262683,-365.721473702416),.UNSPECIFIED.);
#4786=B_SPLINE_CURVE_WITH_KNOTS('',3,(#31281,#31282,#31283,#31284,#31285,
#31286,#31287,#31288,#31289,#31290,#31291,#31292,#31293,#31294,#31295,#31296,
#31297,#31298,#31299,#31300,#31301,#31302,#31303,#31304,#31305,#31306,#31307,
#31308),.UNSPECIFIED.,.F.,.F.,(4,3,3,3,3,3,3,3,3,4),(362.748636941676,363.209449172846,
364.207277329914,365.205105486982,366.202933644051,366.701847722585,367.200761801119,
367.699675879653,368.198589958187,369.031822248856),.UNSPECIFIED.);
#4787=B_SPLINE_CURVE_WITH_KNOTS('',3,(#31313,#31314,#31315,#31316,#31317,
#31318,#31319,#31320,#31321,#31322,#31323,#31324,#31325,#31326,#31327,#31328,
#31329,#31330,#31331,#31332,#31333,#31334,#31335,#31336,#31337,#31338,#31339,
#31340,#31341,#31342,#31343),.UNSPECIFIED.,.F.,.F.,(4,3,3,3,3,3,3,3,3,3,
4),(-378.287844316776,-378.17687152887,-377.179043371801,-376.181215214733,
-375.183387057665,-374.684472979131,-374.185558900597,-373.686644822062,
-373.187730743528,-372.18990258646,-372.004659009596),.UNSPECIFIED.);
#4788=B_SPLINE_CURVE_WITH_KNOTS('',3,(#31344,#31345,#31346,#31347,#31348,
#31349,#31350,#31351,#31352,#31353,#31354,#31355,#31356,#31357,#31358,#31359,
#31360,#31361,#31362,#31363,#31364,#31365,#31366,#31367,#31368),
 .UNSPECIFIED.,.F.,.F.,(4,3,3,3,3,3,3,3,4),(369.031822248856,369.894742784129,
370.757663319402,371.620583854675,372.483504389948,373.346424925221,374.209345460494,
375.072265995767,375.315007556035),.UNSPECIFIED.);
#4789=B_SPLINE_CURVE_WITH_KNOTS('',3,(#31373,#31374,#31375,#31376,#31377,
#31378,#31379,#31380,#31381,#31382,#31383,#31384,#31385,#31386,#31387,#31388,
#31389,#31390,#31391,#31392,#31393,#31394,#31395,#31396,#31397,#31398,#31399,
#31400),.UNSPECIFIED.,.F.,.F.,(4,3,3,3,3,3,3,3,3,4),(-384.571029623955,
-384.163840471279,-383.166012314211,-382.168184157143,-381.669270078608,
-381.170356000074,-380.67144192154,-380.172527843006,-379.174699685938,
-378.287844316776),.UNSPECIFIED.);
#4790=B_SPLINE_CURVE_WITH_KNOTS('',3,(#31401,#31402,#31403,#31404,#31405,
#31406,#31407,#31408,#31409,#31410,#31411,#31412,#31413,#31414,#31415,#31416,
#31417,#31418,#31419,#31420,#31421,#31422,#31423,#31424,#31425),
 .UNSPECIFIED.,.F.,.F.,(4,3,3,3,3,3,3,3,4),(375.315007556035,376.181215214733,
377.179043371801,378.17687152887,379.174699685938,380.172527843006,380.67144192154,
381.170356000074,381.598192863215),.UNSPECIFIED.);
#4791=B_SPLINE_CURVE_WITH_KNOTS('',3,(#31430,#31431,#31432,#31433,#31434,
#31435,#31436,#31437,#31438,#31439,#31440,#31441,#31442,#31443,#31444,#31445,
#31446,#31447,#31448,#31449,#31450,#31451,#31452,#31453,#31454,#31455,#31456,
#31457),.UNSPECIFIED.,.F.,.F.,(4,3,3,3,3,3,3,3,3,4),(-390.854214931135,
-390.150809413689,-389.15298125662,-388.654067178086,-388.155153099552,
-387.656239021018,-387.157324942484,-386.159496785416,-385.161668628347,
-384.571029623955),.UNSPECIFIED.);
#4792=B_SPLINE_CURVE_WITH_KNOTS('',3,(#31458,#31459,#31460,#31461,#31462,
#31463,#31464,#31465,#31466,#31467,#31468,#31469,#31470,#31471,#31472,#31473,
#31474,#31475,#31476,#31477,#31478,#31479,#31480,#31481,#31482,#31483,#31484,
#31485),.UNSPECIFIED.,.F.,.F.,(4,3,3,3,3,3,3,3,3,4),(381.598192863215,381.669270078609,
382.168184157143,383.166012314211,384.163840471279,385.161668628347,386.159496785416,
387.157324942484,387.656239021018,387.881378170394),.UNSPECIFIED.);
#4793=B_SPLINE_CURVE_WITH_KNOTS('',3,(#31491,#31492,#31493,#31494,#31495,
#31496,#31497,#31498,#31499,#31500,#31501,#31502,#31503),.UNSPECIFIED.,
 .F.,.F.,(4,3,3,3,4),(-3.8100000088729,-3.48648673068836,-2.98841719773288,
-2.4903476647774,-2.07135887395545),.UNSPECIFIED.);
#4794=B_SPLINE_CURVE_WITH_KNOTS('',3,(#31511,#31512,#31513,#31514,#31515,
#31516,#31517),.UNSPECIFIED.,.F.,.F.,(4,3,4),(0.,0.498069532955476,0.837163248131365),
 .UNSPECIFIED.);
#4795=B_SPLINE_CURVE_WITH_KNOTS('',3,(#31522,#31523,#31524,#31525,#31526,
#31527,#31528,#31529,#31530,#31531,#31532,#31533,#31534,#31535,#31536,#31537,
#31538,#31539,#31540,#31541,#31542,#31543,#31544,#31545,#31546,#31547,#31548,
#31549,#31550,#31551,#31552,#31553,#31554,#31555,#31556,#31557,#31558,#31559,
#31560,#31561,#31562,#31563,#31564),.UNSPECIFIED.,.F.,.F.,(4,3,3,3,3,3,
3,3,3,3,3,3,3,3,4),(-10.0931853160525,-9.96139065910959,-9.46332112615411,
-8.96525159319863,-8.46718206024316,-7.96911252728767,-7.47104299433219,
-6.97297346137671,-6.47490392842124,-5.97683439546575,-5.47876486251027,
-4.9806953295548,-4.48262579659932,-3.98455626364384,-3.8100000088729),
 .UNSPECIFIED.);
#4796=B_SPLINE_CURVE_WITH_KNOTS('',3,(#31565,#31566,#31567,#31568,#31569,
#31570,#31571,#31572,#31573,#31574,#31575,#31576,#31577,#31578,#31579,#31580,
#31581,#31582,#31583,#31584,#31585,#31586,#31587,#31588,#31589,#31590,#31591,
#31592,#31593,#31594,#31595,#31596,#31597,#31598,#31599,#31600,#31601,#31602,
#31603,#31604,#31605,#31606,#31607),.UNSPECIFIED.,.F.,.F.,(4,3,3,3,3,3,
3,3,3,3,3,3,3,3,4),(0.837163248131365,0.996139065910959,1.49420859886644,
1.99227813182192,2.4903476647774,2.98841719773287,3.48648673068835,3.98455626364383,
4.48262579659931,4.98069532955479,5.47876486251027,5.97683439546575,6.47490392842123,
6.97297346137671,7.12034855531095),.UNSPECIFIED.);
#4797=B_SPLINE_CURVE_WITH_KNOTS('',3,(#31612,#31613,#31614,#31615,#31616,
#31617,#31618,#31619,#31620,#31621,#31622,#31623,#31624,#31625,#31626,#31627,
#31628,#31629,#31630,#31631,#31632,#31633,#31634,#31635,#31636,#31637,#31638,
#31639,#31640,#31641,#31642,#31643,#31644,#31645,#31646,#31647,#31648,#31649,
#31650,#31651),.UNSPECIFIED.,.F.,.F.,(4,3,3,3,3,3,3,3,3,3,3,3,3,4),(-16.3763706232321,
-15.9382250545753,-15.4401555216199,-14.9420859886644,-14.4440164557089,
-13.9459469227534,-13.4478773897979,-12.9498078568425,-12.451738323887,
-11.9536687909315,-11.455599257976,-10.9575297250205,-10.4594601920651,
-10.0931853160525),.UNSPECIFIED.);
#4798=B_SPLINE_CURVE_WITH_KNOTS('',3,(#31652,#31653,#31654,#31655,#31656,
#31657,#31658,#31659,#31660,#31661,#31662,#31663,#31664,#31665,#31666,#31667,
#31668,#31669,#31670,#31671,#31672,#31673,#31674,#31675,#31676,#31677,#31678,
#31679,#31680,#31681,#31682,#31683,#31684,#31685,#31686,#31687,#31688,#31689,
#31690,#31691),.UNSPECIFIED.,.F.,.F.,(4,3,3,3,3,3,3,3,3,3,3,3,3,4),(7.12034855531095,
7.47104299433219,7.96911252728767,8.46718206024315,8.96525159319863,9.46332112615411,
9.96139065910959,10.4594601920651,10.9575297250206,11.455599257976,11.9536687909315,
12.451738323887,12.9498078568425,13.4035338624905),.UNSPECIFIED.);
#4799=B_SPLINE_CURVE_WITH_KNOTS('',3,(#31696,#31697,#31698,#31699,#31700,
#31701,#31702,#31703,#31704,#31705,#31706,#31707,#31708,#31709,#31710,#31711,
#31712,#31713,#31714,#31715,#31716,#31717,#31718,#31719,#31720,#31721,#31722,
#31723,#31724,#31725,#31726,#31727,#31728,#31729,#31730,#31731,#31732,#31733,
#31734,#31735,#31736,#31737,#31738),.UNSPECIFIED.,.F.,.F.,(4,3,3,3,3,3,
3,3,3,3,3,3,3,3,4),(-22.6595559304117,-22.4131289829966,-21.9150594500411,
-21.4169899170856,-20.9189203841301,-20.4208508511747,-19.9227813182192,
-19.4247117852637,-18.9266422523082,-18.4285727193527,-17.9305031863973,
-17.4324336534418,-16.9343641204863,-16.4362945875308,-16.3763706232321),
 .UNSPECIFIED.);
#4800=B_SPLINE_CURVE_WITH_KNOTS('',3,(#31739,#31740,#31741,#31742,#31743,
#31744,#31745,#31746,#31747,#31748,#31749,#31750,#31751,#31752,#31753,#31754,
#31755,#31756,#31757,#31758,#31759,#31760,#31761,#31762,#31763,#31764,#31765,
#31766,#31767,#31768,#31769,#31770,#31771,#31772,#31773,#31774,#31775,#31776,
#31777,#31778,#31779,#31780,#31781),.UNSPECIFIED.,.F.,.F.,(4,3,3,3,3,3,
3,3,3,3,3,3,3,3,4),(13.4035338624905,13.447877389798,13.9459469227534,14.4440164557089,
14.9420859886644,15.4401555216199,15.9382250545754,16.4362945875308,16.9343641204863,
17.4324336534418,17.9305031863973,18.4285727193527,18.9266422523082,19.4247117852637,
19.6867191696701),.UNSPECIFIED.);
#4801=B_SPLINE_CURVE_WITH_KNOTS('',3,(#31786,#31787,#31788,#31789,#31790,
#31791,#31792,#31793,#31794,#31795,#31796,#31797,#31798,#31799,#31800,#31801,
#31802,#31803,#31804,#31805,#31806,#31807,#31808,#31809,#31810,#31811,#31812,
#31813,#31814,#31815,#31816,#31817,#31818,#31819,#31820,#31821,#31822,#31823,
#31824,#31825,#31826,#31827,#31828),.UNSPECIFIED.,.F.,.F.,(4,3,3,3,3,3,
3,3,3,3,3,3,3,3,4),(-28.9427412375912,-28.8880329114178,-28.3899633784623,
-27.8918938455068,-27.3938243125514,-26.8957547795959,-26.3976852466404,
-25.8996157136849,-25.4015461807295,-24.903476647774,-24.4054071148185,
-23.907337581863,-23.4092680489075,-22.9111985159521,-22.6595559304117),
 .UNSPECIFIED.);
#4802=B_SPLINE_CURVE_WITH_KNOTS('',3,(#31829,#31830,#31831,#31832,#31833,
#31834,#31835,#31836,#31837,#31838,#31839,#31840,#31841,#31842,#31843,#31844,
#31845,#31846,#31847,#31848,#31849,#31850,#31851,#31852,#31853,#31854,#31855,
#31856,#31857,#31858,#31859,#31860,#31861,#31862,#31863,#31864,#31865,#31866,
#31867,#31868,#31869,#31870,#31871),.UNSPECIFIED.,.F.,.F.,(4,3,3,3,3,3,
3,3,3,3,3,3,3,3,4),(19.6867191696701,19.9227813182192,20.4208508511747,
20.9189203841301,21.4169899170856,21.9150594500411,22.4131289829966,22.9111985159521,
23.4092680489075,23.907337581863,24.4054071148185,24.903476647774,25.4015461807295,
25.899615713685,25.9699044768497),.UNSPECIFIED.);
#4803=B_SPLINE_CURVE_WITH_KNOTS('',3,(#31876,#31877,#31878,#31879,#31880,
#31881,#31882,#31883,#31884,#31885,#31886,#31887,#31888,#31889,#31890,#31891,
#31892,#31893,#31894,#31895,#31896,#31897,#31898,#31899,#31900,#31901,#31902,
#31903,#31904,#31905,#31906,#31907,#31908,#31909,#31910,#31911,#31912,#31913,
#31914,#31915),.UNSPECIFIED.,.F.,.F.,(4,3,3,3,3,3,3,3,3,3,3,3,3,4),(-35.2259265447708,
-34.8648673068836,-34.3667977739281,-33.8687282409726,-33.3706587080171,
-32.8725891750617,-32.3745196421062,-31.8764501091507,-31.3783805761952,
-30.8803110432397,-30.3822415102843,-29.8841719773288,-29.3861024443733,
-28.9427412375912),.UNSPECIFIED.);
#4804=B_SPLINE_CURVE_WITH_KNOTS('',3,(#31916,#31917,#31918,#31919,#31920,
#31921,#31922,#31923,#31924,#31925,#31926,#31927,#31928,#31929,#31930,#31931,
#31932,#31933,#31934,#31935,#31936,#31937,#31938,#31939,#31940,#31941,#31942,
#31943,#31944,#31945,#31946,#31947,#31948,#31949,#31950,#31951,#31952,#31953,
#31954,#31955),.UNSPECIFIED.,.F.,.F.,(4,3,3,3,3,3,3,3,3,3,3,3,3,4),(25.9699044768497,
26.3976852466404,26.8957547795959,27.3938243125514,27.8918938455069,28.3899633784623,
28.8880329114178,29.3861024443733,29.8841719773288,30.3822415102843,30.8803110432397,
31.3783805761952,31.8764501091507,32.2530897840293),.UNSPECIFIED.);
#4805=B_SPLINE_CURVE_WITH_KNOTS('',3,(#31960,#31961,#31962,#31963,#31964,
#31965,#31966,#31967,#31968,#31969,#31970,#31971,#31972,#31973,#31974,#31975,
#31976,#31977,#31978,#31979,#31980,#31981,#31982,#31983,#31984,#31985,#31986,
#31987,#31988,#31989,#31990,#31991,#31992,#31993,#31994,#31995,#31996,#31997,
#31998,#31999,#32000,#32001,#32002),.UNSPECIFIED.,.F.,.F.,(4,3,3,3,3,3,
3,3,3,3,3,3,3,3,4),(-41.5091118519504,-41.3397712353048,-40.8417017023493,
-40.3436321693938,-39.8455626364384,-39.3474931034829,-38.8494235705274,
-38.3513540375719,-37.8532845046164,-37.355214971661,-36.8571454387055,
-36.35907590575,-35.8610063727945,-35.362936839839,-35.2259265447708),
 .UNSPECIFIED.);
#4806=B_SPLINE_CURVE_WITH_KNOTS('',3,(#32003,#32004,#32005,#32006,#32007,
#32008,#32009,#32010,#32011,#32012,#32013,#32014,#32015,#32016,#32017,#32018,
#32019,#32020,#32021,#32022,#32023,#32024,#32025,#32026,#32027,#32028,#32029,
#32030,#32031,#32032,#32033,#32034,#32035,#32036,#32037,#32038,#32039,#32040,
#32041,#32042,#32043,#32044,#32045),.UNSPECIFIED.,.F.,.F.,(4,3,3,3,3,3,
3,3,3,3,3,3,3,3,4),(32.2530897840293,32.3745196421062,32.8725891750617,
33.3706587080171,33.8687282409726,34.3667977739281,34.8648673068836,35.3629368398391,
35.8610063727945,36.35907590575,36.8571454387055,37.355214971661,37.8532845046165,
38.3513540375719,38.5362750912089),.UNSPECIFIED.);
#4807=B_SPLINE_CURVE_WITH_KNOTS('',3,(#32050,#32051,#32052,#32053,#32054,
#32055,#32056,#32057,#32058,#32059,#32060,#32061,#32062,#32063,#32064,#32065,
#32066,#32067,#32068,#32069,#32070,#32071,#32072,#32073,#32074,#32075,#32076,
#32077,#32078,#32079,#32080,#32081,#32082,#32083,#32084,#32085,#32086,#32087,
#32088,#32089),.UNSPECIFIED.,.F.,.F.,(4,3,3,3,3,3,3,3,3,3,3,3,3,4),(-47.79229715913,
-47.3166056307706,-46.8185360978151,-46.3204665648596,-45.8223970319041,
-45.3243274989486,-44.8262579659932,-44.3281884330377,-43.8301189000822,
-43.3320493671267,-42.8339798341712,-42.3359103012158,-41.8378407682603,
-41.5091118519504),.UNSPECIFIED.);
#4808=B_SPLINE_CURVE_WITH_KNOTS('',3,(#32090,#32091,#32092,#32093,#32094,
#32095,#32096,#32097,#32098,#32099,#32100,#32101,#32102,#32103,#32104,#32105,
#32106,#32107,#32108,#32109,#32110,#32111,#32112,#32113,#32114,#32115,#32116,
#32117,#32118,#32119,#32120,#32121,#32122,#32123,#32124,#32125,#32126,#32127,
#32128,#32129),.UNSPECIFIED.,.F.,.F.,(4,3,3,3,3,3,3,3,3,3,3,3,3,4),(38.5362750912089,
38.8494235705274,39.3474931034829,39.8455626364384,40.3436321693939,40.8417017023493,
41.3397712353048,41.8378407682603,42.3359103012158,42.8339798341713,43.3320493671267,
43.8301189000822,44.3281884330377,44.8194603983885),.UNSPECIFIED.);
#4809=B_SPLINE_CURVE_WITH_KNOTS('',3,(#32134,#32135,#32136,#32137,#32138,
#32139,#32140,#32141,#32142,#32143,#32144,#32145,#32146,#32147,#32148,#32149,
#32150,#32151,#32152,#32153,#32154,#32155,#32156,#32157,#32158,#32159,#32160,
#32161,#32162,#32163,#32164,#32165,#32166,#32167,#32168,#32169,#32170,#32171,
#32172,#32173,#32174,#32175,#32176),.UNSPECIFIED.,.F.,.F.,(4,3,3,3,3,3,
3,3,3,3,3,3,3,3,4),(-54.0754824663096,-53.7915095591918,-53.2934400262363,
-52.7953704932808,-52.2973009603254,-51.7992314273699,-51.3011618944144,
-50.8030923614589,-50.3050228285034,-49.8069532955479,-49.3088837625925,
-48.810814229637,-48.3127446966815,-47.814675163726,-47.79229715913),
 .UNSPECIFIED.);
#4810=B_SPLINE_CURVE_WITH_KNOTS('',3,(#32177,#32178,#32179,#32180,#32181,
#32182,#32183,#32184,#32185,#32186,#32187,#32188,#32189,#32190,#32191,#32192,
#32193,#32194,#32195,#32196,#32197,#32198,#32199,#32200,#32201,#32202,#32203,
#32204,#32205,#32206,#32207,#32208,#32209,#32210,#32211,#32212,#32213,#32214,
#32215,#32216,#32217,#32218,#32219),.UNSPECIFIED.,.F.,.F.,(4,3,3,3,3,3,
3,3,3,3,3,3,3,3,4),(44.8194603983885,44.8262579659932,45.3243274989487,
45.8223970319041,46.3204665648596,46.8185360978151,47.3166056307706,47.8146751637261,
48.3127446966815,48.810814229637,49.3088837625925,49.806953295548,50.3050228285035,
50.8030923614589,51.1026457055681),.UNSPECIFIED.);
#4811=B_SPLINE_CURVE_WITH_KNOTS('',3,(#32224,#32225,#32226,#32227,#32228,
#32229,#32230,#32231,#32232,#32233,#32234,#32235,#32236,#32237,#32238,#32239,
#32240,#32241,#32242,#32243,#32244,#32245,#32246,#32247,#32248,#32249,#32250,
#32251,#32252,#32253,#32254,#32255,#32256,#32257,#32258,#32259,#32260,#32261,
#32262,#32263,#32264,#32265,#32266),.UNSPECIFIED.,.F.,.F.,(4,3,3,3,3,3,
3,3,3,3,3,3,3,3,4),(-60.3586677734892,-60.266413487613,-59.7683439546575,
-59.2702744217021,-58.7722048887466,-58.2741353557911,-57.7760658228356,
-57.2779962898802,-56.7799267569247,-56.2818572239692,-55.7837876910137,
-55.2857181580582,-54.7876486251028,-54.2895790921473,-54.0754824663096),
 .UNSPECIFIED.);
#4812=B_SPLINE_CURVE_WITH_KNOTS('',3,(#32267,#32268,#32269,#32270,#32271,
#32272,#32273,#32274,#32275,#32276,#32277,#32278,#32279,#32280,#32281,#32282,
#32283,#32284,#32285,#32286,#32287,#32288,#32289,#32290,#32291,#32292,#32293,
#32294,#32295,#32296,#32297,#32298,#32299,#32300,#32301,#32302,#32303,#32304,
#32305,#32306,#32307,#32308,#32309),.UNSPECIFIED.,.F.,.F.,(4,3,3,3,3,3,
3,3,3,3,3,3,3,3,4),(51.1026457055681,51.3011618944144,51.7992314273699,
52.2973009603254,52.7953704932809,53.2934400262363,53.7915095591918,54.2895790921473,
54.7876486251028,55.2857181580583,55.7837876910137,56.2818572239692,56.7799267569247,
57.2779962898802,57.3858310127477),.UNSPECIFIED.);
#4813=B_SPLINE_CURVE_WITH_KNOTS('',3,(#32314,#32315,#32316,#32317,#32318,
#32319,#32320,#32321,#32322,#32323,#32324,#32325,#32326,#32327,#32328,#32329,
#32330,#32331,#32332,#32333,#32334,#32335,#32336,#32337,#32338,#32339,#32340,
#32341,#32342,#32343,#32344,#32345,#32346,#32347,#32348,#32349,#32350,#32351,
#32352,#32353),.UNSPECIFIED.,.F.,.F.,(4,3,3,3,3,3,3,3,3,3,3,3,3,4),(-66.6418530806688,
-66.2432478830788,-65.7451783501233,-65.2471088171678,-64.7490392842123,
-64.2509697512569,-63.7529002183014,-63.2548306853459,-62.7567611523904,
-62.2586916194349,-61.7606220864795,-61.262552553524,-60.7644830205685,
-60.3586677734892),.UNSPECIFIED.);
#4814=B_SPLINE_CURVE_WITH_KNOTS('',3,(#32354,#32355,#32356,#32357,#32358,
#32359,#32360,#32361,#32362,#32363,#32364,#32365,#32366,#32367,#32368,#32369,
#32370,#32371,#32372,#32373,#32374,#32375,#32376,#32377,#32378,#32379,#32380,
#32381,#32382,#32383,#32384,#32385,#32386,#32387,#32388,#32389,#32390,#32391,
#32392,#32393),.UNSPECIFIED.,.F.,.F.,(4,3,3,3,3,3,3,3,3,3,3,3,3,4),(57.3858310127477,
57.7760658228356,58.2741353557911,58.7722048887466,59.2702744217021,59.7683439546576,
60.266413487613,60.7644830205685,61.262552553524,61.7606220864795,62.258691619435,
62.7567611523904,63.2548306853459,63.6690163199273),.UNSPECIFIED.);
#4815=B_SPLINE_CURVE_WITH_KNOTS('',3,(#32398,#32399,#32400,#32401,#32402,
#32403,#32404,#32405,#32406,#32407,#32408,#32409,#32410,#32411,#32412,#32413,
#32414,#32415,#32416,#32417,#32418,#32419,#32420,#32421,#32422,#32423,#32424,
#32425,#32426,#32427,#32428,#32429,#32430,#32431,#32432,#32433,#32434,#32435,
#32436,#32437,#32438,#32439,#32440),.UNSPECIFIED.,.F.,.F.,(4,3,3,3,3,3,
3,3,3,3,3,3,3,3,4),(-72.9250383878484,-72.7181518115,-72.2200822785445,
-71.7220127455891,-71.2239432126336,-70.7258736796781,-70.2278041467226,
-69.7297346137671,-69.2316650808116,-68.7335955478562,-68.2355260149007,
-67.7374564819452,-67.2393869489897,-66.7413174160342,-66.6418530806688),
 .UNSPECIFIED.);
#4816=B_SPLINE_CURVE_WITH_KNOTS('',3,(#32441,#32442,#32443,#32444,#32445,
#32446,#32447,#32448,#32449,#32450,#32451,#32452,#32453,#32454,#32455,#32456,
#32457,#32458,#32459,#32460,#32461,#32462,#32463,#32464,#32465,#32466,#32467,
#32468,#32469,#32470,#32471,#32472,#32473,#32474,#32475,#32476,#32477,#32478,
#32479,#32480,#32481,#32482,#32483),.UNSPECIFIED.,.F.,.F.,(4,3,3,3,3,3,
3,3,3,3,3,3,3,3,4),(63.6690163199273,63.7529002183014,64.2509697512569,
64.7490392842124,65.2471088171678,65.7451783501233,66.2432478830788,66.7413174160343,
67.2393869489897,67.7374564819452,68.2355260149007,68.7335955478562,69.2316650808117,
69.7297346137671,69.9522016271069),.UNSPECIFIED.);
#4817=B_SPLINE_CURVE_WITH_KNOTS('',3,(#32488,#32489,#32490,#32491,#32492,
#32493,#32494,#32495,#32496,#32497,#32498,#32499,#32500,#32501,#32502,#32503,
#32504,#32505,#32506,#32507,#32508,#32509,#32510,#32511,#32512,#32513,#32514,
#32515,#32516,#32517,#32518,#32519,#32520,#32521,#32522,#32523,#32524,#32525,
#32526,#32527,#32528,#32529,#32530),.UNSPECIFIED.,.F.,.F.,(4,3,3,3,3,3,
3,3,3,3,3,3,3,3,4),(-79.208223695028,-79.1930557399212,-78.6949862069658,
-78.1969166740103,-77.6988471410548,-77.2007776080993,-76.7027080751438,
-76.2046385421883,-75.7065690092329,-75.2084994762774,-74.7104299433219,
-74.2123604103664,-73.714290877411,-73.2162213444555,-72.9250383878484),
 .UNSPECIFIED.);
#4818=B_SPLINE_CURVE_WITH_KNOTS('',3,(#32531,#32532,#32533,#32534,#32535,
#32536,#32537,#32538,#32539,#32540,#32541,#32542,#32543,#32544,#32545,#32546,
#32547,#32548,#32549,#32550,#32551,#32552,#32553,#32554,#32555,#32556,#32557,
#32558,#32559,#32560,#32561,#32562,#32563,#32564,#32565,#32566,#32567,#32568,
#32569,#32570,#32571,#32572,#32573),.UNSPECIFIED.,.F.,.F.,(4,3,3,3,3,3,
3,3,3,3,3,3,3,3,4),(69.9522016271069,70.2278041467226,70.7258736796781,
71.2239432126336,71.7220127455891,72.2200822785446,72.7181518115,73.2162213444555,
73.714290877411,74.2123604103665,74.7104299433219,75.2084994762774,75.7065690092329,
76.2046385421884,76.2353869342864),.UNSPECIFIED.);
#4819=B_SPLINE_CURVE_WITH_KNOTS('',3,(#32578,#32579,#32580,#32581,#32582,
#32583,#32584,#32585,#32586,#32587,#32588,#32589,#32590,#32591,#32592,#32593,
#32594,#32595,#32596,#32597,#32598,#32599,#32600,#32601,#32602,#32603,#32604,
#32605,#32606,#32607,#32608,#32609,#32610,#32611,#32612,#32613,#32614,#32615,
#32616,#32617),.UNSPECIFIED.,.F.,.F.,(4,3,3,3,3,3,3,3,3,3,3,3,3,4),(-85.4914090022076,
-85.169890135387,-84.6718206024315,-84.1737510694761,-83.6756815365206,
-83.1776120035651,-82.6795424706096,-82.1814729376541,-81.6834034046987,
-81.1853338717432,-80.6872643387877,-80.1891948058322,-79.6911252728767,
-79.208223695028),.UNSPECIFIED.);
#4820=B_SPLINE_CURVE_WITH_KNOTS('',3,(#32618,#32619,#32620,#32621,#32622,
#32623,#32624,#32625,#32626,#32627,#32628,#32629,#32630,#32631,#32632,#32633,
#32634,#32635,#32636,#32637,#32638,#32639,#32640,#32641,#32642,#32643,#32644,
#32645,#32646,#32647,#32648,#32649,#32650,#32651,#32652,#32653,#32654,#32655,
#32656,#32657),.UNSPECIFIED.,.F.,.F.,(4,3,3,3,3,3,3,3,3,3,3,3,3,4),(76.2353869342864,
76.7027080751439,77.2007776080993,77.6988471410548,78.1969166740103,78.6949862069658,
79.1930557399212,79.6911252728767,80.1891948058322,80.6872643387877,81.1853338717432,
81.6834034046987,82.1814729376541,82.5185722414661),.UNSPECIFIED.);
#4821=B_SPLINE_CURVE_WITH_KNOTS('',3,(#32662,#32663,#32664,#32665,#32666,
#32667,#32668,#32669,#32670,#32671,#32672,#32673,#32674,#32675,#32676,#32677,
#32678,#32679,#32680,#32681,#32682,#32683,#32684,#32685,#32686,#32687,#32688,
#32689,#32690,#32691,#32692,#32693,#32694,#32695,#32696,#32697,#32698,#32699,
#32700,#32701,#32702,#32703,#32704),.UNSPECIFIED.,.F.,.F.,(4,3,3,3,3,3,
3,3,3,3,3,3,3,3,4),(-91.7745943093872,-91.6447940638082,-91.1467245308528,
-90.6486549978973,-90.1505854649418,-89.6525159319863,-89.1544463990308,
-88.6563768660754,-88.1583073331199,-87.6602378001644,-87.1621682672089,
-86.6640987342534,-86.166029201298,-85.6679596683425,-85.4914090022076),
 .UNSPECIFIED.);
#4822=B_SPLINE_CURVE_WITH_KNOTS('',3,(#32705,#32706,#32707,#32708,#32709,
#32710,#32711,#32712,#32713,#32714,#32715,#32716,#32717,#32718,#32719,#32720,
#32721,#32722,#32723,#32724,#32725,#32726,#32727,#32728,#32729,#32730,#32731,
#32732,#32733,#32734,#32735,#32736,#32737,#32738,#32739,#32740,#32741,#32742,
#32743,#32744,#32745,#32746,#32747),.UNSPECIFIED.,.F.,.F.,(4,3,3,3,3,3,
3,3,3,3,3,3,3,3,4),(82.5185722414661,82.6795424706096,83.1776120035651,
83.6756815365206,84.1737510694761,84.6718206024316,85.169890135387,85.6679596683425,
86.166029201298,86.6640987342535,87.1621682672089,87.6602378001644,88.1583073331199,
88.6563768660754,88.8017575486456),.UNSPECIFIED.);
#4823=B_SPLINE_CURVE_WITH_KNOTS('',3,(#32752,#32753,#32754,#32755,#32756,
#32757,#32758,#32759,#32760,#32761,#32762,#32763,#32764,#32765,#32766,#32767,
#32768,#32769,#32770,#32771,#32772,#32773,#32774,#32775,#32776,#32777,#32778,
#32779,#32780,#32781,#32782,#32783,#32784,#32785,#32786,#32787,#32788,#32789,
#32790,#32791),.UNSPECIFIED.,.F.,.F.,(4,3,3,3,3,3,3,3,3,3,3,3,3,4),(-98.0577796165668,
-97.621628459274,-97.1235589263185,-96.625489393363,-96.1274198604075,-95.6293503274521,
-95.1312807944966,-94.6332112615411,-94.1351417285857,-93.6370721956302,
-93.1390026626747,-92.6409331297192,-92.1428635967637,-91.7745943093872),
 .UNSPECIFIED.);
#4824=B_SPLINE_CURVE_WITH_KNOTS('',3,(#32792,#32793,#32794,#32795,#32796,
#32797,#32798,#32799,#32800,#32801,#32802,#32803,#32804,#32805,#32806,#32807,
#32808,#32809,#32810,#32811,#32812,#32813,#32814,#32815,#32816,#32817,#32818,
#32819,#32820,#32821,#32822,#32823,#32824,#32825,#32826,#32827,#32828,#32829,
#32830,#32831),.UNSPECIFIED.,.F.,.F.,(4,3,3,3,3,3,3,3,3,3,3,3,3,4),(88.8017575486456,
89.1544463990309,89.6525159319864,90.1505854649418,90.6486549978973,91.1467245308528,
91.6447940638083,92.1428635967637,92.6409331297192,93.1390026626747,93.6370721956302,
94.1351417285857,94.6332112615411,95.0849428558252),.UNSPECIFIED.);
#4825=B_SPLINE_CURVE_WITH_KNOTS('',3,(#32837,#32838,#32839,#32840,#32841,
#32842,#32843,#32844,#32845),.UNSPECIFIED.,.F.,.F.,(4,1,1,1,1,1,4),(109.955742875643,
110.017661251305,110.515730784261,111.013800317216,111.511869850172,112.009939383127,
112.428928173949),.UNSPECIFIED.);
#4826=B_SPLINE_CURVE_WITH_KNOTS('',3,(#32848,#32849,#32850,#32851,#32852,
#32853),.UNSPECIFIED.,.F.,.F.,(4,1,1,4),(109.955742875643,110.193799435556,
110.691868968511,111.189938501467),.UNSPECIFIED.);
#4827=B_SPLINE_CURVE_WITH_KNOTS('',3,(#32858,#32859,#32860,#32861,#32862,
#32863,#32864,#32865,#32866,#32867,#32868,#32869,#32870,#32871,#32872,#32873),
 .UNSPECIFIED.,.F.,.F.,(4,1,1,1,1,1,1,1,1,1,1,1,1,4),(103.672557568463,
104.04082685584,104.538896388795,105.036965921751,105.535035454706,106.033104987662,
106.531174520617,107.029244053573,107.527313586528,108.025383119484,108.523452652439,
109.021522185394,109.51959171835,109.955742875643),.UNSPECIFIED.);
#4828=B_SPLINE_CURVE_WITH_KNOTS('',3,(#32874,#32875,#32876,#32877,#32878,
#32879,#32880,#32881,#32882,#32883,#32884,#32885,#32886,#32887,#32888,#32889,
#32890),.UNSPECIFIED.,.F.,.F.,(4,1,1,1,1,1,1,1,1,1,1,1,1,1,4),(103.672557568463,
103.718895507134,104.21696504009,104.715034573045,105.213104106001,105.711173638956,
106.209243171912,106.707312704867,107.205382237823,107.703451770778,108.201521303734,
108.699590836689,109.197660369645,109.6957299026,109.955742875643),
 .UNSPECIFIED.);
#4829=B_SPLINE_CURVE_WITH_KNOTS('',3,(#32895,#32896,#32897,#32898,#32899,
#32900,#32901,#32902,#32903,#32904,#32905,#32906,#32907,#32908,#32909,#32910,
#32911),.UNSPECIFIED.,.F.,.F.,(4,1,1,1,1,1,1,1,1,1,1,1,1,1,4),(97.3893722612836,
97.5659229274184,98.0639924603739,98.5620619933294,99.0601315262849,99.5582010592404,
100.056270592196,100.554340125151,101.052409658107,101.550479191062,102.048548724018,
102.546618256973,103.044687789929,103.542757322884,103.672557568463),
 .UNSPECIFIED.);
#4830=B_SPLINE_CURVE_WITH_KNOTS('',3,(#32912,#32913,#32914,#32915,#32916,
#32917,#32918,#32919,#32920,#32921,#32922,#32923,#32924,#32925,#32926,#32927),
 .UNSPECIFIED.,.F.,.F.,(4,1,1,1,1,1,1,1,1,1,1,1,1,4),(97.3893722612836,
97.7420611116687,98.2401306446242,98.7382001775796,99.2362697105351,99.7343392434906,
100.232408776446,100.730478309402,101.228547842357,101.726617375313,102.224686908268,
102.722756441223,103.220825974179,103.672557568463),.UNSPECIFIED.);
#4831=B_SPLINE_CURVE_WITH_KNOTS('',3,(#32932,#32933,#32934,#32935,#32936,
#32937,#32938,#32939,#32940,#32941,#32942,#32943,#32944,#32945,#32946,#32947),
 .UNSPECIFIED.,.F.,.F.,(4,1,1,1,1,1,1,1,1,1,1,1,1,4),(91.106186954104,91.5890885319527,
92.0871580649082,92.5852275978636,93.0832971308191,93.5813666637746,94.0794361967301,
94.5775057296856,95.0755752626411,95.5736447955965,96.071714328552,96.5697838615075,
97.067853394463,97.3893722612836),.UNSPECIFIED.);
#4832=B_SPLINE_CURVE_WITH_KNOTS('',3,(#32948,#32949,#32950,#32951,#32952,
#32953,#32954,#32955,#32956,#32957,#32958,#32959,#32960,#32961,#32962,#32963,
#32964),.UNSPECIFIED.,.F.,.F.,(4,1,1,1,1,1,1,1,1,1,1,1,1,1,4),(91.106186954104,
91.2671571832475,91.7652267162029,92.2632962491584,92.7613657821139,93.2594353150694,
93.7575048480249,94.2555743809803,94.7536439139358,95.2517134468913,95.7497829798468,
96.2478525128023,96.7459220457577,97.2439915787132,97.3893722612836),
 .UNSPECIFIED.);
#4833=B_SPLINE_CURVE_WITH_KNOTS('',3,(#32969,#32970,#32971,#32972,#32973,
#32974,#32975,#32976,#32977,#32978,#32979,#32980,#32981,#32982,#32983,#32984,
#32985),.UNSPECIFIED.,.F.,.F.,(4,1,1,1,1,1,1,1,1,1,1,1,1,1,4),(84.8230016469244,
85.1141846035315,85.6122541364869,86.1103236694424,86.6083932023979,87.1064627353534,
87.6045322683088,88.1026018012643,88.6006713342198,89.0987408671753,89.5968104001308,
90.0948799330862,90.5929494660417,91.0910189989972,91.106186954104),
 .UNSPECIFIED.);
#4834=B_SPLINE_CURVE_WITH_KNOTS('',3,(#32986,#32987,#32988,#32989,#32990,
#32991,#32992,#32993,#32994,#32995,#32996,#32997,#32998,#32999,#33000,#33001),
 .UNSPECIFIED.,.F.,.F.,(4,1,1,1,1,1,1,1,1,1,1,1,1,4),(84.8230016469244,
85.2903227877817,85.7883923207372,86.2864618536927,86.7845313866481,87.2826009196036,
87.7806704525591,88.2787399855146,88.7768095184701,89.2748790514255,89.772948584381,
90.2710181173365,90.769087650292,91.106186954104),.UNSPECIFIED.);
#4835=B_SPLINE_CURVE_WITH_KNOTS('',3,(#33006,#33007,#33008,#33009,#33010,
#33011,#33012,#33013,#33014,#33015,#33016,#33017,#33018,#33019,#33020,#33021,
#33022),.UNSPECIFIED.,.F.,.F.,(4,1,1,1,1,1,1,1,1,1,1,1,1,1,4),(78.5398163397448,
78.6392806751102,79.1373502080657,79.6354197410212,80.1334892739767,80.6315588069321,
81.1296283398876,81.6276978728431,82.1257674057986,82.6238369387541,83.1219064717095,
83.619976004665,84.1180455376205,84.616115070576,84.8230016469244),
 .UNSPECIFIED.);
#4836=B_SPLINE_CURVE_WITH_KNOTS('',3,(#33023,#33024,#33025,#33026,#33027,
#33028,#33029,#33030,#33031,#33032,#33033,#33034,#33035,#33036,#33037,#33038,
#33039),.UNSPECIFIED.,.F.,.F.,(4,1,1,1,1,1,1,1,1,1,1,1,1,1,4),(78.5398163397448,
78.8154188593605,79.3134883923159,79.8115579252714,80.3096274582269,80.8076969911824,
81.3057665241379,81.8038360570933,82.3019055900488,82.7999751230043,83.2980446559598,
83.7961141889153,84.2941837218707,84.7922532548262,84.8230016469244),
 .UNSPECIFIED.);
#4837=B_SPLINE_CURVE_WITH_KNOTS('',3,(#33044,#33045,#33046,#33047,#33048,
#33049,#33050,#33051,#33052,#33053,#33054,#33055,#33056,#33057,#33058,#33059),
 .UNSPECIFIED.,.F.,.F.,(4,1,1,1,1,1,1,1,1,1,1,1,1,4),(72.2566310325652,
72.6624462796445,73.1605158125999,73.6585853455554,74.1566548785109,74.6547244114664,
75.1527939444219,75.6508634773773,76.1489330103328,76.6470025432883,77.1450720762438,
77.6431416091993,78.1412111421547,78.5398163397448),.UNSPECIFIED.);
#4838=B_SPLINE_CURVE_WITH_KNOTS('',3,(#33060,#33061,#33062,#33063,#33064,
#33065,#33066,#33067,#33068,#33069,#33070,#33071,#33072,#33073,#33074,#33075,
#33076),.UNSPECIFIED.,.F.,.F.,(4,1,1,1,1,1,1,1,1,1,1,1,1,1,4),(72.2566310325652,
72.3405149309392,72.8385844638947,73.3366539968502,73.8347235298057,74.3327930627611,
74.8308625957166,75.3289321286721,75.8270016616276,76.3250711945831,76.8231407275385,
77.321210260494,77.8192797934495,78.317349326405,78.5398163397448),
 .UNSPECIFIED.);
#4839=B_SPLINE_CURVE_WITH_KNOTS('',3,(#33081,#33082,#33083,#33084,#33085,
#33086,#33087,#33088,#33089,#33090,#33091,#33092,#33093,#33094,#33095,#33096,
#33097),.UNSPECIFIED.,.F.,.F.,(4,1,1,1,1,1,1,1,1,1,1,1,1,1,4),(65.9734457253856,
66.1875423512232,66.6856118841787,67.1836814171342,67.6817509500897,68.1798204830451,
68.6778900160006,69.1759595489561,69.6740290819116,70.1720986148671,70.6701681478225,
71.168237680778,71.6663072137335,72.164376746689,72.2566310325652),
 .UNSPECIFIED.);
#4840=B_SPLINE_CURVE_WITH_KNOTS('',3,(#33098,#33099,#33100,#33101,#33102,
#33103,#33104,#33105,#33106,#33107,#33108,#33109,#33110,#33111,#33112,#33113),
 .UNSPECIFIED.,.F.,.F.,(4,1,1,1,1,1,1,1,1,1,1,1,1,4),(65.9734457253856,
66.3636805354735,66.861750068429,67.3598196013844,67.8578891343399,68.3559586672954,
68.8540282002509,69.3520977332063,69.8501672661618,70.3482367991173,70.8463063320728,
71.3443758650283,71.8424453979838,72.2566310325652),.UNSPECIFIED.);
#4841=B_SPLINE_CURVE_WITH_KNOTS('',3,(#33118,#33119,#33120,#33121,#33122,
#33123,#33124,#33125,#33126,#33127,#33128,#33129,#33130,#33131,#33132,#33133,
#33134),.UNSPECIFIED.,.F.,.F.,(4,1,1,1,1,1,1,1,1,1,1,1,1,1,4),(59.690260418206,
59.712638422802,60.2107079557575,60.708777488713,61.2068470216684,61.7049165546239,
62.2029860875794,62.7010556205349,63.1991251534903,63.6971946864458,64.1952642194013,
64.6933337523568,65.1914032853123,65.6894728182677,65.9734457253856),
 .UNSPECIFIED.);
#4842=B_SPLINE_CURVE_WITH_KNOTS('',3,(#33135,#33136,#33137,#33138,#33139,
#33140,#33141,#33142,#33143,#33144,#33145,#33146,#33147,#33148,#33149,#33150,
#33151),.UNSPECIFIED.,.F.,.F.,(4,1,1,1,1,1,1,1,1,1,1,1,1,1,4),(59.690260418206,
59.8887766070523,60.3868461400077,60.8849156729632,61.3829852059187,61.8810547388742,
62.3791242718296,62.8771938047851,63.3752633377406,63.8733328706961,64.3714024036516,
64.869471936607,65.3675414695625,65.865611002518,65.9734457253856),
 .UNSPECIFIED.);
#4843=B_SPLINE_CURVE_WITH_KNOTS('',3,(#33156,#33157,#33158,#33159,#33160,
#33161,#33162,#33163,#33164,#33165,#33166,#33167,#33168,#33169,#33170,#33171),
 .UNSPECIFIED.,.F.,.F.,(4,1,1,1,1,1,1,1,1,1,1,1,1,4),(53.4070751110264,
53.7358040273362,54.2338735602917,54.7319430932472,55.2300126262027,55.7280821591582,
56.2261516921136,56.7242212250691,57.2222907580246,57.7203602909801,58.2184298239356,
58.716499356891,59.2145688898465,59.690260418206),.UNSPECIFIED.);
#4844=B_SPLINE_CURVE_WITH_KNOTS('',3,(#33172,#33173,#33174,#33175,#33176,
#33177,#33178,#33179,#33180,#33181,#33182,#33183,#33184,#33185,#33186,#33187,
#33188),.UNSPECIFIED.,.F.,.F.,(4,1,1,1,1,1,1,1,1,1,1,1,1,1,4),(53.4070751110264,
53.413872678631,53.9119422115865,54.410011744542,54.9080812774974,55.4061508104529,
55.9042203434084,56.4022898763639,56.9003594093194,57.3984289422748,57.8964984752303,
58.3945680081858,58.8926375411413,59.3907070740968,59.690260418206),
 .UNSPECIFIED.);
#4845=B_SPLINE_CURVE_WITH_KNOTS('',3,(#33193,#33194,#33195,#33196,#33197,
#33198,#33199,#33200,#33201,#33202,#33203,#33204,#33205,#33206,#33207,#33208,
#33209),.UNSPECIFIED.,.F.,.F.,(4,1,1,1,1,1,1,1,1,1,1,1,1,1,4),(47.1238898038469,
47.260900098915,47.7589696318705,48.257039164826,48.7551086977815,49.2531782307369,
49.7512477636924,50.2493172966479,50.7473868296034,51.2454563625588,51.7435258955143,
52.2415954284698,52.7396649614253,53.2377344943808,53.4070751110264),
 .UNSPECIFIED.);
#4846=B_SPLINE_CURVE_WITH_KNOTS('',3,(#33210,#33211,#33212,#33213,#33214,
#33215,#33216,#33217,#33218,#33219,#33220,#33221,#33222,#33223,#33224,#33225),
 .UNSPECIFIED.,.F.,.F.,(4,1,1,1,1,1,1,1,1,1,1,1,1,4),(47.1238898038468,
47.4370382831653,47.9351078161207,48.4331773490762,48.9312468820317,49.4293164149872,
49.9273859479427,50.4254554808981,50.9235250138536,51.4215945468091,51.9196640797646,
52.41773361272,52.9158031456755,53.4070751110264),.UNSPECIFIED.);
#4847=B_SPLINE_CURVE_WITH_KNOTS('',3,(#33230,#33231,#33232,#33233,#33234,
#33235,#33236,#33237,#33238,#33239,#33240,#33241,#33242,#33243,#33244,#33245),
 .UNSPECIFIED.,.F.,.F.,(4,1,1,1,1,1,1,1,1,1,1,1,1,4),(40.8407044966672,
41.2840657034493,41.7821352364047,42.2802047693602,42.7782743023157,43.2763438352712,
43.7744133682266,44.2724829011821,44.7705524341376,45.2686219670931,45.7666915000486,
46.264761033004,46.7628305659595,47.1238898038469),.UNSPECIFIED.);
#4848=B_SPLINE_CURVE_WITH_KNOTS('',3,(#33246,#33247,#33248,#33249,#33250,
#33251,#33252,#33253,#33254,#33255,#33256,#33257,#33258,#33259,#33260,#33261,
#33262),.UNSPECIFIED.,.F.,.F.,(4,1,1,1,1,1,1,1,1,1,1,1,1,1,4),(40.8407044966672,
40.962134354744,41.4602038876995,41.958273420655,42.4563429536105,42.9544124865659,
43.4524820195214,43.9505515524769,44.4486210854324,44.9466906183878,45.4447601513433,
45.9428296842988,46.4408992172543,46.9389687502098,47.1238898038468),
 .UNSPECIFIED.);
#4849=B_SPLINE_CURVE_WITH_KNOTS('',3,(#33267,#33268,#33269,#33270,#33271,
#33272,#33273,#33274,#33275,#33276,#33277,#33278,#33279,#33280,#33281,#33282,
#33283),.UNSPECIFIED.,.F.,.F.,(4,1,1,1,1,1,1,1,1,1,1,1,1,1,4),(34.5575191894876,
34.809161775028,35.3072313079835,35.805300840939,36.3033703738945,36.8014399068499,
37.2995094398054,37.7975789727609,38.2956485057164,38.7937180386719,39.2917875716273,
39.7898571045828,40.2879266375383,40.7859961704938,40.8407044966672),
 .UNSPECIFIED.);
#4850=B_SPLINE_CURVE_WITH_KNOTS('',3,(#33284,#33285,#33286,#33287,#33288,
#33289,#33290,#33291,#33292,#33293,#33294,#33295,#33296,#33297,#33298,#33299),
 .UNSPECIFIED.,.F.,.F.,(4,1,1,1,1,1,1,1,1,1,1,1,1,4),(34.5575191894876,
34.9852999592783,35.4833694922337,35.9814390251892,36.4795085581447,36.9775780911002,
37.4756476240557,37.9737171570111,38.4717866899666,38.9698562229221,39.4679257558776,
39.9659952888331,40.4640648217885,40.8407044966672),.UNSPECIFIED.);
#4851=B_SPLINE_CURVE_WITH_KNOTS('',3,(#33304,#33305,#33306,#33307,#33308,
#33309,#33310,#33311,#33312,#33313,#33314,#33315,#33316,#33317,#33318,#33319,
#33320),.UNSPECIFIED.,.F.,.F.,(4,1,1,1,1,1,1,1,1,1,1,1,1,1,4),(28.2743338823081,
28.3342578466068,28.8323273795623,29.3303969125177,29.8284664454732,30.3265359784287,
30.8246055113842,31.3226750443397,31.8207445772951,32.3188141102506,32.8168836432061,
33.3149531761616,33.8130227091171,34.3110922420725,34.5575191894876),
 .UNSPECIFIED.);
#4852=B_SPLINE_CURVE_WITH_KNOTS('',3,(#33321,#33322,#33323,#33324,#33325,
#33326,#33327,#33328,#33329,#33330,#33331,#33332,#33333,#33334,#33335,#33336,
#33337),.UNSPECIFIED.,.F.,.F.,(4,1,1,1,1,1,1,1,1,1,1,1,1,1,4),(28.274333882308,
28.510396030857,29.0084655638125,29.506535096768,30.0046046297235,30.5026741626789,
31.0007436956344,31.4988132285899,31.9968827615454,32.4949522945009,32.9930218274563,
33.4910913604118,33.9891608933673,34.4872304263228,34.5575191894876),
 .UNSPECIFIED.);
#4853=B_SPLINE_CURVE_WITH_KNOTS('',3,(#33342,#33343,#33344,#33345,#33346,
#33347,#33348,#33349,#33350,#33351,#33352,#33353,#33354,#33355,#33356,#33357),
 .UNSPECIFIED.,.F.,.F.,(4,1,1,1,1,1,1,1,1,1,1,1,1,4),(21.9911485751285,
22.357423451141,22.8554929840965,23.353562517052,23.8516320500075,24.349701582963,
24.8477711159184,25.3458406488739,25.8439101818294,26.3419797147849,26.8400492477403,
27.3381187806958,27.8361883136513,28.2743338823081),.UNSPECIFIED.);
#4854=B_SPLINE_CURVE_WITH_KNOTS('',3,(#33358,#33359,#33360,#33361,#33362,
#33363,#33364,#33365,#33366,#33367,#33368,#33369,#33370,#33371,#33372,#33373,
#33374),.UNSPECIFIED.,.F.,.F.,(4,1,1,1,1,1,1,1,1,1,1,1,1,1,4),(21.9911485751285,
22.0354921024358,22.5335616353913,23.0316311683467,23.5297007013022,24.0277702342577,
24.5258397672132,25.0239093001687,25.5219788331241,26.0200483660796,26.5181178990351,
27.0161874319906,27.5142569649461,28.0123264979015,28.274333882308),
 .UNSPECIFIED.);
#4855=B_SPLINE_CURVE_WITH_KNOTS('',3,(#33379,#33380,#33381,#33382,#33383,
#33384,#33385,#33386,#33387,#33388,#33389,#33390,#33391,#33392,#33393,#33394,
#33395),.UNSPECIFIED.,.F.,.F.,(4,1,1,1,1,1,1,1,1,1,1,1,1,1,4),(15.7079632679489,
15.8825195227198,16.3805890556753,16.8786585886308,17.3767281215862,17.8747976545417,
18.3728671874972,18.8709367204527,19.3690062534082,19.8670757863636,20.3651453193191,
20.8632148522746,21.3612843852301,21.8593539181856,21.9911485751285),
 .UNSPECIFIED.);
#4856=B_SPLINE_CURVE_WITH_KNOTS('',3,(#33396,#33397,#33398,#33399,#33400,
#33401,#33402,#33403,#33404,#33405,#33406,#33407,#33408,#33409,#33410,#33411),
 .UNSPECIFIED.,.F.,.F.,(4,1,1,1,1,1,1,1,1,1,1,1,1,4),(15.7079632679489,
16.05865770697,16.5567272399255,17.054796772881,17.5528663058365,18.0509358387919,
18.5490053717474,19.0470749047029,19.5451444376584,20.0432139706139,20.5412835035693,
21.0393530365248,21.5374225694803,21.9911485751285),.UNSPECIFIED.);
#4857=B_SPLINE_CURVE_WITH_KNOTS('',3,(#33417,#33418,#33419,#33420,#33421,
#33422,#33423),.UNSPECIFIED.,.F.,.F.,(4,3,4),(405.265452313083,405.559874952706,
406.482000549955),.UNSPECIFIED.);
#4858=B_SPLINE_CURVE_WITH_KNOTS('',3,(#33429,#33430,#33431,#33432,#33433,
#33434,#33435,#33436,#33437,#33438,#33439,#33440),.UNSPECIFIED.,.F.,.F.,
(4,1,1,1,1,1,1,1,1,4),(398.982267005904,399.572906010296,400.570734167364,
401.568562324433,402.067476402967,402.566390481501,403.065304560035,403.564218638569,
404.562046795637,405.265452313083),.UNSPECIFIED.);
#4859=B_SPLINE_CURVE_WITH_KNOTS('',3,(#33443,#33444,#33445,#33446,#33447,
#33448,#33449,#33450,#33451,#33452,#33453,#33454,#33455),.UNSPECIFIED.,
 .F.,.F.,(4,1,1,1,1,1,1,1,1,1,4),(398.982267005904,399.256041935063,399.754956013597,
400.253870092131,401.251698249199,402.249526406267,403.247354563336,403.74626864187,
404.245182720404,404.744096798938,405.243010877472),.UNSPECIFIED.);
#4860=B_SPLINE_CURVE_WITH_KNOTS('',3,(#33460,#33461,#33462,#33463,#33464,
#33465,#33466,#33467,#33468,#33469,#33470,#33471),.UNSPECIFIED.,.F.,.F.,
(4,1,1,1,1,1,1,1,1,4),(392.699081698724,393.585937067887,394.583765224955,
395.082679303489,395.581593382023,396.080507460557,396.579421539091,397.57724969616,
398.575077853228,398.982267005904),.UNSPECIFIED.);
#4861=B_SPLINE_CURVE_WITH_KNOTS('',3,(#33472,#33473,#33474,#33475,#33476,
#33477,#33478,#33479,#33480,#33481,#33482,#33483),.UNSPECIFIED.,.F.,.F.,
(4,1,1,1,1,1,1,1,1,4),(392.699081698724,392.770158914119,393.269072992653,
394.266901149721,395.26472930679,396.262557463858,397.260385620926,398.258213777994,
398.757127856529,398.982267005904),.UNSPECIFIED.);
#4862=B_SPLINE_CURVE_WITH_KNOTS('',3,(#33488,#33489,#33490,#33491,#33492,
#33493,#33494,#33495,#33496,#33497,#33498,#33499,#33500),.UNSPECIFIED.,
 .F.,.F.,(4,1,1,1,1,1,1,1,1,1,4),(386.415896391544,386.601139968409,387.598968125477,
388.097882204011,388.596796282545,389.095710361079,389.594624439613,390.592452596682,
391.59028075375,392.588108910818,392.699081698724),.UNSPECIFIED.);
#4863=B_SPLINE_CURVE_WITH_KNOTS('',3,(#33501,#33502,#33503,#33504,#33505,
#33506,#33507,#33508,#33509,#33510,#33511),.UNSPECIFIED.,.F.,.F.,(4,1,1,
1,1,1,1,1,4),(386.415896391545,387.282104050244,388.279932207312,389.27776036438,
390.275588521448,391.273416678517,391.772330757051,392.271244835585,392.699081698724),
 .UNSPECIFIED.);
#4864=B_SPLINE_CURVE_WITH_KNOTS('',3,(#33516,#33517,#33518,#33519,#33520,
#33521,#33522,#33523,#33524,#33525,#33526,#33527),.UNSPECIFIED.,.F.,.F.,
(4,1,1,1,1,1,1,1,1,4),(380.132711084365,380.614171025999,381.113085104533,
381.611999183067,382.110913261602,382.609827340136,383.607655497204,384.605483654272,
385.60331181134,386.415896391544),.UNSPECIFIED.);
#4865=B_SPLINE_CURVE_WITH_KNOTS('',3,(#33528,#33529,#33530,#33531,#33532,
#33533,#33534,#33535,#33536,#33537,#33538,#33539,#33540,#33541,#33542,#33543,
#33544,#33545,#33546,#33547,#33548,#33549,#33550,#33551,#33552),
 .UNSPECIFIED.,.F.,.F.,(4,3,3,3,3,3,3,3,4),(380.132711084365,381.019390447226,
381.906069810087,382.792749172948,383.679428535808,384.566107898669,385.45278726153,
386.339466624391,386.415896391545),.UNSPECIFIED.);
#4866=B_SPLINE_CURVE_WITH_KNOTS('',3,(#33557,#33558,#33559,#33560,#33561,
#33562,#33563,#33564,#33565,#33566,#33567,#33568,#33569,#33570,#33571,#33572,
#33573,#33574,#33575,#33576,#33577,#33578,#33579,#33580,#33581),
 .UNSPECIFIED.,.F.,.F.,(4,3,3,3,3,3,3,3,4),(373.849525777185,374.736205140046,
375.622884502907,376.509563865768,377.396243228629,378.28292259149,379.16960195435,
380.056281317211,380.132711084365),.UNSPECIFIED.);
#4867=B_SPLINE_CURVE_WITH_KNOTS('',3,(#33582,#33583,#33584,#33585,#33586,
#33587,#33588,#33589,#33590,#33591,#33592,#33593),.UNSPECIFIED.,.F.,.F.,
(4,1,1,1,1,1,1,1,1,4),(373.849525777185,374.310338008356,375.308166165424,
376.305994322493,377.303822479561,377.802736558095,378.301650636629,378.800564715163,
379.299478793698,380.132711084365),.UNSPECIFIED.);
#4868=B_SPLINE_CURVE_WITH_KNOTS('',3,(#33598,#33599,#33600,#33601,#33602,
#33603,#33604,#33605,#33606,#33607,#33608,#33609),.UNSPECIFIED.,.F.,.F.,
(4,1,1,1,1,1,1,1,1,4),(367.566340470006,367.642404984112,368.141319062646,
368.64023314118,369.638061298248,370.635889455317,371.633717612385,372.631545769453,
373.629373926521,373.849525777185),.UNSPECIFIED.);
#4869=B_SPLINE_CURVE_WITH_KNOTS('',3,(#33610,#33611,#33612,#33613,#33614,
#33615,#33616,#33617,#33618,#33619,#33620,#33621),.UNSPECIFIED.,.F.,.F.,
(4,1,1,1,1,1,1,1,1,4),(367.566340470006,368.323369065947,369.321197223015,
370.319025380083,370.817939458617,371.316853537151,371.815767615686,372.31468169422,
373.312509851288,373.849525777185),.UNSPECIFIED.);
#4870=B_SPLINE_CURVE_WITH_KNOTS('',3,(#33626,#33627,#33628,#33629,#33630,
#33631,#33632,#33633,#33634,#33635,#33636),.UNSPECIFIED.,.F.,.F.,(4,1,1,
1,1,1,1,1,4),(361.283155162826,361.655436041702,362.653264198771,363.651092355839,
364.648920512907,365.646748669975,366.644576827044,367.143490905578,367.566340470006),
 .UNSPECIFIED.);
#4871=B_SPLINE_CURVE_WITH_KNOTS('',3,(#33637,#33638,#33639,#33640,#33641,
#33642,#33643,#33644,#33645,#33646,#33647,#33648,#33649),.UNSPECIFIED.,
 .F.,.F.,(4,1,1,1,1,1,1,1,1,1,4),(361.283155162826,361.338571966469,362.336400123537,
363.334228280605,363.83314235914,364.332056437674,364.830970516208,365.329884594742,
366.32771275181,367.325540908878,367.566340470006),.UNSPECIFIED.);
#4872=B_SPLINE_CURVE_WITH_KNOTS('',3,(#33654,#33655,#33656,#33657,#33658,
#33659,#33660,#33661,#33662,#33663,#33664,#33665,#33666,#33667,#33668,#33669,
#33670,#33671,#33672,#33673,#33674,#33675,#33676,#33677,#33678),
 .UNSPECIFIED.,.F.,.F.,(4,3,3,3,3,3,3,3,4),(354.999969855647,355.886649218508,
356.773328581368,357.660007944229,358.54668730709,359.433366669951,360.320046032812,
361.206725395673,361.283155162826),.UNSPECIFIED.);
#4873=B_SPLINE_CURVE_WITH_KNOTS('',3,(#33679,#33680,#33681,#33682,#33683,
#33684,#33685,#33686,#33687,#33688,#33689,#33690),.UNSPECIFIED.,.F.,.F.,
(4,1,1,1,1,1,1,1,1,4),(354.999969855647,355.351603024059,356.349431181128,
356.848345259662,357.347259338196,357.84617341673,358.345087495264,359.342915652332,
360.340743809401,361.283155162826),.UNSPECIFIED.);
#4874=B_SPLINE_CURVE_WITH_KNOTS('',3,(#33695,#33696,#33697,#33698,#33699,
#33700,#33701,#33702,#33703,#33704,#33705,#33706),.UNSPECIFIED.,.F.,.F.,
(4,1,1,1,1,1,1,1,1,4),(348.716784548467,349.681498156883,350.679326313951,
351.67715447102,352.674982628088,353.173896706622,353.672810785156,354.17172486369,
354.670638942224,354.999969855647),.UNSPECIFIED.);
#4875=B_SPLINE_CURVE_WITH_KNOTS('',3,(#33707,#33708,#33709,#33710,#33711,
#33712,#33713,#33714,#33715,#33716,#33717,#33718,#33719,#33720,#33721,#33722,
#33723,#33724,#33725,#33726,#33727,#33728,#33729,#33730,#33731),
 .UNSPECIFIED.,.F.,.F.,(4,3,3,3,3,3,3,3,4),(348.716784548467,349.603463911328,
350.490143274189,351.37682263705,352.26350199991,353.150181362771,354.036860725632,
354.923540088493,354.999969855647),.UNSPECIFIED.);
#4876=B_SPLINE_CURVE_WITH_KNOTS('',3,(#33736,#33737,#33738,#33739,#33740,
#33741,#33742,#33743,#33744,#33745,#33746,#33747,#33748),.UNSPECIFIED.,
 .F.,.F.,(4,1,1,1,1,1,1,1,1,1,4),(342.433599241288,342.696701057405,343.694529214474,
344.692357371542,345.69018552861,346.189099607144,346.688013685678,347.186927764213,
347.685841842747,348.683669999815,348.716784548467),.UNSPECIFIED.);
#4877=B_SPLINE_CURVE_WITH_KNOTS('',3,(#33749,#33750,#33751,#33752,#33753,
#33754,#33755,#33756,#33757,#33758,#33759,#33760),.UNSPECIFIED.,.F.,.F.,
(4,1,1,1,1,1,1,1,1,4),(342.433599241288,342.878751060706,343.37766513924,
343.876579217774,344.375493296308,345.373321453377,346.371149610445,347.368977767513,
348.366805924582,348.716784548467),.UNSPECIFIED.);
#4878=B_SPLINE_CURVE_WITH_KNOTS('',3,(#33765,#33766,#33767,#33768,#33769,
#33770,#33771,#33772,#33773,#33774,#33775,#33776),.UNSPECIFIED.,.F.,.F.,
(4,1,1,1,1,1,1,1,1,4),(336.150413934108,336.709732114996,337.707560272064,
338.705388429132,339.204302507666,339.703216586201,340.202130664735,340.701044743269,
341.698872900337,342.433599241288),.UNSPECIFIED.);
#4879=B_SPLINE_CURVE_WITH_KNOTS('',3,(#33777,#33778,#33779,#33780,#33781,
#33782,#33783,#33784,#33785,#33786,#33787,#33788),.UNSPECIFIED.,.F.,.F.,
(4,1,1,1,1,1,1,1,1,4),(336.150413934108,336.392868039762,336.891782118297,
337.390696196831,338.388524353899,339.386352510967,340.384180668035,341.382008825104,
342.379836982172,342.433599241288),.UNSPECIFIED.);
#4880=B_SPLINE_CURVE_WITH_KNOTS('',3,(#33793,#33794,#33795,#33796,#33797,
#33798,#33799,#33800,#33801,#33802,#33803,#33804),.UNSPECIFIED.,.F.,.F.,
(4,1,1,1,1,1,1,1,1,4),(329.867228626928,330.722763172586,331.720591329655,
332.219505408189,332.718419486723,333.217333565257,333.716247643791,334.714075800859,
335.711903957928,336.150413934108),.UNSPECIFIED.);
#4881=B_SPLINE_CURVE_WITH_KNOTS('',3,(#33805,#33806,#33807,#33808,#33809,
#33810,#33811,#33812,#33813,#33814,#33815,#33816),.UNSPECIFIED.,.F.,.F.,
(4,1,1,1,1,1,1,1,1,4),(329.867228626929,329.906985018819,330.405899097353,
331.403727254421,332.401555411489,333.399383568558,334.397211725626,335.395039882694,
335.893953961228,336.150413934108),.UNSPECIFIED.);
#4882=B_SPLINE_CURVE_WITH_KNOTS('',3,(#33821,#33822,#33823,#33824,#33825,
#33826,#33827,#33828,#33829,#33830,#33831,#33832,#33833),.UNSPECIFIED.,
 .F.,.F.,(4,1,1,1,1,1,1,1,1,1,4),(323.584043319749,323.737966073108,324.735794230177,
325.234708308711,325.733622387245,326.232536465779,326.731450544313,327.729278701381,
328.72710685845,329.724935015518,329.867228626928),.UNSPECIFIED.);
#4883=B_SPLINE_CURVE_WITH_KNOTS('',3,(#33834,#33835,#33836,#33837,#33838,
#33839,#33840,#33841,#33842,#33843,#33844),.UNSPECIFIED.,.F.,.F.,(4,1,1,
1,1,1,1,1,4),(323.584043319749,324.418930154943,325.416758312012,326.41458646908,
327.412414626148,328.410242783216,328.90915686175,329.408070940285,329.867228626929),
 .UNSPECIFIED.);
#4884=B_SPLINE_CURVE_WITH_KNOTS('',3,(#33849,#33850,#33851,#33852,#33853,
#33854,#33855,#33856,#33857,#33858,#33859,#33860),.UNSPECIFIED.,.F.,.F.,
(4,1,1,1,1,1,1,1,1,4),(317.300858012569,317.750997130699,318.249911209233,
318.748825287767,319.247739366301,319.746653444835,320.744481601904,321.742309758972,
322.74013791604,323.584043319749),.UNSPECIFIED.);
#4885=B_SPLINE_CURVE_WITH_KNOTS('',3,(#33861,#33862,#33863,#33864,#33865,
#33866,#33867,#33868,#33869,#33870,#33871,#33872,#33873,#33874,#33875,#33876,
#33877,#33878,#33879,#33880,#33881,#33882,#33883,#33884,#33885),
 .UNSPECIFIED.,.F.,.F.,(4,3,3,3,3,3,3,3,4),(317.300858012569,318.18753737543,
319.074216738291,319.960896101152,320.847575464013,321.734254826873,322.620934189734,
323.507613552595,323.584043319749),.UNSPECIFIED.);
#4886=B_SPLINE_CURVE_WITH_KNOTS('',3,(#33890,#33891,#33892,#33893,#33894,
#33895,#33896,#33897,#33898,#33899,#33900,#33901,#33902,#33903,#33904,#33905,
#33906,#33907,#33908,#33909,#33910,#33911,#33912,#33913,#33914),
 .UNSPECIFIED.,.F.,.F.,(4,3,3,3,3,3,3,3,4),(311.01767270539,311.90435206825,
312.791031431111,313.677710793972,314.564390156833,315.451069519694,316.337748882555,
317.224428245415,317.300858012569),.UNSPECIFIED.);
#4887=B_SPLINE_CURVE_WITH_KNOTS('',3,(#33915,#33916,#33917,#33918,#33919,
#33920,#33921,#33922,#33923,#33924,#33925,#33926),.UNSPECIFIED.,.F.,.F.,
(4,1,1,1,1,1,1,1,1,4),(311.01767270539,311.447164113056,312.444992270124,
313.442820427192,314.440648584261,314.939562662795,315.438476741329,315.937390819863,
316.436304898397,317.300858012569),.UNSPECIFIED.);
#4888=B_SPLINE_CURVE_WITH_KNOTS('',3,(#33931,#33932,#33933,#33934,#33935,
#33936,#33937,#33938,#33939,#33940,#33941,#33942),.UNSPECIFIED.,.F.,.F.,
(4,1,1,1,1,1,1,1,1,4),(304.73448739821,304.779231088812,305.278145167346,
305.77705924588,306.774887402948,307.772715560016,308.770543717085,309.768371874153,
310.766200031221,311.01767270539),.UNSPECIFIED.);
#4889=B_SPLINE_CURVE_WITH_KNOTS('',3,(#33943,#33944,#33945,#33946,#33947,
#33948,#33949,#33950,#33951,#33952,#33953,#33954),.UNSPECIFIED.,.F.,.F.,
(4,1,1,1,1,1,1,1,1,4),(304.73448739821,305.460195170646,306.458023327715,
307.455851484783,307.954765563317,308.453679641851,308.952593720385,309.451507798919,
310.449335955988,311.01767270539),.UNSPECIFIED.);
#4890=B_SPLINE_CURVE_WITH_KNOTS('',3,(#33959,#33960,#33961,#33962,#33963,
#33964,#33965,#33966,#33967,#33968,#33969),.UNSPECIFIED.,.F.,.F.,(4,1,1,
1,1,1,1,1,4),(298.451302091031,298.792262146402,299.79009030347,300.787918460539,
301.785746617607,302.783574774675,303.781402931743,304.280317010277,304.73448739821),
 .UNSPECIFIED.);
#4891=B_SPLINE_CURVE_WITH_KNOTS('',3,(#33970,#33971,#33972,#33973,#33974,
#33975,#33976,#33977,#33978,#33979,#33980,#33981,#33982),.UNSPECIFIED.,
 .F.,.F.,(4,1,1,1,1,1,1,1,1,1,4),(298.451302091031,298.475398071169,299.473226228237,
300.471054385305,300.969968463839,301.468882542373,301.967796620908,302.466710699442,
303.46453885651,304.462367013578,304.73448739821),.UNSPECIFIED.);
#4892=B_SPLINE_CURVE_WITH_KNOTS('',3,(#33987,#33988,#33989,#33990,#33991,
#33992,#33993,#33994,#33995,#33996,#33997,#33998,#33999,#34000,#34001,#34002,
#34003,#34004,#34005,#34006,#34007,#34008,#34009,#34010,#34011),
 .UNSPECIFIED.,.F.,.F.,(4,3,3,3,3,3,3,3,4),(292.168116783851,293.054796146712,
293.941475509573,294.828154872434,295.714834235294,296.601513598155,297.488192961016,
298.374872323877,298.451302091031),.UNSPECIFIED.);
#4893=B_SPLINE_CURVE_WITH_KNOTS('',3,(#34012,#34013,#34014,#34015,#34016,
#34017,#34018,#34019,#34020,#34021,#34022,#34023),.UNSPECIFIED.,.F.,.F.,
(4,1,1,1,1,1,1,1,1,4),(292.168116783851,292.488429128759,293.486257285827,
293.985171364361,294.484085442896,294.98299952143,295.481913599964,296.479741757032,
297.4775699141,298.451302091031),.UNSPECIFIED.);
#4894=B_SPLINE_CURVE_WITH_KNOTS('',3,(#34028,#34029,#34030,#34031,#34032,
#34033,#34034,#34035,#34036,#34037,#34038,#34039),.UNSPECIFIED.,.F.,.F.,
(4,1,1,1,1,1,1,1,1,4),(285.884931476671,286.818324261583,287.816152418651,
288.813980575719,289.811808732788,290.310722811322,290.809636889856,291.30855096839,
291.807465046924,292.168116783851),.UNSPECIFIED.);
#4895=B_SPLINE_CURVE_WITH_KNOTS('',3,(#34040,#34041,#34042,#34043,#34044,
#34045,#34046,#34047,#34048,#34049,#34050,#34051,#34052,#34053,#34054,#34055,
#34056,#34057,#34058,#34059,#34060,#34061,#34062,#34063,#34064),
 .UNSPECIFIED.,.F.,.F.,(4,3,3,3,3,3,3,3,4),(285.884931476672,286.771610839532,
287.658290202393,288.544969565254,289.431648928115,290.318328290976,291.205007653837,
292.091687016697,292.168116783851),.UNSPECIFIED.);
#4896=B_SPLINE_CURVE_WITH_KNOTS('',3,(#34069,#34070,#34071,#34072,#34073,
#34074,#34075,#34076,#34077,#34078,#34079,#34080,#34081),.UNSPECIFIED.,
 .F.,.F.,(4,1,1,1,1,1,1,1,1,1,4),(279.601746169492,279.833527162105,280.831355319173,
281.829183476242,282.82701163331,283.325925711844,283.824839790378,284.323753868912,
284.822667947446,285.820496104515,285.884931476671),.UNSPECIFIED.);
#4897=B_SPLINE_CURVE_WITH_KNOTS('',3,(#34082,#34083,#34084,#34085,#34086,
#34087,#34088,#34089,#34090,#34091,#34092,#34093),.UNSPECIFIED.,.F.,.F.,
(4,1,1,1,1,1,1,1,1,4),(279.601746169492,280.015577165406,280.51449124394,
281.013405322474,281.512319401008,282.510147558077,283.507975715145,284.505803872213,
285.503632029281,285.884931476672),.UNSPECIFIED.);
#4898=B_SPLINE_CURVE_WITH_KNOTS('',3,(#34098,#34099,#34100,#34101,#34102,
#34103,#34104,#34105,#34106,#34107,#34108,#34109),.UNSPECIFIED.,.F.,.F.,
(4,1,1,1,1,1,1,1,1,4),(273.318560862312,273.846558219696,274.844386376764,
275.842214533832,276.341128612366,276.8400426909,277.338956769435,277.837870847969,
278.835699005037,279.601746169492),.UNSPECIFIED.);
#4899=B_SPLINE_CURVE_WITH_KNOTS('',3,(#34110,#34111,#34112,#34113,#34114,
#34115,#34116,#34117,#34118,#34119,#34120,#34121),.UNSPECIFIED.,.F.,.F.,
(4,1,1,1,1,1,1,1,1,4),(273.318560862312,273.529694144462,274.028608222996,
274.52752230153,275.525350458599,276.523178615667,277.521006772735,278.518834929803,
279.516663086872,279.601746169492),.UNSPECIFIED.);
#4900=B_SPLINE_CURVE_WITH_KNOTS('',3,(#34126,#34127,#34128,#34129,#34130,
#34131,#34132,#34133,#34134,#34135,#34136,#34137),.UNSPECIFIED.,.F.,.F.,
(4,1,1,1,1,1,1,1,1,4),(267.035375555133,267.859589277286,268.857417434354,
269.356331512888,269.855245591423,270.354159669957,270.853073748491,271.850901905559,
272.848730062627,273.318560862312),.UNSPECIFIED.);
#4901=B_SPLINE_CURVE_WITH_KNOTS('',3,(#34138,#34139,#34140,#34141,#34142,
#34143,#34144,#34145,#34146,#34147,#34148,#34149),.UNSPECIFIED.,.F.,.F.,
(4,1,1,1,1,1,1,1,1,4),(267.035375555133,267.043811123519,267.542725202053,
268.540553359121,269.538381516189,270.536209673257,271.534037830326,272.531865987394,
273.030780065928,273.318560862312),.UNSPECIFIED.);
#4902=B_SPLINE_CURVE_WITH_KNOTS('',3,(#34154,#34155,#34156,#34157,#34158,
#34159,#34160,#34161,#34162,#34163,#34164,#34165,#34166),.UNSPECIFIED.,
 .F.,.F.,(4,1,1,1,1,1,1,1,1,1,4),(260.752190247953,260.874792177808,261.872620334877,
262.371534413411,262.870448491945,263.369362570479,263.868276649013,264.866104806081,
265.86393296315,266.861761120218,267.035375555133),.UNSPECIFIED.);
#4903=B_SPLINE_CURVE_WITH_KNOTS('',3,(#34167,#34168,#34169,#34170,#34171,
#34172,#34173,#34174,#34175,#34176,#34177),.UNSPECIFIED.,.F.,.F.,(4,1,1,
1,1,1,1,1,4),(260.752190247953,261.555756259643,262.553584416711,263.55141257378,
264.549240730848,265.547068887916,266.04598296645,266.544897044984,267.035375555133),
 .UNSPECIFIED.);
#4904=B_SPLINE_CURVE_WITH_KNOTS('',3,(#34182,#34183,#34184,#34185,#34186,
#34187,#34188,#34189,#34190,#34191,#34192,#34193),.UNSPECIFIED.,.F.,.F.,
(4,1,1,1,1,1,1,1,1,4),(254.469004940774,254.887823235399,255.386737313933,
255.885651392467,256.384565471001,256.883479549535,257.881307706603,258.879135863672,
259.87696402074,260.752190247953),.UNSPECIFIED.);
#4905=B_SPLINE_CURVE_WITH_KNOTS('',3,(#34194,#34195,#34196,#34197,#34198,
#34199,#34200,#34201,#34202,#34203,#34204,#34205,#34206,#34207,#34208,#34209,
#34210,#34211,#34212,#34213,#34214,#34215,#34216,#34217,#34218),
 .UNSPECIFIED.,.F.,.F.,(4,3,3,3,3,3,3,3,4),(254.469004940774,255.355684303635,
256.242363666495,257.129043029356,258.015722392217,258.902401755078,259.789081117939,
260.6757604808,260.752190247953),.UNSPECIFIED.);
#4906=B_SPLINE_CURVE_WITH_KNOTS('',3,(#34223,#34224,#34225,#34226,#34227,
#34228,#34229,#34230,#34231,#34232,#34233,#34234,#34235,#34236,#34237,#34238,
#34239,#34240,#34241,#34242,#34243,#34244,#34245,#34246,#34247),
 .UNSPECIFIED.,.F.,.F.,(4,3,3,3,3,3,3,3,4),(248.185819633594,249.072498996455,
249.959178359316,250.845857722176,251.732537085037,252.619216447898,253.505895810759,
254.392575173619,254.469004940774),.UNSPECIFIED.);
#4907=B_SPLINE_CURVE_WITH_KNOTS('',3,(#34248,#34249,#34250,#34251,#34252,
#34253,#34254,#34255,#34256,#34257,#34258,#34259),.UNSPECIFIED.,.F.,.F.,
(4,1,1,1,1,1,1,1,1,4),(248.185819633594,248.583990217756,249.581818374824,
250.579646531892,251.577474688961,252.076388767495,252.575302846029,253.074216924563,
253.573131003097,254.469004940774),.UNSPECIFIED.);
#4908=B_SPLINE_CURVE_WITH_KNOTS('',3,(#34264,#34265,#34266,#34267,#34268,
#34269,#34270,#34271,#34272,#34273,#34274,#34275),.UNSPECIFIED.,.F.,.F.,
(4,1,1,1,1,1,1,1,1,4),(241.902634326414,241.916057193511,242.414971272045,
242.91388535058,243.911713507648,244.909541664716,245.907369821784,246.905197978853,
247.903026135921,248.185819633594),.UNSPECIFIED.);
#4909=B_SPLINE_CURVE_WITH_KNOTS('',3,(#34276,#34277,#34278,#34279,#34280,
#34281,#34282,#34283,#34284,#34285,#34286,#34287),.UNSPECIFIED.,.F.,.F.,
(4,1,1,1,1,1,1,1,1,4),(241.902634326415,242.597021275346,243.594849432414,
244.592677589483,245.091591668017,245.590505746551,246.089419825085,246.588333903619,
247.586162060688,248.185819633594),.UNSPECIFIED.);
#4910=B_SPLINE_CURVE_WITH_KNOTS('',3,(#34292,#34293,#34294,#34295,#34296,
#34297,#34298,#34299,#34300,#34301,#34302),.UNSPECIFIED.,.F.,.F.,(4,1,1,
1,1,1,1,1,4),(235.619449019235,235.929088251102,236.92691640817,237.924744565238,
238.922572722307,239.920400879375,240.918229036443,241.417143114977,241.902634326414),
 .UNSPECIFIED.);
#4911=B_SPLINE_CURVE_WITH_KNOTS('',3,(#34303,#34304,#34305,#34306,#34307,
#34308,#34309,#34310,#34311,#34312,#34313,#34314),.UNSPECIFIED.,.F.,.F.,
(4,1,1,1,1,1,1,1,1,4),(235.619449019235,236.610052332937,237.607880490005,
238.106794568539,238.605708647073,239.104622725607,239.603536804141,240.60136496121,
241.599193118278,241.902634326415),.UNSPECIFIED.);
#4912=B_SPLINE_CURVE_WITH_KNOTS('',3,(#34319,#34320,#34321,#34322,#34323,
#34324,#34325,#34326,#34327,#34328,#34329,#34330,#34331,#34332,#34333,#34334,
#34335,#34336,#34337,#34338,#34339,#34340,#34341,#34342,#34343),
 .UNSPECIFIED.,.F.,.F.,(4,3,3,3,3,3,3,3,4),(229.336263712055,230.222943074916,
231.109622437777,231.996301800638,232.882981163499,233.769660526359,234.65633988922,
235.543019252081,235.619449019235),.UNSPECIFIED.);
#4913=B_SPLINE_CURVE_WITH_KNOTS('',3,(#34344,#34345,#34346,#34347,#34348,
#34349,#34350,#34351,#34352,#34353,#34354,#34355,#34356),.UNSPECIFIED.,
 .F.,.F.,(4,1,1,1,1,1,1,1,1,1,4),(229.336263712055,229.625255233459,230.623083390527,
231.121997469061,231.620911547595,232.11982562613,232.618739704664,233.616567861732,
234.6143960188,235.612224175868,235.619449019235),.UNSPECIFIED.);
#4914=B_SPLINE_CURVE_WITH_KNOTS('',3,(#34361,#34362,#34363,#34364,#34365,
#34366,#34367,#34368,#34369,#34370,#34371,#34372),.UNSPECIFIED.,.F.,.F.,
(4,1,1,1,1,1,1,1,1,4),(223.053078404876,223.955150366283,224.952978523351,
225.950806680419,226.948634837488,227.447548916022,227.946462994556,228.44537707309,
228.944291151624,229.336263712055),.UNSPECIFIED.);
#4915=B_SPLINE_CURVE_WITH_KNOTS('',3,(#34373,#34374,#34375,#34376,#34377,
#34378,#34379,#34380,#34381,#34382,#34383,#34384,#34385,#34386,#34387,#34388,
#34389,#34390,#34391,#34392,#34393,#34394,#34395,#34396,#34397),
 .UNSPECIFIED.,.F.,.F.,(4,3,3,3,3,3,3,3,4),(223.053078404876,223.939757767737,
224.826437130597,225.713116493458,226.599795856319,227.48647521918,228.373154582041,
229.259833944901,229.336263712055),.UNSPECIFIED.);
#4916=B_SPLINE_CURVE_WITH_KNOTS('',3,(#34402,#34403,#34404,#34405,#34406,
#34407,#34408,#34409,#34410,#34411,#34412,#34413,#34414),.UNSPECIFIED.,
 .F.,.F.,(4,1,1,1,1,1,1,1,1,1,4),(216.769893097696,216.970353266805,217.968181423873,
218.966009580941,219.96383773801,220.462751816544,220.961665895078,221.460579973612,
221.959494052146,222.957322209214,223.053078404876),.UNSPECIFIED.);
#4917=B_SPLINE_CURVE_WITH_KNOTS('',3,(#34415,#34416,#34417,#34418,#34419,
#34420,#34421,#34422,#34423,#34424,#34425,#34426),.UNSPECIFIED.,.F.,.F.,
(4,1,1,1,1,1,1,1,1,4),(216.769893097696,217.152403270106,217.65131734864,
218.150231427174,218.649145505708,219.646973662776,220.644801819845,221.642629976913,
222.640458133981,223.053078404876),.UNSPECIFIED.);
#4918=B_SPLINE_CURVE_WITH_KNOTS('',3,(#34431,#34432,#34433,#34434,#34435,
#34436,#34437,#34438,#34439,#34440,#34441),.UNSPECIFIED.,.F.,.F.,(4,1,1,
1,1,1,1,1,4),(210.486707790517,210.983384324395,211.981212481464,212.979040638532,
213.9768687956,214.974696952668,215.972525109737,216.471439188271,216.769893097696),
 .UNSPECIFIED.);
#4919=B_SPLINE_CURVE_WITH_KNOTS('',3,(#34442,#34443,#34444,#34445,#34446,
#34447,#34448,#34449,#34450,#34451,#34452,#34453),.UNSPECIFIED.,.F.,.F.,
(4,1,1,1,1,1,1,1,1,4),(210.486707790517,210.666520249162,211.66434840623,
212.662176563298,213.161090641833,213.660004720367,214.657832877435,215.655661034503,
216.653489191572,216.769893097696),.UNSPECIFIED.);
#4920=B_SPLINE_CURVE_WITH_KNOTS('',3,(#34458,#34459,#34460,#34461,#34462,
#34463,#34464,#34465,#34466,#34467,#34468,#34469,#34470,#34471,#34472,#34473,
#34474,#34475,#34476,#34477,#34478,#34479,#34480,#34481,#34482),
 .UNSPECIFIED.,.F.,.F.,(4,3,3,3,3,3,3,3,4),(204.203522483337,205.090201846198,
205.976881209059,206.86356057192,207.75023993478,208.636919297641,209.523598660502,
210.410278023363,210.486707790517),.UNSPECIFIED.);
#4921=B_SPLINE_CURVE_WITH_KNOTS('',3,(#34483,#34484,#34485,#34486,#34487,
#34488,#34489,#34490,#34491,#34492,#34493,#34494),.UNSPECIFIED.,.F.,.F.,
(4,1,1,1,1,1,1,1,1,4),(204.203522483337,204.679551306752,205.178465385287,
205.677379463821,206.176293542355,206.675207620889,207.673035777957,208.670863935025,
209.668692092094,210.486707790517),.UNSPECIFIED.);
#4922=B_SPLINE_CURVE_WITH_KNOTS('',3,(#34499,#34500,#34501,#34502,#34503,
#34504,#34505,#34506,#34507,#34508,#34509,#34510,#34511),.UNSPECIFIED.,
 .F.,.F.,(4,1,1,1,1,1,1,1,1,1,4),(197.920337176158,198.011618282508,199.009446439576,
200.007274596645,201.005102753713,201.504016832247,202.002930910781,202.501844989315,
203.000759067849,203.998587224918,204.203522483337),.UNSPECIFIED.);
#4923=B_SPLINE_CURVE_WITH_KNOTS('',3,(#34512,#34513,#34514,#34515,#34516,
#34517,#34518,#34519,#34520,#34521,#34522,#34523,#34524,#34525,#34526,#34527,
#34528,#34529,#34530,#34531,#34532,#34533,#34534,#34535,#34536),
 .UNSPECIFIED.,.F.,.F.,(4,3,3,3,3,3,3,3,4),(197.920337176158,198.807016539019,
199.693695901879,200.58037526474,201.467054627601,202.353733990462,203.240413353323,
204.127092716184,204.203522483337),.UNSPECIFIED.);
#4924=B_SPLINE_CURVE_WITH_KNOTS('',3,(#34541,#34542,#34543,#34544,#34545,
#34546,#34547,#34548,#34549,#34550,#34551,#34552),.UNSPECIFIED.,.F.,.F.,
(4,1,1,1,1,1,1,1,1,4),(191.637151868978,192.024649340099,193.022477497167,
194.020305654235,194.519219732769,195.018133811303,195.517047889837,196.015961968372,
197.01379012544,197.920337176158),.UNSPECIFIED.);
#4925=B_SPLINE_CURVE_WITH_KNOTS('',3,(#34553,#34554,#34555,#34556,#34557,
#34558,#34559,#34560,#34561,#34562,#34563,#34564),.UNSPECIFIED.,.F.,.F.,
(4,1,1,1,1,1,1,1,1,4),(191.637151868978,191.707785264865,192.206699343399,
192.705613421933,193.703441579002,194.70126973607,195.699097893138,196.696926050206,
197.694754207275,197.920337176158),.UNSPECIFIED.);
#4926=B_SPLINE_CURVE_WITH_KNOTS('',3,(#34569,#34570,#34571,#34572,#34573,
#34574,#34575,#34576,#34577,#34578,#34579,#34580),.UNSPECIFIED.,.F.,.F.,
(4,1,1,1,1,1,1,1,1,4),(185.353966561798,186.037680397689,187.035508554757,
187.534422633291,188.033336711825,188.53225079036,189.031164868894,190.028993025962,
191.02682118303,191.637151868978),.UNSPECIFIED.);
#4927=B_SPLINE_CURVE_WITH_KNOTS('',3,(#34581,#34582,#34583,#34584,#34585,
#34586,#34587,#34588,#34589,#34590,#34591),.UNSPECIFIED.,.F.,.F.,(4,1,1,
1,1,1,1,1,4),(185.353966561799,185.720816322456,186.718644479524,187.716472636592,
188.71430079366,189.712128950729,190.709957107797,191.208871186331,191.637151868978),
 .UNSPECIFIED.);
#4928=B_SPLINE_CURVE_WITH_KNOTS('',3,(#34596,#34597,#34598,#34599,#34600,
#34601,#34602,#34603,#34604,#34605,#34606,#34607),.UNSPECIFIED.,.F.,.F.,
(4,1,1,1,1,1,1,1,1,4),(179.070781254619,180.050711455279,180.549625533814,
181.048539612348,181.547453690882,182.046367769416,183.044195926484,184.042024083552,
185.039852240621,185.353966561798),.UNSPECIFIED.);
#4929=B_SPLINE_CURVE_WITH_KNOTS('',3,(#34608,#34609,#34610,#34611,#34612,
#34613,#34614,#34615,#34616,#34617,#34618,#34619,#34620,#34621,#34622,#34623,
#34624,#34625,#34626,#34627,#34628,#34629,#34630,#34631,#34632),
 .UNSPECIFIED.,.F.,.F.,(4,3,3,3,3,3,3,3,4),(179.070781254619,179.95746061748,
180.844139980341,181.730819343202,182.617498706062,183.504178068923,184.390857431784,
185.277536794645,185.353966561799),.UNSPECIFIED.);
#4930=B_SPLINE_CURVE_WITH_KNOTS('',3,(#34637,#34638,#34639,#34640,#34641,
#34642,#34643,#34644,#34645,#34646,#34647,#34648,#34649),.UNSPECIFIED.,
 .F.,.F.,(4,1,1,1,1,1,1,1,1,1,4),(172.787595947439,173.065914355802,173.564828434336,
174.06374251287,174.562656591404,175.061570669938,176.059398827006,177.057226984075,
178.055055141143,179.052883298211,179.070781254619),.UNSPECIFIED.);
#4931=B_SPLINE_CURVE_WITH_KNOTS('',3,(#34650,#34651,#34652,#34653,#34654,
#34655,#34656,#34657,#34658,#34659,#34660,#34661),.UNSPECIFIED.,.F.,.F.,
(4,1,1,1,1,1,1,1,1,4),(172.787595947439,173.746878437636,174.744706594705,
175.742534751773,176.740362908841,177.239276987375,177.738191065909,178.237105144444,
178.736019222978,179.070781254619),.UNSPECIFIED.);
#4932=B_SPLINE_CURVE_WITH_KNOTS('',3,(#34666,#34667,#34668,#34669,#34670,
#34671,#34672,#34673,#34674,#34675,#34676,#34677,#34678,#34679,#34680,#34681,
#34682,#34683,#34684,#34685,#34686,#34687,#34688,#34689,#34690),
 .UNSPECIFIED.,.F.,.F.,(4,3,3,3,3,3,3,3,4),(166.50441064026,167.391090003121,
168.277769365981,169.164448728842,170.051128091703,170.937807454564,171.824486817425,
172.711166180286,172.787595947439),.UNSPECIFIED.);
#4933=B_SPLINE_CURVE_WITH_KNOTS('',3,(#34691,#34692,#34693,#34694,#34695,
#34696,#34697,#34698,#34699,#34700,#34701,#34702,#34703),.UNSPECIFIED.,
 .F.,.F.,(4,1,1,1,1,1,1,1,1,1,4),(166.50441064026,166.762081338159,167.759909495227,
168.757737652295,169.755565809363,170.254479887898,170.753393966432,171.252308044966,
171.7512221235,172.749050280568,172.787595947439),.UNSPECIFIED.);
#4934=B_SPLINE_CURVE_WITH_KNOTS('',3,(#34708,#34709,#34710,#34711,#34712,
#34713,#34714,#34715,#34716,#34717,#34718),.UNSPECIFIED.,.F.,.F.,(4,1,1,
1,1,1,1,1,4),(160.22122533308,160.593062392448,161.091976470983,162.089804628051,
163.087632785119,164.085460942187,165.083289099256,166.081117256324,166.50441064026),
 .UNSPECIFIED.);
#4935=B_SPLINE_CURVE_WITH_KNOTS('',3,(#34719,#34720,#34721,#34722,#34723,
#34724,#34725,#34726,#34727,#34728,#34729,#34730),.UNSPECIFIED.,.F.,.F.,
(4,1,1,1,1,1,1,1,1,4),(160.22122533308,160.775112395749,161.772940552817,
162.770768709886,163.26968278842,163.768596866954,164.267510945488,164.766425024022,
165.76425318109,166.50441064026),.UNSPECIFIED.);
#4936=B_SPLINE_CURVE_WITH_KNOTS('',3,(#34735,#34736,#34737,#34738,#34739,
#34740,#34741,#34742,#34743,#34744,#34745,#34746,#34747,#34748,#34749,#34750,
#34751,#34752,#34753,#34754,#34755,#34756,#34757,#34758,#34759),
 .UNSPECIFIED.,.F.,.F.,(4,3,3,3,3,3,3,3,4),(153.938040025901,154.824719388761,
155.711398751622,156.598078114483,157.484757477344,158.371436840205,159.258116203066,
160.144795565927,160.22122533308),.UNSPECIFIED.);
#4937=B_SPLINE_CURVE_WITH_KNOTS('',3,(#34760,#34761,#34762,#34763,#34764,
#34765,#34766,#34767,#34768,#34769,#34770,#34771),.UNSPECIFIED.,.F.,.F.,
(4,1,1,1,1,1,1,1,1,4),(153.938040025901,154.78814345334,155.785971610408,
156.284885688942,156.783799767476,157.28271384601,157.781627924544,158.779456081613,
159.777284238681,160.22122533308),.UNSPECIFIED.);
#4938=B_SPLINE_CURVE_WITH_KNOTS('',3,(#34776,#34777,#34778,#34779,#34780,
#34781,#34782,#34783,#34784,#34785,#34786,#34787),.UNSPECIFIED.,.F.,.F.,
(4,1,1,1,1,1,1,1,1,4),(147.654854718721,148.120210429095,149.118038586163,
150.115866743232,151.1136949003,152.111523057368,152.610437135902,153.109351214436,
153.608265292971,153.938040025901),.UNSPECIFIED.);
#4939=B_SPLINE_CURVE_WITH_KNOTS('',3,(#34788,#34789,#34790,#34791,#34792,
#34793,#34794,#34795,#34796,#34797,#34798,#34799,#34800),.UNSPECIFIED.,
 .F.,.F.,(4,1,1,1,1,1,1,1,1,1,4),(147.654854718721,147.803346353862,148.80117451093,
149.300088589464,149.799002667998,150.297916746532,150.796830825067,151.794658982135,
152.792487139203,153.790315296271,153.938040025901),.UNSPECIFIED.);
#4940=B_SPLINE_CURVE_WITH_KNOTS('',3,(#34805,#34806,#34807,#34808,#34809,
#34810,#34811,#34812,#34813,#34814,#34815,#34816,#34817,#34818,#34819,#34820,
#34821,#34822,#34823,#34824,#34825,#34826,#34827,#34828,#34829),
 .UNSPECIFIED.,.F.,.F.,(4,3,3,3,3,3,3,3,4),(141.371669411541,142.258348774402,
143.145028137263,144.031707500124,144.918386862985,145.805066225846,146.691745588707,
147.578424951567,147.654854718721),.UNSPECIFIED.);
#4941=B_SPLINE_CURVE_WITH_KNOTS('',3,(#34830,#34831,#34832,#34833,#34834,
#34835,#34836,#34837,#34838,#34839,#34840,#34841),.UNSPECIFIED.,.F.,.F.,
(4,1,1,1,1,1,1,1,1,4),(141.371669411542,141.816377411452,142.315291489986,
142.81420556852,143.313119647055,143.812033725589,144.809861882657,145.807690039725,
146.805518196793,147.654854718721),.UNSPECIFIED.);
#4942=B_SPLINE_CURVE_WITH_KNOTS('',3,(#34846,#34847,#34848,#34849,#34850,
#34851,#34852,#34853,#34854,#34855,#34856,#34857,#34858),.UNSPECIFIED.,
 .F.,.F.,(4,1,1,1,1,1,1,1,1,1,4),(135.088484104362,135.148444387208,136.146272544276,
137.144100701344,138.141928858413,138.640842936947,139.139757015481,139.638671094015,
140.137585172549,141.135413329617,141.371669411541),.UNSPECIFIED.);
#4943=B_SPLINE_CURVE_WITH_KNOTS('',3,(#34859,#34860,#34861,#34862,#34863,
#34864,#34865,#34866,#34867,#34868,#34869,#34870,#34871,#34872,#34873,#34874,
#34875,#34876,#34877,#34878,#34879,#34880,#34881,#34882,#34883),
 .UNSPECIFIED.,.F.,.F.,(4,3,3,3,3,3,3,3,4),(135.088484104362,135.975163467223,
136.861842830084,137.748522192945,138.635201555806,139.521880918667,140.408560281528,
141.295239644388,141.371669411542),.UNSPECIFIED.);
#4944=B_SPLINE_CURVE_WITH_KNOTS('',3,(#34888,#34889,#34890,#34891,#34892,
#34893,#34894,#34895,#34896,#34897,#34898,#34899),.UNSPECIFIED.,.F.,.F.,
(4,1,1,1,1,1,1,1,1,4),(128.805298797182,129.161475444798,130.159303601867,
131.157131758935,131.656045837469,132.154959916003,132.653873994537,133.152788073071,
134.15061623014,135.088484104362),.UNSPECIFIED.);
#4945=B_SPLINE_CURVE_WITH_KNOTS('',3,(#34900,#34901,#34902,#34903,#34904,
#34905,#34906,#34907,#34908,#34909,#34910,#34911),.UNSPECIFIED.,.F.,.F.,
(4,1,1,1,1,1,1,1,1,4),(128.805298797182,128.844611369565,129.343525448099,
129.842439526633,130.840267683701,131.83809584077,132.835923997838,133.833752154906,
134.831580311974,135.088484104362),.UNSPECIFIED.);
#4946=B_SPLINE_CURVE_WITH_KNOTS('',3,(#34916,#34917,#34918,#34919,#34920,
#34921,#34922,#34923,#34924,#34925,#34926,#34927),.UNSPECIFIED.,.F.,.F.,
(4,1,1,1,1,1,1,1,1,4),(122.522113490003,123.174506502389,124.172334659457,
124.671248737991,125.170162816525,125.669076895059,126.167990973594,127.165819130662,
128.16364728773,128.805298797182),.UNSPECIFIED.);
#4947=B_SPLINE_CURVE_WITH_KNOTS('',3,(#34928,#34929,#34930,#34931,#34932,
#34933,#34934,#34935,#34936,#34937,#34938),.UNSPECIFIED.,.F.,.F.,(4,1,1,
1,1,1,1,1,4),(122.522113490003,122.857642427155,123.855470584224,124.853298741292,
125.85112689836,126.848955055428,127.846783212497,128.345697291031,128.805298797182),
 .UNSPECIFIED.);
#4948=B_SPLINE_CURVE_WITH_KNOTS('',3,(#34943,#34944,#34945,#34946,#34947,
#34948,#34949,#34950,#34951,#34952,#34953,#34954),.UNSPECIFIED.,.F.,.F.,
(4,1,1,1,1,1,1,1,1,4),(116.238928182823,117.187537559979,117.686451638513,
118.185365717047,118.684279795582,119.183193874116,120.181022031184,121.178850188252,
122.17667834532,122.522113490003),.UNSPECIFIED.);
#4949=B_SPLINE_CURVE_WITH_KNOTS('',3,(#34955,#34956,#34957,#34958,#34959,
#34960,#34961,#34962,#34963,#34964,#34965,#34966,#34967,#34968,#34969,#34970,
#34971,#34972,#34973,#34974,#34975,#34976,#34977,#34978,#34979),
 .UNSPECIFIED.,.F.,.F.,(4,3,3,3,3,3,3,3,4),(116.238928182823,117.125607545684,
118.012286908545,118.898966271406,119.785645634267,120.672324997128,121.559004359989,
122.445683722849,122.522113490003),.UNSPECIFIED.);
#4950=B_SPLINE_CURVE_WITH_KNOTS('',3,(#34984,#34985,#34986,#34987,#34988,
#34989,#34990,#34991,#34992,#34993,#34994,#34995,#34996),.UNSPECIFIED.,
 .F.,.F.,(4,1,1,1,1,1,1,1,1,1,4),(109.955742875644,110.202740460501,110.701654539036,
111.20056861757,111.699482696104,112.198396774638,113.196224931706,114.194053088774,
115.191881245843,116.189709402911,116.238928182823),.UNSPECIFIED.);
#4951=B_SPLINE_CURVE_WITH_KNOTS('',3,(#34997,#34998,#34999,#35000,#35001,
#35002,#35003,#35004,#35005,#35006,#35007,#35008),.UNSPECIFIED.,.F.,.F.,
(4,1,1,1,1,1,1,1,1,4),(109.955742875644,110.883704542336,111.881532699404,
112.879360856473,113.877189013541,114.376103092075,114.875017170609,115.373931249143,
115.872845327677,116.238928182823),.UNSPECIFIED.);
#4952=B_SPLINE_CURVE_WITH_KNOTS('',3,(#35013,#35014,#35015,#35016,#35017,
#35018,#35019,#35020,#35021,#35022,#35023,#35024),.UNSPECIFIED.,.F.,.F.,
(4,1,1,1,1,1,1,1,1,4),(103.672557568464,103.716857439558,104.215771518092,
104.714685596626,105.21359967516,106.211427832228,107.209255989297,108.207084146365,
109.204912303433,109.955742875644),.UNSPECIFIED.);
#4953=B_SPLINE_CURVE_WITH_KNOTS('',3,(#35025,#35026,#35027,#35028,#35029,
#35030,#35031,#35032,#35033,#35034,#35035,#35036,#35037),.UNSPECIFIED.,
 .F.,.F.,(4,1,1,1,1,1,1,1,1,1,4),(103.672557568464,103.898907442858,104.896735599927,
105.894563756995,106.892391914063,107.391305992597,107.890220071131,108.389134149666,
108.8880482282,109.885876385268,109.955742875644),.UNSPECIFIED.);
#4954=B_SPLINE_CURVE_WITH_KNOTS('',3,(#35042,#35043,#35044,#35045,#35046,
#35047,#35048,#35049,#35050,#35051,#35052),.UNSPECIFIED.,.F.,.F.,(4,1,1,
1,1,1,1,1,4),(97.3893722612844,97.7298884971482,98.2288025756823,99.2266307327506,
100.224458889819,101.222287046887,102.220115203955,103.217943361024,103.672557568464),
 .UNSPECIFIED.);
#4955=B_SPLINE_CURVE_WITH_KNOTS('',3,(#35053,#35054,#35055,#35056,#35057,
#35058,#35059,#35060,#35061,#35062,#35063,#35064),.UNSPECIFIED.,.F.,.F.,
(4,1,1,1,1,1,1,1,1,4),(97.3893722612845,97.9119385004489,98.9097666575171,
99.9075948145854,100.406508893119,100.905422971654,101.404337050188,101.903251128722,
102.90107928579,103.672557568464),.UNSPECIFIED.);
#4956=B_SPLINE_CURVE_WITH_KNOTS('',3,(#35069,#35070,#35071,#35072,#35073,
#35074,#35075,#35076,#35077,#35078,#35079,#35080,#35081,#35082,#35083,#35084,
#35085,#35086,#35087,#35088,#35089,#35090,#35091,#35092,#35093),
 .UNSPECIFIED.,.F.,.F.,(4,3,3,3,3,3,3,3,4),(91.1061869541048,91.9928663169656,
92.8795456798265,93.7662250426873,94.6529044055482,95.539583768409,96.4262631312698,
97.3129424941307,97.3893722612844),.UNSPECIFIED.);
#4957=B_SPLINE_CURVE_WITH_KNOTS('',3,(#35094,#35095,#35096,#35097,#35098,
#35099,#35100,#35101,#35102,#35103,#35104,#35105),.UNSPECIFIED.,.F.,.F.,
(4,1,1,1,1,1,1,1,1,4),(91.1061869541048,91.9249695580393,92.9227977151076,
93.4217117936417,93.9206258721758,94.4195399507099,94.9184540292441,95.9162821863123,
96.9141103433806,97.3893722612845),.UNSPECIFIED.);
#4958=B_SPLINE_CURVE_WITH_KNOTS('',3,(#35110,#35111,#35112,#35113,#35114,
#35115,#35116,#35117,#35118,#35119,#35120,#35121),.UNSPECIFIED.,.F.,.F.,
(4,1,1,1,1,1,1,1,1,4),(84.8230016469252,85.257036533795,86.2548646908632,
87.2526928479315,88.2505210049997,89.248349162068,89.7472632406021,90.2461773191363,
90.7450913976704,91.1061869541048),.UNSPECIFIED.);
#4959=B_SPLINE_CURVE_WITH_KNOTS('',3,(#35122,#35123,#35124,#35125,#35126,
#35127,#35128,#35129,#35130,#35131,#35132,#35133,#35134),.UNSPECIFIED.,
 .F.,.F.,(4,1,1,1,1,1,1,1,1,1,4),(84.8230016469253,84.9401724585615,85.9380006156298,
86.4369146941639,86.935828772698,87.4347428512321,87.9336569297663,88.9314850868345,
89.9293132439028,90.927141400971,91.1061869541048),.UNSPECIFIED.);
#4960=B_SPLINE_CURVE_WITH_KNOTS('',3,(#35139,#35140,#35141,#35142,#35143,
#35144,#35145,#35146,#35147,#35148,#35149,#35150,#35151,#35152,#35153,#35154,
#35155,#35156,#35157,#35158,#35159,#35160,#35161,#35162,#35163),
 .UNSPECIFIED.,.F.,.F.,(4,3,3,3,3,3,3,3,4),(78.5398163397456,79.4264957026064,
80.3131750654673,81.1998544283281,82.086533791189,82.9732131540499,83.8598925169107,
84.7465718797716,84.8230016469252),.UNSPECIFIED.);
#4961=B_SPLINE_CURVE_WITH_KNOTS('',3,(#35164,#35165,#35166,#35167,#35168,
#35169,#35170,#35171,#35172,#35173,#35174,#35175),.UNSPECIFIED.,.F.,.F.,
(4,1,1,1,1,1,1,1,1,4),(78.5398163397457,78.953203516152,79.4521175946861,
79.9510316732202,80.4499457517543,80.9488598302885,81.9466879873567,82.944516144425,
83.9423443014932,84.8230016469253),.UNSPECIFIED.);
#4962=B_SPLINE_CURVE_WITH_KNOTS('',3,(#35180,#35181,#35182,#35183,#35184,
#35185,#35186,#35187,#35188,#35189,#35190,#35191,#35192),.UNSPECIFIED.,
 .F.,.F.,(4,1,1,1,1,1,1,1,1,1,4),(72.256631032566,72.2852704919076,73.2830986489759,
74.2809268060441,75.2787549631124,75.7776690416465,76.2765831201806,76.7754971987148,
77.2744112772489,78.2722394343172,78.5398163397456),.UNSPECIFIED.);
#4963=B_SPLINE_CURVE_WITH_KNOTS('',3,(#35193,#35194,#35195,#35196,#35197,
#35198,#35199,#35200,#35201,#35202,#35203,#35204,#35205,#35206,#35207,#35208,
#35209,#35210,#35211,#35212,#35213,#35214,#35215,#35216,#35217),
 .UNSPECIFIED.,.F.,.F.,(4,3,3,3,3,3,3,3,4),(72.2566310325661,73.143310395427,
74.0299897582878,74.9166691211487,75.8033484840095,76.6900278468704,77.5767072097313,
78.4633865725921,78.5398163397457),.UNSPECIFIED.);
#4964=B_SPLINE_CURVE_WITH_KNOTS('',3,(#35222,#35223,#35224,#35225,#35226,
#35227,#35228,#35229,#35230,#35231,#35232,#35233),.UNSPECIFIED.,.F.,.F.,
(4,1,1,1,1,1,1,1,1,4),(65.9734457253864,66.2983015494981,67.2961297065663,
68.2939578636346,68.7928719421687,69.2917860207028,69.790700099237,70.2896141777711,
71.2874423348394,72.256631032566),.UNSPECIFIED.);
#4965=B_SPLINE_CURVE_WITH_KNOTS('',3,(#35234,#35235,#35236,#35237,#35238,
#35239,#35240,#35241,#35242,#35243,#35244,#35245),.UNSPECIFIED.,.F.,.F.,
(4,1,1,1,1,1,1,1,1,4),(65.9734457253865,65.9814374742646,66.4803515527987,
66.9792656313329,67.9770937884011,68.9749219454694,69.9727501025376,70.9705782596059,
71.9684064166742,72.2566310325661),.UNSPECIFIED.);
#4966=B_SPLINE_CURVE_WITH_KNOTS('',3,(#35250,#35251,#35252,#35253,#35254,
#35255,#35256,#35257,#35258,#35259,#35260,#35261),.UNSPECIFIED.,.F.,.F.,
(4,1,1,1,1,1,1,1,1,4),(59.6902604182068,60.3113326070885,61.3091607641568,
61.8080748426909,62.306988921225,62.8059029997592,63.3048170782933,64.3026452353616,
65.3004733924298,65.9734457253864),.UNSPECIFIED.);
#4967=B_SPLINE_CURVE_WITH_KNOTS('',3,(#35262,#35263,#35264,#35265,#35266,
#35267,#35268,#35269,#35270,#35271,#35272),.UNSPECIFIED.,.F.,.F.,(4,1,1,
1,1,1,1,1,4),(59.6902604182069,59.9944685318551,60.9922966889233,61.9901248459916,
62.9879530030598,63.9857811601281,64.9836093171964,65.4825233957305,65.9734457253865),
 .UNSPECIFIED.);
#4968=B_SPLINE_CURVE_WITH_KNOTS('',3,(#35277,#35278,#35279,#35280,#35281,
#35282,#35283,#35284,#35285,#35286,#35287,#35288),.UNSPECIFIED.,.F.,.F.,
(4,1,1,1,1,1,1,1,1,4),(53.4070751110272,54.324363664679,54.8232777432131,
55.3221918217472,55.8211059002814,56.3200199788155,57.3178481358838,58.315676292952,
59.3135044500203,59.6902604182068),.UNSPECIFIED.);
#4969=B_SPLINE_CURVE_WITH_KNOTS('',3,(#35289,#35290,#35291,#35292,#35293,
#35294,#35295,#35296,#35297,#35298,#35299,#35300,#35301,#35302,#35303,#35304,
#35305,#35306,#35307,#35308,#35309,#35310,#35311,#35312,#35313),
 .UNSPECIFIED.,.F.,.F.,(4,3,3,3,3,3,3,3,4),(53.4070751110273,54.2937544738882,
55.180433836749,56.0671131996099,56.9537925624707,57.8404719253316,58.7271512881924,
59.6138306510532,59.6902604182069),.UNSPECIFIED.);
#4970=B_SPLINE_CURVE_WITH_KNOTS('',3,(#35318,#35319,#35320,#35321,#35322,
#35323,#35324,#35325,#35326,#35327,#35328,#35329,#35330),.UNSPECIFIED.,
 .F.,.F.,(4,1,1,1,1,1,1,1,1,1,4),(47.1238898038476,47.3395665652012,47.8384806437353,
48.3373947222694,48.8363088008036,49.3352228793377,50.333051036406,51.3308791934742,
52.3287073505425,53.3265355076107,53.4070751110272),.UNSPECIFIED.);
#4971=B_SPLINE_CURVE_WITH_KNOTS('',3,(#35331,#35332,#35333,#35334,#35335,
#35336,#35337,#35338,#35339,#35340,#35341,#35342),.UNSPECIFIED.,.F.,.F.,
(4,1,1,1,1,1,1,1,1,4),(47.1238898038477,48.020530647036,49.0183588041042,
50.0161869611725,51.0140151182407,51.5129291967749,52.011843275309,52.5107573538431,
53.0096714323773,53.4070751110273),.UNSPECIFIED.);
#4972=B_SPLINE_CURVE_WITH_KNOTS('',3,(#35347,#35348,#35349,#35350,#35351,
#35352,#35353,#35354,#35355,#35356,#35357,#35358),.UNSPECIFIED.,.F.,.F.,
(4,1,1,1,1,1,1,1,1,4),(40.840704496668,40.8536835442575,41.3525976227916,
41.8515117013258,42.3504257798599,43.3482539369282,44.3460820939964,45.3439102510647,
46.3417384081329,47.1238898038476),.UNSPECIFIED.);
#4973=B_SPLINE_CURVE_WITH_KNOTS('',3,(#35359,#35360,#35361,#35362,#35363,
#35364,#35365,#35366,#35367,#35368,#35369,#35370,#35371),.UNSPECIFIED.,
 .F.,.F.,(4,1,1,1,1,1,1,1,1,1,4),(40.8407044966681,41.0357335475582,42.0335617046264,
43.0313898616947,44.0292180187629,44.5281320972971,45.0270461758312,45.5259602543653,
46.0248743328995,47.0227024899677,47.1238898038477),.UNSPECIFIED.);
#4974=B_SPLINE_CURVE_WITH_KNOTS('',3,(#35376,#35377,#35378,#35379,#35380,
#35381,#35382,#35383,#35384,#35385,#35386),.UNSPECIFIED.,.F.,.F.,(4,1,1,
1,1,1,1,1,4),(34.5575191894884,34.866714601848,35.3656286803821,36.3634568374504,
37.3612849945186,38.3591131515869,39.3569413086551,40.3547694657234,40.840704496668),
 .UNSPECIFIED.);
#4975=B_SPLINE_CURVE_WITH_KNOTS('',3,(#35387,#35388,#35389,#35390,#35391,
#35392,#35393,#35394,#35395,#35396,#35397,#35398),.UNSPECIFIED.,.F.,.F.,
(4,1,1,1,1,1,1,1,1,4),(34.5575191894886,35.0487646051486,36.0465927622169,
37.0444209192851,37.5433349978193,38.0422490763534,38.5411631548875,39.0400772334217,
40.0379053904899,40.8407044966681),.UNSPECIFIED.);
#4976=B_SPLINE_CURVE_WITH_KNOTS('',3,(#35403,#35404,#35405,#35406,#35407,
#35408,#35409,#35410,#35411,#35412,#35413,#35414),.UNSPECIFIED.,.F.,.F.,
(4,1,1,1,1,1,1,1,1,4),(28.2743338823088,28.3808315809043,29.3786597379725,
30.3764878950408,31.3743160521091,32.3721442091773,33.3699723662456,33.8688864447797,
34.3678005233138,34.5575191894884),.UNSPECIFIED.);
#4977=B_SPLINE_CURVE_WITH_KNOTS('',3,(#35415,#35416,#35417,#35418,#35419,
#35420,#35421,#35422,#35423,#35424,#35425,#35426),.UNSPECIFIED.,.F.,.F.,
(4,1,1,1,1,1,1,1,1,4),(28.274333882309,29.0617956627391,30.0596238198073,
30.5585378983415,31.0574519768756,31.5563660554097,32.0552801339438,33.0531082910121,
34.0509364480804,34.5575191894886),.UNSPECIFIED.);
#4978=B_SPLINE_CURVE_WITH_KNOTS('',3,(#35431,#35432,#35433,#35434,#35435,
#35436,#35437,#35438,#35439,#35440,#35441,#35442),.UNSPECIFIED.,.F.,.F.,
(4,1,1,1,1,1,1,1,1,4),(21.9911485751293,22.3938626384947,23.391690795563,
24.3895189526313,25.3873471096995,26.3851752667678,26.8840893453019,27.383003423836,
27.8819175023702,28.2743338823088),.UNSPECIFIED.);
#4979=B_SPLINE_CURVE_WITH_KNOTS('',3,(#35443,#35444,#35445,#35446,#35447,
#35448,#35449,#35450,#35451,#35452,#35453,#35454,#35455),.UNSPECIFIED.,
 .F.,.F.,(4,1,1,1,1,1,1,1,1,1,4),(21.9911485751294,22.0769985632613,23.0748267203295,
23.5737407988637,24.0726548773978,24.5715689559319,25.070483034466,26.0683111915343,
27.0661393486026,28.0639675056708,28.274333882309),.UNSPECIFIED.);
#4980=B_SPLINE_CURVE_WITH_KNOTS('',3,(#35460,#35461,#35462,#35463,#35464,
#35465,#35466,#35467,#35468,#35469,#35470,#35471,#35472,#35473,#35474,#35475,
#35476,#35477,#35478,#35479,#35480,#35481,#35482,#35483,#35484),
 .UNSPECIFIED.,.F.,.F.,(4,3,3,3,3,3,3,3,4),(15.7079632679497,16.5946426308105,
17.4813219936714,18.3680013565322,19.2546807193931,20.1413600822539,21.0280394451148,
21.9147188079757,21.9911485751293),.UNSPECIFIED.);
#4981=B_SPLINE_CURVE_WITH_KNOTS('',3,(#35485,#35486,#35487,#35488,#35489,
#35490,#35491,#35492,#35493,#35494,#35495,#35496),.UNSPECIFIED.,.F.,.F.,
(4,1,1,1,1,1,1,1,1,4),(15.7079632679498,16.0900296208517,16.5889436993859,
17.08785777792,17.5867718564541,18.0856859349882,19.0835140920565,20.0813422491248,
21.079170406193,21.9911485751294),.UNSPECIFIED.);
#4982=B_SPLINE_CURVE_WITH_KNOTS('',3,(#35507,#35508,#35509,#35510,#35511,
#35512,#35513,#35514,#35515,#35516,#35517,#35518,#35519,#35520,#35521,#35522,
#35523,#35524,#35525,#35526,#35527,#35528,#35529,#35530,#35531,#35532,#35533,
#35534,#35535,#35536,#35537,#35538,#35539,#35540,#35541,#35542,#35543,#35544,
#35545,#35546,#35547,#35548,#35549,#35550,#35551,#35552,#35553,#35554,#35555,
#35556,#35557,#35558,#35559,#35560,#35561,#35562,#35563,#35564,#35565,#35566,
#35567,#35568,#35569,#35570,#35571,#35572,#35573,#35574,#35575,#35576,#35577,
#35578,#35579,#35580,#35581,#35582,#35583,#35584,#35585,#35586,#35587,#35588,
#35589,#35590,#35591,#35592,#35593,#35594,#35595,#35596,#35597,#35598,#35599,
#35600,#35601,#35602,#35603,#35604,#35605,#35606,#35607,#35608,#35609,#35610,
#35611,#35612,#35613,#35614,#35615,#35616,#35617,#35618,#35619,#35620,#35621),
 .UNSPECIFIED.,.F.,.F.,(4,3,3,3,3,3,3,3,3,3,3,3,3,3,3,3,3,3,3,3,3,3,3,3,
3,3,3,3,3,3,3,3,3,3,3,3,3,3,4),(-1.3692760959275,-1.32188407678287,-1.27030325921837,
-1.23707822338629,-1.21785653354885,-1.20762469097439,-1.20007327221632,
-1.14735554371125,-1.09412617639606,-1.04931457447893,-1.04159068760046,
-1.03430007797452,-1.0045029725618,-0.950888266579126,-0.89680471903519,
-0.84212054701269,-0.801107417995814,-0.789867050271914,-0.783408395715883,
-0.728461154792874,-0.678068030945187,-0.623694406368148,-0.568930241759064,
-0.540708132249945,-0.532050528924746,-0.526074465104164,-0.470965504745358,
-0.415386731915167,-0.359836412129592,-0.343153365686116,-0.300259194975351,
-0.281492995289392,-0.271248085886408,-0.263224158006185,-0.207778571458046,
-0.151390901540102,-0.0948961475607414,-0.0389343418850663,0.),
 .UNSPECIFIED.);
#4983=B_SPLINE_CURVE_WITH_KNOTS('',3,(#35626,#35627,#35628,#35629,#35630,
#35631,#35632,#35633,#35634,#35635,#35636,#35637,#35638,#35639,#35640,#35641,
#35642,#35643,#35644,#35645,#35646,#35647,#35648,#35649,#35650,#35651,#35652,
#35653,#35654,#35655,#35656,#35657,#35658,#35659,#35660,#35661,#35662,#35663,
#35664,#35665,#35666,#35667,#35668,#35669,#35670,#35671,#35672,#35673,#35674,
#35675,#35676,#35677,#35678,#35679,#35680,#35681,#35682,#35683,#35684,#35685,
#35686,#35687,#35688,#35689,#35690,#35691,#35692,#35693,#35694,#35695,#35696,
#35697,#35698,#35699,#35700,#35701,#35702,#35703,#35704,#35705,#35706,#35707,
#35708,#35709,#35710,#35711,#35712,#35713,#35714,#35715,#35716,#35717,#35718,
#35719,#35720,#35721,#35722,#35723,#35724,#35725,#35726,#35727,#35728,#35729,
#35730,#35731,#35732,#35733,#35734,#35735,#35736,#35737,#35738,#35739,#35740),
 .UNSPECIFIED.,.F.,.F.,(4,3,3,3,3,3,3,3,3,3,3,3,3,3,3,3,3,3,3,3,3,3,3,3,
3,3,3,3,3,3,3,3,3,3,3,3,3,3,4),(-1.36616069392048,-1.3137619280474,-1.25760160850714,
-1.22204589932935,-1.20367987885411,-1.19122237291581,-1.18211951562472,
-1.12620867774649,-1.07028337971536,-1.02171965740005,-1.01246054855555,
-1.00560804218958,-0.973155935084748,-0.917891839945078,-0.862525668265144,
-0.806980972162821,-0.765322450086079,-0.751609718974351,-0.744373329264913,
-0.690070032077305,-0.640346883855853,-0.585898585520381,-0.531637706409828,
-0.504668943522143,-0.497129766489843,-0.490727294658046,-0.437156215864939,
-0.383621580535774,-0.330780907748743,-0.315887603308346,-0.276401652894803,
-0.259126549588878,-0.248755897899905,-0.240651076682722,-0.188174524652693,
-0.135375645330914,-0.0828505825103873,-0.0312642022900974,0.),
 .UNSPECIFIED.);
#4984=B_SPLINE_CURVE_WITH_KNOTS('',3,(#37793,#37794,#37795,#37796,#37797,
#37798,#37799,#37800,#37801,#37802,#37803,#37804,#37805,#37806,#37807,#37808,
#37809,#37810,#37811),.UNSPECIFIED.,.F.,.F.,(4,3,3,3,3,3,4),(387.881378170394,
388.155153099552,388.654067178086,389.152981256621,390.150809413689,391.148637570757,
392.070763168006),.UNSPECIFIED.);
#4985=B_SPLINE_CURVE_WITH_KNOTS('',3,(#37813,#37814,#37815,#37816,#37817,
#37818,#37819,#37820,#37821,#37822,#37823,#37824,#37825,#37826,#37827,#37828,
#37829,#37830,#37831,#37832,#37833,#37834,#37835,#37836,#37837,#37838,#37839,
#37840,#37841,#37842,#37843,#37844,#37845,#37846,#37847,#37848,#37849,#37850,
#37851,#37852,#37853,#37854,#37855,#37856,#37857,#37858,#37859,#37860,#37861,
#37862,#37863,#37864,#37865,#37866,#37867,#37868,#37869,#37870,#37871,#37872,
#37873,#37874,#37875,#37876,#37877,#37878,#37879,#37880,#37881,#37882,#37883,
#37884,#37885,#37886,#37887,#37888,#37889,#37890,#37891,#37892,#37893,#37894,
#37895,#37896,#37897,#37898,#37899,#37900,#37901,#37902,#37903,#37904,#37905,
#37906,#37907,#37908,#37909,#37910,#37911,#37912,#37913,#37914,#37915,#37916,
#37917,#37918,#37919,#37920,#37921,#37922,#37923,#37924,#37925,#37926,#37927),
 .UNSPECIFIED.,.F.,.F.,(4,3,3,3,3,3,3,3,3,3,3,3,3,3,3,3,3,3,3,3,3,3,3,3,
3,3,3,3,3,3,3,3,3,3,3,3,3,3,4),(-1.36927609592744,-1.32188407678276,-1.27030325921983,
-1.23707822338756,-1.21785653354656,-1.20762469155833,-1.20007327197696,
-1.14735554346642,-1.09412617616831,-1.04931457436499,-1.04159068704494,
-1.03430007789804,-1.00450297256166,-0.950888266553232,-0.896804719012292,
-0.84212054699549,-0.801107417982889,-0.789867050267934,-0.783408395762924,
-0.728461154848662,-0.678068030945084,-0.623694406361887,-0.56893024176975,
-0.540708132259289,-0.532050527890794,-0.526074465591946,-0.47096550523936,
-0.415386732454638,-0.359836412657358,-0.34315336568606,-0.300259194975303,
-0.281492995289346,-0.271248085891861,-0.263224157987078,-0.207778571445273,
-0.151390901525645,-0.0948961475312077,-0.0389343418600114,0.),
 .UNSPECIFIED.);
#4986=B_SPLINE_CURVE_WITH_KNOTS('',3,(#37928,#37929,#37930,#37931,#37932,
#37933),.UNSPECIFIED.,.F.,.F.,(4,1,1,4),(13.172247709466,14.0943733067152,
15.0922014637835,15.7079632679498),.UNSPECIFIED.);
#4987=B_SPLINE_CURVE_WITH_KNOTS('',3,(#37936,#37937,#37938,#37939,#37940,
#37941,#37942,#37943,#37944,#37945,#37946,#37947,#37948,#37949,#37950,#37951,
#37952,#37953,#37954,#37955,#37956,#37957,#37958,#37959,#37960,#37961,#37962,
#37963,#37964,#37965,#37966,#37967,#37968,#37969,#37970,#37971,#37972,#37973,
#37974,#37975,#37976,#37977,#37978,#37979,#37980,#37981,#37982,#37983,#37984,
#37985,#37986,#37987,#37988,#37989,#37990,#37991,#37992,#37993,#37994,#37995,
#37996,#37997,#37998,#37999,#38000,#38001,#38002,#38003,#38004,#38005,#38006,
#38007,#38008,#38009,#38010,#38011,#38012,#38013,#38014,#38015,#38016,#38017,
#38018,#38019,#38020,#38021,#38022,#38023,#38024,#38025,#38026,#38027,#38028,
#38029,#38030,#38031,#38032,#38033,#38034,#38035,#38036,#38037,#38038,#38039,
#38040,#38041,#38042,#38043,#38044,#38045,#38046,#38047,#38048,#38049,#38050),
 .UNSPECIFIED.,.F.,.F.,(4,3,3,3,3,3,3,3,3,3,3,3,3,3,3,3,3,3,3,3,3,3,3,3,
3,3,3,3,3,3,3,3,3,3,3,3,3,3,4),(-1.36616069392051,-1.31376192804741,-1.25760160853096,
-1.2220458993502,-1.20367987891242,-1.19122237324406,-1.1821195135026,-1.12620867561135,
-1.07028337760104,-1.02171965634293,-1.01246054749485,-1.00560804142907,
-0.973155935084823,-0.917891839934146,-0.862525668228774,-0.806980972135536,
-0.765322450065607,-0.75160971907717,-0.74437332928858,-0.690070032095365,
-0.64034688385582,-0.585898585517151,-0.531637706406087,-0.504668943518871,
-0.497129767239748,-0.490727295531997,-0.437156216738527,-0.383621581401278,
-0.330780908606657,-0.315887603308359,-0.276401652894814,-0.259126549588888,
-0.248755897909084,-0.240651077132608,-0.188174525113787,-0.135375645789863,
-0.0828505829447398,-0.0312642027293569,0.),.UNSPECIFIED.);
#4988=B_SPLINE_CURVE_WITH_KNOTS('',3,(#38053,#38054,#38055,#38056,#38057,
#38058),.UNSPECIFIED.,.F.,.F.,(4,1,1,4),(14.4112373819487,14.9101514604828,
15.4090655390169,15.7079632679497),.UNSPECIFIED.);
#4989=B_SPLINE_CURVE_WITH_KNOTS('',3,(#40111,#40112,#40113,#40114,#40115,
#40116,#40117,#40118,#40119,#40120,#40121,#40122,#40123,#40124,#40125,#40126,
#40127,#40128,#40129),.UNSPECIFIED.,.F.,.F.,(4,3,3,3,3,3,4),(-394.142122041962,
-393.643207963428,-393.144293884893,-392.645379806359,-392.146465727825,
-391.148637570757,-390.854214931135),.UNSPECIFIED.);
#4990=B_SPLINE_CURVE_WITH_KNOTS('',3,(#40132,#40133,#40134,#40135,#40136,
#40137,#40138,#40139,#40140,#40141,#40142,#40143,#40144,#40145,#40146,#40147,
#40148,#40149,#40150,#40151,#40152,#40153,#40154,#40155,#40156,#40157,#40158,
#40159,#40160,#40161,#40162,#40163,#40164,#40165,#40166,#40167,#40168,#40169,
#40170,#40171,#40172,#40173,#40174,#40175,#40176,#40177,#40178,#40179,#40180,
#40181,#40182,#40183,#40184,#40185,#40186,#40187,#40188,#40189,#40190,#40191,
#40192,#40193,#40194,#40195,#40196,#40197,#40198,#40199,#40200,#40201,#40202,
#40203,#40204,#40205,#40206,#40207,#40208,#40209,#40210,#40211,#40212,#40213,
#40214,#40215,#40216,#40217,#40218,#40219,#40220,#40221,#40222,#40223,#40224,
#40225,#40226,#40227,#40228,#40229,#40230,#40231,#40232,#40233,#40234,#40235,
#40236,#40237,#40238,#40239,#40240,#40241,#40242,#40243),.UNSPECIFIED.,
 .F.,.F.,(4,3,3,3,3,3,3,3,3,3,3,3,3,3,3,3,3,3,3,3,3,3,3,3,3,3,3,3,3,3,3,
3,3,3,3,3,3,4),(-1.36927609592741,-1.31976302467547,-1.2674742744568,-1.23439849328534,
-1.21163835138631,-1.20085128479468,-1.14769397227967,-1.09436197408657,
-1.04861499958584,-1.04164621982373,-1.03428540169754,-1.00286802508512,
-0.949812476279694,-0.896070170266004,-0.841289386086885,-0.800203797952546,
-0.788785995023541,-0.782022675529197,-0.727256626595045,-0.67694703354953,
-0.622431301271701,-0.567625470663003,-0.539494668235961,-0.53224730158684,
-0.526366577252169,-0.471123972311258,-0.415492601545496,-0.359953143368869,
-0.342579051246667,-0.299756669840834,-0.281021877975781,-0.270604933475851,
-0.263553420126647,-0.20815816146705,-0.151770314335523,-0.0952750360977028,
-0.03935989507387,0.),.UNSPECIFIED.);
#4991=B_SPLINE_CURVE_WITH_KNOTS('',3,(#40248,#40249,#40250,#40251,#40252,
#40253,#40254,#40255,#40256,#40257,#40258,#40259,#40260,#40261,#40262,#40263,
#40264,#40265,#40266,#40267,#40268,#40269,#40270,#40271,#40272,#40273,#40274,
#40275,#40276,#40277,#40278,#40279,#40280,#40281,#40282,#40283,#40284,#40285,
#40286,#40287,#40288,#40289,#40290,#40291,#40292,#40293,#40294,#40295,#40296,
#40297,#40298,#40299,#40300,#40301,#40302,#40303,#40304,#40305,#40306,#40307,
#40308,#40309,#40310,#40311,#40312,#40313,#40314,#40315,#40316,#40317,#40318,
#40319,#40320,#40321,#40322,#40323,#40324,#40325,#40326,#40327,#40328,#40329,
#40330,#40331,#40332,#40333,#40334,#40335,#40336,#40337,#40338,#40339,#40340,
#40341,#40342,#40343,#40344,#40345,#40346,#40347,#40348,#40349,#40350,#40351,
#40352,#40353,#40354,#40355,#40356,#40357,#40358,#40359,#40360,#40361,#40362),
 .UNSPECIFIED.,.F.,.F.,(4,3,3,3,3,3,3,3,3,3,3,3,3,3,3,3,3,3,3,3,3,3,3,3,
3,3,3,3,3,3,3,3,3,3,3,3,3,3,4),(-1.36616069392046,-1.31142638897199,-1.25498626984362,
-1.21954375073289,-1.19734069803303,-1.18767642039703,-1.17959396109305,
-1.12369342935424,-1.06807187425649,-1.01975899560714,-1.01204767220352,
-1.00441384808788,-0.97144611695779,-0.91645908715266,-0.861167890840583,
-0.805684136616207,-0.764071320947925,-0.752912961187079,-0.746308512839135,
-0.691965003401675,-0.63923287394308,-0.584768581393643,-0.530513315239903,
-0.503617313135893,-0.496026441221278,-0.48914350076485,-0.435553954734991,
-0.382024894959837,-0.329152210381291,-0.315345298407825,-0.275927136106847,
-0.258681690100169,-0.24846788515743,-0.240610235241747,-0.188114192777283,
-0.135324807824555,-0.0828541010340507,-0.0314047502190577,0.),
 .UNSPECIFIED.);
#4992=B_SPLINE_CURVE_WITH_KNOTS('',3,(#41199,#41200,#41201,#41202,#41203,
#41204,#41205,#41206,#41207,#41208,#41209,#41210,#41211,#41212,#41213,#41214,
#41215,#41216,#41217,#41218,#41219,#41220,#41221,#41222,#41223,#41224,#41225,
#41226,#41227,#41228,#41229,#41230,#41231,#41232,#41233,#41234,#41235),
 .UNSPECIFIED.,.F.,.F.,(4,3,3,3,3,3,3,3,3,3,3,3,4),(95.0849428558252,95.1312807944966,
95.6293503274521,96.1274198604076,96.6254893933631,97.1235589263185,97.621628459274,
98.1196979922295,98.617767525185,99.1158370581404,99.6139065910959,100.111976124051,
100.530964914873),.UNSPECIFIED.);
#4993=B_SPLINE_CURVE_WITH_KNOTS('',3,(#41237,#41238,#41239,#41240,#41241,
#41242,#41243,#41244,#41245,#41246,#41247,#41248,#41249,#41250,#41251,#41252,
#41253,#41254,#41255,#41256,#41257,#41258,#41259,#41260,#41261,#41262,#41263,
#41264,#41265,#41266,#41267,#41268,#41269,#41270,#41271,#41272,#41273,#41274,
#41275,#41276,#41277,#41278,#41279,#41280,#41281,#41282,#41283,#41284,#41285,
#41286,#41287,#41288,#41289,#41290,#41291,#41292,#41293,#41294,#41295,#41296,
#41297,#41298,#41299,#41300,#41301,#41302,#41303,#41304,#41305,#41306,#41307,
#41308,#41309,#41310,#41311,#41312,#41313,#41314,#41315,#41316,#41317,#41318,
#41319,#41320,#41321,#41322,#41323,#41324,#41325,#41326,#41327,#41328,#41329,
#41330,#41331,#41332,#41333,#41334,#41335,#41336,#41337,#41338,#41339,#41340,
#41341,#41342,#41343,#41344,#41345,#41346,#41347,#41348),.UNSPECIFIED.,
 .F.,.F.,(4,3,3,3,3,3,3,3,3,3,3,3,3,3,3,3,3,3,3,3,3,3,3,3,3,3,3,3,3,3,3,
3,3,3,3,3,3,4),(-1.3692760959275,-1.31976302467557,-1.26747427578708,-1.23439849444934,
-1.21163835086635,-1.20085128503299,-1.14769397303989,-1.09436197457134,
-1.04861499982825,-1.04164622051909,-1.03428540176251,-1.00286802508516,
-0.949812474675958,-0.896070168269673,-0.841289384589646,-0.800203796829625,
-0.788785992753292,-0.782022674895381,-0.727256625791858,-0.676947033549563,
-0.622431298515392,-0.567625467803214,-0.539494665733644,-0.532247290384895,
-0.526366563048055,-0.471123955098454,-0.415492583526853,-0.359953130535847,
-0.342579051246657,-0.299756669840825,-0.281021877975773,-0.270604933188539,
-0.263553420220014,-0.208158173018763,-0.151770330552895,-0.0952750507295094,
-0.0393598974769998,0.),.UNSPECIFIED.);
#4994=B_SPLINE_CURVE_WITH_KNOTS('',3,(#41349,#41350,#41351,#41352,#41353,
#41354,#41355,#41356,#41357,#41358,#41359,#41360,#41361,#41362),
 .UNSPECIFIED.,.F.,.F.,(4,1,1,1,1,1,1,1,1,1,1,4),(10.6589735865933,11.0779623774152,
11.5760319103707,12.0741014433262,12.5721709762817,13.0702405092372,13.5683100421926,
14.0663795751481,14.5644491081036,15.0625186410591,15.5605881740146,15.7079632679489),
 .UNSPECIFIED.);
#4995=B_SPLINE_CURVE_WITH_KNOTS('',3,(#41365,#41366,#41367,#41368,#41369,
#41370,#41371,#41372,#41373,#41374,#41375,#41376,#41377,#41378,#41379,#41380,
#41381,#41382,#41383,#41384,#41385,#41386,#41387,#41388,#41389,#41390,#41391,
#41392,#41393,#41394,#41395,#41396,#41397,#41398,#41399,#41400,#41401,#41402,
#41403,#41404,#41405,#41406,#41407,#41408,#41409,#41410,#41411,#41412,#41413,
#41414,#41415,#41416,#41417,#41418,#41419,#41420,#41421,#41422,#41423,#41424,
#41425,#41426,#41427,#41428,#41429,#41430,#41431,#41432,#41433,#41434,#41435,
#41436,#41437,#41438,#41439,#41440,#41441,#41442,#41443,#41444,#41445,#41446,
#41447,#41448,#41449,#41450,#41451,#41452,#41453,#41454,#41455,#41456,#41457,
#41458,#41459,#41460,#41461,#41462,#41463,#41464,#41465,#41466,#41467,#41468,
#41469,#41470,#41471,#41472,#41473,#41474,#41475,#41476,#41477,#41478,#41479),
 .UNSPECIFIED.,.F.,.F.,(4,3,3,3,3,3,3,3,3,3,3,3,3,3,3,3,3,3,3,3,3,3,3,3,
3,3,3,3,3,3,3,3,3,3,3,3,3,3,4),(-1.36616069392038,-1.31142638897197,-1.25498626979377,
-1.21954375068927,-1.19734069753713,-1.18767641877559,-1.17959396063584,
-1.12369342906595,-1.06807187393295,-1.01975899544537,-1.01204767193382,
-1.00441384808241,-0.971446116957786,-0.916459086968053,-0.861167891330158,
-0.805684136983392,-0.764071321223317,-0.752912961782954,-0.746308513132906,
-0.691965005739893,-0.639232873943093,-0.584768580907417,-0.53051330855053,
-0.50361730728269,-0.496026418883006,-0.489143497419182,-0.435553950836429,
-0.382024885820224,-0.329152189052059,-0.315345298407804,-0.275927136106829,
-0.258681690100152,-0.248467885303507,-0.240610235431388,-0.188114185716531,
-0.135324804513882,-0.082854107800741,-0.0314047741919013,0.),
 .UNSPECIFIED.);
#4996=B_SPLINE_CURVE_WITH_KNOTS('',3,(#41482,#41483,#41484,#41485,#41486,
#41487,#41488,#41489,#41490,#41491,#41492),.UNSPECIFIED.,.F.,.F.,(4,1,1,
1,1,1,1,1,4),(11.897963259076,12.3960327920314,12.8941023249869,13.3921718579424,
13.8902413908979,14.3883109238534,14.8863804568088,15.3844499897643,15.7079632679489),
 .UNSPECIFIED.);
#4997=B_SPLINE_CURVE_WITH_KNOTS('',3,(#42329,#42330,#42331,#42332,#42333,
#42334,#42335,#42336,#42337,#42338,#42339,#42340,#42341,#42342,#42343,#42344,
#42345,#42346,#42347,#42348,#42349,#42350,#42351,#42352,#42353,#42354,#42355,
#42356,#42357,#42358,#42359),.UNSPECIFIED.,.F.,.F.,(4,3,3,3,3,3,3,3,3,3,
4),(-102.602323788829,-102.104254255873,-101.606184722918,-101.108115189962,
-100.610045657007,-100.111976124051,-99.6139065910959,-99.1158370581404,
-98.6177675251849,-98.1196979922295,-98.0577796165668),.UNSPECIFIED.);
#4998=B_SPLINE_CURVE_WITH_KNOTS('',3,(#42504,#42505,#42506,#42507),
 .UNSPECIFIED.,.F.,.F.,(4,4),(0.,0.0936682560791196),.UNSPECIFIED.);
#4999=B_SPLINE_CURVE_WITH_KNOTS('',3,(#42537,#42538,#42539,#42540,#42541,
#42542),.UNSPECIFIED.,.F.,.F.,(4,2,4),(0.664134112378609,0.666288650481674,
0.834782922241236),.UNSPECIFIED.);
#5000=B_SPLINE_CURVE_WITH_KNOTS('',3,(#42543,#42544,#42545,#42546),
 .UNSPECIFIED.,.F.,.F.,(4,4),(0.,1.5),.UNSPECIFIED.);
#5001=B_SPLINE_CURVE_WITH_KNOTS('',3,(#42632,#42633,#42634,#42635,#42636,
#42637,#42638),.UNSPECIFIED.,.F.,.F.,(4,3,4),(0.00777826218664459,0.048552619044639,
0.0850249535915979),.UNSPECIFIED.);
#5002=B_SPLINE_CURVE_WITH_KNOTS('',3,(#42640,#42641,#42642,#42643),
 .UNSPECIFIED.,.F.,.F.,(4,4),(0.,1.5),.UNSPECIFIED.);
#5003=B_SPLINE_CURVE_WITH_KNOTS('',3,(#42645,#42646,#42647,#42648,#42649,
#42650,#42651),.UNSPECIFIED.,.F.,.F.,(4,3,4),(0.,0.0468232933785311,0.0773537975132304),
 .UNSPECIFIED.);
#5004=B_SPLINE_CURVE_WITH_KNOTS('',3,(#42687,#42688,#42689,#42690),
 .UNSPECIFIED.,.F.,.F.,(4,4),(0.0949433903987894,0.171326334486879),
 .UNSPECIFIED.);
#5005=B_SPLINE_CURVE_WITH_KNOTS('',3,(#42696,#42697,#42698,#42699),
 .UNSPECIFIED.,.F.,.F.,(4,4),(0.,0.0936682560793217),.UNSPECIFIED.);
#5006=B_SPLINE_CURVE_WITH_KNOTS('',3,(#42704,#42705,#42706,#42707),
 .UNSPECIFIED.,.F.,.F.,(4,4),(0.,1.5),.UNSPECIFIED.);
#5007=B_SPLINE_CURVE_WITH_KNOTS('',3,(#42711,#42712,#42713,#42714),
 .UNSPECIFIED.,.F.,.F.,(4,4),(0.,0.0771717558746826),.UNSPECIFIED.);
#5008=B_SPLINE_CURVE_WITH_KNOTS('',3,(#42856,#42857,#42858,#42859),
 .UNSPECIFIED.,.F.,.F.,(4,4),(0.,0.0936682560792406),.UNSPECIFIED.);
#5009=B_SPLINE_CURVE_WITH_KNOTS('',3,(#42889,#42890,#42891,#42892,#42893,
#42894),.UNSPECIFIED.,.F.,.F.,(4,2,4),(0.66413411238557,0.666288650489319,
0.834782922257957),.UNSPECIFIED.);
#5010=B_SPLINE_CURVE_WITH_KNOTS('',3,(#42895,#42896,#42897,#42898),
 .UNSPECIFIED.,.F.,.F.,(4,4),(0.,1.5),.UNSPECIFIED.);
#5011=B_SPLINE_CURVE_WITH_KNOTS('',3,(#43018,#43019,#43020,#43021),
 .UNSPECIFIED.,.F.,.F.,(4,4),(0.0949433903987529,0.171326334486776),
 .UNSPECIFIED.);
#5012=B_SPLINE_CURVE_WITH_KNOTS('',3,(#43026,#43027,#43028,#43029),
 .UNSPECIFIED.,.F.,.F.,(4,4),(0.,1.5),.UNSPECIFIED.);
#5013=B_SPLINE_CURVE_WITH_KNOTS('',3,(#43033,#43034,#43035,#43036),
 .UNSPECIFIED.,.F.,.F.,(4,4),(0.,0.0771717558741193),.UNSPECIFIED.);
#5014=B_SPLINE_CURVE_WITH_KNOTS('',3,(#43178,#43179,#43180,#43181),
 .UNSPECIFIED.,.F.,.F.,(4,4),(0.,0.0936682560792162),.UNSPECIFIED.);
#5015=B_SPLINE_CURVE_WITH_KNOTS('',3,(#43211,#43212,#43213,#43214,#43215,
#43216),.UNSPECIFIED.,.F.,.F.,(4,2,4),(0.664134112375963,0.666288650477681,
0.834782922235844),.UNSPECIFIED.);
#5016=B_SPLINE_CURVE_WITH_KNOTS('',3,(#43217,#43218,#43219,#43220),
 .UNSPECIFIED.,.F.,.F.,(4,4),(0.,1.5),.UNSPECIFIED.);
#5017=B_SPLINE_CURVE_WITH_KNOTS('',3,(#43340,#43341,#43342,#43343),
 .UNSPECIFIED.,.F.,.F.,(4,4),(0.0895792937411446,0.166038797206149),
 .UNSPECIFIED.);
#5018=B_SPLINE_CURVE_WITH_KNOTS('',3,(#43348,#43349,#43350,#43351),
 .UNSPECIFIED.,.F.,.F.,(4,4),(0.,1.5),.UNSPECIFIED.);
#5019=B_SPLINE_CURVE_WITH_KNOTS('',3,(#43355,#43356,#43357,#43358),
 .UNSPECIFIED.,.F.,.F.,(4,4),(0.,0.0771946366775442),.UNSPECIFIED.);
#5020=B_SPLINE_CURVE_WITH_KNOTS('',3,(#43500,#43501,#43502,#43503),
 .UNSPECIFIED.,.F.,.F.,(4,4),(0.,0.0936682560793148),.UNSPECIFIED.);
#5021=B_SPLINE_CURVE_WITH_KNOTS('',3,(#43533,#43534,#43535,#43536,#43537,
#43538),.UNSPECIFIED.,.F.,.F.,(4,2,4),(0.646941188901376,0.687030553871696,
0.838090507429105),.UNSPECIFIED.);
#5022=B_SPLINE_CURVE_WITH_KNOTS('',3,(#43539,#43540,#43541,#43542),
 .UNSPECIFIED.,.F.,.F.,(4,4),(0.,1.5),.UNSPECIFIED.);
#5023=B_SPLINE_CURVE_WITH_KNOTS('',3,(#43662,#43663,#43664,#43665),
 .UNSPECIFIED.,.F.,.F.,(4,4),(0.027979075972516,0.105105315913476),
 .UNSPECIFIED.);
#5024=B_SPLINE_CURVE_WITH_KNOTS('',3,(#43670,#43671,#43672,#43673),
 .UNSPECIFIED.,.F.,.F.,(4,4),(0.,1.5),.UNSPECIFIED.);
#5025=B_SPLINE_CURVE_WITH_KNOTS('',3,(#43677,#43678,#43679,#43680),
 .UNSPECIFIED.,.F.,.F.,(4,4),(0.,0.0773597620762172),.UNSPECIFIED.);
#5026=B_SPLINE_CURVE_WITH_KNOTS('',3,(#43822,#43823,#43824,#43825),
 .UNSPECIFIED.,.F.,.F.,(4,4),(0.,0.093668256079297),.UNSPECIFIED.);
#5027=B_SPLINE_CURVE_WITH_KNOTS('',3,(#43855,#43856,#43857,#43858,#43859,
#43860,#43861,#43862,#43863,#43864,#43865,#43866,#43867,#43868,#43869,#43870,
#43871,#43872,#43873),.UNSPECIFIED.,.F.,.F.,(4,3,3,3,3,3,4),(0.648956304782129,
0.690807645944959,0.735062548516529,0.758873076278325,0.788602851685956,
0.813152022949223,0.816613420545173),.UNSPECIFIED.);
#5028=B_SPLINE_CURVE_WITH_KNOTS('',3,(#43874,#43875,#43876,#43877),
 .UNSPECIFIED.,.F.,.F.,(4,4),(0.,1.5),.UNSPECIFIED.);
#5029=B_SPLINE_CURVE_WITH_KNOTS('',3,(#43997,#43998,#43999,#44000),
 .UNSPECIFIED.,.F.,.F.,(4,4),(0.0949433903987678,0.171326334486587),
 .UNSPECIFIED.);
#5030=B_SPLINE_CURVE_WITH_KNOTS('',3,(#44005,#44006,#44007,#44008),
 .UNSPECIFIED.,.F.,.F.,(4,4),(0.,1.5),.UNSPECIFIED.);
#5031=B_SPLINE_CURVE_WITH_KNOTS('',3,(#44012,#44013,#44014,#44015),
 .UNSPECIFIED.,.F.,.F.,(4,4),(0.,0.0771717558746195),.UNSPECIFIED.);
#5032=B_SPLINE_CURVE_WITH_KNOTS('',3,(#44157,#44158,#44159,#44160),
 .UNSPECIFIED.,.F.,.F.,(4,4),(0.,0.0936682560791507),.UNSPECIFIED.);
#5033=B_SPLINE_CURVE_WITH_KNOTS('',3,(#44190,#44191,#44192,#44193,#44194,
#44195),.UNSPECIFIED.,.F.,.F.,(4,2,4),(0.664134112375084,0.66628865047855,
0.834782922233775),.UNSPECIFIED.);
#5034=B_SPLINE_CURVE_WITH_KNOTS('',3,(#44196,#44197,#44198,#44199),
 .UNSPECIFIED.,.F.,.F.,(4,4),(0.,1.5),.UNSPECIFIED.);
#5035=B_SPLINE_CURVE_WITH_KNOTS('',3,(#44319,#44320,#44321,#44322),
 .UNSPECIFIED.,.F.,.F.,(4,4),(0.0949433904009592,0.171326334491679),
 .UNSPECIFIED.);
#5036=B_SPLINE_CURVE_WITH_KNOTS('',3,(#44327,#44328,#44329,#44330),
 .UNSPECIFIED.,.F.,.F.,(4,4),(0.,1.5),.UNSPECIFIED.);
#5037=B_SPLINE_CURVE_WITH_KNOTS('',3,(#44334,#44335,#44336,#44337),
 .UNSPECIFIED.,.F.,.F.,(4,4),(0.,0.0771717558747488),.UNSPECIFIED.);
#5038=B_SPLINE_CURVE_WITH_KNOTS('',3,(#44479,#44480,#44481,#44482),
 .UNSPECIFIED.,.F.,.F.,(4,4),(0.,0.0936682560792248),.UNSPECIFIED.);
#5039=B_SPLINE_CURVE_WITH_KNOTS('',3,(#44512,#44513,#44514,#44515,#44516,
#44517),.UNSPECIFIED.,.F.,.F.,(4,2,4),(0.664134112390545,0.666288650493472,
0.834782922267389),.UNSPECIFIED.);
#5040=B_SPLINE_CURVE_WITH_KNOTS('',3,(#44518,#44519,#44520,#44521),
 .UNSPECIFIED.,.F.,.F.,(4,4),(0.,1.5),.UNSPECIFIED.);
#5041=B_SPLINE_CURVE_WITH_KNOTS('',3,(#44641,#44642,#44643,#44644),
 .UNSPECIFIED.,.F.,.F.,(4,4),(0.0415520628988323,0.118563606137955),
 .UNSPECIFIED.);
#5042=B_SPLINE_CURVE_WITH_KNOTS('',3,(#44649,#44650,#44651,#44652),
 .UNSPECIFIED.,.F.,.F.,(4,4),(0.,1.5),.UNSPECIFIED.);
#5043=B_SPLINE_CURVE_WITH_KNOTS('',3,(#44656,#44657,#44658,#44659),
 .UNSPECIFIED.,.F.,.F.,(4,4),(0.,0.0773423902580483),.UNSPECIFIED.);
#5044=B_SPLINE_CURVE_WITH_KNOTS('',3,(#44803,#44804,#44805,#44806,#44807,
#44808),.UNSPECIFIED.,.F.,.F.,(4,2,4),(0.,0.0823790100552426,0.0949061944490219),
 .UNSPECIFIED.);
#5045=B_SPLINE_CURVE_WITH_KNOTS('',3,(#44838,#44839,#44840,#44841,#44842,
#44843),.UNSPECIFIED.,.F.,.F.,(4,2,4),(0.0444437679303765,0.055294838243425,
0.103828820469121),.UNSPECIFIED.);
#5046=B_SPLINE_CURVE_WITH_KNOTS('',3,(#44844,#44845,#44846,#44847),
 .UNSPECIFIED.,.F.,.F.,(4,4),(0.,1.5),.UNSPECIFIED.);
#5047=B_SPLINE_CURVE_WITH_KNOTS('',3,(#44969,#44970,#44971,#44972),
 .UNSPECIFIED.,.F.,.F.,(4,4),(0.060413669704354,0.137235209115667),
 .UNSPECIFIED.);
#5048=B_SPLINE_CURVE_WITH_KNOTS('',3,(#44977,#44978,#44979,#44980),
 .UNSPECIFIED.,.F.,.F.,(4,4),(0.,1.5),.UNSPECIFIED.);
#5049=B_SPLINE_CURVE_WITH_KNOTS('',3,(#44984,#44985,#44986,#44987),
 .UNSPECIFIED.,.F.,.F.,(4,4),(0.,0.0772979364659118),.UNSPECIFIED.);
#5050=B_SPLINE_CURVE_WITH_KNOTS('',3,(#45129,#45130,#45131,#45132),
 .UNSPECIFIED.,.F.,.F.,(4,4),(0.,0.0936682560792101),.UNSPECIFIED.);
#5051=B_SPLINE_CURVE_WITH_KNOTS('',3,(#45162,#45163,#45164,#45165,#45166,
#45167),.UNSPECIFIED.,.F.,.F.,(4,2,4),(0.640100729216595,0.692644753706222,
0.794134458427311),.UNSPECIFIED.);
#5052=B_SPLINE_CURVE_WITH_KNOTS('',3,(#45168,#45169,#45170,#45171),
 .UNSPECIFIED.,.F.,.F.,(4,4),(0.,1.5),.UNSPECIFIED.);
#5053=B_SPLINE_CURVE_WITH_KNOTS('',3,(#45291,#45292,#45293,#45294),
 .UNSPECIFIED.,.F.,.F.,(4,4),(0.0949433903984102,0.17132633448589),
 .UNSPECIFIED.);
#5054=B_SPLINE_CURVE_WITH_KNOTS('',3,(#45299,#45300,#45301,#45302),
 .UNSPECIFIED.,.F.,.F.,(4,4),(0.,1.5),.UNSPECIFIED.);
#5055=B_SPLINE_CURVE_WITH_KNOTS('',3,(#45306,#45307,#45308,#45309),
 .UNSPECIFIED.,.F.,.F.,(4,4),(0.,0.0771717558744038),.UNSPECIFIED.);
#5056=B_SPLINE_CURVE_WITH_KNOTS('',3,(#45451,#45452,#45453,#45454),
 .UNSPECIFIED.,.F.,.F.,(4,4),(0.,0.0936682560792258),.UNSPECIFIED.);
#5057=B_SPLINE_CURVE_WITH_KNOTS('',3,(#45484,#45485,#45486,#45487,#45488,
#45489),.UNSPECIFIED.,.F.,.F.,(4,2,4),(0.664134112379071,0.666288650482174,
0.834782922244795),.UNSPECIFIED.);
#5058=B_SPLINE_CURVE_WITH_KNOTS('',3,(#45490,#45491,#45492,#45493),
 .UNSPECIFIED.,.F.,.F.,(4,4),(0.,1.5),.UNSPECIFIED.);
#5059=B_SPLINE_CURVE_WITH_KNOTS('',3,(#45613,#45614,#45615,#45616),
 .UNSPECIFIED.,.F.,.F.,(4,4),(0.0949433903977092,0.171326334484129),
 .UNSPECIFIED.);
#5060=B_SPLINE_CURVE_WITH_KNOTS('',3,(#45621,#45622,#45623,#45624),
 .UNSPECIFIED.,.F.,.F.,(4,4),(0.,1.5),.UNSPECIFIED.);
#5061=B_SPLINE_CURVE_WITH_KNOTS('',3,(#45628,#45629,#45630,#45631),
 .UNSPECIFIED.,.F.,.F.,(4,4),(0.,0.0771717558746607),.UNSPECIFIED.);
#5062=B_SPLINE_CURVE_WITH_KNOTS('',3,(#45773,#45774,#45775,#45776),
 .UNSPECIFIED.,.F.,.F.,(4,4),(0.,0.093668256079299),.UNSPECIFIED.);
#5063=B_SPLINE_CURVE_WITH_KNOTS('',3,(#45806,#45807,#45808,#45809,#45810,
#45811),.UNSPECIFIED.,.F.,.F.,(4,2,4),(0.664134112381964,0.666288650485371,
0.834782922251792),.UNSPECIFIED.);
#5064=B_SPLINE_CURVE_WITH_KNOTS('',3,(#45812,#45813,#45814,#45815),
 .UNSPECIFIED.,.F.,.F.,(4,4),(0.,1.5),.UNSPECIFIED.);
#5065=B_SPLINE_CURVE_WITH_KNOTS('',3,(#45935,#45936,#45937,#45938,#45939,
#45940,#45941),.UNSPECIFIED.,.F.,.F.,(4,3,4),(0.010983168869138,0.0518472130937835,
0.0882158993716873),.UNSPECIFIED.);
#5066=B_SPLINE_CURVE_WITH_KNOTS('',3,(#45946,#45947,#45948,#45949),
 .UNSPECIFIED.,.F.,.F.,(4,4),(0.,1.5),.UNSPECIFIED.);
#5067=B_SPLINE_CURVE_WITH_KNOTS('',3,(#45953,#45954,#45955,#45956,#45957,
#45958,#45959),.UNSPECIFIED.,.F.,.F.,(4,3,4),(0.,0.0437124803990652,0.0773577392014732),
 .UNSPECIFIED.);
#5068=B_SPLINE_CURVE_WITH_KNOTS('',3,(#46101,#46102,#46103,#46104),
 .UNSPECIFIED.,.F.,.F.,(4,4),(0.,0.0936682560792125),.UNSPECIFIED.);
#5069=B_SPLINE_CURVE_WITH_KNOTS('',3,(#46134,#46135,#46136,#46137,#46138,
#46139),.UNSPECIFIED.,.F.,.F.,(4,2,4),(0.610800819740342,0.676516947854421,
0.787792634400649),.UNSPECIFIED.);
#5070=B_SPLINE_CURVE_WITH_KNOTS('',3,(#46140,#46141,#46142,#46143),
 .UNSPECIFIED.,.F.,.F.,(4,4),(0.,1.5),.UNSPECIFIED.);
#5071=B_SPLINE_CURVE_WITH_KNOTS('',3,(#46263,#46264,#46265,#46266),
 .UNSPECIFIED.,.F.,.F.,(4,4),(0.0949433903987918,0.171326334487022),
 .UNSPECIFIED.);
#5072=B_SPLINE_CURVE_WITH_KNOTS('',3,(#46271,#46272,#46273,#46274),
 .UNSPECIFIED.,.F.,.F.,(4,4),(0.,1.5),.UNSPECIFIED.);
#5073=B_SPLINE_CURVE_WITH_KNOTS('',3,(#46278,#46279,#46280,#46281),
 .UNSPECIFIED.,.F.,.F.,(4,4),(0.,0.0771717558745271),.UNSPECIFIED.);
#5074=B_SPLINE_CURVE_WITH_KNOTS('',3,(#46423,#46424,#46425,#46426),
 .UNSPECIFIED.,.F.,.F.,(4,4),(0.,0.0936682560791833),.UNSPECIFIED.);
#5075=B_SPLINE_CURVE_WITH_KNOTS('',3,(#46456,#46457,#46458,#46459,#46460,
#46461),.UNSPECIFIED.,.F.,.F.,(4,2,4),(0.666123023340529,0.674012769702091,
0.844667464106696),.UNSPECIFIED.);
#5076=B_SPLINE_CURVE_WITH_KNOTS('',3,(#46462,#46463,#46464,#46465),
 .UNSPECIFIED.,.F.,.F.,(4,4),(0.,1.5),.UNSPECIFIED.);
#5077=B_SPLINE_CURVE_WITH_KNOTS('',3,(#46585,#46586,#46587,#46588),
 .UNSPECIFIED.,.F.,.F.,(4,4),(0.0949433904001744,0.171326334490195),
 .UNSPECIFIED.);
#5078=B_SPLINE_CURVE_WITH_KNOTS('',3,(#46593,#46594,#46595,#46596),
 .UNSPECIFIED.,.F.,.F.,(4,4),(0.,1.5),.UNSPECIFIED.);
#5079=B_SPLINE_CURVE_WITH_KNOTS('',3,(#46600,#46601,#46602,#46603),
 .UNSPECIFIED.,.F.,.F.,(4,4),(0.,0.0771717558751156),.UNSPECIFIED.);
#5080=B_SPLINE_CURVE_WITH_KNOTS('',3,(#46745,#46746,#46747,#46748),
 .UNSPECIFIED.,.F.,.F.,(4,4),(0.,0.0936682560791758),.UNSPECIFIED.);
#5081=B_SPLINE_CURVE_WITH_KNOTS('',3,(#46778,#46779,#46780,#46781,#46782,
#46783),.UNSPECIFIED.,.F.,.F.,(4,2,4),(0.6641341123862,0.666288650490994,
0.83478292226001),.UNSPECIFIED.);
#5082=B_SPLINE_CURVE_WITH_KNOTS('',3,(#46784,#46785,#46786,#46787),
 .UNSPECIFIED.,.F.,.F.,(4,4),(0.,1.5),.UNSPECIFIED.);
#5083=B_SPLINE_CURVE_WITH_KNOTS('',3,(#46907,#46908,#46909,#46910),
 .UNSPECIFIED.,.F.,.F.,(4,4),(0.0949433903985646,0.171326334486267),
 .UNSPECIFIED.);
#5084=B_SPLINE_CURVE_WITH_KNOTS('',3,(#46915,#46916,#46917,#46918),
 .UNSPECIFIED.,.F.,.F.,(4,4),(0.,1.5),.UNSPECIFIED.);
#5085=B_SPLINE_CURVE_WITH_KNOTS('',3,(#46922,#46923,#46924,#46925),
 .UNSPECIFIED.,.F.,.F.,(4,4),(0.,0.0771717558742884),.UNSPECIFIED.);
#5086=B_SPLINE_CURVE_WITH_KNOTS('',3,(#47182,#47183,#47184,#47185,#47186,
#47187),.UNSPECIFIED.,.F.,.F.,(4,2,4),(0.6641341123769,0.666288650478339,
0.834782922237864),.UNSPECIFIED.);
#5087=B_SPLINE_CURVE_WITH_KNOTS('',3,(#47188,#47189,#47190,#47191),
 .UNSPECIFIED.,.F.,.F.,(4,4),(0.,1.5),.UNSPECIFIED.);
#5442=LINE('',#27824,#6334);
#5443=LINE('',#27854,#6335);
#5444=LINE('',#27858,#6336);
#5445=LINE('',#27862,#6337);
#5446=LINE('',#27867,#6338);
#5447=LINE('',#27895,#6339);
#5448=LINE('',#27899,#6340);
#5449=LINE('',#27904,#6341);
#5450=LINE('',#27964,#6342);
#5451=LINE('',#28024,#6343);
#5452=LINE('',#28081,#6344);
#5453=LINE('',#28141,#6345);
#5454=LINE('',#28201,#6346);
#5455=LINE('',#28261,#6347);
#5456=LINE('',#28318,#6348);
#5457=LINE('',#28375,#6349);
#5458=LINE('',#28438,#6350);
#5459=LINE('',#28492,#6351);
#5460=LINE('',#28552,#6352);
#5461=LINE('',#28612,#6353);
#5462=LINE('',#28669,#6354);
#5463=LINE('',#28726,#6355);
#5464=LINE('',#28792,#6356);
#5465=LINE('',#28852,#6357);
#5466=LINE('',#28909,#6358);
#5467=LINE('',#28966,#6359);
#5468=LINE('',#29029,#6360);
#5469=LINE('',#29083,#6361);
#5470=LINE('',#29140,#6362);
#5471=LINE('',#29200,#6363);
#5472=LINE('',#29257,#6364);
#5473=LINE('',#29314,#6365);
#5474=LINE('',#29380,#6366);
#5475=LINE('',#29440,#6367);
#5476=LINE('',#29497,#6368);
#5477=LINE('',#29554,#6369);
#5478=LINE('',#29614,#6370);
#5479=LINE('',#29668,#6371);
#5480=LINE('',#29725,#6372);
#5481=LINE('',#29788,#6373);
#5482=LINE('',#29848,#6374);
#5483=LINE('',#29902,#6375);
#5484=LINE('',#29962,#6376);
#5485=LINE('',#30022,#6377);
#5486=LINE('',#30079,#6378);
#5487=LINE('',#30139,#6379);
#5488=LINE('',#30199,#6380);
#5489=LINE('',#30256,#6381);
#5490=LINE('',#30316,#6382);
#5491=LINE('',#30376,#6383);
#5492=LINE('',#30436,#6384);
#5493=LINE('',#30490,#6385);
#5494=LINE('',#30547,#6386);
#5495=LINE('',#30610,#6387);
#5496=LINE('',#30667,#6388);
#5497=LINE('',#30727,#6389);
#5498=LINE('',#30787,#6390);
#5499=LINE('',#30844,#6391);
#5500=LINE('',#30904,#6392);
#5501=LINE('',#30967,#6393);
#5502=LINE('',#31027,#6394);
#5503=LINE('',#31081,#6395);
#5504=LINE('',#31138,#6396);
#5505=LINE('',#31198,#6397);
#5506=LINE('',#31255,#6398);
#5507=LINE('',#31312,#6399);
#5508=LINE('',#31372,#6400);
#5509=LINE('',#31429,#6401);
#5510=LINE('',#31489,#6402);
#5511=LINE('',#31507,#6403);
#5512=LINE('',#31521,#6404);
#5513=LINE('',#31611,#6405);
#5514=LINE('',#31695,#6406);
#5515=LINE('',#31785,#6407);
#5516=LINE('',#31875,#6408);
#5517=LINE('',#31959,#6409);
#5518=LINE('',#32049,#6410);
#5519=LINE('',#32133,#6411);
#5520=LINE('',#32223,#6412);
#5521=LINE('',#32313,#6413);
#5522=LINE('',#32397,#6414);
#5523=LINE('',#32487,#6415);
#5524=LINE('',#32577,#6416);
#5525=LINE('',#32661,#6417);
#5526=LINE('',#32751,#6418);
#5527=LINE('',#32835,#6419);
#5528=LINE('',#32857,#6420);
#5529=LINE('',#32894,#6421);
#5530=LINE('',#32931,#6422);
#5531=LINE('',#32968,#6423);
#5532=LINE('',#33005,#6424);
#5533=LINE('',#33043,#6425);
#5534=LINE('',#33080,#6426);
#5535=LINE('',#33117,#6427);
#5536=LINE('',#33155,#6428);
#5537=LINE('',#33192,#6429);
#5538=LINE('',#33229,#6430);
#5539=LINE('',#33266,#6431);
#5540=LINE('',#33303,#6432);
#5541=LINE('',#33341,#6433);
#5542=LINE('',#33378,#6434);
#5543=LINE('',#33415,#6435);
#5544=LINE('',#33428,#6436);
#5545=LINE('',#33459,#6437);
#5546=LINE('',#33487,#6438);
#5547=LINE('',#33515,#6439);
#5548=LINE('',#33556,#6440);
#5549=LINE('',#33597,#6441);
#5550=LINE('',#33625,#6442);
#5551=LINE('',#33653,#6443);
#5552=LINE('',#33694,#6444);
#5553=LINE('',#33735,#6445);
#5554=LINE('',#33764,#6446);
#5555=LINE('',#33792,#6447);
#5556=LINE('',#33820,#6448);
#5557=LINE('',#33848,#6449);
#5558=LINE('',#33889,#6450);
#5559=LINE('',#33930,#6451);
#5560=LINE('',#33958,#6452);
#5561=LINE('',#33986,#6453);
#5562=LINE('',#34027,#6454);
#5563=LINE('',#34068,#6455);
#5564=LINE('',#34097,#6456);
#5565=LINE('',#34125,#6457);
#5566=LINE('',#34153,#6458);
#5567=LINE('',#34181,#6459);
#5568=LINE('',#34222,#6460);
#5569=LINE('',#34263,#6461);
#5570=LINE('',#34291,#6462);
#5571=LINE('',#34318,#6463);
#5572=LINE('',#34360,#6464);
#5573=LINE('',#34401,#6465);
#5574=LINE('',#34430,#6466);
#5575=LINE('',#34457,#6467);
#5576=LINE('',#34498,#6468);
#5577=LINE('',#34540,#6469);
#5578=LINE('',#34568,#6470);
#5579=LINE('',#34595,#6471);
#5580=LINE('',#34636,#6472);
#5581=LINE('',#34665,#6473);
#5582=LINE('',#34707,#6474);
#5583=LINE('',#34734,#6475);
#5584=LINE('',#34775,#6476);
#5585=LINE('',#34804,#6477);
#5586=LINE('',#34845,#6478);
#5587=LINE('',#34887,#6479);
#5588=LINE('',#34915,#6480);
#5589=LINE('',#34942,#6481);
#5590=LINE('',#34983,#6482);
#5591=LINE('',#35012,#6483);
#5592=LINE('',#35041,#6484);
#5593=LINE('',#35068,#6485);
#5594=LINE('',#35109,#6486);
#5595=LINE('',#35138,#6487);
#5596=LINE('',#35179,#6488);
#5597=LINE('',#35221,#6489);
#5598=LINE('',#35249,#6490);
#5599=LINE('',#35276,#6491);
#5600=LINE('',#35317,#6492);
#5601=LINE('',#35346,#6493);
#5602=LINE('',#35375,#6494);
#5603=LINE('',#35402,#6495);
#5604=LINE('',#35430,#6496);
#5605=LINE('',#35459,#6497);
#5606=LINE('',#35498,#6498);
#5607=LINE('',#35499,#6499);
#5608=LINE('',#35501,#6500);
#5609=LINE('',#35503,#6501);
#5610=LINE('',#42509,#6502);
#5611=LINE('',#42549,#6503);
#5612=LINE('',#42861,#6504);
#5613=LINE('',#42901,#6505);
#5614=LINE('',#43183,#6506);
#5615=LINE('',#43223,#6507);
#5616=LINE('',#43505,#6508);
#5617=LINE('',#43545,#6509);
#5618=LINE('',#43827,#6510);
#5619=LINE('',#43880,#6511);
#5620=LINE('',#44162,#6512);
#5621=LINE('',#44202,#6513);
#5622=LINE('',#44484,#6514);
#5623=LINE('',#44524,#6515);
#5624=LINE('',#44810,#6516);
#5625=LINE('',#44850,#6517);
#5626=LINE('',#45134,#6518);
#5627=LINE('',#45174,#6519);
#5628=LINE('',#45456,#6520);
#5629=LINE('',#45496,#6521);
#5630=LINE('',#45778,#6522);
#5631=LINE('',#45818,#6523);
#5632=LINE('',#46106,#6524);
#5633=LINE('',#46146,#6525);
#5634=LINE('',#46428,#6526);
#5635=LINE('',#46468,#6527);
#5636=LINE('',#46750,#6528);
#5637=LINE('',#46790,#6529);
#5638=LINE('',#47037,#6530);
#5639=LINE('',#47099,#6531);
#5640=LINE('',#47227,#6532);
#5641=LINE('',#47229,#6533);
#5642=LINE('',#47231,#6534);
#5643=LINE('',#47237,#6535);
#6334=VECTOR('',#22409,7.);
#6335=VECTOR('',#22412,7.);
#6336=VECTOR('',#22415,10.);
#6337=VECTOR('',#22418,7.);
#6338=VECTOR('',#22423,10.);
#6339=VECTOR('',#22428,10.);
#6340=VECTOR('',#22431,10.);
#6341=VECTOR('',#22436,7.);
#6342=VECTOR('',#22439,7.);
#6343=VECTOR('',#22442,7.);
#6344=VECTOR('',#22445,7.);
#6345=VECTOR('',#22448,7.);
#6346=VECTOR('',#22451,7.);
#6347=VECTOR('',#22454,7.);
#6348=VECTOR('',#22457,7.);
#6349=VECTOR('',#22460,7.);
#6350=VECTOR('',#22463,7.);
#6351=VECTOR('',#22466,7.);
#6352=VECTOR('',#22469,7.);
#6353=VECTOR('',#22472,7.);
#6354=VECTOR('',#22475,7.);
#6355=VECTOR('',#22478,7.);
#6356=VECTOR('',#22481,7.);
#6357=VECTOR('',#22484,7.);
#6358=VECTOR('',#22487,7.);
#6359=VECTOR('',#22490,7.);
#6360=VECTOR('',#22493,7.);
#6361=VECTOR('',#22496,7.);
#6362=VECTOR('',#22499,7.);
#6363=VECTOR('',#22502,7.);
#6364=VECTOR('',#22505,7.);
#6365=VECTOR('',#22508,7.);
#6366=VECTOR('',#22511,7.);
#6367=VECTOR('',#22514,7.);
#6368=VECTOR('',#22517,7.);
#6369=VECTOR('',#22520,7.);
#6370=VECTOR('',#22523,7.);
#6371=VECTOR('',#22526,7.);
#6372=VECTOR('',#22529,7.);
#6373=VECTOR('',#22532,7.);
#6374=VECTOR('',#22535,7.);
#6375=VECTOR('',#22538,7.);
#6376=VECTOR('',#22541,7.);
#6377=VECTOR('',#22544,7.);
#6378=VECTOR('',#22547,7.);
#6379=VECTOR('',#22550,7.);
#6380=VECTOR('',#22553,7.);
#6381=VECTOR('',#22556,7.);
#6382=VECTOR('',#22559,7.);
#6383=VECTOR('',#22562,7.);
#6384=VECTOR('',#22565,7.);
#6385=VECTOR('',#22568,7.);
#6386=VECTOR('',#22571,7.);
#6387=VECTOR('',#22574,7.);
#6388=VECTOR('',#22577,7.);
#6389=VECTOR('',#22580,7.);
#6390=VECTOR('',#22583,7.);
#6391=VECTOR('',#22586,7.);
#6392=VECTOR('',#22589,7.);
#6393=VECTOR('',#22592,7.);
#6394=VECTOR('',#22595,7.);
#6395=VECTOR('',#22598,7.);
#6396=VECTOR('',#22601,7.);
#6397=VECTOR('',#22604,7.);
#6398=VECTOR('',#22607,7.);
#6399=VECTOR('',#22610,7.);
#6400=VECTOR('',#22613,7.);
#6401=VECTOR('',#22616,7.);
#6402=VECTOR('',#22619,7.);
#6403=VECTOR('',#22622,7.);
#6404=VECTOR('',#22629,7.);
#6405=VECTOR('',#22632,7.);
#6406=VECTOR('',#22635,7.);
#6407=VECTOR('',#22638,7.);
#6408=VECTOR('',#22641,7.);
#6409=VECTOR('',#22644,7.);
#6410=VECTOR('',#22647,7.);
#6411=VECTOR('',#22650,7.);
#6412=VECTOR('',#22653,7.);
#6413=VECTOR('',#22656,7.);
#6414=VECTOR('',#22659,7.);
#6415=VECTOR('',#22662,7.);
#6416=VECTOR('',#22665,7.);
#6417=VECTOR('',#22668,7.);
#6418=VECTOR('',#22671,7.);
#6419=VECTOR('',#22674,6.21925);
#6420=VECTOR('',#22679,6.21925);
#6421=VECTOR('',#22682,6.21925);
#6422=VECTOR('',#22685,6.21925);
#6423=VECTOR('',#22688,6.21925);
#6424=VECTOR('',#22691,6.21925);
#6425=VECTOR('',#22694,6.21925);
#6426=VECTOR('',#22697,6.21925);
#6427=VECTOR('',#22700,6.21925);
#6428=VECTOR('',#22703,6.21925);
#6429=VECTOR('',#22706,6.21925);
#6430=VECTOR('',#22709,6.21925);
#6431=VECTOR('',#22712,6.21925);
#6432=VECTOR('',#22715,6.21925);
#6433=VECTOR('',#22718,6.21925);
#6434=VECTOR('',#22721,6.21925);
#6435=VECTOR('',#22724,6.21925);
#6436=VECTOR('',#22729,6.21925);
#6437=VECTOR('',#22734,6.21925);
#6438=VECTOR('',#22737,6.21925);
#6439=VECTOR('',#22740,6.21925);
#6440=VECTOR('',#22743,6.21925);
#6441=VECTOR('',#22746,6.21925);
#6442=VECTOR('',#22749,6.21925);
#6443=VECTOR('',#22752,6.21925);
#6444=VECTOR('',#22755,6.21925);
#6445=VECTOR('',#22758,6.21925);
#6446=VECTOR('',#22761,6.21925);
#6447=VECTOR('',#22764,6.21925);
#6448=VECTOR('',#22767,6.21925);
#6449=VECTOR('',#22770,6.21925);
#6450=VECTOR('',#22773,6.21925);
#6451=VECTOR('',#22776,6.21925);
#6452=VECTOR('',#22779,6.21925);
#6453=VECTOR('',#22782,6.21925);
#6454=VECTOR('',#22785,6.21925);
#6455=VECTOR('',#22788,6.21925);
#6456=VECTOR('',#22791,6.21925);
#6457=VECTOR('',#22794,6.21925);
#6458=VECTOR('',#22797,6.21925);
#6459=VECTOR('',#22800,6.21925);
#6460=VECTOR('',#22803,6.21925);
#6461=VECTOR('',#22806,6.21925);
#6462=VECTOR('',#22809,6.21925);
#6463=VECTOR('',#22812,6.21925);
#6464=VECTOR('',#22815,6.21925);
#6465=VECTOR('',#22818,6.21925);
#6466=VECTOR('',#22821,6.21925);
#6467=VECTOR('',#22824,6.21925);
#6468=VECTOR('',#22827,6.21925);
#6469=VECTOR('',#22830,6.21925);
#6470=VECTOR('',#22833,6.21925);
#6471=VECTOR('',#22836,6.21925);
#6472=VECTOR('',#22839,6.21925);
#6473=VECTOR('',#22842,6.21925);
#6474=VECTOR('',#22845,6.21925);
#6475=VECTOR('',#22848,6.21925);
#6476=VECTOR('',#22851,6.21925);
#6477=VECTOR('',#22854,6.21925);
#6478=VECTOR('',#22857,6.21925);
#6479=VECTOR('',#22860,6.21925);
#6480=VECTOR('',#22863,6.21925);
#6481=VECTOR('',#22866,6.21925);
#6482=VECTOR('',#22869,6.21925);
#6483=VECTOR('',#22872,6.21925);
#6484=VECTOR('',#22875,6.21925);
#6485=VECTOR('',#22878,6.21925);
#6486=VECTOR('',#22881,6.21925);
#6487=VECTOR('',#22884,6.21925);
#6488=VECTOR('',#22887,6.21925);
#6489=VECTOR('',#22890,6.21925);
#6490=VECTOR('',#22893,6.21925);
#6491=VECTOR('',#22896,6.21925);
#6492=VECTOR('',#22899,6.21925);
#6493=VECTOR('',#22902,6.21925);
#6494=VECTOR('',#22905,6.21925);
#6495=VECTOR('',#22908,6.21925);
#6496=VECTOR('',#22911,6.21925);
#6497=VECTOR('',#22914,6.21925);
#6498=VECTOR('',#22917,10.);
#6499=VECTOR('',#22918,10.);
#6500=VECTOR('',#22921,10.);
#6501=VECTOR('',#22924,10.);
#6502=VECTOR('',#22961,10.);
#6503=VECTOR('',#22964,10.);
#6504=VECTOR('',#22997,10.);
#6505=VECTOR('',#23000,10.);
#6506=VECTOR('',#23027,10.);
#6507=VECTOR('',#23030,10.);
#6508=VECTOR('',#23057,10.);
#6509=VECTOR('',#23060,10.);
#6510=VECTOR('',#23087,10.);
#6511=VECTOR('',#23090,10.);
#6512=VECTOR('',#23117,10.);
#6513=VECTOR('',#23120,10.);
#6514=VECTOR('',#23147,10.);
#6515=VECTOR('',#23150,10.);
#6516=VECTOR('',#23179,10.);
#6517=VECTOR('',#23182,10.);
#6518=VECTOR('',#23211,10.);
#6519=VECTOR('',#23214,10.);
#6520=VECTOR('',#23241,10.);
#6521=VECTOR('',#23244,10.);
#6522=VECTOR('',#23271,10.);
#6523=VECTOR('',#23274,10.);
#6524=VECTOR('',#23301,10.);
#6525=VECTOR('',#23304,10.);
#6526=VECTOR('',#23331,10.);
#6527=VECTOR('',#23334,10.);
#6528=VECTOR('',#23361,10.);
#6529=VECTOR('',#23364,10.);
#6530=VECTOR('',#23385,10.);
#6531=VECTOR('',#23396,10.);
#6532=VECTOR('',#23415,6.5);
#6533=VECTOR('',#23418,8.5625);
#6534=VECTOR('',#23421,8.5625);
#6535=VECTOR('',#23430,6.5);
#7226=VERTEX_POINT('',#27822);
#7227=VERTEX_POINT('',#27823);
#7228=VERTEX_POINT('',#27825);
#7229=VERTEX_POINT('',#27851);
#7230=VERTEX_POINT('',#27853);
#7231=VERTEX_POINT('',#27855);
#7232=VERTEX_POINT('',#27857);
#7233=VERTEX_POINT('',#27859);
#7234=VERTEX_POINT('',#27861);
#7235=VERTEX_POINT('',#27864);
#7236=VERTEX_POINT('',#27866);
#7237=VERTEX_POINT('',#27869);
#7238=VERTEX_POINT('',#27893);
#7239=VERTEX_POINT('',#27894);
#7240=VERTEX_POINT('',#27896);
#7241=VERTEX_POINT('',#27898);
#7242=VERTEX_POINT('',#27902);
#7243=VERTEX_POINT('',#27903);
#7244=VERTEX_POINT('',#27962);
#7245=VERTEX_POINT('',#27963);
#7246=VERTEX_POINT('',#28022);
#7247=VERTEX_POINT('',#28023);
#7248=VERTEX_POINT('',#28079);
#7249=VERTEX_POINT('',#28080);
#7250=VERTEX_POINT('',#28139);
#7251=VERTEX_POINT('',#28140);
#7252=VERTEX_POINT('',#28199);
#7253=VERTEX_POINT('',#28200);
#7254=VERTEX_POINT('',#28259);
#7255=VERTEX_POINT('',#28260);
#7256=VERTEX_POINT('',#28316);
#7257=VERTEX_POINT('',#28317);
#7258=VERTEX_POINT('',#28373);
#7259=VERTEX_POINT('',#28374);
#7260=VERTEX_POINT('',#28436);
#7261=VERTEX_POINT('',#28437);
#7262=VERTEX_POINT('',#28490);
#7263=VERTEX_POINT('',#28491);
#7264=VERTEX_POINT('',#28550);
#7265=VERTEX_POINT('',#28551);
#7266=VERTEX_POINT('',#28610);
#7267=VERTEX_POINT('',#28611);
#7268=VERTEX_POINT('',#28667);
#7269=VERTEX_POINT('',#28668);
#7270=VERTEX_POINT('',#28724);
#7271=VERTEX_POINT('',#28725);
#7272=VERTEX_POINT('',#28790);
#7273=VERTEX_POINT('',#28791);
#7274=VERTEX_POINT('',#28850);
#7275=VERTEX_POINT('',#28851);
#7276=VERTEX_POINT('',#28907);
#7277=VERTEX_POINT('',#28908);
#7278=VERTEX_POINT('',#28964);
#7279=VERTEX_POINT('',#28965);
#7280=VERTEX_POINT('',#29027);
#7281=VERTEX_POINT('',#29028);
#7282=VERTEX_POINT('',#29081);
#7283=VERTEX_POINT('',#29082);
#7284=VERTEX_POINT('',#29138);
#7285=VERTEX_POINT('',#29139);
#7286=VERTEX_POINT('',#29198);
#7287=VERTEX_POINT('',#29199);
#7288=VERTEX_POINT('',#29255);
#7289=VERTEX_POINT('',#29256);
#7290=VERTEX_POINT('',#29312);
#7291=VERTEX_POINT('',#29313);
#7292=VERTEX_POINT('',#29378);
#7293=VERTEX_POINT('',#29379);
#7294=VERTEX_POINT('',#29438);
#7295=VERTEX_POINT('',#29439);
#7296=VERTEX_POINT('',#29495);
#7297=VERTEX_POINT('',#29496);
#7298=VERTEX_POINT('',#29552);
#7299=VERTEX_POINT('',#29553);
#7300=VERTEX_POINT('',#29612);
#7301=VERTEX_POINT('',#29613);
#7302=VERTEX_POINT('',#29666);
#7303=VERTEX_POINT('',#29667);
#7304=VERTEX_POINT('',#29723);
#7305=VERTEX_POINT('',#29724);
#7306=VERTEX_POINT('',#29786);
#7307=VERTEX_POINT('',#29787);
#7308=VERTEX_POINT('',#29846);
#7309=VERTEX_POINT('',#29847);
#7310=VERTEX_POINT('',#29900);
#7311=VERTEX_POINT('',#29901);
#7312=VERTEX_POINT('',#29960);
#7313=VERTEX_POINT('',#29961);
#7314=VERTEX_POINT('',#30020);
#7315=VERTEX_POINT('',#30021);
#7316=VERTEX_POINT('',#30077);
#7317=VERTEX_POINT('',#30078);
#7318=VERTEX_POINT('',#30137);
#7319=VERTEX_POINT('',#30138);
#7320=VERTEX_POINT('',#30197);
#7321=VERTEX_POINT('',#30198);
#7322=VERTEX_POINT('',#30254);
#7323=VERTEX_POINT('',#30255);
#7324=VERTEX_POINT('',#30314);
#7325=VERTEX_POINT('',#30315);
#7326=VERTEX_POINT('',#30374);
#7327=VERTEX_POINT('',#30375);
#7328=VERTEX_POINT('',#30434);
#7329=VERTEX_POINT('',#30435);
#7330=VERTEX_POINT('',#30488);
#7331=VERTEX_POINT('',#30489);
#7332=VERTEX_POINT('',#30545);
#7333=VERTEX_POINT('',#30546);
#7334=VERTEX_POINT('',#30608);
#7335=VERTEX_POINT('',#30609);
#7336=VERTEX_POINT('',#30665);
#7337=VERTEX_POINT('',#30666);
#7338=VERTEX_POINT('',#30725);
#7339=VERTEX_POINT('',#30726);
#7340=VERTEX_POINT('',#30785);
#7341=VERTEX_POINT('',#30786);
#7342=VERTEX_POINT('',#30842);
#7343=VERTEX_POINT('',#30843);
#7344=VERTEX_POINT('',#30902);
#7345=VERTEX_POINT('',#30903);
#7346=VERTEX_POINT('',#30965);
#7347=VERTEX_POINT('',#30966);
#7348=VERTEX_POINT('',#31025);
#7349=VERTEX_POINT('',#31026);
#7350=VERTEX_POINT('',#31079);
#7351=VERTEX_POINT('',#31080);
#7352=VERTEX_POINT('',#31136);
#7353=VERTEX_POINT('',#31137);
#7354=VERTEX_POINT('',#31196);
#7355=VERTEX_POINT('',#31197);
#7356=VERTEX_POINT('',#31253);
#7357=VERTEX_POINT('',#31254);
#7358=VERTEX_POINT('',#31310);
#7359=VERTEX_POINT('',#31311);
#7360=VERTEX_POINT('',#31370);
#7361=VERTEX_POINT('',#31371);
#7362=VERTEX_POINT('',#31427);
#7363=VERTEX_POINT('',#31428);
#7364=VERTEX_POINT('',#31487);
#7365=VERTEX_POINT('',#31488);
#7366=VERTEX_POINT('',#31490);
#7367=VERTEX_POINT('',#31504);
#7368=VERTEX_POINT('',#31506);
#7369=VERTEX_POINT('',#31509);
#7370=VERTEX_POINT('',#31519);
#7371=VERTEX_POINT('',#31520);
#7372=VERTEX_POINT('',#31609);
#7373=VERTEX_POINT('',#31610);
#7374=VERTEX_POINT('',#31693);
#7375=VERTEX_POINT('',#31694);
#7376=VERTEX_POINT('',#31783);
#7377=VERTEX_POINT('',#31784);
#7378=VERTEX_POINT('',#31873);
#7379=VERTEX_POINT('',#31874);
#7380=VERTEX_POINT('',#31957);
#7381=VERTEX_POINT('',#31958);
#7382=VERTEX_POINT('',#32047);
#7383=VERTEX_POINT('',#32048);
#7384=VERTEX_POINT('',#32131);
#7385=VERTEX_POINT('',#32132);
#7386=VERTEX_POINT('',#32221);
#7387=VERTEX_POINT('',#32222);
#7388=VERTEX_POINT('',#32311);
#7389=VERTEX_POINT('',#32312);
#7390=VERTEX_POINT('',#32395);
#7391=VERTEX_POINT('',#32396);
#7392=VERTEX_POINT('',#32485);
#7393=VERTEX_POINT('',#32486);
#7394=VERTEX_POINT('',#32575);
#7395=VERTEX_POINT('',#32576);
#7396=VERTEX_POINT('',#32659);
#7397=VERTEX_POINT('',#32660);
#7398=VERTEX_POINT('',#32749);
#7399=VERTEX_POINT('',#32750);
#7400=VERTEX_POINT('',#32833);
#7401=VERTEX_POINT('',#32834);
#7402=VERTEX_POINT('',#32836);
#7403=VERTEX_POINT('',#32846);
#7404=VERTEX_POINT('',#32855);
#7405=VERTEX_POINT('',#32856);
#7406=VERTEX_POINT('',#32892);
#7407=VERTEX_POINT('',#32893);
#7408=VERTEX_POINT('',#32929);
#7409=VERTEX_POINT('',#32930);
#7410=VERTEX_POINT('',#32966);
#7411=VERTEX_POINT('',#32967);
#7412=VERTEX_POINT('',#33003);
#7413=VERTEX_POINT('',#33004);
#7414=VERTEX_POINT('',#33041);
#7415=VERTEX_POINT('',#33042);
#7416=VERTEX_POINT('',#33078);
#7417=VERTEX_POINT('',#33079);
#7418=VERTEX_POINT('',#33115);
#7419=VERTEX_POINT('',#33116);
#7420=VERTEX_POINT('',#33153);
#7421=VERTEX_POINT('',#33154);
#7422=VERTEX_POINT('',#33190);
#7423=VERTEX_POINT('',#33191);
#7424=VERTEX_POINT('',#33227);
#7425=VERTEX_POINT('',#33228);
#7426=VERTEX_POINT('',#33264);
#7427=VERTEX_POINT('',#33265);
#7428=VERTEX_POINT('',#33301);
#7429=VERTEX_POINT('',#33302);
#7430=VERTEX_POINT('',#33339);
#7431=VERTEX_POINT('',#33340);
#7432=VERTEX_POINT('',#33376);
#7433=VERTEX_POINT('',#33377);
#7434=VERTEX_POINT('',#33413);
#7435=VERTEX_POINT('',#33414);
#7436=VERTEX_POINT('',#33416);
#7437=VERTEX_POINT('',#33426);
#7438=VERTEX_POINT('',#33427);
#7439=VERTEX_POINT('',#33441);
#7440=VERTEX_POINT('',#33457);
#7441=VERTEX_POINT('',#33458);
#7442=VERTEX_POINT('',#33485);
#7443=VERTEX_POINT('',#33486);
#7444=VERTEX_POINT('',#33513);
#7445=VERTEX_POINT('',#33514);
#7446=VERTEX_POINT('',#33554);
#7447=VERTEX_POINT('',#33555);
#7448=VERTEX_POINT('',#33595);
#7449=VERTEX_POINT('',#33596);
#7450=VERTEX_POINT('',#33623);
#7451=VERTEX_POINT('',#33624);
#7452=VERTEX_POINT('',#33651);
#7453=VERTEX_POINT('',#33652);
#7454=VERTEX_POINT('',#33692);
#7455=VERTEX_POINT('',#33693);
#7456=VERTEX_POINT('',#33733);
#7457=VERTEX_POINT('',#33734);
#7458=VERTEX_POINT('',#33762);
#7459=VERTEX_POINT('',#33763);
#7460=VERTEX_POINT('',#33790);
#7461=VERTEX_POINT('',#33791);
#7462=VERTEX_POINT('',#33818);
#7463=VERTEX_POINT('',#33819);
#7464=VERTEX_POINT('',#33846);
#7465=VERTEX_POINT('',#33847);
#7466=VERTEX_POINT('',#33887);
#7467=VERTEX_POINT('',#33888);
#7468=VERTEX_POINT('',#33928);
#7469=VERTEX_POINT('',#33929);
#7470=VERTEX_POINT('',#33956);
#7471=VERTEX_POINT('',#33957);
#7472=VERTEX_POINT('',#33984);
#7473=VERTEX_POINT('',#33985);
#7474=VERTEX_POINT('',#34025);
#7475=VERTEX_POINT('',#34026);
#7476=VERTEX_POINT('',#34066);
#7477=VERTEX_POINT('',#34067);
#7478=VERTEX_POINT('',#34095);
#7479=VERTEX_POINT('',#34096);
#7480=VERTEX_POINT('',#34123);
#7481=VERTEX_POINT('',#34124);
#7482=VERTEX_POINT('',#34151);
#7483=VERTEX_POINT('',#34152);
#7484=VERTEX_POINT('',#34179);
#7485=VERTEX_POINT('',#34180);
#7486=VERTEX_POINT('',#34220);
#7487=VERTEX_POINT('',#34221);
#7488=VERTEX_POINT('',#34261);
#7489=VERTEX_POINT('',#34262);
#7490=VERTEX_POINT('',#34289);
#7491=VERTEX_POINT('',#34290);
#7492=VERTEX_POINT('',#34316);
#7493=VERTEX_POINT('',#34317);
#7494=VERTEX_POINT('',#34358);
#7495=VERTEX_POINT('',#34359);
#7496=VERTEX_POINT('',#34399);
#7497=VERTEX_POINT('',#34400);
#7498=VERTEX_POINT('',#34428);
#7499=VERTEX_POINT('',#34429);
#7500=VERTEX_POINT('',#34455);
#7501=VERTEX_POINT('',#34456);
#7502=VERTEX_POINT('',#34496);
#7503=VERTEX_POINT('',#34497);
#7504=VERTEX_POINT('',#34538);
#7505=VERTEX_POINT('',#34539);
#7506=VERTEX_POINT('',#34566);
#7507=VERTEX_POINT('',#34567);
#7508=VERTEX_POINT('',#34593);
#7509=VERTEX_POINT('',#34594);
#7510=VERTEX_POINT('',#34634);
#7511=VERTEX_POINT('',#34635);
#7512=VERTEX_POINT('',#34663);
#7513=VERTEX_POINT('',#34664);
#7514=VERTEX_POINT('',#34705);
#7515=VERTEX_POINT('',#34706);
#7516=VERTEX_POINT('',#34732);
#7517=VERTEX_POINT('',#34733);
#7518=VERTEX_POINT('',#34773);
#7519=VERTEX_POINT('',#34774);
#7520=VERTEX_POINT('',#34802);
#7521=VERTEX_POINT('',#34803);
#7522=VERTEX_POINT('',#34843);
#7523=VERTEX_POINT('',#34844);
#7524=VERTEX_POINT('',#34885);
#7525=VERTEX_POINT('',#34886);
#7526=VERTEX_POINT('',#34913);
#7527=VERTEX_POINT('',#34914);
#7528=VERTEX_POINT('',#34940);
#7529=VERTEX_POINT('',#34941);
#7530=VERTEX_POINT('',#34981);
#7531=VERTEX_POINT('',#34982);
#7532=VERTEX_POINT('',#35010);
#7533=VERTEX_POINT('',#35011);
#7534=VERTEX_POINT('',#35039);
#7535=VERTEX_POINT('',#35040);
#7536=VERTEX_POINT('',#35066);
#7537=VERTEX_POINT('',#35067);
#7538=VERTEX_POINT('',#35107);
#7539=VERTEX_POINT('',#35108);
#7540=VERTEX_POINT('',#35136);
#7541=VERTEX_POINT('',#35137);
#7542=VERTEX_POINT('',#35177);
#7543=VERTEX_POINT('',#35178);
#7544=VERTEX_POINT('',#35219);
#7545=VERTEX_POINT('',#35220);
#7546=VERTEX_POINT('',#35247);
#7547=VERTEX_POINT('',#35248);
#7548=VERTEX_POINT('',#35274);
#7549=VERTEX_POINT('',#35275);
#7550=VERTEX_POINT('',#35315);
#7551=VERTEX_POINT('',#35316);
#7552=VERTEX_POINT('',#35344);
#7553=VERTEX_POINT('',#35345);
#7554=VERTEX_POINT('',#35373);
#7555=VERTEX_POINT('',#35374);
#7556=VERTEX_POINT('',#35400);
#7557=VERTEX_POINT('',#35401);
#7558=VERTEX_POINT('',#35428);
#7559=VERTEX_POINT('',#35429);
#7560=VERTEX_POINT('',#35457);
#7561=VERTEX_POINT('',#35458);
#7562=VERTEX_POINT('',#35506);
#7563=VERTEX_POINT('',#35622);
#7564=VERTEX_POINT('',#35624);
#7565=VERTEX_POINT('',#37812);
#7566=VERTEX_POINT('',#37935);
#7567=VERTEX_POINT('',#40131);
#7568=VERTEX_POINT('',#40244);
#7569=VERTEX_POINT('',#40246);
#7570=VERTEX_POINT('',#41236);
#7571=VERTEX_POINT('',#41364);
#7572=VERTEX_POINT('',#42363);
#7573=VERTEX_POINT('',#42364);
#7574=VERTEX_POINT('',#42366);
#7575=VERTEX_POINT('',#42396);
#7576=VERTEX_POINT('',#42503);
#7577=VERTEX_POINT('',#42508);
#7578=VERTEX_POINT('',#42510);
#7579=VERTEX_POINT('',#42536);
#7580=VERTEX_POINT('',#42548);
#7581=VERTEX_POINT('',#42631);
#7582=VERTEX_POINT('',#42639);
#7583=VERTEX_POINT('',#42644);
#7584=VERTEX_POINT('',#42684);
#7585=VERTEX_POINT('',#42686);
#7586=VERTEX_POINT('',#42693);
#7587=VERTEX_POINT('',#42695);
#7588=VERTEX_POINT('',#42702);
#7589=VERTEX_POINT('',#42709);
#7590=VERTEX_POINT('',#42716);
#7591=VERTEX_POINT('',#42718);
#7592=VERTEX_POINT('',#42748);
#7593=VERTEX_POINT('',#42855);
#7594=VERTEX_POINT('',#42860);
#7595=VERTEX_POINT('',#42862);
#7596=VERTEX_POINT('',#42888);
#7597=VERTEX_POINT('',#42900);
#7598=VERTEX_POINT('',#43015);
#7599=VERTEX_POINT('',#43017);
#7600=VERTEX_POINT('',#43024);
#7601=VERTEX_POINT('',#43031);
#7602=VERTEX_POINT('',#43038);
#7603=VERTEX_POINT('',#43040);
#7604=VERTEX_POINT('',#43070);
#7605=VERTEX_POINT('',#43177);
#7606=VERTEX_POINT('',#43182);
#7607=VERTEX_POINT('',#43184);
#7608=VERTEX_POINT('',#43210);
#7609=VERTEX_POINT('',#43222);
#7610=VERTEX_POINT('',#43337);
#7611=VERTEX_POINT('',#43339);
#7612=VERTEX_POINT('',#43346);
#7613=VERTEX_POINT('',#43353);
#7614=VERTEX_POINT('',#43360);
#7615=VERTEX_POINT('',#43362);
#7616=VERTEX_POINT('',#43392);
#7617=VERTEX_POINT('',#43499);
#7618=VERTEX_POINT('',#43504);
#7619=VERTEX_POINT('',#43506);
#7620=VERTEX_POINT('',#43532);
#7621=VERTEX_POINT('',#43544);
#7622=VERTEX_POINT('',#43659);
#7623=VERTEX_POINT('',#43661);
#7624=VERTEX_POINT('',#43668);
#7625=VERTEX_POINT('',#43675);
#7626=VERTEX_POINT('',#43682);
#7627=VERTEX_POINT('',#43684);
#7628=VERTEX_POINT('',#43714);
#7629=VERTEX_POINT('',#43821);
#7630=VERTEX_POINT('',#43826);
#7631=VERTEX_POINT('',#43828);
#7632=VERTEX_POINT('',#43854);
#7633=VERTEX_POINT('',#43879);
#7634=VERTEX_POINT('',#43994);
#7635=VERTEX_POINT('',#43996);
#7636=VERTEX_POINT('',#44003);
#7637=VERTEX_POINT('',#44010);
#7638=VERTEX_POINT('',#44017);
#7639=VERTEX_POINT('',#44019);
#7640=VERTEX_POINT('',#44049);
#7641=VERTEX_POINT('',#44156);
#7642=VERTEX_POINT('',#44161);
#7643=VERTEX_POINT('',#44163);
#7644=VERTEX_POINT('',#44189);
#7645=VERTEX_POINT('',#44201);
#7646=VERTEX_POINT('',#44316);
#7647=VERTEX_POINT('',#44318);
#7648=VERTEX_POINT('',#44325);
#7649=VERTEX_POINT('',#44332);
#7650=VERTEX_POINT('',#44339);
#7651=VERTEX_POINT('',#44341);
#7652=VERTEX_POINT('',#44371);
#7653=VERTEX_POINT('',#44478);
#7654=VERTEX_POINT('',#44483);
#7655=VERTEX_POINT('',#44485);
#7656=VERTEX_POINT('',#44511);
#7657=VERTEX_POINT('',#44523);
#7658=VERTEX_POINT('',#44638);
#7659=VERTEX_POINT('',#44640);
#7660=VERTEX_POINT('',#44647);
#7661=VERTEX_POINT('',#44654);
#7662=VERTEX_POINT('',#44661);
#7663=VERTEX_POINT('',#44662);
#7664=VERTEX_POINT('',#44665);
#7665=VERTEX_POINT('',#44695);
#7666=VERTEX_POINT('',#44802);
#7667=VERTEX_POINT('',#44809);
#7668=VERTEX_POINT('',#44811);
#7669=VERTEX_POINT('',#44837);
#7670=VERTEX_POINT('',#44849);
#7671=VERTEX_POINT('',#44962);
#7672=VERTEX_POINT('',#44966);
#7673=VERTEX_POINT('',#44968);
#7674=VERTEX_POINT('',#44975);
#7675=VERTEX_POINT('',#44982);
#7676=VERTEX_POINT('',#44989);
#7677=VERTEX_POINT('',#44991);
#7678=VERTEX_POINT('',#45021);
#7679=VERTEX_POINT('',#45128);
#7680=VERTEX_POINT('',#45133);
#7681=VERTEX_POINT('',#45135);
#7682=VERTEX_POINT('',#45161);
#7683=VERTEX_POINT('',#45173);
#7684=VERTEX_POINT('',#45288);
#7685=VERTEX_POINT('',#45290);
#7686=VERTEX_POINT('',#45297);
#7687=VERTEX_POINT('',#45304);
#7688=VERTEX_POINT('',#45311);
#7689=VERTEX_POINT('',#45313);
#7690=VERTEX_POINT('',#45343);
#7691=VERTEX_POINT('',#45450);
#7692=VERTEX_POINT('',#45455);
#7693=VERTEX_POINT('',#45457);
#7694=VERTEX_POINT('',#45483);
#7695=VERTEX_POINT('',#45495);
#7696=VERTEX_POINT('',#45610);
#7697=VERTEX_POINT('',#45612);
#7698=VERTEX_POINT('',#45619);
#7699=VERTEX_POINT('',#45626);
#7700=VERTEX_POINT('',#45633);
#7701=VERTEX_POINT('',#45635);
#7702=VERTEX_POINT('',#45665);
#7703=VERTEX_POINT('',#45772);
#7704=VERTEX_POINT('',#45777);
#7705=VERTEX_POINT('',#45779);
#7706=VERTEX_POINT('',#45805);
#7707=VERTEX_POINT('',#45817);
#7708=VERTEX_POINT('',#45932);
#7709=VERTEX_POINT('',#45934);
#7710=VERTEX_POINT('',#45944);
#7711=VERTEX_POINT('',#45951);
#7712=VERTEX_POINT('',#45961);
#7713=VERTEX_POINT('',#45963);
#7714=VERTEX_POINT('',#45993);
#7715=VERTEX_POINT('',#46100);
#7716=VERTEX_POINT('',#46105);
#7717=VERTEX_POINT('',#46107);
#7718=VERTEX_POINT('',#46133);
#7719=VERTEX_POINT('',#46145);
#7720=VERTEX_POINT('',#46260);
#7721=VERTEX_POINT('',#46262);
#7722=VERTEX_POINT('',#46269);
#7723=VERTEX_POINT('',#46276);
#7724=VERTEX_POINT('',#46283);
#7725=VERTEX_POINT('',#46285);
#7726=VERTEX_POINT('',#46315);
#7727=VERTEX_POINT('',#46422);
#7728=VERTEX_POINT('',#46427);
#7729=VERTEX_POINT('',#46429);
#7730=VERTEX_POINT('',#46455);
#7731=VERTEX_POINT('',#46467);
#7732=VERTEX_POINT('',#46582);
#7733=VERTEX_POINT('',#46584);
#7734=VERTEX_POINT('',#46591);
#7735=VERTEX_POINT('',#46598);
#7736=VERTEX_POINT('',#46605);
#7737=VERTEX_POINT('',#46607);
#7738=VERTEX_POINT('',#46637);
#7739=VERTEX_POINT('',#46744);
#7740=VERTEX_POINT('',#46749);
#7741=VERTEX_POINT('',#46751);
#7742=VERTEX_POINT('',#46777);
#7743=VERTEX_POINT('',#46789);
#7744=VERTEX_POINT('',#46904);
#7745=VERTEX_POINT('',#46906);
#7746=VERTEX_POINT('',#46913);
#7747=VERTEX_POINT('',#46920);
#7748=VERTEX_POINT('',#47006);
#7749=VERTEX_POINT('',#47036);
#7750=VERTEX_POINT('',#47069);
#7751=VERTEX_POINT('',#47097);
#7752=VERTEX_POINT('',#47180);
#7753=VERTEX_POINT('',#47181);
#7754=VERTEX_POINT('',#47224);
#7755=VERTEX_POINT('',#47235);
#9127=EDGE_CURVE('',#7226,#7227,#5442,.T.);
#9128=EDGE_CURVE('',#7226,#7228,#4669,.T.);
#9129=EDGE_CURVE('',#7228,#7229,#3542,.T.);
#9130=EDGE_CURVE('',#7229,#7230,#5443,.T.);
#9131=EDGE_CURVE('',#7230,#7231,#3543,.T.);
#9132=EDGE_CURVE('',#7231,#7232,#5444,.T.);
#9133=EDGE_CURVE('',#7232,#7233,#3544,.T.);
#9134=EDGE_CURVE('',#7233,#7234,#5445,.T.);
#9135=EDGE_CURVE('',#7234,#7234,#3545,.F.);
#9136=EDGE_CURVE('',#7233,#7235,#3546,.T.);
#9137=EDGE_CURVE('',#7235,#7236,#5446,.T.);
#9138=EDGE_CURVE('',#7236,#7230,#3547,.T.);
#9139=EDGE_CURVE('',#7229,#7237,#3548,.T.);
#9140=EDGE_CURVE('',#7237,#7227,#4670,.T.);
#9141=EDGE_CURVE('',#7238,#7239,#5447,.T.);
#9142=EDGE_CURVE('',#7239,#7240,#3549,.T.);
#9143=EDGE_CURVE('',#7240,#7241,#5448,.T.);
#9144=EDGE_CURVE('',#7241,#7238,#3550,.T.);
#9145=EDGE_CURVE('',#7242,#7243,#5449,.T.);
#9146=EDGE_CURVE('',#7242,#7226,#4671,.T.);
#9147=EDGE_CURVE('',#7227,#7243,#4672,.T.);
#9148=EDGE_CURVE('',#7244,#7245,#5450,.T.);
#9149=EDGE_CURVE('',#7244,#7242,#4673,.T.);
#9150=EDGE_CURVE('',#7243,#7245,#4674,.T.);
#9151=EDGE_CURVE('',#7246,#7247,#5451,.T.);
#9152=EDGE_CURVE('',#7246,#7244,#4675,.T.);
#9153=EDGE_CURVE('',#7245,#7247,#4676,.T.);
#9154=EDGE_CURVE('',#7248,#7249,#5452,.T.);
#9155=EDGE_CURVE('',#7248,#7246,#4677,.T.);
#9156=EDGE_CURVE('',#7247,#7249,#4678,.T.);
#9157=EDGE_CURVE('',#7250,#7251,#5453,.T.);
#9158=EDGE_CURVE('',#7250,#7248,#4679,.T.);
#9159=EDGE_CURVE('',#7249,#7251,#4680,.T.);
#9160=EDGE_CURVE('',#7252,#7253,#5454,.T.);
#9161=EDGE_CURVE('',#7252,#7250,#4681,.T.);
#9162=EDGE_CURVE('',#7251,#7253,#4682,.T.);
#9163=EDGE_CURVE('',#7254,#7255,#5455,.T.);
#9164=EDGE_CURVE('',#7254,#7252,#4683,.T.);
#9165=EDGE_CURVE('',#7253,#7255,#4684,.T.);
#9166=EDGE_CURVE('',#7256,#7257,#5456,.T.);
#9167=EDGE_CURVE('',#7256,#7254,#4685,.T.);
#9168=EDGE_CURVE('',#7255,#7257,#4686,.T.);
#9169=EDGE_CURVE('',#7258,#7259,#5457,.T.);
#9170=EDGE_CURVE('',#7258,#7256,#4687,.T.);
#9171=EDGE_CURVE('',#7257,#7259,#4688,.T.);
#9172=EDGE_CURVE('',#7260,#7261,#5458,.T.);
#9173=EDGE_CURVE('',#7260,#7258,#4689,.T.);
#9174=EDGE_CURVE('',#7259,#7261,#4690,.T.);
#9175=EDGE_CURVE('',#7262,#7263,#5459,.T.);
#9176=EDGE_CURVE('',#7262,#7260,#4691,.T.);
#9177=EDGE_CURVE('',#7261,#7263,#4692,.T.);
#9178=EDGE_CURVE('',#7264,#7265,#5460,.T.);
#9179=EDGE_CURVE('',#7264,#7262,#4693,.T.);
#9180=EDGE_CURVE('',#7263,#7265,#4694,.T.);
#9181=EDGE_CURVE('',#7266,#7267,#5461,.T.);
#9182=EDGE_CURVE('',#7266,#7264,#4695,.T.);
#9183=EDGE_CURVE('',#7265,#7267,#4696,.T.);
#9184=EDGE_CURVE('',#7268,#7269,#5462,.T.);
#9185=EDGE_CURVE('',#7268,#7266,#4697,.T.);
#9186=EDGE_CURVE('',#7267,#7269,#4698,.T.);
#9187=EDGE_CURVE('',#7270,#7271,#5463,.T.);
#9188=EDGE_CURVE('',#7270,#7268,#4699,.T.);
#9189=EDGE_CURVE('',#7269,#7271,#4700,.T.);
#9190=EDGE_CURVE('',#7272,#7273,#5464,.T.);
#9191=EDGE_CURVE('',#7272,#7270,#4701,.T.);
#9192=EDGE_CURVE('',#7271,#7273,#4702,.T.);
#9193=EDGE_CURVE('',#7274,#7275,#5465,.T.);
#9194=EDGE_CURVE('',#7274,#7272,#4703,.T.);
#9195=EDGE_CURVE('',#7273,#7275,#4704,.T.);
#9196=EDGE_CURVE('',#7276,#7277,#5466,.T.);
#9197=EDGE_CURVE('',#7276,#7274,#4705,.T.);
#9198=EDGE_CURVE('',#7275,#7277,#4706,.T.);
#9199=EDGE_CURVE('',#7278,#7279,#5467,.T.);
#9200=EDGE_CURVE('',#7278,#7276,#4707,.T.);
#9201=EDGE_CURVE('',#7277,#7279,#4708,.T.);
#9202=EDGE_CURVE('',#7280,#7281,#5468,.T.);
#9203=EDGE_CURVE('',#7280,#7278,#4709,.T.);
#9204=EDGE_CURVE('',#7279,#7281,#4710,.T.);
#9205=EDGE_CURVE('',#7282,#7283,#5469,.T.);
#9206=EDGE_CURVE('',#7282,#7280,#4711,.T.);
#9207=EDGE_CURVE('',#7281,#7283,#4712,.T.);
#9208=EDGE_CURVE('',#7284,#7285,#5470,.T.);
#9209=EDGE_CURVE('',#7284,#7282,#4713,.T.);
#9210=EDGE_CURVE('',#7283,#7285,#4714,.T.);
#9211=EDGE_CURVE('',#7286,#7287,#5471,.T.);
#9212=EDGE_CURVE('',#7286,#7284,#4715,.T.);
#9213=EDGE_CURVE('',#7285,#7287,#4716,.T.);
#9214=EDGE_CURVE('',#7288,#7289,#5472,.T.);
#9215=EDGE_CURVE('',#7288,#7286,#4717,.T.);
#9216=EDGE_CURVE('',#7287,#7289,#4718,.T.);
#9217=EDGE_CURVE('',#7290,#7291,#5473,.T.);
#9218=EDGE_CURVE('',#7290,#7288,#4719,.T.);
#9219=EDGE_CURVE('',#7289,#7291,#4720,.T.);
#9220=EDGE_CURVE('',#7292,#7293,#5474,.T.);
#9221=EDGE_CURVE('',#7292,#7290,#4721,.T.);
#9222=EDGE_CURVE('',#7291,#7293,#4722,.T.);
#9223=EDGE_CURVE('',#7294,#7295,#5475,.T.);
#9224=EDGE_CURVE('',#7294,#7292,#4723,.T.);
#9225=EDGE_CURVE('',#7293,#7295,#4724,.T.);
#9226=EDGE_CURVE('',#7296,#7297,#5476,.T.);
#9227=EDGE_CURVE('',#7296,#7294,#4725,.T.);
#9228=EDGE_CURVE('',#7295,#7297,#4726,.T.);
#9229=EDGE_CURVE('',#7298,#7299,#5477,.T.);
#9230=EDGE_CURVE('',#7298,#7296,#4727,.T.);
#9231=EDGE_CURVE('',#7297,#7299,#4728,.T.);
#9232=EDGE_CURVE('',#7300,#7301,#5478,.T.);
#9233=EDGE_CURVE('',#7300,#7298,#4729,.T.);
#9234=EDGE_CURVE('',#7299,#7301,#4730,.T.);
#9235=EDGE_CURVE('',#7302,#7303,#5479,.T.);
#9236=EDGE_CURVE('',#7302,#7300,#4731,.T.);
#9237=EDGE_CURVE('',#7301,#7303,#4732,.T.);
#9238=EDGE_CURVE('',#7304,#7305,#5480,.T.);
#9239=EDGE_CURVE('',#7304,#7302,#4733,.T.);
#9240=EDGE_CURVE('',#7303,#7305,#4734,.T.);
#9241=EDGE_CURVE('',#7306,#7307,#5481,.T.);
#9242=EDGE_CURVE('',#7306,#7304,#4735,.T.);
#9243=EDGE_CURVE('',#7305,#7307,#4736,.T.);
#9244=EDGE_CURVE('',#7308,#7309,#5482,.T.);
#9245=EDGE_CURVE('',#7308,#7306,#4737,.T.);
#9246=EDGE_CURVE('',#7307,#7309,#4738,.T.);
#9247=EDGE_CURVE('',#7310,#7311,#5483,.T.);
#9248=EDGE_CURVE('',#7310,#7308,#4739,.T.);
#9249=EDGE_CURVE('',#7309,#7311,#4740,.T.);
#9250=EDGE_CURVE('',#7312,#7313,#5484,.T.);
#9251=EDGE_CURVE('',#7312,#7310,#4741,.T.);
#9252=EDGE_CURVE('',#7311,#7313,#4742,.T.);
#9253=EDGE_CURVE('',#7314,#7315,#5485,.T.);
#9254=EDGE_CURVE('',#7314,#7312,#4743,.T.);
#9255=EDGE_CURVE('',#7313,#7315,#4744,.T.);
#9256=EDGE_CURVE('',#7316,#7317,#5486,.T.);
#9257=EDGE_CURVE('',#7316,#7314,#4745,.T.);
#9258=EDGE_CURVE('',#7315,#7317,#4746,.T.);
#9259=EDGE_CURVE('',#7318,#7319,#5487,.T.);
#9260=EDGE_CURVE('',#7318,#7316,#4747,.T.);
#9261=EDGE_CURVE('',#7317,#7319,#4748,.T.);
#9262=EDGE_CURVE('',#7320,#7321,#5488,.T.);
#9263=EDGE_CURVE('',#7320,#7318,#4749,.T.);
#9264=EDGE_CURVE('',#7319,#7321,#4750,.T.);
#9265=EDGE_CURVE('',#7322,#7323,#5489,.T.);
#9266=EDGE_CURVE('',#7322,#7320,#4751,.T.);
#9267=EDGE_CURVE('',#7321,#7323,#4752,.T.);
#9268=EDGE_CURVE('',#7324,#7325,#5490,.T.);
#9269=EDGE_CURVE('',#7324,#7322,#4753,.T.);
#9270=EDGE_CURVE('',#7323,#7325,#4754,.T.);
#9271=EDGE_CURVE('',#7326,#7327,#5491,.T.);
#9272=EDGE_CURVE('',#7326,#7324,#4755,.T.);
#9273=EDGE_CURVE('',#7325,#7327,#4756,.T.);
#9274=EDGE_CURVE('',#7328,#7329,#5492,.T.);
#9275=EDGE_CURVE('',#7328,#7326,#4757,.T.);
#9276=EDGE_CURVE('',#7327,#7329,#4758,.T.);
#9277=EDGE_CURVE('',#7330,#7331,#5493,.T.);
#9278=EDGE_CURVE('',#7330,#7328,#4759,.T.);
#9279=EDGE_CURVE('',#7329,#7331,#4760,.T.);
#9280=EDGE_CURVE('',#7332,#7333,#5494,.T.);
#9281=EDGE_CURVE('',#7332,#7330,#4761,.T.);
#9282=EDGE_CURVE('',#7331,#7333,#4762,.T.);
#9283=EDGE_CURVE('',#7334,#7335,#5495,.T.);
#9284=EDGE_CURVE('',#7334,#7332,#4763,.T.);
#9285=EDGE_CURVE('',#7333,#7335,#4764,.T.);
#9286=EDGE_CURVE('',#7336,#7337,#5496,.T.);
#9287=EDGE_CURVE('',#7336,#7334,#4765,.T.);
#9288=EDGE_CURVE('',#7335,#7337,#4766,.T.);
#9289=EDGE_CURVE('',#7338,#7339,#5497,.T.);
#9290=EDGE_CURVE('',#7338,#7336,#4767,.T.);
#9291=EDGE_CURVE('',#7337,#7339,#4768,.T.);
#9292=EDGE_CURVE('',#7340,#7341,#5498,.T.);
#9293=EDGE_CURVE('',#7340,#7338,#4769,.T.);
#9294=EDGE_CURVE('',#7339,#7341,#4770,.T.);
#9295=EDGE_CURVE('',#7342,#7343,#5499,.T.);
#9296=EDGE_CURVE('',#7342,#7340,#4771,.T.);
#9297=EDGE_CURVE('',#7341,#7343,#4772,.T.);
#9298=EDGE_CURVE('',#7344,#7345,#5500,.T.);
#9299=EDGE_CURVE('',#7344,#7342,#4773,.T.);
#9300=EDGE_CURVE('',#7343,#7345,#4774,.T.);
#9301=EDGE_CURVE('',#7346,#7347,#5501,.T.);
#9302=EDGE_CURVE('',#7346,#7344,#4775,.T.);
#9303=EDGE_CURVE('',#7345,#7347,#4776,.T.);
#9304=EDGE_CURVE('',#7348,#7349,#5502,.T.);
#9305=EDGE_CURVE('',#7348,#7346,#4777,.T.);
#9306=EDGE_CURVE('',#7347,#7349,#4778,.T.);
#9307=EDGE_CURVE('',#7350,#7351,#5503,.T.);
#9308=EDGE_CURVE('',#7350,#7348,#4779,.T.);
#9309=EDGE_CURVE('',#7349,#7351,#4780,.T.);
#9310=EDGE_CURVE('',#7352,#7353,#5504,.T.);
#9311=EDGE_CURVE('',#7352,#7350,#4781,.T.);
#9312=EDGE_CURVE('',#7351,#7353,#4782,.T.);
#9313=EDGE_CURVE('',#7354,#7355,#5505,.T.);
#9314=EDGE_CURVE('',#7354,#7352,#4783,.T.);
#9315=EDGE_CURVE('',#7353,#7355,#4784,.T.);
#9316=EDGE_CURVE('',#7356,#7357,#5506,.T.);
#9317=EDGE_CURVE('',#7356,#7354,#4785,.T.);
#9318=EDGE_CURVE('',#7355,#7357,#4786,.T.);
#9319=EDGE_CURVE('',#7358,#7359,#5507,.T.);
#9320=EDGE_CURVE('',#7358,#7356,#4787,.T.);
#9321=EDGE_CURVE('',#7357,#7359,#4788,.T.);
#9322=EDGE_CURVE('',#7360,#7361,#5508,.T.);
#9323=EDGE_CURVE('',#7360,#7358,#4789,.T.);
#9324=EDGE_CURVE('',#7359,#7361,#4790,.T.);
#9325=EDGE_CURVE('',#7362,#7363,#5509,.T.);
#9326=EDGE_CURVE('',#7362,#7360,#4791,.T.);
#9327=EDGE_CURVE('',#7361,#7363,#4792,.T.);
#9328=EDGE_CURVE('',#7364,#7365,#5510,.T.);
#9329=EDGE_CURVE('',#7364,#7366,#4793,.T.);
#9330=EDGE_CURVE('',#7366,#7367,#3551,.T.);
#9331=EDGE_CURVE('',#7367,#7368,#5511,.T.);
#9332=EDGE_CURVE('',#7368,#7368,#3552,.T.);
#9333=EDGE_CURVE('',#7367,#7369,#3553,.T.);
#9334=EDGE_CURVE('',#7369,#7365,#4794,.T.);
#9335=EDGE_CURVE('',#7370,#7371,#5512,.T.);
#9336=EDGE_CURVE('',#7370,#7364,#4795,.T.);
#9337=EDGE_CURVE('',#7365,#7371,#4796,.T.);
#9338=EDGE_CURVE('',#7372,#7373,#5513,.T.);
#9339=EDGE_CURVE('',#7372,#7370,#4797,.T.);
#9340=EDGE_CURVE('',#7371,#7373,#4798,.T.);
#9341=EDGE_CURVE('',#7374,#7375,#5514,.T.);
#9342=EDGE_CURVE('',#7374,#7372,#4799,.T.);
#9343=EDGE_CURVE('',#7373,#7375,#4800,.T.);
#9344=EDGE_CURVE('',#7376,#7377,#5515,.T.);
#9345=EDGE_CURVE('',#7376,#7374,#4801,.T.);
#9346=EDGE_CURVE('',#7375,#7377,#4802,.T.);
#9347=EDGE_CURVE('',#7378,#7379,#5516,.T.);
#9348=EDGE_CURVE('',#7378,#7376,#4803,.T.);
#9349=EDGE_CURVE('',#7377,#7379,#4804,.T.);
#9350=EDGE_CURVE('',#7380,#7381,#5517,.T.);
#9351=EDGE_CURVE('',#7380,#7378,#4805,.T.);
#9352=EDGE_CURVE('',#7379,#7381,#4806,.T.);
#9353=EDGE_CURVE('',#7382,#7383,#5518,.T.);
#9354=EDGE_CURVE('',#7382,#7380,#4807,.T.);
#9355=EDGE_CURVE('',#7381,#7383,#4808,.T.);
#9356=EDGE_CURVE('',#7384,#7385,#5519,.T.);
#9357=EDGE_CURVE('',#7384,#7382,#4809,.T.);
#9358=EDGE_CURVE('',#7383,#7385,#4810,.T.);
#9359=EDGE_CURVE('',#7386,#7387,#5520,.T.);
#9360=EDGE_CURVE('',#7386,#7384,#4811,.T.);
#9361=EDGE_CURVE('',#7385,#7387,#4812,.T.);
#9362=EDGE_CURVE('',#7388,#7389,#5521,.T.);
#9363=EDGE_CURVE('',#7388,#7386,#4813,.T.);
#9364=EDGE_CURVE('',#7387,#7389,#4814,.T.);
#9365=EDGE_CURVE('',#7390,#7391,#5522,.T.);
#9366=EDGE_CURVE('',#7390,#7388,#4815,.T.);
#9367=EDGE_CURVE('',#7389,#7391,#4816,.T.);
#9368=EDGE_CURVE('',#7392,#7393,#5523,.T.);
#9369=EDGE_CURVE('',#7392,#7390,#4817,.T.);
#9370=EDGE_CURVE('',#7391,#7393,#4818,.T.);
#9371=EDGE_CURVE('',#7394,#7395,#5524,.T.);
#9372=EDGE_CURVE('',#7394,#7392,#4819,.T.);
#9373=EDGE_CURVE('',#7393,#7395,#4820,.T.);
#9374=EDGE_CURVE('',#7396,#7397,#5525,.T.);
#9375=EDGE_CURVE('',#7396,#7394,#4821,.T.);
#9376=EDGE_CURVE('',#7395,#7397,#4822,.T.);
#9377=EDGE_CURVE('',#7398,#7399,#5526,.T.);
#9378=EDGE_CURVE('',#7398,#7396,#4823,.T.);
#9379=EDGE_CURVE('',#7397,#7399,#4824,.T.);
#9380=EDGE_CURVE('',#7400,#7401,#5527,.T.);
#9381=EDGE_CURVE('',#7400,#7402,#4825,.T.);
#9382=EDGE_CURVE('',#7403,#7402,#3554,.T.);
#9383=EDGE_CURVE('',#7401,#7403,#4826,.T.);
#9384=EDGE_CURVE('',#7404,#7405,#5528,.T.);
#9385=EDGE_CURVE('',#7404,#7400,#4827,.T.);
#9386=EDGE_CURVE('',#7405,#7401,#4828,.T.);
#9387=EDGE_CURVE('',#7406,#7407,#5529,.T.);
#9388=EDGE_CURVE('',#7406,#7404,#4829,.T.);
#9389=EDGE_CURVE('',#7407,#7405,#4830,.T.);
#9390=EDGE_CURVE('',#7408,#7409,#5530,.T.);
#9391=EDGE_CURVE('',#7408,#7406,#4831,.T.);
#9392=EDGE_CURVE('',#7409,#7407,#4832,.T.);
#9393=EDGE_CURVE('',#7410,#7411,#5531,.T.);
#9394=EDGE_CURVE('',#7410,#7408,#4833,.T.);
#9395=EDGE_CURVE('',#7411,#7409,#4834,.T.);
#9396=EDGE_CURVE('',#7412,#7413,#5532,.T.);
#9397=EDGE_CURVE('',#7412,#7410,#4835,.T.);
#9398=EDGE_CURVE('',#7413,#7411,#4836,.T.);
#9399=EDGE_CURVE('',#7414,#7415,#5533,.T.);
#9400=EDGE_CURVE('',#7414,#7412,#4837,.T.);
#9401=EDGE_CURVE('',#7415,#7413,#4838,.T.);
#9402=EDGE_CURVE('',#7416,#7417,#5534,.T.);
#9403=EDGE_CURVE('',#7416,#7414,#4839,.T.);
#9404=EDGE_CURVE('',#7417,#7415,#4840,.T.);
#9405=EDGE_CURVE('',#7418,#7419,#5535,.T.);
#9406=EDGE_CURVE('',#7418,#7416,#4841,.T.);
#9407=EDGE_CURVE('',#7419,#7417,#4842,.T.);
#9408=EDGE_CURVE('',#7420,#7421,#5536,.T.);
#9409=EDGE_CURVE('',#7420,#7418,#4843,.T.);
#9410=EDGE_CURVE('',#7421,#7419,#4844,.T.);
#9411=EDGE_CURVE('',#7422,#7423,#5537,.T.);
#9412=EDGE_CURVE('',#7422,#7420,#4845,.T.);
#9413=EDGE_CURVE('',#7423,#7421,#4846,.T.);
#9414=EDGE_CURVE('',#7424,#7425,#5538,.T.);
#9415=EDGE_CURVE('',#7424,#7422,#4847,.T.);
#9416=EDGE_CURVE('',#7425,#7423,#4848,.T.);
#9417=EDGE_CURVE('',#7426,#7427,#5539,.T.);
#9418=EDGE_CURVE('',#7426,#7424,#4849,.T.);
#9419=EDGE_CURVE('',#7427,#7425,#4850,.T.);
#9420=EDGE_CURVE('',#7428,#7429,#5540,.T.);
#9421=EDGE_CURVE('',#7428,#7426,#4851,.T.);
#9422=EDGE_CURVE('',#7429,#7427,#4852,.T.);
#9423=EDGE_CURVE('',#7430,#7431,#5541,.T.);
#9424=EDGE_CURVE('',#7430,#7428,#4853,.T.);
#9425=EDGE_CURVE('',#7431,#7429,#4854,.T.);
#9426=EDGE_CURVE('',#7432,#7433,#5542,.T.);
#9427=EDGE_CURVE('',#7432,#7430,#4855,.T.);
#9428=EDGE_CURVE('',#7433,#7431,#4856,.T.);
#9429=EDGE_CURVE('',#7434,#7435,#5543,.T.);
#9430=EDGE_CURVE('',#7434,#7436,#4857,.T.);
#9431=EDGE_CURVE('',#7435,#7436,#3555,.T.);
#9432=EDGE_CURVE('',#7437,#7438,#5544,.T.);
#9433=EDGE_CURVE('',#7437,#7434,#4858,.T.);
#9434=EDGE_CURVE('',#7439,#7435,#3556,.T.);
#9435=EDGE_CURVE('',#7438,#7439,#4859,.T.);
#9436=EDGE_CURVE('',#7440,#7441,#5545,.T.);
#9437=EDGE_CURVE('',#7440,#7437,#4860,.T.);
#9438=EDGE_CURVE('',#7441,#7438,#4861,.T.);
#9439=EDGE_CURVE('',#7442,#7443,#5546,.T.);
#9440=EDGE_CURVE('',#7442,#7440,#4862,.T.);
#9441=EDGE_CURVE('',#7443,#7441,#4863,.T.);
#9442=EDGE_CURVE('',#7444,#7445,#5547,.T.);
#9443=EDGE_CURVE('',#7444,#7442,#4864,.T.);
#9444=EDGE_CURVE('',#7445,#7443,#4865,.T.);
#9445=EDGE_CURVE('',#7446,#7447,#5548,.T.);
#9446=EDGE_CURVE('',#7446,#7444,#4866,.T.);
#9447=EDGE_CURVE('',#7447,#7445,#4867,.T.);
#9448=EDGE_CURVE('',#7448,#7449,#5549,.T.);
#9449=EDGE_CURVE('',#7448,#7446,#4868,.T.);
#9450=EDGE_CURVE('',#7449,#7447,#4869,.T.);
#9451=EDGE_CURVE('',#7450,#7451,#5550,.T.);
#9452=EDGE_CURVE('',#7450,#7448,#4870,.T.);
#9453=EDGE_CURVE('',#7451,#7449,#4871,.T.);
#9454=EDGE_CURVE('',#7452,#7453,#5551,.T.);
#9455=EDGE_CURVE('',#7452,#7450,#4872,.T.);
#9456=EDGE_CURVE('',#7453,#7451,#4873,.T.);
#9457=EDGE_CURVE('',#7454,#7455,#5552,.T.);
#9458=EDGE_CURVE('',#7454,#7452,#4874,.T.);
#9459=EDGE_CURVE('',#7455,#7453,#4875,.T.);
#9460=EDGE_CURVE('',#7456,#7457,#5553,.T.);
#9461=EDGE_CURVE('',#7456,#7454,#4876,.T.);
#9462=EDGE_CURVE('',#7457,#7455,#4877,.T.);
#9463=EDGE_CURVE('',#7458,#7459,#5554,.T.);
#9464=EDGE_CURVE('',#7458,#7456,#4878,.T.);
#9465=EDGE_CURVE('',#7459,#7457,#4879,.T.);
#9466=EDGE_CURVE('',#7460,#7461,#5555,.T.);
#9467=EDGE_CURVE('',#7460,#7458,#4880,.T.);
#9468=EDGE_CURVE('',#7461,#7459,#4881,.T.);
#9469=EDGE_CURVE('',#7462,#7463,#5556,.T.);
#9470=EDGE_CURVE('',#7462,#7460,#4882,.T.);
#9471=EDGE_CURVE('',#7463,#7461,#4883,.T.);
#9472=EDGE_CURVE('',#7464,#7465,#5557,.T.);
#9473=EDGE_CURVE('',#7464,#7462,#4884,.T.);
#9474=EDGE_CURVE('',#7465,#7463,#4885,.T.);
#9475=EDGE_CURVE('',#7466,#7467,#5558,.T.);
#9476=EDGE_CURVE('',#7466,#7464,#4886,.T.);
#9477=EDGE_CURVE('',#7467,#7465,#4887,.T.);
#9478=EDGE_CURVE('',#7468,#7469,#5559,.T.);
#9479=EDGE_CURVE('',#7468,#7466,#4888,.T.);
#9480=EDGE_CURVE('',#7469,#7467,#4889,.T.);
#9481=EDGE_CURVE('',#7470,#7471,#5560,.T.);
#9482=EDGE_CURVE('',#7470,#7468,#4890,.T.);
#9483=EDGE_CURVE('',#7471,#7469,#4891,.T.);
#9484=EDGE_CURVE('',#7472,#7473,#5561,.T.);
#9485=EDGE_CURVE('',#7472,#7470,#4892,.T.);
#9486=EDGE_CURVE('',#7473,#7471,#4893,.T.);
#9487=EDGE_CURVE('',#7474,#7475,#5562,.T.);
#9488=EDGE_CURVE('',#7474,#7472,#4894,.T.);
#9489=EDGE_CURVE('',#7475,#7473,#4895,.T.);
#9490=EDGE_CURVE('',#7476,#7477,#5563,.T.);
#9491=EDGE_CURVE('',#7476,#7474,#4896,.T.);
#9492=EDGE_CURVE('',#7477,#7475,#4897,.T.);
#9493=EDGE_CURVE('',#7478,#7479,#5564,.T.);
#9494=EDGE_CURVE('',#7478,#7476,#4898,.T.);
#9495=EDGE_CURVE('',#7479,#7477,#4899,.T.);
#9496=EDGE_CURVE('',#7480,#7481,#5565,.T.);
#9497=EDGE_CURVE('',#7480,#7478,#4900,.T.);
#9498=EDGE_CURVE('',#7481,#7479,#4901,.T.);
#9499=EDGE_CURVE('',#7482,#7483,#5566,.T.);
#9500=EDGE_CURVE('',#7482,#7480,#4902,.T.);
#9501=EDGE_CURVE('',#7483,#7481,#4903,.T.);
#9502=EDGE_CURVE('',#7484,#7485,#5567,.T.);
#9503=EDGE_CURVE('',#7484,#7482,#4904,.T.);
#9504=EDGE_CURVE('',#7485,#7483,#4905,.T.);
#9505=EDGE_CURVE('',#7486,#7487,#5568,.T.);
#9506=EDGE_CURVE('',#7486,#7484,#4906,.T.);
#9507=EDGE_CURVE('',#7487,#7485,#4907,.T.);
#9508=EDGE_CURVE('',#7488,#7489,#5569,.T.);
#9509=EDGE_CURVE('',#7488,#7486,#4908,.T.);
#9510=EDGE_CURVE('',#7489,#7487,#4909,.T.);
#9511=EDGE_CURVE('',#7490,#7491,#5570,.T.);
#9512=EDGE_CURVE('',#7490,#7488,#4910,.T.);
#9513=EDGE_CURVE('',#7491,#7489,#4911,.T.);
#9514=EDGE_CURVE('',#7492,#7493,#5571,.T.);
#9515=EDGE_CURVE('',#7492,#7490,#4912,.T.);
#9516=EDGE_CURVE('',#7493,#7491,#4913,.T.);
#9517=EDGE_CURVE('',#7494,#7495,#5572,.T.);
#9518=EDGE_CURVE('',#7494,#7492,#4914,.T.);
#9519=EDGE_CURVE('',#7495,#7493,#4915,.T.);
#9520=EDGE_CURVE('',#7496,#7497,#5573,.T.);
#9521=EDGE_CURVE('',#7496,#7494,#4916,.T.);
#9522=EDGE_CURVE('',#7497,#7495,#4917,.T.);
#9523=EDGE_CURVE('',#7498,#7499,#5574,.T.);
#9524=EDGE_CURVE('',#7498,#7496,#4918,.T.);
#9525=EDGE_CURVE('',#7499,#7497,#4919,.T.);
#9526=EDGE_CURVE('',#7500,#7501,#5575,.T.);
#9527=EDGE_CURVE('',#7500,#7498,#4920,.T.);
#9528=EDGE_CURVE('',#7501,#7499,#4921,.T.);
#9529=EDGE_CURVE('',#7502,#7503,#5576,.T.);
#9530=EDGE_CURVE('',#7502,#7500,#4922,.T.);
#9531=EDGE_CURVE('',#7503,#7501,#4923,.T.);
#9532=EDGE_CURVE('',#7504,#7505,#5577,.T.);
#9533=EDGE_CURVE('',#7504,#7502,#4924,.T.);
#9534=EDGE_CURVE('',#7505,#7503,#4925,.T.);
#9535=EDGE_CURVE('',#7506,#7507,#5578,.T.);
#9536=EDGE_CURVE('',#7506,#7504,#4926,.T.);
#9537=EDGE_CURVE('',#7507,#7505,#4927,.T.);
#9538=EDGE_CURVE('',#7508,#7509,#5579,.T.);
#9539=EDGE_CURVE('',#7508,#7506,#4928,.T.);
#9540=EDGE_CURVE('',#7509,#7507,#4929,.T.);
#9541=EDGE_CURVE('',#7510,#7511,#5580,.T.);
#9542=EDGE_CURVE('',#7510,#7508,#4930,.T.);
#9543=EDGE_CURVE('',#7511,#7509,#4931,.T.);
#9544=EDGE_CURVE('',#7512,#7513,#5581,.T.);
#9545=EDGE_CURVE('',#7512,#7510,#4932,.T.);
#9546=EDGE_CURVE('',#7513,#7511,#4933,.T.);
#9547=EDGE_CURVE('',#7514,#7515,#5582,.T.);
#9548=EDGE_CURVE('',#7514,#7512,#4934,.T.);
#9549=EDGE_CURVE('',#7515,#7513,#4935,.T.);
#9550=EDGE_CURVE('',#7516,#7517,#5583,.T.);
#9551=EDGE_CURVE('',#7516,#7514,#4936,.T.);
#9552=EDGE_CURVE('',#7517,#7515,#4937,.T.);
#9553=EDGE_CURVE('',#7518,#7519,#5584,.T.);
#9554=EDGE_CURVE('',#7518,#7516,#4938,.T.);
#9555=EDGE_CURVE('',#7519,#7517,#4939,.T.);
#9556=EDGE_CURVE('',#7520,#7521,#5585,.T.);
#9557=EDGE_CURVE('',#7520,#7518,#4940,.T.);
#9558=EDGE_CURVE('',#7521,#7519,#4941,.T.);
#9559=EDGE_CURVE('',#7522,#7523,#5586,.T.);
#9560=EDGE_CURVE('',#7522,#7520,#4942,.T.);
#9561=EDGE_CURVE('',#7523,#7521,#4943,.T.);
#9562=EDGE_CURVE('',#7524,#7525,#5587,.T.);
#9563=EDGE_CURVE('',#7524,#7522,#4944,.T.);
#9564=EDGE_CURVE('',#7525,#7523,#4945,.T.);
#9565=EDGE_CURVE('',#7526,#7527,#5588,.T.);
#9566=EDGE_CURVE('',#7526,#7524,#4946,.T.);
#9567=EDGE_CURVE('',#7527,#7525,#4947,.T.);
#9568=EDGE_CURVE('',#7528,#7529,#5589,.T.);
#9569=EDGE_CURVE('',#7528,#7526,#4948,.T.);
#9570=EDGE_CURVE('',#7529,#7527,#4949,.T.);
#9571=EDGE_CURVE('',#7530,#7531,#5590,.T.);
#9572=EDGE_CURVE('',#7530,#7528,#4950,.T.);
#9573=EDGE_CURVE('',#7531,#7529,#4951,.T.);
#9574=EDGE_CURVE('',#7532,#7533,#5591,.T.);
#9575=EDGE_CURVE('',#7532,#7530,#4952,.T.);
#9576=EDGE_CURVE('',#7533,#7531,#4953,.T.);
#9577=EDGE_CURVE('',#7534,#7535,#5592,.T.);
#9578=EDGE_CURVE('',#7534,#7532,#4954,.T.);
#9579=EDGE_CURVE('',#7535,#7533,#4955,.T.);
#9580=EDGE_CURVE('',#7536,#7537,#5593,.T.);
#9581=EDGE_CURVE('',#7536,#7534,#4956,.T.);
#9582=EDGE_CURVE('',#7537,#7535,#4957,.T.);
#9583=EDGE_CURVE('',#7538,#7539,#5594,.T.);
#9584=EDGE_CURVE('',#7538,#7536,#4958,.T.);
#9585=EDGE_CURVE('',#7539,#7537,#4959,.T.);
#9586=EDGE_CURVE('',#7540,#7541,#5595,.T.);
#9587=EDGE_CURVE('',#7540,#7538,#4960,.T.);
#9588=EDGE_CURVE('',#7541,#7539,#4961,.T.);
#9589=EDGE_CURVE('',#7542,#7543,#5596,.T.);
#9590=EDGE_CURVE('',#7542,#7540,#4962,.T.);
#9591=EDGE_CURVE('',#7543,#7541,#4963,.T.);
#9592=EDGE_CURVE('',#7544,#7545,#5597,.T.);
#9593=EDGE_CURVE('',#7544,#7542,#4964,.T.);
#9594=EDGE_CURVE('',#7545,#7543,#4965,.T.);
#9595=EDGE_CURVE('',#7546,#7547,#5598,.T.);
#9596=EDGE_CURVE('',#7546,#7544,#4966,.T.);
#9597=EDGE_CURVE('',#7547,#7545,#4967,.T.);
#9598=EDGE_CURVE('',#7548,#7549,#5599,.T.);
#9599=EDGE_CURVE('',#7548,#7546,#4968,.T.);
#9600=EDGE_CURVE('',#7549,#7547,#4969,.T.);
#9601=EDGE_CURVE('',#7550,#7551,#5600,.T.);
#9602=EDGE_CURVE('',#7550,#7548,#4970,.T.);
#9603=EDGE_CURVE('',#7551,#7549,#4971,.T.);
#9604=EDGE_CURVE('',#7552,#7553,#5601,.T.);
#9605=EDGE_CURVE('',#7552,#7550,#4972,.T.);
#9606=EDGE_CURVE('',#7553,#7551,#4973,.T.);
#9607=EDGE_CURVE('',#7554,#7555,#5602,.T.);
#9608=EDGE_CURVE('',#7554,#7552,#4974,.T.);
#9609=EDGE_CURVE('',#7555,#7553,#4975,.T.);
#9610=EDGE_CURVE('',#7556,#7557,#5603,.T.);
#9611=EDGE_CURVE('',#7556,#7554,#4976,.T.);
#9612=EDGE_CURVE('',#7557,#7555,#4977,.T.);
#9613=EDGE_CURVE('',#7558,#7559,#5604,.T.);
#9614=EDGE_CURVE('',#7558,#7556,#4978,.T.);
#9615=EDGE_CURVE('',#7559,#7557,#4979,.T.);
#9616=EDGE_CURVE('',#7560,#7561,#5605,.T.);
#9617=EDGE_CURVE('',#7560,#7558,#4980,.T.);
#9618=EDGE_CURVE('',#7561,#7559,#4981,.T.);
#9619=EDGE_CURVE('',#7236,#7240,#5606,.T.);
#9620=EDGE_CURVE('',#7241,#7235,#5607,.T.);
#9621=EDGE_CURVE('',#7232,#7238,#5608,.T.);
#9622=EDGE_CURVE('',#7239,#7231,#5609,.T.);
#9623=EDGE_CURVE('',#7436,#7562,#4982,.T.);
#9624=EDGE_CURVE('',#7563,#7562,#3557,.F.);
#9625=EDGE_CURVE('',#7564,#7563,#3558,.F.);
#9626=EDGE_CURVE('',#7564,#7439,#4983,.T.);
#9627=EDGE_CURVE('',#7363,#7564,#4984,.T.);
#9628=EDGE_CURVE('',#7565,#7237,#4985,.T.);
#9629=EDGE_CURVE('',#7565,#7561,#4986,.T.);
#9630=EDGE_CURVE('',#7228,#7566,#4987,.T.);
#9631=EDGE_CURVE('',#7566,#7565,#3559,.T.);
#9632=EDGE_CURVE('',#7566,#7560,#4988,.T.);
#9633=EDGE_CURVE('',#7562,#7362,#4989,.T.);
#9634=EDGE_CURVE('',#7402,#7567,#4990,.T.);
#9635=EDGE_CURVE('',#7568,#7567,#3560,.T.);
#9636=EDGE_CURVE('',#7569,#7568,#3561,.T.);
#9637=EDGE_CURVE('',#7569,#7403,#4991,.T.);
#9638=EDGE_CURVE('',#7399,#7569,#4992,.T.);
#9639=EDGE_CURVE('',#7570,#7369,#4993,.T.);
#9640=EDGE_CURVE('',#7570,#7433,#4994,.T.);
#9641=EDGE_CURVE('',#7366,#7571,#4995,.T.);
#9642=EDGE_CURVE('',#7571,#7570,#3562,.T.);
#9643=EDGE_CURVE('',#7571,#7432,#4996,.T.);
#9644=EDGE_CURVE('',#7567,#7398,#4997,.T.);
#9645=EDGE_CURVE('',#7567,#7569,#3563,.T.);
#9646=EDGE_CURVE('',#7572,#7573,#3564,.T.);
#9647=EDGE_CURVE('',#7574,#7573,#608,.T.);
#9648=EDGE_CURVE('',#7575,#7574,#3565,.T.);
#9649=EDGE_CURVE('',#7572,#7575,#609,.T.);
#9650=EDGE_CURVE('',#7572,#7576,#4998,.T.);
#9651=EDGE_CURVE('',#7575,#7577,#5610,.T.);
#9652=EDGE_CURVE('',#7577,#7578,#610,.T.);
#9653=EDGE_CURVE('',#7579,#7578,#4999,.T.);
#9654=EDGE_CURVE('',#7576,#7579,#5000,.T.);
#9655=EDGE_CURVE('',#7574,#7580,#5611,.T.);
#9656=EDGE_CURVE('',#7580,#7577,#3566,.T.);
#9657=EDGE_CURVE('',#7581,#7573,#5001,.T.);
#9658=EDGE_CURVE('',#7582,#7581,#5002,.T.);
#9659=EDGE_CURVE('',#7583,#7582,#5003,.T.);
#9660=EDGE_CURVE('',#7583,#7580,#611,.T.);
#9661=EDGE_CURVE('',#7578,#7583,#3567,.T.);
#9662=EDGE_CURVE('',#7584,#7576,#3568,.T.);
#9663=EDGE_CURVE('',#7584,#7585,#5004,.T.);
#9664=EDGE_CURVE('',#7585,#7572,#3569,.T.);
#9665=EDGE_CURVE('',#7573,#7586,#3570,.T.);
#9666=EDGE_CURVE('',#7586,#7587,#5005,.T.);
#9667=EDGE_CURVE('',#7581,#7587,#3571,.T.);
#9668=EDGE_CURVE('',#7588,#7579,#3572,.T.);
#9669=EDGE_CURVE('',#7588,#7584,#5006,.T.);
#9670=EDGE_CURVE('',#7589,#7578,#3573,.T.);
#9671=EDGE_CURVE('',#7589,#7588,#5007,.T.);
#9672=EDGE_CURVE('',#7590,#7585,#3574,.T.);
#9673=EDGE_CURVE('',#7591,#7585,#612,.T.);
#9674=EDGE_CURVE('',#7592,#7591,#3575,.T.);
#9675=EDGE_CURVE('',#7590,#7592,#613,.T.);
#9676=EDGE_CURVE('',#7590,#7593,#5008,.T.);
#9677=EDGE_CURVE('',#7592,#7594,#5612,.T.);
#9678=EDGE_CURVE('',#7594,#7595,#614,.T.);
#9679=EDGE_CURVE('',#7596,#7595,#5009,.T.);
#9680=EDGE_CURVE('',#7593,#7596,#5010,.T.);
#9681=EDGE_CURVE('',#7591,#7597,#5613,.T.);
#9682=EDGE_CURVE('',#7597,#7594,#3576,.T.);
#9683=EDGE_CURVE('',#7589,#7597,#615,.T.);
#9684=EDGE_CURVE('',#7595,#7589,#3577,.T.);
#9685=EDGE_CURVE('',#7598,#7593,#3578,.T.);
#9686=EDGE_CURVE('',#7598,#7599,#5011,.T.);
#9687=EDGE_CURVE('',#7599,#7590,#3579,.T.);
#9688=EDGE_CURVE('',#7600,#7596,#3580,.T.);
#9689=EDGE_CURVE('',#7600,#7598,#5012,.T.);
#9690=EDGE_CURVE('',#7601,#7595,#3581,.T.);
#9691=EDGE_CURVE('',#7601,#7600,#5013,.T.);
#9692=EDGE_CURVE('',#7602,#7599,#3582,.T.);
#9693=EDGE_CURVE('',#7603,#7599,#616,.T.);
#9694=EDGE_CURVE('',#7604,#7603,#3583,.T.);
#9695=EDGE_CURVE('',#7602,#7604,#617,.T.);
#9696=EDGE_CURVE('',#7602,#7605,#5014,.T.);
#9697=EDGE_CURVE('',#7604,#7606,#5614,.T.);
#9698=EDGE_CURVE('',#7606,#7607,#618,.T.);
#9699=EDGE_CURVE('',#7608,#7607,#5015,.T.);
#9700=EDGE_CURVE('',#7605,#7608,#5016,.T.);
#9701=EDGE_CURVE('',#7603,#7609,#5615,.T.);
#9702=EDGE_CURVE('',#7609,#7606,#3584,.T.);
#9703=EDGE_CURVE('',#7601,#7609,#619,.T.);
#9704=EDGE_CURVE('',#7607,#7601,#3585,.T.);
#9705=EDGE_CURVE('',#7610,#7605,#3586,.T.);
#9706=EDGE_CURVE('',#7610,#7611,#5017,.T.);
#9707=EDGE_CURVE('',#7611,#7602,#3587,.T.);
#9708=EDGE_CURVE('',#7612,#7608,#3588,.T.);
#9709=EDGE_CURVE('',#7612,#7610,#5018,.T.);
#9710=EDGE_CURVE('',#7613,#7607,#3589,.T.);
#9711=EDGE_CURVE('',#7613,#7612,#5019,.T.);
#9712=EDGE_CURVE('',#7614,#7611,#3590,.T.);
#9713=EDGE_CURVE('',#7615,#7611,#620,.T.);
#9714=EDGE_CURVE('',#7616,#7615,#3591,.T.);
#9715=EDGE_CURVE('',#7614,#7616,#621,.T.);
#9716=EDGE_CURVE('',#7614,#7617,#5020,.T.);
#9717=EDGE_CURVE('',#7616,#7618,#5616,.T.);
#9718=EDGE_CURVE('',#7618,#7619,#622,.T.);
#9719=EDGE_CURVE('',#7620,#7619,#5021,.T.);
#9720=EDGE_CURVE('',#7617,#7620,#5022,.T.);
#9721=EDGE_CURVE('',#7615,#7621,#5617,.T.);
#9722=EDGE_CURVE('',#7621,#7618,#3592,.T.);
#9723=EDGE_CURVE('',#7613,#7621,#623,.T.);
#9724=EDGE_CURVE('',#7619,#7613,#3593,.T.);
#9725=EDGE_CURVE('',#7622,#7617,#3594,.T.);
#9726=EDGE_CURVE('',#7622,#7623,#5023,.T.);
#9727=EDGE_CURVE('',#7623,#7614,#3595,.T.);
#9728=EDGE_CURVE('',#7624,#7620,#3596,.T.);
#9729=EDGE_CURVE('',#7624,#7622,#5024,.T.);
#9730=EDGE_CURVE('',#7625,#7619,#3597,.T.);
#9731=EDGE_CURVE('',#7625,#7624,#5025,.T.);
#9732=EDGE_CURVE('',#7626,#7623,#3598,.T.);
#9733=EDGE_CURVE('',#7627,#7623,#624,.T.);
#9734=EDGE_CURVE('',#7628,#7627,#3599,.T.);
#9735=EDGE_CURVE('',#7626,#7628,#625,.T.);
#9736=EDGE_CURVE('',#7626,#7629,#5026,.T.);
#9737=EDGE_CURVE('',#7628,#7630,#5618,.T.);
#9738=EDGE_CURVE('',#7630,#7631,#626,.T.);
#9739=EDGE_CURVE('',#7632,#7631,#5027,.T.);
#9740=EDGE_CURVE('',#7629,#7632,#5028,.T.);
#9741=EDGE_CURVE('',#7627,#7633,#5619,.T.);
#9742=EDGE_CURVE('',#7633,#7630,#3600,.T.);
#9743=EDGE_CURVE('',#7625,#7633,#627,.T.);
#9744=EDGE_CURVE('',#7631,#7625,#3601,.T.);
#9745=EDGE_CURVE('',#7634,#7629,#3602,.T.);
#9746=EDGE_CURVE('',#7634,#7635,#5029,.T.);
#9747=EDGE_CURVE('',#7635,#7626,#3603,.T.);
#9748=EDGE_CURVE('',#7636,#7632,#3604,.T.);
#9749=EDGE_CURVE('',#7636,#7634,#5030,.T.);
#9750=EDGE_CURVE('',#7637,#7631,#3605,.T.);
#9751=EDGE_CURVE('',#7637,#7636,#5031,.T.);
#9752=EDGE_CURVE('',#7638,#7635,#3606,.T.);
#9753=EDGE_CURVE('',#7639,#7635,#628,.T.);
#9754=EDGE_CURVE('',#7640,#7639,#3607,.T.);
#9755=EDGE_CURVE('',#7638,#7640,#629,.T.);
#9756=EDGE_CURVE('',#7638,#7641,#5032,.T.);
#9757=EDGE_CURVE('',#7640,#7642,#5620,.T.);
#9758=EDGE_CURVE('',#7642,#7643,#630,.T.);
#9759=EDGE_CURVE('',#7644,#7643,#5033,.T.);
#9760=EDGE_CURVE('',#7641,#7644,#5034,.T.);
#9761=EDGE_CURVE('',#7639,#7645,#5621,.T.);
#9762=EDGE_CURVE('',#7645,#7642,#3608,.T.);
#9763=EDGE_CURVE('',#7637,#7645,#631,.T.);
#9764=EDGE_CURVE('',#7643,#7637,#3609,.T.);
#9765=EDGE_CURVE('',#7646,#7641,#3610,.T.);
#9766=EDGE_CURVE('',#7646,#7647,#5035,.T.);
#9767=EDGE_CURVE('',#7647,#7638,#3611,.T.);
#9768=EDGE_CURVE('',#7648,#7644,#3612,.T.);
#9769=EDGE_CURVE('',#7648,#7646,#5036,.T.);
#9770=EDGE_CURVE('',#7649,#7643,#3613,.T.);
#9771=EDGE_CURVE('',#7649,#7648,#5037,.T.);
#9772=EDGE_CURVE('',#7650,#7647,#3614,.T.);
#9773=EDGE_CURVE('',#7651,#7647,#632,.T.);
#9774=EDGE_CURVE('',#7652,#7651,#3615,.T.);
#9775=EDGE_CURVE('',#7650,#7652,#633,.T.);
#9776=EDGE_CURVE('',#7650,#7653,#5038,.T.);
#9777=EDGE_CURVE('',#7652,#7654,#5622,.T.);
#9778=EDGE_CURVE('',#7654,#7655,#634,.T.);
#9779=EDGE_CURVE('',#7656,#7655,#5039,.T.);
#9780=EDGE_CURVE('',#7653,#7656,#5040,.T.);
#9781=EDGE_CURVE('',#7651,#7657,#5623,.T.);
#9782=EDGE_CURVE('',#7657,#7654,#3616,.T.);
#9783=EDGE_CURVE('',#7649,#7657,#635,.T.);
#9784=EDGE_CURVE('',#7655,#7649,#3617,.T.);
#9785=EDGE_CURVE('',#7658,#7653,#3618,.T.);
#9786=EDGE_CURVE('',#7658,#7659,#5041,.T.);
#9787=EDGE_CURVE('',#7659,#7650,#3619,.T.);
#9788=EDGE_CURVE('',#7660,#7656,#3620,.T.);
#9789=EDGE_CURVE('',#7660,#7658,#5042,.T.);
#9790=EDGE_CURVE('',#7661,#7655,#3621,.T.);
#9791=EDGE_CURVE('',#7661,#7660,#5043,.T.);
#9792=EDGE_CURVE('',#7662,#7663,#3622,.T.);
#9793=EDGE_CURVE('',#7663,#7659,#3623,.T.);
#9794=EDGE_CURVE('',#7664,#7659,#636,.T.);
#9795=EDGE_CURVE('',#7665,#7664,#3624,.T.);
#9796=EDGE_CURVE('',#7662,#7665,#637,.T.);
#9797=EDGE_CURVE('',#7662,#7666,#5044,.T.);
#9798=EDGE_CURVE('',#7665,#7667,#5624,.T.);
#9799=EDGE_CURVE('',#7667,#7668,#638,.T.);
#9800=EDGE_CURVE('',#7669,#7668,#5045,.T.);
#9801=EDGE_CURVE('',#7666,#7669,#5046,.T.);
#9802=EDGE_CURVE('',#7664,#7670,#5625,.T.);
#9803=EDGE_CURVE('',#7670,#7667,#3625,.T.);
#9804=EDGE_CURVE('',#7661,#7670,#639,.T.);
#9805=EDGE_CURVE('',#7668,#7671,#3626,.T.);
#9806=EDGE_CURVE('',#7671,#7661,#3627,.T.);
#9807=EDGE_CURVE('',#7672,#7666,#3628,.T.);
#9808=EDGE_CURVE('',#7672,#7673,#5047,.T.);
#9809=EDGE_CURVE('',#7673,#7662,#3629,.T.);
#9810=EDGE_CURVE('',#7674,#7669,#3630,.T.);
#9811=EDGE_CURVE('',#7674,#7672,#5048,.T.);
#9812=EDGE_CURVE('',#7675,#7668,#3631,.T.);
#9813=EDGE_CURVE('',#7675,#7674,#5049,.T.);
#9814=EDGE_CURVE('',#7676,#7673,#3632,.T.);
#9815=EDGE_CURVE('',#7677,#7673,#640,.T.);
#9816=EDGE_CURVE('',#7678,#7677,#3633,.T.);
#9817=EDGE_CURVE('',#7676,#7678,#641,.T.);
#9818=EDGE_CURVE('',#7676,#7679,#5050,.T.);
#9819=EDGE_CURVE('',#7678,#7680,#5626,.T.);
#9820=EDGE_CURVE('',#7680,#7681,#642,.T.);
#9821=EDGE_CURVE('',#7682,#7681,#5051,.T.);
#9822=EDGE_CURVE('',#7679,#7682,#5052,.T.);
#9823=EDGE_CURVE('',#7677,#7683,#5627,.T.);
#9824=EDGE_CURVE('',#7683,#7680,#3634,.T.);
#9825=EDGE_CURVE('',#7675,#7683,#643,.T.);
#9826=EDGE_CURVE('',#7681,#7675,#3635,.T.);
#9827=EDGE_CURVE('',#7684,#7679,#3636,.T.);
#9828=EDGE_CURVE('',#7684,#7685,#5053,.T.);
#9829=EDGE_CURVE('',#7685,#7676,#3637,.T.);
#9830=EDGE_CURVE('',#7686,#7682,#3638,.T.);
#9831=EDGE_CURVE('',#7686,#7684,#5054,.T.);
#9832=EDGE_CURVE('',#7687,#7681,#3639,.T.);
#9833=EDGE_CURVE('',#7687,#7686,#5055,.T.);
#9834=EDGE_CURVE('',#7688,#7685,#3640,.T.);
#9835=EDGE_CURVE('',#7689,#7685,#644,.T.);
#9836=EDGE_CURVE('',#7690,#7689,#3641,.T.);
#9837=EDGE_CURVE('',#7688,#7690,#645,.T.);
#9838=EDGE_CURVE('',#7688,#7691,#5056,.T.);
#9839=EDGE_CURVE('',#7690,#7692,#5628,.T.);
#9840=EDGE_CURVE('',#7692,#7693,#646,.T.);
#9841=EDGE_CURVE('',#7694,#7693,#5057,.T.);
#9842=EDGE_CURVE('',#7691,#7694,#5058,.T.);
#9843=EDGE_CURVE('',#7689,#7695,#5629,.T.);
#9844=EDGE_CURVE('',#7695,#7692,#3642,.T.);
#9845=EDGE_CURVE('',#7687,#7695,#647,.T.);
#9846=EDGE_CURVE('',#7693,#7687,#3643,.T.);
#9847=EDGE_CURVE('',#7696,#7691,#3644,.T.);
#9848=EDGE_CURVE('',#7696,#7697,#5059,.T.);
#9849=EDGE_CURVE('',#7697,#7688,#3645,.T.);
#9850=EDGE_CURVE('',#7698,#7694,#3646,.T.);
#9851=EDGE_CURVE('',#7698,#7696,#5060,.T.);
#9852=EDGE_CURVE('',#7699,#7693,#3647,.T.);
#9853=EDGE_CURVE('',#7699,#7698,#5061,.T.);
#9854=EDGE_CURVE('',#7700,#7697,#3648,.T.);
#9855=EDGE_CURVE('',#7701,#7697,#648,.T.);
#9856=EDGE_CURVE('',#7702,#7701,#3649,.T.);
#9857=EDGE_CURVE('',#7700,#7702,#649,.T.);
#9858=EDGE_CURVE('',#7700,#7703,#5062,.T.);
#9859=EDGE_CURVE('',#7702,#7704,#5630,.T.);
#9860=EDGE_CURVE('',#7704,#7705,#650,.T.);
#9861=EDGE_CURVE('',#7706,#7705,#5063,.T.);
#9862=EDGE_CURVE('',#7703,#7706,#5064,.T.);
#9863=EDGE_CURVE('',#7701,#7707,#5631,.T.);
#9864=EDGE_CURVE('',#7707,#7704,#3650,.T.);
#9865=EDGE_CURVE('',#7699,#7707,#651,.T.);
#9866=EDGE_CURVE('',#7705,#7699,#3651,.T.);
#9867=EDGE_CURVE('',#7708,#7703,#3652,.T.);
#9868=EDGE_CURVE('',#7708,#7709,#5065,.T.);
#9869=EDGE_CURVE('',#7709,#7700,#3653,.T.);
#9870=EDGE_CURVE('',#7710,#7706,#3654,.T.);
#9871=EDGE_CURVE('',#7710,#7708,#5066,.T.);
#9872=EDGE_CURVE('',#7711,#7705,#3655,.T.);
#9873=EDGE_CURVE('',#7711,#7710,#5067,.T.);
#9874=EDGE_CURVE('',#7712,#7709,#3656,.T.);
#9875=EDGE_CURVE('',#7713,#7709,#652,.T.);
#9876=EDGE_CURVE('',#7714,#7713,#3657,.T.);
#9877=EDGE_CURVE('',#7712,#7714,#653,.T.);
#9878=EDGE_CURVE('',#7712,#7715,#5068,.T.);
#9879=EDGE_CURVE('',#7714,#7716,#5632,.T.);
#9880=EDGE_CURVE('',#7716,#7717,#654,.T.);
#9881=EDGE_CURVE('',#7718,#7717,#5069,.T.);
#9882=EDGE_CURVE('',#7715,#7718,#5070,.T.);
#9883=EDGE_CURVE('',#7713,#7719,#5633,.T.);
#9884=EDGE_CURVE('',#7719,#7716,#3658,.T.);
#9885=EDGE_CURVE('',#7711,#7719,#655,.T.);
#9886=EDGE_CURVE('',#7717,#7711,#3659,.T.);
#9887=EDGE_CURVE('',#7720,#7715,#3660,.T.);
#9888=EDGE_CURVE('',#7720,#7721,#5071,.T.);
#9889=EDGE_CURVE('',#7721,#7712,#3661,.T.);
#9890=EDGE_CURVE('',#7722,#7718,#3662,.T.);
#9891=EDGE_CURVE('',#7722,#7720,#5072,.T.);
#9892=EDGE_CURVE('',#7723,#7717,#3663,.T.);
#9893=EDGE_CURVE('',#7723,#7722,#5073,.T.);
#9894=EDGE_CURVE('',#7724,#7721,#3664,.T.);
#9895=EDGE_CURVE('',#7725,#7721,#656,.T.);
#9896=EDGE_CURVE('',#7726,#7725,#3665,.T.);
#9897=EDGE_CURVE('',#7724,#7726,#657,.T.);
#9898=EDGE_CURVE('',#7724,#7727,#5074,.T.);
#9899=EDGE_CURVE('',#7726,#7728,#5634,.T.);
#9900=EDGE_CURVE('',#7728,#7729,#658,.T.);
#9901=EDGE_CURVE('',#7730,#7729,#5075,.T.);
#9902=EDGE_CURVE('',#7727,#7730,#5076,.T.);
#9903=EDGE_CURVE('',#7725,#7731,#5635,.T.);
#9904=EDGE_CURVE('',#7731,#7728,#3666,.T.);
#9905=EDGE_CURVE('',#7723,#7731,#659,.T.);
#9906=EDGE_CURVE('',#7729,#7723,#3667,.T.);
#9907=EDGE_CURVE('',#7732,#7727,#3668,.T.);
#9908=EDGE_CURVE('',#7732,#7733,#5077,.T.);
#9909=EDGE_CURVE('',#7733,#7724,#3669,.T.);
#9910=EDGE_CURVE('',#7734,#7730,#3670,.T.);
#9911=EDGE_CURVE('',#7734,#7732,#5078,.T.);
#9912=EDGE_CURVE('',#7735,#7729,#3671,.T.);
#9913=EDGE_CURVE('',#7735,#7734,#5079,.T.);
#9914=EDGE_CURVE('',#7736,#7733,#3672,.T.);
#9915=EDGE_CURVE('',#7737,#7733,#660,.T.);
#9916=EDGE_CURVE('',#7738,#7737,#3673,.T.);
#9917=EDGE_CURVE('',#7736,#7738,#661,.T.);
#9918=EDGE_CURVE('',#7736,#7739,#5080,.T.);
#9919=EDGE_CURVE('',#7738,#7740,#5636,.T.);
#9920=EDGE_CURVE('',#7740,#7741,#662,.T.);
#9921=EDGE_CURVE('',#7742,#7741,#5081,.T.);
#9922=EDGE_CURVE('',#7739,#7742,#5082,.T.);
#9923=EDGE_CURVE('',#7737,#7743,#5637,.T.);
#9924=EDGE_CURVE('',#7743,#7740,#3674,.T.);
#9925=EDGE_CURVE('',#7735,#7743,#663,.T.);
#9926=EDGE_CURVE('',#7741,#7735,#3675,.T.);
#9927=EDGE_CURVE('',#7744,#7739,#3676,.T.);
#9928=EDGE_CURVE('',#7744,#7745,#5083,.T.);
#9929=EDGE_CURVE('',#7745,#7736,#3677,.T.);
#9930=EDGE_CURVE('',#7746,#7742,#3678,.T.);
#9931=EDGE_CURVE('',#7746,#7744,#5084,.T.);
#9932=EDGE_CURVE('',#7747,#7741,#3679,.T.);
#9933=EDGE_CURVE('',#7747,#7746,#5085,.T.);
#9934=EDGE_CURVE('',#7747,#7748,#664,.T.);
#9935=EDGE_CURVE('',#7749,#7748,#5638,.T.);
#9936=EDGE_CURVE('',#7749,#7745,#665,.T.);
#9937=EDGE_CURVE('',#7586,#7745,#3680,.T.);
#9938=EDGE_CURVE('',#7750,#7749,#3681,.T.);
#9939=EDGE_CURVE('',#7586,#7750,#666,.T.);
#9940=EDGE_CURVE('',#7748,#7751,#3682,.T.);
#9941=EDGE_CURVE('',#7750,#7751,#5639,.T.);
#9942=EDGE_CURVE('',#7752,#7753,#5086,.T.);
#9943=EDGE_CURVE('',#7587,#7752,#5087,.T.);
#9944=EDGE_CURVE('',#7751,#7753,#667,.T.);
#9945=EDGE_CURVE('',#7753,#7747,#3683,.T.);
#9946=EDGE_CURVE('',#7582,#7752,#3684,.T.);
#9947=EDGE_CURVE('',#7583,#7753,#3685,.T.);
#9948=EDGE_CURVE('',#7754,#7754,#3686,.T.);
#9949=EDGE_CURVE('',#7368,#7754,#5640,.T.);
#9950=EDGE_CURVE('',#7663,#7568,#5641,.T.);
#9951=EDGE_CURVE('',#7234,#7671,#5642,.T.);
#9952=EDGE_CURVE('',#7562,#7564,#3687,.F.);
#9953=EDGE_CURVE('',#7755,#7755,#3688,.T.);
#9954=EDGE_CURVE('',#7755,#7563,#5643,.T.);
#12188=ORIENTED_EDGE('',*,*,#9127,.F.);
#12189=ORIENTED_EDGE('',*,*,#9128,.T.);
#12190=ORIENTED_EDGE('',*,*,#9129,.T.);
#12191=ORIENTED_EDGE('',*,*,#9130,.T.);
#12192=ORIENTED_EDGE('',*,*,#9131,.T.);
#12193=ORIENTED_EDGE('',*,*,#9132,.T.);
#12194=ORIENTED_EDGE('',*,*,#9133,.T.);
#12195=ORIENTED_EDGE('',*,*,#9134,.T.);
#12196=ORIENTED_EDGE('',*,*,#9135,.T.);
#12197=ORIENTED_EDGE('',*,*,#9134,.F.);
#12198=ORIENTED_EDGE('',*,*,#9136,.T.);
#12199=ORIENTED_EDGE('',*,*,#9137,.T.);
#12200=ORIENTED_EDGE('',*,*,#9138,.T.);
#12201=ORIENTED_EDGE('',*,*,#9130,.F.);
#12202=ORIENTED_EDGE('',*,*,#9139,.T.);
#12203=ORIENTED_EDGE('',*,*,#9140,.T.);
#12204=ORIENTED_EDGE('',*,*,#9141,.T.);
#12205=ORIENTED_EDGE('',*,*,#9142,.T.);
#12206=ORIENTED_EDGE('',*,*,#9143,.T.);
#12207=ORIENTED_EDGE('',*,*,#9144,.T.);
#12208=ORIENTED_EDGE('',*,*,#9145,.F.);
#12209=ORIENTED_EDGE('',*,*,#9146,.T.);
#12210=ORIENTED_EDGE('',*,*,#9127,.T.);
#12211=ORIENTED_EDGE('',*,*,#9147,.T.);
#12212=ORIENTED_EDGE('',*,*,#9148,.F.);
#12213=ORIENTED_EDGE('',*,*,#9149,.T.);
#12214=ORIENTED_EDGE('',*,*,#9145,.T.);
#12215=ORIENTED_EDGE('',*,*,#9150,.T.);
#12216=ORIENTED_EDGE('',*,*,#9151,.F.);
#12217=ORIENTED_EDGE('',*,*,#9152,.T.);
#12218=ORIENTED_EDGE('',*,*,#9148,.T.);
#12219=ORIENTED_EDGE('',*,*,#9153,.T.);
#12220=ORIENTED_EDGE('',*,*,#9154,.F.);
#12221=ORIENTED_EDGE('',*,*,#9155,.T.);
#12222=ORIENTED_EDGE('',*,*,#9151,.T.);
#12223=ORIENTED_EDGE('',*,*,#9156,.T.);
#12224=ORIENTED_EDGE('',*,*,#9157,.F.);
#12225=ORIENTED_EDGE('',*,*,#9158,.T.);
#12226=ORIENTED_EDGE('',*,*,#9154,.T.);
#12227=ORIENTED_EDGE('',*,*,#9159,.T.);
#12228=ORIENTED_EDGE('',*,*,#9160,.F.);
#12229=ORIENTED_EDGE('',*,*,#9161,.T.);
#12230=ORIENTED_EDGE('',*,*,#9157,.T.);
#12231=ORIENTED_EDGE('',*,*,#9162,.T.);
#12232=ORIENTED_EDGE('',*,*,#9163,.F.);
#12233=ORIENTED_EDGE('',*,*,#9164,.T.);
#12234=ORIENTED_EDGE('',*,*,#9160,.T.);
#12235=ORIENTED_EDGE('',*,*,#9165,.T.);
#12236=ORIENTED_EDGE('',*,*,#9166,.F.);
#12237=ORIENTED_EDGE('',*,*,#9167,.T.);
#12238=ORIENTED_EDGE('',*,*,#9163,.T.);
#12239=ORIENTED_EDGE('',*,*,#9168,.T.);
#12240=ORIENTED_EDGE('',*,*,#9169,.F.);
#12241=ORIENTED_EDGE('',*,*,#9170,.T.);
#12242=ORIENTED_EDGE('',*,*,#9166,.T.);
#12243=ORIENTED_EDGE('',*,*,#9171,.T.);
#12244=ORIENTED_EDGE('',*,*,#9172,.F.);
#12245=ORIENTED_EDGE('',*,*,#9173,.T.);
#12246=ORIENTED_EDGE('',*,*,#9169,.T.);
#12247=ORIENTED_EDGE('',*,*,#9174,.T.);
#12248=ORIENTED_EDGE('',*,*,#9175,.F.);
#12249=ORIENTED_EDGE('',*,*,#9176,.T.);
#12250=ORIENTED_EDGE('',*,*,#9172,.T.);
#12251=ORIENTED_EDGE('',*,*,#9177,.T.);
#12252=ORIENTED_EDGE('',*,*,#9178,.F.);
#12253=ORIENTED_EDGE('',*,*,#9179,.T.);
#12254=ORIENTED_EDGE('',*,*,#9175,.T.);
#12255=ORIENTED_EDGE('',*,*,#9180,.T.);
#12256=ORIENTED_EDGE('',*,*,#9181,.F.);
#12257=ORIENTED_EDGE('',*,*,#9182,.T.);
#12258=ORIENTED_EDGE('',*,*,#9178,.T.);
#12259=ORIENTED_EDGE('',*,*,#9183,.T.);
#12260=ORIENTED_EDGE('',*,*,#9184,.F.);
#12261=ORIENTED_EDGE('',*,*,#9185,.T.);
#12262=ORIENTED_EDGE('',*,*,#9181,.T.);
#12263=ORIENTED_EDGE('',*,*,#9186,.T.);
#12264=ORIENTED_EDGE('',*,*,#9187,.F.);
#12265=ORIENTED_EDGE('',*,*,#9188,.T.);
#12266=ORIENTED_EDGE('',*,*,#9184,.T.);
#12267=ORIENTED_EDGE('',*,*,#9189,.T.);
#12268=ORIENTED_EDGE('',*,*,#9190,.F.);
#12269=ORIENTED_EDGE('',*,*,#9191,.T.);
#12270=ORIENTED_EDGE('',*,*,#9187,.T.);
#12271=ORIENTED_EDGE('',*,*,#9192,.T.);
#12272=ORIENTED_EDGE('',*,*,#9193,.F.);
#12273=ORIENTED_EDGE('',*,*,#9194,.T.);
#12274=ORIENTED_EDGE('',*,*,#9190,.T.);
#12275=ORIENTED_EDGE('',*,*,#9195,.T.);
#12276=ORIENTED_EDGE('',*,*,#9196,.F.);
#12277=ORIENTED_EDGE('',*,*,#9197,.T.);
#12278=ORIENTED_EDGE('',*,*,#9193,.T.);
#12279=ORIENTED_EDGE('',*,*,#9198,.T.);
#12280=ORIENTED_EDGE('',*,*,#9199,.F.);
#12281=ORIENTED_EDGE('',*,*,#9200,.T.);
#12282=ORIENTED_EDGE('',*,*,#9196,.T.);
#12283=ORIENTED_EDGE('',*,*,#9201,.T.);
#12284=ORIENTED_EDGE('',*,*,#9202,.F.);
#12285=ORIENTED_EDGE('',*,*,#9203,.T.);
#12286=ORIENTED_EDGE('',*,*,#9199,.T.);
#12287=ORIENTED_EDGE('',*,*,#9204,.T.);
#12288=ORIENTED_EDGE('',*,*,#9205,.F.);
#12289=ORIENTED_EDGE('',*,*,#9206,.T.);
#12290=ORIENTED_EDGE('',*,*,#9202,.T.);
#12291=ORIENTED_EDGE('',*,*,#9207,.T.);
#12292=ORIENTED_EDGE('',*,*,#9208,.F.);
#12293=ORIENTED_EDGE('',*,*,#9209,.T.);
#12294=ORIENTED_EDGE('',*,*,#9205,.T.);
#12295=ORIENTED_EDGE('',*,*,#9210,.T.);
#12296=ORIENTED_EDGE('',*,*,#9211,.F.);
#12297=ORIENTED_EDGE('',*,*,#9212,.T.);
#12298=ORIENTED_EDGE('',*,*,#9208,.T.);
#12299=ORIENTED_EDGE('',*,*,#9213,.T.);
#12300=ORIENTED_EDGE('',*,*,#9214,.F.);
#12301=ORIENTED_EDGE('',*,*,#9215,.T.);
#12302=ORIENTED_EDGE('',*,*,#9211,.T.);
#12303=ORIENTED_EDGE('',*,*,#9216,.T.);
#12304=ORIENTED_EDGE('',*,*,#9217,.F.);
#12305=ORIENTED_EDGE('',*,*,#9218,.T.);
#12306=ORIENTED_EDGE('',*,*,#9214,.T.);
#12307=ORIENTED_EDGE('',*,*,#9219,.T.);
#12308=ORIENTED_EDGE('',*,*,#9220,.F.);
#12309=ORIENTED_EDGE('',*,*,#9221,.T.);
#12310=ORIENTED_EDGE('',*,*,#9217,.T.);
#12311=ORIENTED_EDGE('',*,*,#9222,.T.);
#12312=ORIENTED_EDGE('',*,*,#9223,.F.);
#12313=ORIENTED_EDGE('',*,*,#9224,.T.);
#12314=ORIENTED_EDGE('',*,*,#9220,.T.);
#12315=ORIENTED_EDGE('',*,*,#9225,.T.);
#12316=ORIENTED_EDGE('',*,*,#9226,.F.);
#12317=ORIENTED_EDGE('',*,*,#9227,.T.);
#12318=ORIENTED_EDGE('',*,*,#9223,.T.);
#12319=ORIENTED_EDGE('',*,*,#9228,.T.);
#12320=ORIENTED_EDGE('',*,*,#9229,.F.);
#12321=ORIENTED_EDGE('',*,*,#9230,.T.);
#12322=ORIENTED_EDGE('',*,*,#9226,.T.);
#12323=ORIENTED_EDGE('',*,*,#9231,.T.);
#12324=ORIENTED_EDGE('',*,*,#9232,.F.);
#12325=ORIENTED_EDGE('',*,*,#9233,.T.);
#12326=ORIENTED_EDGE('',*,*,#9229,.T.);
#12327=ORIENTED_EDGE('',*,*,#9234,.T.);
#12328=ORIENTED_EDGE('',*,*,#9235,.F.);
#12329=ORIENTED_EDGE('',*,*,#9236,.T.);
#12330=ORIENTED_EDGE('',*,*,#9232,.T.);
#12331=ORIENTED_EDGE('',*,*,#9237,.T.);
#12332=ORIENTED_EDGE('',*,*,#9238,.F.);
#12333=ORIENTED_EDGE('',*,*,#9239,.T.);
#12334=ORIENTED_EDGE('',*,*,#9235,.T.);
#12335=ORIENTED_EDGE('',*,*,#9240,.T.);
#12336=ORIENTED_EDGE('',*,*,#9241,.F.);
#12337=ORIENTED_EDGE('',*,*,#9242,.T.);
#12338=ORIENTED_EDGE('',*,*,#9238,.T.);
#12339=ORIENTED_EDGE('',*,*,#9243,.T.);
#12340=ORIENTED_EDGE('',*,*,#9244,.F.);
#12341=ORIENTED_EDGE('',*,*,#9245,.T.);
#12342=ORIENTED_EDGE('',*,*,#9241,.T.);
#12343=ORIENTED_EDGE('',*,*,#9246,.T.);
#12344=ORIENTED_EDGE('',*,*,#9247,.F.);
#12345=ORIENTED_EDGE('',*,*,#9248,.T.);
#12346=ORIENTED_EDGE('',*,*,#9244,.T.);
#12347=ORIENTED_EDGE('',*,*,#9249,.T.);
#12348=ORIENTED_EDGE('',*,*,#9250,.F.);
#12349=ORIENTED_EDGE('',*,*,#9251,.T.);
#12350=ORIENTED_EDGE('',*,*,#9247,.T.);
#12351=ORIENTED_EDGE('',*,*,#9252,.T.);
#12352=ORIENTED_EDGE('',*,*,#9253,.F.);
#12353=ORIENTED_EDGE('',*,*,#9254,.T.);
#12354=ORIENTED_EDGE('',*,*,#9250,.T.);
#12355=ORIENTED_EDGE('',*,*,#9255,.T.);
#12356=ORIENTED_EDGE('',*,*,#9256,.F.);
#12357=ORIENTED_EDGE('',*,*,#9257,.T.);
#12358=ORIENTED_EDGE('',*,*,#9253,.T.);
#12359=ORIENTED_EDGE('',*,*,#9258,.T.);
#12360=ORIENTED_EDGE('',*,*,#9259,.F.);
#12361=ORIENTED_EDGE('',*,*,#9260,.T.);
#12362=ORIENTED_EDGE('',*,*,#9256,.T.);
#12363=ORIENTED_EDGE('',*,*,#9261,.T.);
#12364=ORIENTED_EDGE('',*,*,#9262,.F.);
#12365=ORIENTED_EDGE('',*,*,#9263,.T.);
#12366=ORIENTED_EDGE('',*,*,#9259,.T.);
#12367=ORIENTED_EDGE('',*,*,#9264,.T.);
#12368=ORIENTED_EDGE('',*,*,#9265,.F.);
#12369=ORIENTED_EDGE('',*,*,#9266,.T.);
#12370=ORIENTED_EDGE('',*,*,#9262,.T.);
#12371=ORIENTED_EDGE('',*,*,#9267,.T.);
#12372=ORIENTED_EDGE('',*,*,#9268,.F.);
#12373=ORIENTED_EDGE('',*,*,#9269,.T.);
#12374=ORIENTED_EDGE('',*,*,#9265,.T.);
#12375=ORIENTED_EDGE('',*,*,#9270,.T.);
#12376=ORIENTED_EDGE('',*,*,#9271,.F.);
#12377=ORIENTED_EDGE('',*,*,#9272,.T.);
#12378=ORIENTED_EDGE('',*,*,#9268,.T.);
#12379=ORIENTED_EDGE('',*,*,#9273,.T.);
#12380=ORIENTED_EDGE('',*,*,#9274,.F.);
#12381=ORIENTED_EDGE('',*,*,#9275,.T.);
#12382=ORIENTED_EDGE('',*,*,#9271,.T.);
#12383=ORIENTED_EDGE('',*,*,#9276,.T.);
#12384=ORIENTED_EDGE('',*,*,#9277,.F.);
#12385=ORIENTED_EDGE('',*,*,#9278,.T.);
#12386=ORIENTED_EDGE('',*,*,#9274,.T.);
#12387=ORIENTED_EDGE('',*,*,#9279,.T.);
#12388=ORIENTED_EDGE('',*,*,#9280,.F.);
#12389=ORIENTED_EDGE('',*,*,#9281,.T.);
#12390=ORIENTED_EDGE('',*,*,#9277,.T.);
#12391=ORIENTED_EDGE('',*,*,#9282,.T.);
#12392=ORIENTED_EDGE('',*,*,#9283,.F.);
#12393=ORIENTED_EDGE('',*,*,#9284,.T.);
#12394=ORIENTED_EDGE('',*,*,#9280,.T.);
#12395=ORIENTED_EDGE('',*,*,#9285,.T.);
#12396=ORIENTED_EDGE('',*,*,#9286,.F.);
#12397=ORIENTED_EDGE('',*,*,#9287,.T.);
#12398=ORIENTED_EDGE('',*,*,#9283,.T.);
#12399=ORIENTED_EDGE('',*,*,#9288,.T.);
#12400=ORIENTED_EDGE('',*,*,#9289,.F.);
#12401=ORIENTED_EDGE('',*,*,#9290,.T.);
#12402=ORIENTED_EDGE('',*,*,#9286,.T.);
#12403=ORIENTED_EDGE('',*,*,#9291,.T.);
#12404=ORIENTED_EDGE('',*,*,#9292,.F.);
#12405=ORIENTED_EDGE('',*,*,#9293,.T.);
#12406=ORIENTED_EDGE('',*,*,#9289,.T.);
#12407=ORIENTED_EDGE('',*,*,#9294,.T.);
#12408=ORIENTED_EDGE('',*,*,#9295,.F.);
#12409=ORIENTED_EDGE('',*,*,#9296,.T.);
#12410=ORIENTED_EDGE('',*,*,#9292,.T.);
#12411=ORIENTED_EDGE('',*,*,#9297,.T.);
#12412=ORIENTED_EDGE('',*,*,#9298,.F.);
#12413=ORIENTED_EDGE('',*,*,#9299,.T.);
#12414=ORIENTED_EDGE('',*,*,#9295,.T.);
#12415=ORIENTED_EDGE('',*,*,#9300,.T.);
#12416=ORIENTED_EDGE('',*,*,#9301,.F.);
#12417=ORIENTED_EDGE('',*,*,#9302,.T.);
#12418=ORIENTED_EDGE('',*,*,#9298,.T.);
#12419=ORIENTED_EDGE('',*,*,#9303,.T.);
#12420=ORIENTED_EDGE('',*,*,#9304,.F.);
#12421=ORIENTED_EDGE('',*,*,#9305,.T.);
#12422=ORIENTED_EDGE('',*,*,#9301,.T.);
#12423=ORIENTED_EDGE('',*,*,#9306,.T.);
#12424=ORIENTED_EDGE('',*,*,#9307,.F.);
#12425=ORIENTED_EDGE('',*,*,#9308,.T.);
#12426=ORIENTED_EDGE('',*,*,#9304,.T.);
#12427=ORIENTED_EDGE('',*,*,#9309,.T.);
#12428=ORIENTED_EDGE('',*,*,#9310,.F.);
#12429=ORIENTED_EDGE('',*,*,#9311,.T.);
#12430=ORIENTED_EDGE('',*,*,#9307,.T.);
#12431=ORIENTED_EDGE('',*,*,#9312,.T.);
#12432=ORIENTED_EDGE('',*,*,#9313,.F.);
#12433=ORIENTED_EDGE('',*,*,#9314,.T.);
#12434=ORIENTED_EDGE('',*,*,#9310,.T.);
#12435=ORIENTED_EDGE('',*,*,#9315,.T.);
#12436=ORIENTED_EDGE('',*,*,#9316,.F.);
#12437=ORIENTED_EDGE('',*,*,#9317,.T.);
#12438=ORIENTED_EDGE('',*,*,#9313,.T.);
#12439=ORIENTED_EDGE('',*,*,#9318,.T.);
#12440=ORIENTED_EDGE('',*,*,#9319,.F.);
#12441=ORIENTED_EDGE('',*,*,#9320,.T.);
#12442=ORIENTED_EDGE('',*,*,#9316,.T.);
#12443=ORIENTED_EDGE('',*,*,#9321,.T.);
#12444=ORIENTED_EDGE('',*,*,#9322,.F.);
#12445=ORIENTED_EDGE('',*,*,#9323,.T.);
#12446=ORIENTED_EDGE('',*,*,#9319,.T.);
#12447=ORIENTED_EDGE('',*,*,#9324,.T.);
#12448=ORIENTED_EDGE('',*,*,#9325,.F.);
#12449=ORIENTED_EDGE('',*,*,#9326,.T.);
#12450=ORIENTED_EDGE('',*,*,#9322,.T.);
#12451=ORIENTED_EDGE('',*,*,#9327,.T.);
#12452=ORIENTED_EDGE('',*,*,#9328,.F.);
#12453=ORIENTED_EDGE('',*,*,#9329,.T.);
#12454=ORIENTED_EDGE('',*,*,#9330,.T.);
#12455=ORIENTED_EDGE('',*,*,#9331,.T.);
#12456=ORIENTED_EDGE('',*,*,#9332,.T.);
#12457=ORIENTED_EDGE('',*,*,#9331,.F.);
#12458=ORIENTED_EDGE('',*,*,#9333,.T.);
#12459=ORIENTED_EDGE('',*,*,#9334,.T.);
#12460=ORIENTED_EDGE('',*,*,#9335,.F.);
#12461=ORIENTED_EDGE('',*,*,#9336,.T.);
#12462=ORIENTED_EDGE('',*,*,#9328,.T.);
#12463=ORIENTED_EDGE('',*,*,#9337,.T.);
#12464=ORIENTED_EDGE('',*,*,#9338,.F.);
#12465=ORIENTED_EDGE('',*,*,#9339,.T.);
#12466=ORIENTED_EDGE('',*,*,#9335,.T.);
#12467=ORIENTED_EDGE('',*,*,#9340,.T.);
#12468=ORIENTED_EDGE('',*,*,#9341,.F.);
#12469=ORIENTED_EDGE('',*,*,#9342,.T.);
#12470=ORIENTED_EDGE('',*,*,#9338,.T.);
#12471=ORIENTED_EDGE('',*,*,#9343,.T.);
#12472=ORIENTED_EDGE('',*,*,#9344,.F.);
#12473=ORIENTED_EDGE('',*,*,#9345,.T.);
#12474=ORIENTED_EDGE('',*,*,#9341,.T.);
#12475=ORIENTED_EDGE('',*,*,#9346,.T.);
#12476=ORIENTED_EDGE('',*,*,#9347,.F.);
#12477=ORIENTED_EDGE('',*,*,#9348,.T.);
#12478=ORIENTED_EDGE('',*,*,#9344,.T.);
#12479=ORIENTED_EDGE('',*,*,#9349,.T.);
#12480=ORIENTED_EDGE('',*,*,#9350,.F.);
#12481=ORIENTED_EDGE('',*,*,#9351,.T.);
#12482=ORIENTED_EDGE('',*,*,#9347,.T.);
#12483=ORIENTED_EDGE('',*,*,#9352,.T.);
#12484=ORIENTED_EDGE('',*,*,#9353,.F.);
#12485=ORIENTED_EDGE('',*,*,#9354,.T.);
#12486=ORIENTED_EDGE('',*,*,#9350,.T.);
#12487=ORIENTED_EDGE('',*,*,#9355,.T.);
#12488=ORIENTED_EDGE('',*,*,#9356,.F.);
#12489=ORIENTED_EDGE('',*,*,#9357,.T.);
#12490=ORIENTED_EDGE('',*,*,#9353,.T.);
#12491=ORIENTED_EDGE('',*,*,#9358,.T.);
#12492=ORIENTED_EDGE('',*,*,#9359,.F.);
#12493=ORIENTED_EDGE('',*,*,#9360,.T.);
#12494=ORIENTED_EDGE('',*,*,#9356,.T.);
#12495=ORIENTED_EDGE('',*,*,#9361,.T.);
#12496=ORIENTED_EDGE('',*,*,#9362,.F.);
#12497=ORIENTED_EDGE('',*,*,#9363,.T.);
#12498=ORIENTED_EDGE('',*,*,#9359,.T.);
#12499=ORIENTED_EDGE('',*,*,#9364,.T.);
#12500=ORIENTED_EDGE('',*,*,#9365,.F.);
#12501=ORIENTED_EDGE('',*,*,#9366,.T.);
#12502=ORIENTED_EDGE('',*,*,#9362,.T.);
#12503=ORIENTED_EDGE('',*,*,#9367,.T.);
#12504=ORIENTED_EDGE('',*,*,#9368,.F.);
#12505=ORIENTED_EDGE('',*,*,#9369,.T.);
#12506=ORIENTED_EDGE('',*,*,#9365,.T.);
#12507=ORIENTED_EDGE('',*,*,#9370,.T.);
#12508=ORIENTED_EDGE('',*,*,#9371,.F.);
#12509=ORIENTED_EDGE('',*,*,#9372,.T.);
#12510=ORIENTED_EDGE('',*,*,#9368,.T.);
#12511=ORIENTED_EDGE('',*,*,#9373,.T.);
#12512=ORIENTED_EDGE('',*,*,#9374,.F.);
#12513=ORIENTED_EDGE('',*,*,#9375,.T.);
#12514=ORIENTED_EDGE('',*,*,#9371,.T.);
#12515=ORIENTED_EDGE('',*,*,#9376,.T.);
#12516=ORIENTED_EDGE('',*,*,#9377,.F.);
#12517=ORIENTED_EDGE('',*,*,#9378,.T.);
#12518=ORIENTED_EDGE('',*,*,#9374,.T.);
#12519=ORIENTED_EDGE('',*,*,#9379,.T.);
#12520=ORIENTED_EDGE('',*,*,#9380,.F.);
#12521=ORIENTED_EDGE('',*,*,#9381,.T.);
#12522=ORIENTED_EDGE('',*,*,#9382,.F.);
#12523=ORIENTED_EDGE('',*,*,#9383,.F.);
#12524=ORIENTED_EDGE('',*,*,#9384,.F.);
#12525=ORIENTED_EDGE('',*,*,#9385,.T.);
#12526=ORIENTED_EDGE('',*,*,#9380,.T.);
#12527=ORIENTED_EDGE('',*,*,#9386,.F.);
#12528=ORIENTED_EDGE('',*,*,#9387,.F.);
#12529=ORIENTED_EDGE('',*,*,#9388,.T.);
#12530=ORIENTED_EDGE('',*,*,#9384,.T.);
#12531=ORIENTED_EDGE('',*,*,#9389,.F.);
#12532=ORIENTED_EDGE('',*,*,#9390,.F.);
#12533=ORIENTED_EDGE('',*,*,#9391,.T.);
#12534=ORIENTED_EDGE('',*,*,#9387,.T.);
#12535=ORIENTED_EDGE('',*,*,#9392,.F.);
#12536=ORIENTED_EDGE('',*,*,#9393,.F.);
#12537=ORIENTED_EDGE('',*,*,#9394,.T.);
#12538=ORIENTED_EDGE('',*,*,#9390,.T.);
#12539=ORIENTED_EDGE('',*,*,#9395,.F.);
#12540=ORIENTED_EDGE('',*,*,#9396,.F.);
#12541=ORIENTED_EDGE('',*,*,#9397,.T.);
#12542=ORIENTED_EDGE('',*,*,#9393,.T.);
#12543=ORIENTED_EDGE('',*,*,#9398,.F.);
#12544=ORIENTED_EDGE('',*,*,#9399,.F.);
#12545=ORIENTED_EDGE('',*,*,#9400,.T.);
#12546=ORIENTED_EDGE('',*,*,#9396,.T.);
#12547=ORIENTED_EDGE('',*,*,#9401,.F.);
#12548=ORIENTED_EDGE('',*,*,#9402,.F.);
#12549=ORIENTED_EDGE('',*,*,#9403,.T.);
#12550=ORIENTED_EDGE('',*,*,#9399,.T.);
#12551=ORIENTED_EDGE('',*,*,#9404,.F.);
#12552=ORIENTED_EDGE('',*,*,#9405,.F.);
#12553=ORIENTED_EDGE('',*,*,#9406,.T.);
#12554=ORIENTED_EDGE('',*,*,#9402,.T.);
#12555=ORIENTED_EDGE('',*,*,#9407,.F.);
#12556=ORIENTED_EDGE('',*,*,#9408,.F.);
#12557=ORIENTED_EDGE('',*,*,#9409,.T.);
#12558=ORIENTED_EDGE('',*,*,#9405,.T.);
#12559=ORIENTED_EDGE('',*,*,#9410,.F.);
#12560=ORIENTED_EDGE('',*,*,#9411,.F.);
#12561=ORIENTED_EDGE('',*,*,#9412,.T.);
#12562=ORIENTED_EDGE('',*,*,#9408,.T.);
#12563=ORIENTED_EDGE('',*,*,#9413,.F.);
#12564=ORIENTED_EDGE('',*,*,#9414,.F.);
#12565=ORIENTED_EDGE('',*,*,#9415,.T.);
#12566=ORIENTED_EDGE('',*,*,#9411,.T.);
#12567=ORIENTED_EDGE('',*,*,#9416,.F.);
#12568=ORIENTED_EDGE('',*,*,#9417,.F.);
#12569=ORIENTED_EDGE('',*,*,#9418,.T.);
#12570=ORIENTED_EDGE('',*,*,#9414,.T.);
#12571=ORIENTED_EDGE('',*,*,#9419,.F.);
#12572=ORIENTED_EDGE('',*,*,#9420,.F.);
#12573=ORIENTED_EDGE('',*,*,#9421,.T.);
#12574=ORIENTED_EDGE('',*,*,#9417,.T.);
#12575=ORIENTED_EDGE('',*,*,#9422,.F.);
#12576=ORIENTED_EDGE('',*,*,#9423,.F.);
#12577=ORIENTED_EDGE('',*,*,#9424,.T.);
#12578=ORIENTED_EDGE('',*,*,#9420,.T.);
#12579=ORIENTED_EDGE('',*,*,#9425,.F.);
#12580=ORIENTED_EDGE('',*,*,#9426,.F.);
#12581=ORIENTED_EDGE('',*,*,#9427,.T.);
#12582=ORIENTED_EDGE('',*,*,#9423,.T.);
#12583=ORIENTED_EDGE('',*,*,#9428,.F.);
#12584=ORIENTED_EDGE('',*,*,#9429,.F.);
#12585=ORIENTED_EDGE('',*,*,#9430,.T.);
#12586=ORIENTED_EDGE('',*,*,#9431,.F.);
#12587=ORIENTED_EDGE('',*,*,#9432,.F.);
#12588=ORIENTED_EDGE('',*,*,#9433,.T.);
#12589=ORIENTED_EDGE('',*,*,#9429,.T.);
#12590=ORIENTED_EDGE('',*,*,#9434,.F.);
#12591=ORIENTED_EDGE('',*,*,#9435,.F.);
#12592=ORIENTED_EDGE('',*,*,#9436,.F.);
#12593=ORIENTED_EDGE('',*,*,#9437,.T.);
#12594=ORIENTED_EDGE('',*,*,#9432,.T.);
#12595=ORIENTED_EDGE('',*,*,#9438,.F.);
#12596=ORIENTED_EDGE('',*,*,#9439,.F.);
#12597=ORIENTED_EDGE('',*,*,#9440,.T.);
#12598=ORIENTED_EDGE('',*,*,#9436,.T.);
#12599=ORIENTED_EDGE('',*,*,#9441,.F.);
#12600=ORIENTED_EDGE('',*,*,#9442,.F.);
#12601=ORIENTED_EDGE('',*,*,#9443,.T.);
#12602=ORIENTED_EDGE('',*,*,#9439,.T.);
#12603=ORIENTED_EDGE('',*,*,#9444,.F.);
#12604=ORIENTED_EDGE('',*,*,#9445,.F.);
#12605=ORIENTED_EDGE('',*,*,#9446,.T.);
#12606=ORIENTED_EDGE('',*,*,#9442,.T.);
#12607=ORIENTED_EDGE('',*,*,#9447,.F.);
#12608=ORIENTED_EDGE('',*,*,#9448,.F.);
#12609=ORIENTED_EDGE('',*,*,#9449,.T.);
#12610=ORIENTED_EDGE('',*,*,#9445,.T.);
#12611=ORIENTED_EDGE('',*,*,#9450,.F.);
#12612=ORIENTED_EDGE('',*,*,#9451,.F.);
#12613=ORIENTED_EDGE('',*,*,#9452,.T.);
#12614=ORIENTED_EDGE('',*,*,#9448,.T.);
#12615=ORIENTED_EDGE('',*,*,#9453,.F.);
#12616=ORIENTED_EDGE('',*,*,#9454,.F.);
#12617=ORIENTED_EDGE('',*,*,#9455,.T.);
#12618=ORIENTED_EDGE('',*,*,#9451,.T.);
#12619=ORIENTED_EDGE('',*,*,#9456,.F.);
#12620=ORIENTED_EDGE('',*,*,#9457,.F.);
#12621=ORIENTED_EDGE('',*,*,#9458,.T.);
#12622=ORIENTED_EDGE('',*,*,#9454,.T.);
#12623=ORIENTED_EDGE('',*,*,#9459,.F.);
#12624=ORIENTED_EDGE('',*,*,#9460,.F.);
#12625=ORIENTED_EDGE('',*,*,#9461,.T.);
#12626=ORIENTED_EDGE('',*,*,#9457,.T.);
#12627=ORIENTED_EDGE('',*,*,#9462,.F.);
#12628=ORIENTED_EDGE('',*,*,#9463,.F.);
#12629=ORIENTED_EDGE('',*,*,#9464,.T.);
#12630=ORIENTED_EDGE('',*,*,#9460,.T.);
#12631=ORIENTED_EDGE('',*,*,#9465,.F.);
#12632=ORIENTED_EDGE('',*,*,#9466,.F.);
#12633=ORIENTED_EDGE('',*,*,#9467,.T.);
#12634=ORIENTED_EDGE('',*,*,#9463,.T.);
#12635=ORIENTED_EDGE('',*,*,#9468,.F.);
#12636=ORIENTED_EDGE('',*,*,#9469,.F.);
#12637=ORIENTED_EDGE('',*,*,#9470,.T.);
#12638=ORIENTED_EDGE('',*,*,#9466,.T.);
#12639=ORIENTED_EDGE('',*,*,#9471,.F.);
#12640=ORIENTED_EDGE('',*,*,#9472,.F.);
#12641=ORIENTED_EDGE('',*,*,#9473,.T.);
#12642=ORIENTED_EDGE('',*,*,#9469,.T.);
#12643=ORIENTED_EDGE('',*,*,#9474,.F.);
#12644=ORIENTED_EDGE('',*,*,#9475,.F.);
#12645=ORIENTED_EDGE('',*,*,#9476,.T.);
#12646=ORIENTED_EDGE('',*,*,#9472,.T.);
#12647=ORIENTED_EDGE('',*,*,#9477,.F.);
#12648=ORIENTED_EDGE('',*,*,#9478,.F.);
#12649=ORIENTED_EDGE('',*,*,#9479,.T.);
#12650=ORIENTED_EDGE('',*,*,#9475,.T.);
#12651=ORIENTED_EDGE('',*,*,#9480,.F.);
#12652=ORIENTED_EDGE('',*,*,#9481,.F.);
#12653=ORIENTED_EDGE('',*,*,#9482,.T.);
#12654=ORIENTED_EDGE('',*,*,#9478,.T.);
#12655=ORIENTED_EDGE('',*,*,#9483,.F.);
#12656=ORIENTED_EDGE('',*,*,#9484,.F.);
#12657=ORIENTED_EDGE('',*,*,#9485,.T.);
#12658=ORIENTED_EDGE('',*,*,#9481,.T.);
#12659=ORIENTED_EDGE('',*,*,#9486,.F.);
#12660=ORIENTED_EDGE('',*,*,#9487,.F.);
#12661=ORIENTED_EDGE('',*,*,#9488,.T.);
#12662=ORIENTED_EDGE('',*,*,#9484,.T.);
#12663=ORIENTED_EDGE('',*,*,#9489,.F.);
#12664=ORIENTED_EDGE('',*,*,#9490,.F.);
#12665=ORIENTED_EDGE('',*,*,#9491,.T.);
#12666=ORIENTED_EDGE('',*,*,#9487,.T.);
#12667=ORIENTED_EDGE('',*,*,#9492,.F.);
#12668=ORIENTED_EDGE('',*,*,#9493,.F.);
#12669=ORIENTED_EDGE('',*,*,#9494,.T.);
#12670=ORIENTED_EDGE('',*,*,#9490,.T.);
#12671=ORIENTED_EDGE('',*,*,#9495,.F.);
#12672=ORIENTED_EDGE('',*,*,#9496,.F.);
#12673=ORIENTED_EDGE('',*,*,#9497,.T.);
#12674=ORIENTED_EDGE('',*,*,#9493,.T.);
#12675=ORIENTED_EDGE('',*,*,#9498,.F.);
#12676=ORIENTED_EDGE('',*,*,#9499,.F.);
#12677=ORIENTED_EDGE('',*,*,#9500,.T.);
#12678=ORIENTED_EDGE('',*,*,#9496,.T.);
#12679=ORIENTED_EDGE('',*,*,#9501,.F.);
#12680=ORIENTED_EDGE('',*,*,#9502,.F.);
#12681=ORIENTED_EDGE('',*,*,#9503,.T.);
#12682=ORIENTED_EDGE('',*,*,#9499,.T.);
#12683=ORIENTED_EDGE('',*,*,#9504,.F.);
#12684=ORIENTED_EDGE('',*,*,#9505,.F.);
#12685=ORIENTED_EDGE('',*,*,#9506,.T.);
#12686=ORIENTED_EDGE('',*,*,#9502,.T.);
#12687=ORIENTED_EDGE('',*,*,#9507,.F.);
#12688=ORIENTED_EDGE('',*,*,#9508,.F.);
#12689=ORIENTED_EDGE('',*,*,#9509,.T.);
#12690=ORIENTED_EDGE('',*,*,#9505,.T.);
#12691=ORIENTED_EDGE('',*,*,#9510,.F.);
#12692=ORIENTED_EDGE('',*,*,#9511,.F.);
#12693=ORIENTED_EDGE('',*,*,#9512,.T.);
#12694=ORIENTED_EDGE('',*,*,#9508,.T.);
#12695=ORIENTED_EDGE('',*,*,#9513,.F.);
#12696=ORIENTED_EDGE('',*,*,#9514,.F.);
#12697=ORIENTED_EDGE('',*,*,#9515,.T.);
#12698=ORIENTED_EDGE('',*,*,#9511,.T.);
#12699=ORIENTED_EDGE('',*,*,#9516,.F.);
#12700=ORIENTED_EDGE('',*,*,#9517,.F.);
#12701=ORIENTED_EDGE('',*,*,#9518,.T.);
#12702=ORIENTED_EDGE('',*,*,#9514,.T.);
#12703=ORIENTED_EDGE('',*,*,#9519,.F.);
#12704=ORIENTED_EDGE('',*,*,#9520,.F.);
#12705=ORIENTED_EDGE('',*,*,#9521,.T.);
#12706=ORIENTED_EDGE('',*,*,#9517,.T.);
#12707=ORIENTED_EDGE('',*,*,#9522,.F.);
#12708=ORIENTED_EDGE('',*,*,#9523,.F.);
#12709=ORIENTED_EDGE('',*,*,#9524,.T.);
#12710=ORIENTED_EDGE('',*,*,#9520,.T.);
#12711=ORIENTED_EDGE('',*,*,#9525,.F.);
#12712=ORIENTED_EDGE('',*,*,#9526,.F.);
#12713=ORIENTED_EDGE('',*,*,#9527,.T.);
#12714=ORIENTED_EDGE('',*,*,#9523,.T.);
#12715=ORIENTED_EDGE('',*,*,#9528,.F.);
#12716=ORIENTED_EDGE('',*,*,#9529,.F.);
#12717=ORIENTED_EDGE('',*,*,#9530,.T.);
#12718=ORIENTED_EDGE('',*,*,#9526,.T.);
#12719=ORIENTED_EDGE('',*,*,#9531,.F.);
#12720=ORIENTED_EDGE('',*,*,#9532,.F.);
#12721=ORIENTED_EDGE('',*,*,#9533,.T.);
#12722=ORIENTED_EDGE('',*,*,#9529,.T.);
#12723=ORIENTED_EDGE('',*,*,#9534,.F.);
#12724=ORIENTED_EDGE('',*,*,#9535,.F.);
#12725=ORIENTED_EDGE('',*,*,#9536,.T.);
#12726=ORIENTED_EDGE('',*,*,#9532,.T.);
#12727=ORIENTED_EDGE('',*,*,#9537,.F.);
#12728=ORIENTED_EDGE('',*,*,#9538,.F.);
#12729=ORIENTED_EDGE('',*,*,#9539,.T.);
#12730=ORIENTED_EDGE('',*,*,#9535,.T.);
#12731=ORIENTED_EDGE('',*,*,#9540,.F.);
#12732=ORIENTED_EDGE('',*,*,#9541,.F.);
#12733=ORIENTED_EDGE('',*,*,#9542,.T.);
#12734=ORIENTED_EDGE('',*,*,#9538,.T.);
#12735=ORIENTED_EDGE('',*,*,#9543,.F.);
#12736=ORIENTED_EDGE('',*,*,#9544,.F.);
#12737=ORIENTED_EDGE('',*,*,#9545,.T.);
#12738=ORIENTED_EDGE('',*,*,#9541,.T.);
#12739=ORIENTED_EDGE('',*,*,#9546,.F.);
#12740=ORIENTED_EDGE('',*,*,#9547,.F.);
#12741=ORIENTED_EDGE('',*,*,#9548,.T.);
#12742=ORIENTED_EDGE('',*,*,#9544,.T.);
#12743=ORIENTED_EDGE('',*,*,#9549,.F.);
#12744=ORIENTED_EDGE('',*,*,#9550,.F.);
#12745=ORIENTED_EDGE('',*,*,#9551,.T.);
#12746=ORIENTED_EDGE('',*,*,#9547,.T.);
#12747=ORIENTED_EDGE('',*,*,#9552,.F.);
#12748=ORIENTED_EDGE('',*,*,#9553,.F.);
#12749=ORIENTED_EDGE('',*,*,#9554,.T.);
#12750=ORIENTED_EDGE('',*,*,#9550,.T.);
#12751=ORIENTED_EDGE('',*,*,#9555,.F.);
#12752=ORIENTED_EDGE('',*,*,#9556,.F.);
#12753=ORIENTED_EDGE('',*,*,#9557,.T.);
#12754=ORIENTED_EDGE('',*,*,#9553,.T.);
#12755=ORIENTED_EDGE('',*,*,#9558,.F.);
#12756=ORIENTED_EDGE('',*,*,#9559,.F.);
#12757=ORIENTED_EDGE('',*,*,#9560,.T.);
#12758=ORIENTED_EDGE('',*,*,#9556,.T.);
#12759=ORIENTED_EDGE('',*,*,#9561,.F.);
#12760=ORIENTED_EDGE('',*,*,#9562,.F.);
#12761=ORIENTED_EDGE('',*,*,#9563,.T.);
#12762=ORIENTED_EDGE('',*,*,#9559,.T.);
#12763=ORIENTED_EDGE('',*,*,#9564,.F.);
#12764=ORIENTED_EDGE('',*,*,#9565,.F.);
#12765=ORIENTED_EDGE('',*,*,#9566,.T.);
#12766=ORIENTED_EDGE('',*,*,#9562,.T.);
#12767=ORIENTED_EDGE('',*,*,#9567,.F.);
#12768=ORIENTED_EDGE('',*,*,#9568,.F.);
#12769=ORIENTED_EDGE('',*,*,#9569,.T.);
#12770=ORIENTED_EDGE('',*,*,#9565,.T.);
#12771=ORIENTED_EDGE('',*,*,#9570,.F.);
#12772=ORIENTED_EDGE('',*,*,#9571,.F.);
#12773=ORIENTED_EDGE('',*,*,#9572,.T.);
#12774=ORIENTED_EDGE('',*,*,#9568,.T.);
#12775=ORIENTED_EDGE('',*,*,#9573,.F.);
#12776=ORIENTED_EDGE('',*,*,#9574,.F.);
#12777=ORIENTED_EDGE('',*,*,#9575,.T.);
#12778=ORIENTED_EDGE('',*,*,#9571,.T.);
#12779=ORIENTED_EDGE('',*,*,#9576,.F.);
#12780=ORIENTED_EDGE('',*,*,#9577,.F.);
#12781=ORIENTED_EDGE('',*,*,#9578,.T.);
#12782=ORIENTED_EDGE('',*,*,#9574,.T.);
#12783=ORIENTED_EDGE('',*,*,#9579,.F.);
#12784=ORIENTED_EDGE('',*,*,#9580,.F.);
#12785=ORIENTED_EDGE('',*,*,#9581,.T.);
#12786=ORIENTED_EDGE('',*,*,#9577,.T.);
#12787=ORIENTED_EDGE('',*,*,#9582,.F.);
#12788=ORIENTED_EDGE('',*,*,#9583,.F.);
#12789=ORIENTED_EDGE('',*,*,#9584,.T.);
#12790=ORIENTED_EDGE('',*,*,#9580,.T.);
#12791=ORIENTED_EDGE('',*,*,#9585,.F.);
#12792=ORIENTED_EDGE('',*,*,#9586,.F.);
#12793=ORIENTED_EDGE('',*,*,#9587,.T.);
#12794=ORIENTED_EDGE('',*,*,#9583,.T.);
#12795=ORIENTED_EDGE('',*,*,#9588,.F.);
#12796=ORIENTED_EDGE('',*,*,#9589,.F.);
#12797=ORIENTED_EDGE('',*,*,#9590,.T.);
#12798=ORIENTED_EDGE('',*,*,#9586,.T.);
#12799=ORIENTED_EDGE('',*,*,#9591,.F.);
#12800=ORIENTED_EDGE('',*,*,#9592,.F.);
#12801=ORIENTED_EDGE('',*,*,#9593,.T.);
#12802=ORIENTED_EDGE('',*,*,#9589,.T.);
#12803=ORIENTED_EDGE('',*,*,#9594,.F.);
#12804=ORIENTED_EDGE('',*,*,#9595,.F.);
#12805=ORIENTED_EDGE('',*,*,#9596,.T.);
#12806=ORIENTED_EDGE('',*,*,#9592,.T.);
#12807=ORIENTED_EDGE('',*,*,#9597,.F.);
#12808=ORIENTED_EDGE('',*,*,#9598,.F.);
#12809=ORIENTED_EDGE('',*,*,#9599,.T.);
#12810=ORIENTED_EDGE('',*,*,#9595,.T.);
#12811=ORIENTED_EDGE('',*,*,#9600,.F.);
#12812=ORIENTED_EDGE('',*,*,#9601,.F.);
#12813=ORIENTED_EDGE('',*,*,#9602,.T.);
#12814=ORIENTED_EDGE('',*,*,#9598,.T.);
#12815=ORIENTED_EDGE('',*,*,#9603,.F.);
#12816=ORIENTED_EDGE('',*,*,#9604,.F.);
#12817=ORIENTED_EDGE('',*,*,#9605,.T.);
#12818=ORIENTED_EDGE('',*,*,#9601,.T.);
#12819=ORIENTED_EDGE('',*,*,#9606,.F.);
#12820=ORIENTED_EDGE('',*,*,#9607,.F.);
#12821=ORIENTED_EDGE('',*,*,#9608,.T.);
#12822=ORIENTED_EDGE('',*,*,#9604,.T.);
#12823=ORIENTED_EDGE('',*,*,#9609,.F.);
#12824=ORIENTED_EDGE('',*,*,#9610,.F.);
#12825=ORIENTED_EDGE('',*,*,#9611,.T.);
#12826=ORIENTED_EDGE('',*,*,#9607,.T.);
#12827=ORIENTED_EDGE('',*,*,#9612,.F.);
#12828=ORIENTED_EDGE('',*,*,#9613,.F.);
#12829=ORIENTED_EDGE('',*,*,#9614,.T.);
#12830=ORIENTED_EDGE('',*,*,#9610,.T.);
#12831=ORIENTED_EDGE('',*,*,#9615,.F.);
#12832=ORIENTED_EDGE('',*,*,#9616,.F.);
#12833=ORIENTED_EDGE('',*,*,#9617,.T.);
#12834=ORIENTED_EDGE('',*,*,#9613,.T.);
#12835=ORIENTED_EDGE('',*,*,#9618,.F.);
#12836=ORIENTED_EDGE('',*,*,#9143,.F.);
#12837=ORIENTED_EDGE('',*,*,#9619,.F.);
#12838=ORIENTED_EDGE('',*,*,#9137,.F.);
#12839=ORIENTED_EDGE('',*,*,#9620,.F.);
#12840=ORIENTED_EDGE('',*,*,#9144,.F.);
#12841=ORIENTED_EDGE('',*,*,#9620,.T.);
#12842=ORIENTED_EDGE('',*,*,#9136,.F.);
#12843=ORIENTED_EDGE('',*,*,#9133,.F.);
#12844=ORIENTED_EDGE('',*,*,#9621,.T.);
#12845=ORIENTED_EDGE('',*,*,#9141,.F.);
#12846=ORIENTED_EDGE('',*,*,#9621,.F.);
#12847=ORIENTED_EDGE('',*,*,#9132,.F.);
#12848=ORIENTED_EDGE('',*,*,#9622,.F.);
#12849=ORIENTED_EDGE('',*,*,#9142,.F.);
#12850=ORIENTED_EDGE('',*,*,#9622,.T.);
#12851=ORIENTED_EDGE('',*,*,#9131,.F.);
#12852=ORIENTED_EDGE('',*,*,#9138,.F.);
#12853=ORIENTED_EDGE('',*,*,#9619,.T.);
#12854=ORIENTED_EDGE('',*,*,#9434,.T.);
#12855=ORIENTED_EDGE('',*,*,#9431,.T.);
#12856=ORIENTED_EDGE('',*,*,#9623,.T.);
#12857=ORIENTED_EDGE('',*,*,#9624,.F.);
#12858=ORIENTED_EDGE('',*,*,#9625,.F.);
#12859=ORIENTED_EDGE('',*,*,#9626,.T.);
#12860=ORIENTED_EDGE('',*,*,#9626,.F.);
#12861=ORIENTED_EDGE('',*,*,#9627,.F.);
#12862=ORIENTED_EDGE('',*,*,#9327,.F.);
#12863=ORIENTED_EDGE('',*,*,#9324,.F.);
#12864=ORIENTED_EDGE('',*,*,#9321,.F.);
#12865=ORIENTED_EDGE('',*,*,#9318,.F.);
#12866=ORIENTED_EDGE('',*,*,#9315,.F.);
#12867=ORIENTED_EDGE('',*,*,#9312,.F.);
#12868=ORIENTED_EDGE('',*,*,#9309,.F.);
#12869=ORIENTED_EDGE('',*,*,#9306,.F.);
#12870=ORIENTED_EDGE('',*,*,#9303,.F.);
#12871=ORIENTED_EDGE('',*,*,#9300,.F.);
#12872=ORIENTED_EDGE('',*,*,#9297,.F.);
#12873=ORIENTED_EDGE('',*,*,#9294,.F.);
#12874=ORIENTED_EDGE('',*,*,#9291,.F.);
#12875=ORIENTED_EDGE('',*,*,#9288,.F.);
#12876=ORIENTED_EDGE('',*,*,#9285,.F.);
#12877=ORIENTED_EDGE('',*,*,#9282,.F.);
#12878=ORIENTED_EDGE('',*,*,#9279,.F.);
#12879=ORIENTED_EDGE('',*,*,#9276,.F.);
#12880=ORIENTED_EDGE('',*,*,#9273,.F.);
#12881=ORIENTED_EDGE('',*,*,#9270,.F.);
#12882=ORIENTED_EDGE('',*,*,#9267,.F.);
#12883=ORIENTED_EDGE('',*,*,#9264,.F.);
#12884=ORIENTED_EDGE('',*,*,#9261,.F.);
#12885=ORIENTED_EDGE('',*,*,#9258,.F.);
#12886=ORIENTED_EDGE('',*,*,#9255,.F.);
#12887=ORIENTED_EDGE('',*,*,#9252,.F.);
#12888=ORIENTED_EDGE('',*,*,#9249,.F.);
#12889=ORIENTED_EDGE('',*,*,#9246,.F.);
#12890=ORIENTED_EDGE('',*,*,#9243,.F.);
#12891=ORIENTED_EDGE('',*,*,#9240,.F.);
#12892=ORIENTED_EDGE('',*,*,#9237,.F.);
#12893=ORIENTED_EDGE('',*,*,#9234,.F.);
#12894=ORIENTED_EDGE('',*,*,#9231,.F.);
#12895=ORIENTED_EDGE('',*,*,#9228,.F.);
#12896=ORIENTED_EDGE('',*,*,#9225,.F.);
#12897=ORIENTED_EDGE('',*,*,#9222,.F.);
#12898=ORIENTED_EDGE('',*,*,#9219,.F.);
#12899=ORIENTED_EDGE('',*,*,#9216,.F.);
#12900=ORIENTED_EDGE('',*,*,#9213,.F.);
#12901=ORIENTED_EDGE('',*,*,#9210,.F.);
#12902=ORIENTED_EDGE('',*,*,#9207,.F.);
#12903=ORIENTED_EDGE('',*,*,#9204,.F.);
#12904=ORIENTED_EDGE('',*,*,#9201,.F.);
#12905=ORIENTED_EDGE('',*,*,#9198,.F.);
#12906=ORIENTED_EDGE('',*,*,#9195,.F.);
#12907=ORIENTED_EDGE('',*,*,#9192,.F.);
#12908=ORIENTED_EDGE('',*,*,#9189,.F.);
#12909=ORIENTED_EDGE('',*,*,#9186,.F.);
#12910=ORIENTED_EDGE('',*,*,#9183,.F.);
#12911=ORIENTED_EDGE('',*,*,#9180,.F.);
#12912=ORIENTED_EDGE('',*,*,#9177,.F.);
#12913=ORIENTED_EDGE('',*,*,#9174,.F.);
#12914=ORIENTED_EDGE('',*,*,#9171,.F.);
#12915=ORIENTED_EDGE('',*,*,#9168,.F.);
#12916=ORIENTED_EDGE('',*,*,#9165,.F.);
#12917=ORIENTED_EDGE('',*,*,#9162,.F.);
#12918=ORIENTED_EDGE('',*,*,#9159,.F.);
#12919=ORIENTED_EDGE('',*,*,#9156,.F.);
#12920=ORIENTED_EDGE('',*,*,#9153,.F.);
#12921=ORIENTED_EDGE('',*,*,#9150,.F.);
#12922=ORIENTED_EDGE('',*,*,#9147,.F.);
#12923=ORIENTED_EDGE('',*,*,#9140,.F.);
#12924=ORIENTED_EDGE('',*,*,#9628,.F.);
#12925=ORIENTED_EDGE('',*,*,#9629,.T.);
#12926=ORIENTED_EDGE('',*,*,#9618,.T.);
#12927=ORIENTED_EDGE('',*,*,#9615,.T.);
#12928=ORIENTED_EDGE('',*,*,#9612,.T.);
#12929=ORIENTED_EDGE('',*,*,#9609,.T.);
#12930=ORIENTED_EDGE('',*,*,#9606,.T.);
#12931=ORIENTED_EDGE('',*,*,#9603,.T.);
#12932=ORIENTED_EDGE('',*,*,#9600,.T.);
#12933=ORIENTED_EDGE('',*,*,#9597,.T.);
#12934=ORIENTED_EDGE('',*,*,#9594,.T.);
#12935=ORIENTED_EDGE('',*,*,#9591,.T.);
#12936=ORIENTED_EDGE('',*,*,#9588,.T.);
#12937=ORIENTED_EDGE('',*,*,#9585,.T.);
#12938=ORIENTED_EDGE('',*,*,#9582,.T.);
#12939=ORIENTED_EDGE('',*,*,#9579,.T.);
#12940=ORIENTED_EDGE('',*,*,#9576,.T.);
#12941=ORIENTED_EDGE('',*,*,#9573,.T.);
#12942=ORIENTED_EDGE('',*,*,#9570,.T.);
#12943=ORIENTED_EDGE('',*,*,#9567,.T.);
#12944=ORIENTED_EDGE('',*,*,#9564,.T.);
#12945=ORIENTED_EDGE('',*,*,#9561,.T.);
#12946=ORIENTED_EDGE('',*,*,#9558,.T.);
#12947=ORIENTED_EDGE('',*,*,#9555,.T.);
#12948=ORIENTED_EDGE('',*,*,#9552,.T.);
#12949=ORIENTED_EDGE('',*,*,#9549,.T.);
#12950=ORIENTED_EDGE('',*,*,#9546,.T.);
#12951=ORIENTED_EDGE('',*,*,#9543,.T.);
#12952=ORIENTED_EDGE('',*,*,#9540,.T.);
#12953=ORIENTED_EDGE('',*,*,#9537,.T.);
#12954=ORIENTED_EDGE('',*,*,#9534,.T.);
#12955=ORIENTED_EDGE('',*,*,#9531,.T.);
#12956=ORIENTED_EDGE('',*,*,#9528,.T.);
#12957=ORIENTED_EDGE('',*,*,#9525,.T.);
#12958=ORIENTED_EDGE('',*,*,#9522,.T.);
#12959=ORIENTED_EDGE('',*,*,#9519,.T.);
#12960=ORIENTED_EDGE('',*,*,#9516,.T.);
#12961=ORIENTED_EDGE('',*,*,#9513,.T.);
#12962=ORIENTED_EDGE('',*,*,#9510,.T.);
#12963=ORIENTED_EDGE('',*,*,#9507,.T.);
#12964=ORIENTED_EDGE('',*,*,#9504,.T.);
#12965=ORIENTED_EDGE('',*,*,#9501,.T.);
#12966=ORIENTED_EDGE('',*,*,#9498,.T.);
#12967=ORIENTED_EDGE('',*,*,#9495,.T.);
#12968=ORIENTED_EDGE('',*,*,#9492,.T.);
#12969=ORIENTED_EDGE('',*,*,#9489,.T.);
#12970=ORIENTED_EDGE('',*,*,#9486,.T.);
#12971=ORIENTED_EDGE('',*,*,#9483,.T.);
#12972=ORIENTED_EDGE('',*,*,#9480,.T.);
#12973=ORIENTED_EDGE('',*,*,#9477,.T.);
#12974=ORIENTED_EDGE('',*,*,#9474,.T.);
#12975=ORIENTED_EDGE('',*,*,#9471,.T.);
#12976=ORIENTED_EDGE('',*,*,#9468,.T.);
#12977=ORIENTED_EDGE('',*,*,#9465,.T.);
#12978=ORIENTED_EDGE('',*,*,#9462,.T.);
#12979=ORIENTED_EDGE('',*,*,#9459,.T.);
#12980=ORIENTED_EDGE('',*,*,#9456,.T.);
#12981=ORIENTED_EDGE('',*,*,#9453,.T.);
#12982=ORIENTED_EDGE('',*,*,#9450,.T.);
#12983=ORIENTED_EDGE('',*,*,#9447,.T.);
#12984=ORIENTED_EDGE('',*,*,#9444,.T.);
#12985=ORIENTED_EDGE('',*,*,#9441,.T.);
#12986=ORIENTED_EDGE('',*,*,#9438,.T.);
#12987=ORIENTED_EDGE('',*,*,#9435,.T.);
#12988=ORIENTED_EDGE('',*,*,#9129,.F.);
#12989=ORIENTED_EDGE('',*,*,#9630,.T.);
#12990=ORIENTED_EDGE('',*,*,#9631,.T.);
#12991=ORIENTED_EDGE('',*,*,#9628,.T.);
#12992=ORIENTED_EDGE('',*,*,#9139,.F.);
#12993=ORIENTED_EDGE('',*,*,#9616,.T.);
#12994=ORIENTED_EDGE('',*,*,#9629,.F.);
#12995=ORIENTED_EDGE('',*,*,#9631,.F.);
#12996=ORIENTED_EDGE('',*,*,#9632,.T.);
#12997=ORIENTED_EDGE('',*,*,#9623,.F.);
#12998=ORIENTED_EDGE('',*,*,#9430,.F.);
#12999=ORIENTED_EDGE('',*,*,#9433,.F.);
#13000=ORIENTED_EDGE('',*,*,#9437,.F.);
#13001=ORIENTED_EDGE('',*,*,#9440,.F.);
#13002=ORIENTED_EDGE('',*,*,#9443,.F.);
#13003=ORIENTED_EDGE('',*,*,#9446,.F.);
#13004=ORIENTED_EDGE('',*,*,#9449,.F.);
#13005=ORIENTED_EDGE('',*,*,#9452,.F.);
#13006=ORIENTED_EDGE('',*,*,#9455,.F.);
#13007=ORIENTED_EDGE('',*,*,#9458,.F.);
#13008=ORIENTED_EDGE('',*,*,#9461,.F.);
#13009=ORIENTED_EDGE('',*,*,#9464,.F.);
#13010=ORIENTED_EDGE('',*,*,#9467,.F.);
#13011=ORIENTED_EDGE('',*,*,#9470,.F.);
#13012=ORIENTED_EDGE('',*,*,#9473,.F.);
#13013=ORIENTED_EDGE('',*,*,#9476,.F.);
#13014=ORIENTED_EDGE('',*,*,#9479,.F.);
#13015=ORIENTED_EDGE('',*,*,#9482,.F.);
#13016=ORIENTED_EDGE('',*,*,#9485,.F.);
#13017=ORIENTED_EDGE('',*,*,#9488,.F.);
#13018=ORIENTED_EDGE('',*,*,#9491,.F.);
#13019=ORIENTED_EDGE('',*,*,#9494,.F.);
#13020=ORIENTED_EDGE('',*,*,#9497,.F.);
#13021=ORIENTED_EDGE('',*,*,#9500,.F.);
#13022=ORIENTED_EDGE('',*,*,#9503,.F.);
#13023=ORIENTED_EDGE('',*,*,#9506,.F.);
#13024=ORIENTED_EDGE('',*,*,#9509,.F.);
#13025=ORIENTED_EDGE('',*,*,#9512,.F.);
#13026=ORIENTED_EDGE('',*,*,#9515,.F.);
#13027=ORIENTED_EDGE('',*,*,#9518,.F.);
#13028=ORIENTED_EDGE('',*,*,#9521,.F.);
#13029=ORIENTED_EDGE('',*,*,#9524,.F.);
#13030=ORIENTED_EDGE('',*,*,#9527,.F.);
#13031=ORIENTED_EDGE('',*,*,#9530,.F.);
#13032=ORIENTED_EDGE('',*,*,#9533,.F.);
#13033=ORIENTED_EDGE('',*,*,#9536,.F.);
#13034=ORIENTED_EDGE('',*,*,#9539,.F.);
#13035=ORIENTED_EDGE('',*,*,#9542,.F.);
#13036=ORIENTED_EDGE('',*,*,#9545,.F.);
#13037=ORIENTED_EDGE('',*,*,#9548,.F.);
#13038=ORIENTED_EDGE('',*,*,#9551,.F.);
#13039=ORIENTED_EDGE('',*,*,#9554,.F.);
#13040=ORIENTED_EDGE('',*,*,#9557,.F.);
#13041=ORIENTED_EDGE('',*,*,#9560,.F.);
#13042=ORIENTED_EDGE('',*,*,#9563,.F.);
#13043=ORIENTED_EDGE('',*,*,#9566,.F.);
#13044=ORIENTED_EDGE('',*,*,#9569,.F.);
#13045=ORIENTED_EDGE('',*,*,#9572,.F.);
#13046=ORIENTED_EDGE('',*,*,#9575,.F.);
#13047=ORIENTED_EDGE('',*,*,#9578,.F.);
#13048=ORIENTED_EDGE('',*,*,#9581,.F.);
#13049=ORIENTED_EDGE('',*,*,#9584,.F.);
#13050=ORIENTED_EDGE('',*,*,#9587,.F.);
#13051=ORIENTED_EDGE('',*,*,#9590,.F.);
#13052=ORIENTED_EDGE('',*,*,#9593,.F.);
#13053=ORIENTED_EDGE('',*,*,#9596,.F.);
#13054=ORIENTED_EDGE('',*,*,#9599,.F.);
#13055=ORIENTED_EDGE('',*,*,#9602,.F.);
#13056=ORIENTED_EDGE('',*,*,#9605,.F.);
#13057=ORIENTED_EDGE('',*,*,#9608,.F.);
#13058=ORIENTED_EDGE('',*,*,#9611,.F.);
#13059=ORIENTED_EDGE('',*,*,#9614,.F.);
#13060=ORIENTED_EDGE('',*,*,#9617,.F.);
#13061=ORIENTED_EDGE('',*,*,#9632,.F.);
#13062=ORIENTED_EDGE('',*,*,#9630,.F.);
#13063=ORIENTED_EDGE('',*,*,#9128,.F.);
#13064=ORIENTED_EDGE('',*,*,#9146,.F.);
#13065=ORIENTED_EDGE('',*,*,#9149,.F.);
#13066=ORIENTED_EDGE('',*,*,#9152,.F.);
#13067=ORIENTED_EDGE('',*,*,#9155,.F.);
#13068=ORIENTED_EDGE('',*,*,#9158,.F.);
#13069=ORIENTED_EDGE('',*,*,#9161,.F.);
#13070=ORIENTED_EDGE('',*,*,#9164,.F.);
#13071=ORIENTED_EDGE('',*,*,#9167,.F.);
#13072=ORIENTED_EDGE('',*,*,#9170,.F.);
#13073=ORIENTED_EDGE('',*,*,#9173,.F.);
#13074=ORIENTED_EDGE('',*,*,#9176,.F.);
#13075=ORIENTED_EDGE('',*,*,#9179,.F.);
#13076=ORIENTED_EDGE('',*,*,#9182,.F.);
#13077=ORIENTED_EDGE('',*,*,#9185,.F.);
#13078=ORIENTED_EDGE('',*,*,#9188,.F.);
#13079=ORIENTED_EDGE('',*,*,#9191,.F.);
#13080=ORIENTED_EDGE('',*,*,#9194,.F.);
#13081=ORIENTED_EDGE('',*,*,#9197,.F.);
#13082=ORIENTED_EDGE('',*,*,#9200,.F.);
#13083=ORIENTED_EDGE('',*,*,#9203,.F.);
#13084=ORIENTED_EDGE('',*,*,#9206,.F.);
#13085=ORIENTED_EDGE('',*,*,#9209,.F.);
#13086=ORIENTED_EDGE('',*,*,#9212,.F.);
#13087=ORIENTED_EDGE('',*,*,#9215,.F.);
#13088=ORIENTED_EDGE('',*,*,#9218,.F.);
#13089=ORIENTED_EDGE('',*,*,#9221,.F.);
#13090=ORIENTED_EDGE('',*,*,#9224,.F.);
#13091=ORIENTED_EDGE('',*,*,#9227,.F.);
#13092=ORIENTED_EDGE('',*,*,#9230,.F.);
#13093=ORIENTED_EDGE('',*,*,#9233,.F.);
#13094=ORIENTED_EDGE('',*,*,#9236,.F.);
#13095=ORIENTED_EDGE('',*,*,#9239,.F.);
#13096=ORIENTED_EDGE('',*,*,#9242,.F.);
#13097=ORIENTED_EDGE('',*,*,#9245,.F.);
#13098=ORIENTED_EDGE('',*,*,#9248,.F.);
#13099=ORIENTED_EDGE('',*,*,#9251,.F.);
#13100=ORIENTED_EDGE('',*,*,#9254,.F.);
#13101=ORIENTED_EDGE('',*,*,#9257,.F.);
#13102=ORIENTED_EDGE('',*,*,#9260,.F.);
#13103=ORIENTED_EDGE('',*,*,#9263,.F.);
#13104=ORIENTED_EDGE('',*,*,#9266,.F.);
#13105=ORIENTED_EDGE('',*,*,#9269,.F.);
#13106=ORIENTED_EDGE('',*,*,#9272,.F.);
#13107=ORIENTED_EDGE('',*,*,#9275,.F.);
#13108=ORIENTED_EDGE('',*,*,#9278,.F.);
#13109=ORIENTED_EDGE('',*,*,#9281,.F.);
#13110=ORIENTED_EDGE('',*,*,#9284,.F.);
#13111=ORIENTED_EDGE('',*,*,#9287,.F.);
#13112=ORIENTED_EDGE('',*,*,#9290,.F.);
#13113=ORIENTED_EDGE('',*,*,#9293,.F.);
#13114=ORIENTED_EDGE('',*,*,#9296,.F.);
#13115=ORIENTED_EDGE('',*,*,#9299,.F.);
#13116=ORIENTED_EDGE('',*,*,#9302,.F.);
#13117=ORIENTED_EDGE('',*,*,#9305,.F.);
#13118=ORIENTED_EDGE('',*,*,#9308,.F.);
#13119=ORIENTED_EDGE('',*,*,#9311,.F.);
#13120=ORIENTED_EDGE('',*,*,#9314,.F.);
#13121=ORIENTED_EDGE('',*,*,#9317,.F.);
#13122=ORIENTED_EDGE('',*,*,#9320,.F.);
#13123=ORIENTED_EDGE('',*,*,#9323,.F.);
#13124=ORIENTED_EDGE('',*,*,#9326,.F.);
#13125=ORIENTED_EDGE('',*,*,#9633,.F.);
#13126=ORIENTED_EDGE('',*,*,#9382,.T.);
#13127=ORIENTED_EDGE('',*,*,#9634,.T.);
#13128=ORIENTED_EDGE('',*,*,#9635,.F.);
#13129=ORIENTED_EDGE('',*,*,#9636,.F.);
#13130=ORIENTED_EDGE('',*,*,#9637,.T.);
#13131=ORIENTED_EDGE('',*,*,#9637,.F.);
#13132=ORIENTED_EDGE('',*,*,#9638,.F.);
#13133=ORIENTED_EDGE('',*,*,#9379,.F.);
#13134=ORIENTED_EDGE('',*,*,#9376,.F.);
#13135=ORIENTED_EDGE('',*,*,#9373,.F.);
#13136=ORIENTED_EDGE('',*,*,#9370,.F.);
#13137=ORIENTED_EDGE('',*,*,#9367,.F.);
#13138=ORIENTED_EDGE('',*,*,#9364,.F.);
#13139=ORIENTED_EDGE('',*,*,#9361,.F.);
#13140=ORIENTED_EDGE('',*,*,#9358,.F.);
#13141=ORIENTED_EDGE('',*,*,#9355,.F.);
#13142=ORIENTED_EDGE('',*,*,#9352,.F.);
#13143=ORIENTED_EDGE('',*,*,#9349,.F.);
#13144=ORIENTED_EDGE('',*,*,#9346,.F.);
#13145=ORIENTED_EDGE('',*,*,#9343,.F.);
#13146=ORIENTED_EDGE('',*,*,#9340,.F.);
#13147=ORIENTED_EDGE('',*,*,#9337,.F.);
#13148=ORIENTED_EDGE('',*,*,#9334,.F.);
#13149=ORIENTED_EDGE('',*,*,#9639,.F.);
#13150=ORIENTED_EDGE('',*,*,#9640,.T.);
#13151=ORIENTED_EDGE('',*,*,#9428,.T.);
#13152=ORIENTED_EDGE('',*,*,#9425,.T.);
#13153=ORIENTED_EDGE('',*,*,#9422,.T.);
#13154=ORIENTED_EDGE('',*,*,#9419,.T.);
#13155=ORIENTED_EDGE('',*,*,#9416,.T.);
#13156=ORIENTED_EDGE('',*,*,#9413,.T.);
#13157=ORIENTED_EDGE('',*,*,#9410,.T.);
#13158=ORIENTED_EDGE('',*,*,#9407,.T.);
#13159=ORIENTED_EDGE('',*,*,#9404,.T.);
#13160=ORIENTED_EDGE('',*,*,#9401,.T.);
#13161=ORIENTED_EDGE('',*,*,#9398,.T.);
#13162=ORIENTED_EDGE('',*,*,#9395,.T.);
#13163=ORIENTED_EDGE('',*,*,#9392,.T.);
#13164=ORIENTED_EDGE('',*,*,#9389,.T.);
#13165=ORIENTED_EDGE('',*,*,#9386,.T.);
#13166=ORIENTED_EDGE('',*,*,#9383,.T.);
#13167=ORIENTED_EDGE('',*,*,#9330,.F.);
#13168=ORIENTED_EDGE('',*,*,#9641,.T.);
#13169=ORIENTED_EDGE('',*,*,#9642,.T.);
#13170=ORIENTED_EDGE('',*,*,#9639,.T.);
#13171=ORIENTED_EDGE('',*,*,#9333,.F.);
#13172=ORIENTED_EDGE('',*,*,#9426,.T.);
#13173=ORIENTED_EDGE('',*,*,#9640,.F.);
#13174=ORIENTED_EDGE('',*,*,#9642,.F.);
#13175=ORIENTED_EDGE('',*,*,#9643,.T.);
#13176=ORIENTED_EDGE('',*,*,#9634,.F.);
#13177=ORIENTED_EDGE('',*,*,#9381,.F.);
#13178=ORIENTED_EDGE('',*,*,#9385,.F.);
#13179=ORIENTED_EDGE('',*,*,#9388,.F.);
#13180=ORIENTED_EDGE('',*,*,#9391,.F.);
#13181=ORIENTED_EDGE('',*,*,#9394,.F.);
#13182=ORIENTED_EDGE('',*,*,#9397,.F.);
#13183=ORIENTED_EDGE('',*,*,#9400,.F.);
#13184=ORIENTED_EDGE('',*,*,#9403,.F.);
#13185=ORIENTED_EDGE('',*,*,#9406,.F.);
#13186=ORIENTED_EDGE('',*,*,#9409,.F.);
#13187=ORIENTED_EDGE('',*,*,#9412,.F.);
#13188=ORIENTED_EDGE('',*,*,#9415,.F.);
#13189=ORIENTED_EDGE('',*,*,#9418,.F.);
#13190=ORIENTED_EDGE('',*,*,#9421,.F.);
#13191=ORIENTED_EDGE('',*,*,#9424,.F.);
#13192=ORIENTED_EDGE('',*,*,#9427,.F.);
#13193=ORIENTED_EDGE('',*,*,#9643,.F.);
#13194=ORIENTED_EDGE('',*,*,#9641,.F.);
#13195=ORIENTED_EDGE('',*,*,#9329,.F.);
#13196=ORIENTED_EDGE('',*,*,#9336,.F.);
#13197=ORIENTED_EDGE('',*,*,#9339,.F.);
#13198=ORIENTED_EDGE('',*,*,#9342,.F.);
#13199=ORIENTED_EDGE('',*,*,#9345,.F.);
#13200=ORIENTED_EDGE('',*,*,#9348,.F.);
#13201=ORIENTED_EDGE('',*,*,#9351,.F.);
#13202=ORIENTED_EDGE('',*,*,#9354,.F.);
#13203=ORIENTED_EDGE('',*,*,#9357,.F.);
#13204=ORIENTED_EDGE('',*,*,#9360,.F.);
#13205=ORIENTED_EDGE('',*,*,#9363,.F.);
#13206=ORIENTED_EDGE('',*,*,#9366,.F.);
#13207=ORIENTED_EDGE('',*,*,#9369,.F.);
#13208=ORIENTED_EDGE('',*,*,#9372,.F.);
#13209=ORIENTED_EDGE('',*,*,#9375,.F.);
#13210=ORIENTED_EDGE('',*,*,#9378,.F.);
#13211=ORIENTED_EDGE('',*,*,#9644,.F.);
#13212=ORIENTED_EDGE('',*,*,#9377,.T.);
#13213=ORIENTED_EDGE('',*,*,#9638,.T.);
#13214=ORIENTED_EDGE('',*,*,#9645,.F.);
#13215=ORIENTED_EDGE('',*,*,#9644,.T.);
#13216=ORIENTED_EDGE('',*,*,#9646,.T.);
#13217=ORIENTED_EDGE('',*,*,#9647,.F.);
#13218=ORIENTED_EDGE('',*,*,#9648,.F.);
#13219=ORIENTED_EDGE('',*,*,#9649,.F.);
#13220=ORIENTED_EDGE('',*,*,#9650,.F.);
#13221=ORIENTED_EDGE('',*,*,#9649,.T.);
#13222=ORIENTED_EDGE('',*,*,#9651,.T.);
#13223=ORIENTED_EDGE('',*,*,#9652,.T.);
#13224=ORIENTED_EDGE('',*,*,#9653,.F.);
#13225=ORIENTED_EDGE('',*,*,#9654,.F.);
#13226=ORIENTED_EDGE('',*,*,#9648,.T.);
#13227=ORIENTED_EDGE('',*,*,#9655,.T.);
#13228=ORIENTED_EDGE('',*,*,#9656,.T.);
#13229=ORIENTED_EDGE('',*,*,#9651,.F.);
#13230=ORIENTED_EDGE('',*,*,#9657,.F.);
#13231=ORIENTED_EDGE('',*,*,#9658,.F.);
#13232=ORIENTED_EDGE('',*,*,#9659,.F.);
#13233=ORIENTED_EDGE('',*,*,#9660,.T.);
#13234=ORIENTED_EDGE('',*,*,#9655,.F.);
#13235=ORIENTED_EDGE('',*,*,#9647,.T.);
#13236=ORIENTED_EDGE('',*,*,#9661,.F.);
#13237=ORIENTED_EDGE('',*,*,#9652,.F.);
#13238=ORIENTED_EDGE('',*,*,#9656,.F.);
#13239=ORIENTED_EDGE('',*,*,#9660,.F.);
#13240=ORIENTED_EDGE('',*,*,#9650,.T.);
#13241=ORIENTED_EDGE('',*,*,#9662,.F.);
#13242=ORIENTED_EDGE('',*,*,#9663,.T.);
#13243=ORIENTED_EDGE('',*,*,#9664,.T.);
#13244=ORIENTED_EDGE('',*,*,#9657,.T.);
#13245=ORIENTED_EDGE('',*,*,#9665,.T.);
#13246=ORIENTED_EDGE('',*,*,#9666,.T.);
#13247=ORIENTED_EDGE('',*,*,#9667,.F.);
#13248=ORIENTED_EDGE('',*,*,#9654,.T.);
#13249=ORIENTED_EDGE('',*,*,#9668,.F.);
#13250=ORIENTED_EDGE('',*,*,#9669,.T.);
#13251=ORIENTED_EDGE('',*,*,#9662,.T.);
#13252=ORIENTED_EDGE('',*,*,#9653,.T.);
#13253=ORIENTED_EDGE('',*,*,#9670,.F.);
#13254=ORIENTED_EDGE('',*,*,#9671,.T.);
#13255=ORIENTED_EDGE('',*,*,#9668,.T.);
#13256=ORIENTED_EDGE('',*,*,#9672,.T.);
#13257=ORIENTED_EDGE('',*,*,#9673,.F.);
#13258=ORIENTED_EDGE('',*,*,#9674,.F.);
#13259=ORIENTED_EDGE('',*,*,#9675,.F.);
#13260=ORIENTED_EDGE('',*,*,#9676,.F.);
#13261=ORIENTED_EDGE('',*,*,#9675,.T.);
#13262=ORIENTED_EDGE('',*,*,#9677,.T.);
#13263=ORIENTED_EDGE('',*,*,#9678,.T.);
#13264=ORIENTED_EDGE('',*,*,#9679,.F.);
#13265=ORIENTED_EDGE('',*,*,#9680,.F.);
#13266=ORIENTED_EDGE('',*,*,#9674,.T.);
#13267=ORIENTED_EDGE('',*,*,#9681,.T.);
#13268=ORIENTED_EDGE('',*,*,#9682,.T.);
#13269=ORIENTED_EDGE('',*,*,#9677,.F.);
#13270=ORIENTED_EDGE('',*,*,#9663,.F.);
#13271=ORIENTED_EDGE('',*,*,#9669,.F.);
#13272=ORIENTED_EDGE('',*,*,#9671,.F.);
#13273=ORIENTED_EDGE('',*,*,#9683,.T.);
#13274=ORIENTED_EDGE('',*,*,#9681,.F.);
#13275=ORIENTED_EDGE('',*,*,#9673,.T.);
#13276=ORIENTED_EDGE('',*,*,#9684,.F.);
#13277=ORIENTED_EDGE('',*,*,#9678,.F.);
#13278=ORIENTED_EDGE('',*,*,#9682,.F.);
#13279=ORIENTED_EDGE('',*,*,#9683,.F.);
#13280=ORIENTED_EDGE('',*,*,#9676,.T.);
#13281=ORIENTED_EDGE('',*,*,#9685,.F.);
#13282=ORIENTED_EDGE('',*,*,#9686,.T.);
#13283=ORIENTED_EDGE('',*,*,#9687,.T.);
#13284=ORIENTED_EDGE('',*,*,#9680,.T.);
#13285=ORIENTED_EDGE('',*,*,#9688,.F.);
#13286=ORIENTED_EDGE('',*,*,#9689,.T.);
#13287=ORIENTED_EDGE('',*,*,#9685,.T.);
#13288=ORIENTED_EDGE('',*,*,#9679,.T.);
#13289=ORIENTED_EDGE('',*,*,#9690,.F.);
#13290=ORIENTED_EDGE('',*,*,#9691,.T.);
#13291=ORIENTED_EDGE('',*,*,#9688,.T.);
#13292=ORIENTED_EDGE('',*,*,#9692,.T.);
#13293=ORIENTED_EDGE('',*,*,#9693,.F.);
#13294=ORIENTED_EDGE('',*,*,#9694,.F.);
#13295=ORIENTED_EDGE('',*,*,#9695,.F.);
#13296=ORIENTED_EDGE('',*,*,#9696,.F.);
#13297=ORIENTED_EDGE('',*,*,#9695,.T.);
#13298=ORIENTED_EDGE('',*,*,#9697,.T.);
#13299=ORIENTED_EDGE('',*,*,#9698,.T.);
#13300=ORIENTED_EDGE('',*,*,#9699,.F.);
#13301=ORIENTED_EDGE('',*,*,#9700,.F.);
#13302=ORIENTED_EDGE('',*,*,#9694,.T.);
#13303=ORIENTED_EDGE('',*,*,#9701,.T.);
#13304=ORIENTED_EDGE('',*,*,#9702,.T.);
#13305=ORIENTED_EDGE('',*,*,#9697,.F.);
#13306=ORIENTED_EDGE('',*,*,#9686,.F.);
#13307=ORIENTED_EDGE('',*,*,#9689,.F.);
#13308=ORIENTED_EDGE('',*,*,#9691,.F.);
#13309=ORIENTED_EDGE('',*,*,#9703,.T.);
#13310=ORIENTED_EDGE('',*,*,#9701,.F.);
#13311=ORIENTED_EDGE('',*,*,#9693,.T.);
#13312=ORIENTED_EDGE('',*,*,#9704,.F.);
#13313=ORIENTED_EDGE('',*,*,#9698,.F.);
#13314=ORIENTED_EDGE('',*,*,#9702,.F.);
#13315=ORIENTED_EDGE('',*,*,#9703,.F.);
#13316=ORIENTED_EDGE('',*,*,#9696,.T.);
#13317=ORIENTED_EDGE('',*,*,#9705,.F.);
#13318=ORIENTED_EDGE('',*,*,#9706,.T.);
#13319=ORIENTED_EDGE('',*,*,#9707,.T.);
#13320=ORIENTED_EDGE('',*,*,#9700,.T.);
#13321=ORIENTED_EDGE('',*,*,#9708,.F.);
#13322=ORIENTED_EDGE('',*,*,#9709,.T.);
#13323=ORIENTED_EDGE('',*,*,#9705,.T.);
#13324=ORIENTED_EDGE('',*,*,#9699,.T.);
#13325=ORIENTED_EDGE('',*,*,#9710,.F.);
#13326=ORIENTED_EDGE('',*,*,#9711,.T.);
#13327=ORIENTED_EDGE('',*,*,#9708,.T.);
#13328=ORIENTED_EDGE('',*,*,#9712,.T.);
#13329=ORIENTED_EDGE('',*,*,#9713,.F.);
#13330=ORIENTED_EDGE('',*,*,#9714,.F.);
#13331=ORIENTED_EDGE('',*,*,#9715,.F.);
#13332=ORIENTED_EDGE('',*,*,#9716,.F.);
#13333=ORIENTED_EDGE('',*,*,#9715,.T.);
#13334=ORIENTED_EDGE('',*,*,#9717,.T.);
#13335=ORIENTED_EDGE('',*,*,#9718,.T.);
#13336=ORIENTED_EDGE('',*,*,#9719,.F.);
#13337=ORIENTED_EDGE('',*,*,#9720,.F.);
#13338=ORIENTED_EDGE('',*,*,#9714,.T.);
#13339=ORIENTED_EDGE('',*,*,#9721,.T.);
#13340=ORIENTED_EDGE('',*,*,#9722,.T.);
#13341=ORIENTED_EDGE('',*,*,#9717,.F.);
#13342=ORIENTED_EDGE('',*,*,#9706,.F.);
#13343=ORIENTED_EDGE('',*,*,#9709,.F.);
#13344=ORIENTED_EDGE('',*,*,#9711,.F.);
#13345=ORIENTED_EDGE('',*,*,#9723,.T.);
#13346=ORIENTED_EDGE('',*,*,#9721,.F.);
#13347=ORIENTED_EDGE('',*,*,#9713,.T.);
#13348=ORIENTED_EDGE('',*,*,#9724,.F.);
#13349=ORIENTED_EDGE('',*,*,#9718,.F.);
#13350=ORIENTED_EDGE('',*,*,#9722,.F.);
#13351=ORIENTED_EDGE('',*,*,#9723,.F.);
#13352=ORIENTED_EDGE('',*,*,#9716,.T.);
#13353=ORIENTED_EDGE('',*,*,#9725,.F.);
#13354=ORIENTED_EDGE('',*,*,#9726,.T.);
#13355=ORIENTED_EDGE('',*,*,#9727,.T.);
#13356=ORIENTED_EDGE('',*,*,#9720,.T.);
#13357=ORIENTED_EDGE('',*,*,#9728,.F.);
#13358=ORIENTED_EDGE('',*,*,#9729,.T.);
#13359=ORIENTED_EDGE('',*,*,#9725,.T.);
#13360=ORIENTED_EDGE('',*,*,#9719,.T.);
#13361=ORIENTED_EDGE('',*,*,#9730,.F.);
#13362=ORIENTED_EDGE('',*,*,#9731,.T.);
#13363=ORIENTED_EDGE('',*,*,#9728,.T.);
#13364=ORIENTED_EDGE('',*,*,#9732,.T.);
#13365=ORIENTED_EDGE('',*,*,#9733,.F.);
#13366=ORIENTED_EDGE('',*,*,#9734,.F.);
#13367=ORIENTED_EDGE('',*,*,#9735,.F.);
#13368=ORIENTED_EDGE('',*,*,#9736,.F.);
#13369=ORIENTED_EDGE('',*,*,#9735,.T.);
#13370=ORIENTED_EDGE('',*,*,#9737,.T.);
#13371=ORIENTED_EDGE('',*,*,#9738,.T.);
#13372=ORIENTED_EDGE('',*,*,#9739,.F.);
#13373=ORIENTED_EDGE('',*,*,#9740,.F.);
#13374=ORIENTED_EDGE('',*,*,#9734,.T.);
#13375=ORIENTED_EDGE('',*,*,#9741,.T.);
#13376=ORIENTED_EDGE('',*,*,#9742,.T.);
#13377=ORIENTED_EDGE('',*,*,#9737,.F.);
#13378=ORIENTED_EDGE('',*,*,#9726,.F.);
#13379=ORIENTED_EDGE('',*,*,#9729,.F.);
#13380=ORIENTED_EDGE('',*,*,#9731,.F.);
#13381=ORIENTED_EDGE('',*,*,#9743,.T.);
#13382=ORIENTED_EDGE('',*,*,#9741,.F.);
#13383=ORIENTED_EDGE('',*,*,#9733,.T.);
#13384=ORIENTED_EDGE('',*,*,#9744,.F.);
#13385=ORIENTED_EDGE('',*,*,#9738,.F.);
#13386=ORIENTED_EDGE('',*,*,#9742,.F.);
#13387=ORIENTED_EDGE('',*,*,#9743,.F.);
#13388=ORIENTED_EDGE('',*,*,#9736,.T.);
#13389=ORIENTED_EDGE('',*,*,#9745,.F.);
#13390=ORIENTED_EDGE('',*,*,#9746,.T.);
#13391=ORIENTED_EDGE('',*,*,#9747,.T.);
#13392=ORIENTED_EDGE('',*,*,#9740,.T.);
#13393=ORIENTED_EDGE('',*,*,#9748,.F.);
#13394=ORIENTED_EDGE('',*,*,#9749,.T.);
#13395=ORIENTED_EDGE('',*,*,#9745,.T.);
#13396=ORIENTED_EDGE('',*,*,#9739,.T.);
#13397=ORIENTED_EDGE('',*,*,#9750,.F.);
#13398=ORIENTED_EDGE('',*,*,#9751,.T.);
#13399=ORIENTED_EDGE('',*,*,#9748,.T.);
#13400=ORIENTED_EDGE('',*,*,#9752,.T.);
#13401=ORIENTED_EDGE('',*,*,#9753,.F.);
#13402=ORIENTED_EDGE('',*,*,#9754,.F.);
#13403=ORIENTED_EDGE('',*,*,#9755,.F.);
#13404=ORIENTED_EDGE('',*,*,#9756,.F.);
#13405=ORIENTED_EDGE('',*,*,#9755,.T.);
#13406=ORIENTED_EDGE('',*,*,#9757,.T.);
#13407=ORIENTED_EDGE('',*,*,#9758,.T.);
#13408=ORIENTED_EDGE('',*,*,#9759,.F.);
#13409=ORIENTED_EDGE('',*,*,#9760,.F.);
#13410=ORIENTED_EDGE('',*,*,#9754,.T.);
#13411=ORIENTED_EDGE('',*,*,#9761,.T.);
#13412=ORIENTED_EDGE('',*,*,#9762,.T.);
#13413=ORIENTED_EDGE('',*,*,#9757,.F.);
#13414=ORIENTED_EDGE('',*,*,#9746,.F.);
#13415=ORIENTED_EDGE('',*,*,#9749,.F.);
#13416=ORIENTED_EDGE('',*,*,#9751,.F.);
#13417=ORIENTED_EDGE('',*,*,#9763,.T.);
#13418=ORIENTED_EDGE('',*,*,#9761,.F.);
#13419=ORIENTED_EDGE('',*,*,#9753,.T.);
#13420=ORIENTED_EDGE('',*,*,#9764,.F.);
#13421=ORIENTED_EDGE('',*,*,#9758,.F.);
#13422=ORIENTED_EDGE('',*,*,#9762,.F.);
#13423=ORIENTED_EDGE('',*,*,#9763,.F.);
#13424=ORIENTED_EDGE('',*,*,#9756,.T.);
#13425=ORIENTED_EDGE('',*,*,#9765,.F.);
#13426=ORIENTED_EDGE('',*,*,#9766,.T.);
#13427=ORIENTED_EDGE('',*,*,#9767,.T.);
#13428=ORIENTED_EDGE('',*,*,#9760,.T.);
#13429=ORIENTED_EDGE('',*,*,#9768,.F.);
#13430=ORIENTED_EDGE('',*,*,#9769,.T.);
#13431=ORIENTED_EDGE('',*,*,#9765,.T.);
#13432=ORIENTED_EDGE('',*,*,#9759,.T.);
#13433=ORIENTED_EDGE('',*,*,#9770,.F.);
#13434=ORIENTED_EDGE('',*,*,#9771,.T.);
#13435=ORIENTED_EDGE('',*,*,#9768,.T.);
#13436=ORIENTED_EDGE('',*,*,#9772,.T.);
#13437=ORIENTED_EDGE('',*,*,#9773,.F.);
#13438=ORIENTED_EDGE('',*,*,#9774,.F.);
#13439=ORIENTED_EDGE('',*,*,#9775,.F.);
#13440=ORIENTED_EDGE('',*,*,#9776,.F.);
#13441=ORIENTED_EDGE('',*,*,#9775,.T.);
#13442=ORIENTED_EDGE('',*,*,#9777,.T.);
#13443=ORIENTED_EDGE('',*,*,#9778,.T.);
#13444=ORIENTED_EDGE('',*,*,#9779,.F.);
#13445=ORIENTED_EDGE('',*,*,#9780,.F.);
#13446=ORIENTED_EDGE('',*,*,#9774,.T.);
#13447=ORIENTED_EDGE('',*,*,#9781,.T.);
#13448=ORIENTED_EDGE('',*,*,#9782,.T.);
#13449=ORIENTED_EDGE('',*,*,#9777,.F.);
#13450=ORIENTED_EDGE('',*,*,#9766,.F.);
#13451=ORIENTED_EDGE('',*,*,#9769,.F.);
#13452=ORIENTED_EDGE('',*,*,#9771,.F.);
#13453=ORIENTED_EDGE('',*,*,#9783,.T.);
#13454=ORIENTED_EDGE('',*,*,#9781,.F.);
#13455=ORIENTED_EDGE('',*,*,#9773,.T.);
#13456=ORIENTED_EDGE('',*,*,#9784,.F.);
#13457=ORIENTED_EDGE('',*,*,#9778,.F.);
#13458=ORIENTED_EDGE('',*,*,#9782,.F.);
#13459=ORIENTED_EDGE('',*,*,#9783,.F.);
#13460=ORIENTED_EDGE('',*,*,#9776,.T.);
#13461=ORIENTED_EDGE('',*,*,#9785,.F.);
#13462=ORIENTED_EDGE('',*,*,#9786,.T.);
#13463=ORIENTED_EDGE('',*,*,#9787,.T.);
#13464=ORIENTED_EDGE('',*,*,#9780,.T.);
#13465=ORIENTED_EDGE('',*,*,#9788,.F.);
#13466=ORIENTED_EDGE('',*,*,#9789,.T.);
#13467=ORIENTED_EDGE('',*,*,#9785,.T.);
#13468=ORIENTED_EDGE('',*,*,#9779,.T.);
#13469=ORIENTED_EDGE('',*,*,#9790,.F.);
#13470=ORIENTED_EDGE('',*,*,#9791,.T.);
#13471=ORIENTED_EDGE('',*,*,#9788,.T.);
#13472=ORIENTED_EDGE('',*,*,#9792,.T.);
#13473=ORIENTED_EDGE('',*,*,#9793,.T.);
#13474=ORIENTED_EDGE('',*,*,#9794,.F.);
#13475=ORIENTED_EDGE('',*,*,#9795,.F.);
#13476=ORIENTED_EDGE('',*,*,#9796,.F.);
#13477=ORIENTED_EDGE('',*,*,#9797,.F.);
#13478=ORIENTED_EDGE('',*,*,#9796,.T.);
#13479=ORIENTED_EDGE('',*,*,#9798,.T.);
#13480=ORIENTED_EDGE('',*,*,#9799,.T.);
#13481=ORIENTED_EDGE('',*,*,#9800,.F.);
#13482=ORIENTED_EDGE('',*,*,#9801,.F.);
#13483=ORIENTED_EDGE('',*,*,#9795,.T.);
#13484=ORIENTED_EDGE('',*,*,#9802,.T.);
#13485=ORIENTED_EDGE('',*,*,#9803,.T.);
#13486=ORIENTED_EDGE('',*,*,#9798,.F.);
#13487=ORIENTED_EDGE('',*,*,#9786,.F.);
#13488=ORIENTED_EDGE('',*,*,#9789,.F.);
#13489=ORIENTED_EDGE('',*,*,#9791,.F.);
#13490=ORIENTED_EDGE('',*,*,#9804,.T.);
#13491=ORIENTED_EDGE('',*,*,#9802,.F.);
#13492=ORIENTED_EDGE('',*,*,#9794,.T.);
#13493=ORIENTED_EDGE('',*,*,#9805,.F.);
#13494=ORIENTED_EDGE('',*,*,#9799,.F.);
#13495=ORIENTED_EDGE('',*,*,#9803,.F.);
#13496=ORIENTED_EDGE('',*,*,#9804,.F.);
#13497=ORIENTED_EDGE('',*,*,#9806,.F.);
#13498=ORIENTED_EDGE('',*,*,#9797,.T.);
#13499=ORIENTED_EDGE('',*,*,#9807,.F.);
#13500=ORIENTED_EDGE('',*,*,#9808,.T.);
#13501=ORIENTED_EDGE('',*,*,#9809,.T.);
#13502=ORIENTED_EDGE('',*,*,#9801,.T.);
#13503=ORIENTED_EDGE('',*,*,#9810,.F.);
#13504=ORIENTED_EDGE('',*,*,#9811,.T.);
#13505=ORIENTED_EDGE('',*,*,#9807,.T.);
#13506=ORIENTED_EDGE('',*,*,#9800,.T.);
#13507=ORIENTED_EDGE('',*,*,#9812,.F.);
#13508=ORIENTED_EDGE('',*,*,#9813,.T.);
#13509=ORIENTED_EDGE('',*,*,#9810,.T.);
#13510=ORIENTED_EDGE('',*,*,#9814,.T.);
#13511=ORIENTED_EDGE('',*,*,#9815,.F.);
#13512=ORIENTED_EDGE('',*,*,#9816,.F.);
#13513=ORIENTED_EDGE('',*,*,#9817,.F.);
#13514=ORIENTED_EDGE('',*,*,#9818,.F.);
#13515=ORIENTED_EDGE('',*,*,#9817,.T.);
#13516=ORIENTED_EDGE('',*,*,#9819,.T.);
#13517=ORIENTED_EDGE('',*,*,#9820,.T.);
#13518=ORIENTED_EDGE('',*,*,#9821,.F.);
#13519=ORIENTED_EDGE('',*,*,#9822,.F.);
#13520=ORIENTED_EDGE('',*,*,#9816,.T.);
#13521=ORIENTED_EDGE('',*,*,#9823,.T.);
#13522=ORIENTED_EDGE('',*,*,#9824,.T.);
#13523=ORIENTED_EDGE('',*,*,#9819,.F.);
#13524=ORIENTED_EDGE('',*,*,#9808,.F.);
#13525=ORIENTED_EDGE('',*,*,#9811,.F.);
#13526=ORIENTED_EDGE('',*,*,#9813,.F.);
#13527=ORIENTED_EDGE('',*,*,#9825,.T.);
#13528=ORIENTED_EDGE('',*,*,#9823,.F.);
#13529=ORIENTED_EDGE('',*,*,#9815,.T.);
#13530=ORIENTED_EDGE('',*,*,#9826,.F.);
#13531=ORIENTED_EDGE('',*,*,#9820,.F.);
#13532=ORIENTED_EDGE('',*,*,#9824,.F.);
#13533=ORIENTED_EDGE('',*,*,#9825,.F.);
#13534=ORIENTED_EDGE('',*,*,#9818,.T.);
#13535=ORIENTED_EDGE('',*,*,#9827,.F.);
#13536=ORIENTED_EDGE('',*,*,#9828,.T.);
#13537=ORIENTED_EDGE('',*,*,#9829,.T.);
#13538=ORIENTED_EDGE('',*,*,#9822,.T.);
#13539=ORIENTED_EDGE('',*,*,#9830,.F.);
#13540=ORIENTED_EDGE('',*,*,#9831,.T.);
#13541=ORIENTED_EDGE('',*,*,#9827,.T.);
#13542=ORIENTED_EDGE('',*,*,#9821,.T.);
#13543=ORIENTED_EDGE('',*,*,#9832,.F.);
#13544=ORIENTED_EDGE('',*,*,#9833,.T.);
#13545=ORIENTED_EDGE('',*,*,#9830,.T.);
#13546=ORIENTED_EDGE('',*,*,#9834,.T.);
#13547=ORIENTED_EDGE('',*,*,#9835,.F.);
#13548=ORIENTED_EDGE('',*,*,#9836,.F.);
#13549=ORIENTED_EDGE('',*,*,#9837,.F.);
#13550=ORIENTED_EDGE('',*,*,#9838,.F.);
#13551=ORIENTED_EDGE('',*,*,#9837,.T.);
#13552=ORIENTED_EDGE('',*,*,#9839,.T.);
#13553=ORIENTED_EDGE('',*,*,#9840,.T.);
#13554=ORIENTED_EDGE('',*,*,#9841,.F.);
#13555=ORIENTED_EDGE('',*,*,#9842,.F.);
#13556=ORIENTED_EDGE('',*,*,#9836,.T.);
#13557=ORIENTED_EDGE('',*,*,#9843,.T.);
#13558=ORIENTED_EDGE('',*,*,#9844,.T.);
#13559=ORIENTED_EDGE('',*,*,#9839,.F.);
#13560=ORIENTED_EDGE('',*,*,#9828,.F.);
#13561=ORIENTED_EDGE('',*,*,#9831,.F.);
#13562=ORIENTED_EDGE('',*,*,#9833,.F.);
#13563=ORIENTED_EDGE('',*,*,#9845,.T.);
#13564=ORIENTED_EDGE('',*,*,#9843,.F.);
#13565=ORIENTED_EDGE('',*,*,#9835,.T.);
#13566=ORIENTED_EDGE('',*,*,#9846,.F.);
#13567=ORIENTED_EDGE('',*,*,#9840,.F.);
#13568=ORIENTED_EDGE('',*,*,#9844,.F.);
#13569=ORIENTED_EDGE('',*,*,#9845,.F.);
#13570=ORIENTED_EDGE('',*,*,#9838,.T.);
#13571=ORIENTED_EDGE('',*,*,#9847,.F.);
#13572=ORIENTED_EDGE('',*,*,#9848,.T.);
#13573=ORIENTED_EDGE('',*,*,#9849,.T.);
#13574=ORIENTED_EDGE('',*,*,#9842,.T.);
#13575=ORIENTED_EDGE('',*,*,#9850,.F.);
#13576=ORIENTED_EDGE('',*,*,#9851,.T.);
#13577=ORIENTED_EDGE('',*,*,#9847,.T.);
#13578=ORIENTED_EDGE('',*,*,#9841,.T.);
#13579=ORIENTED_EDGE('',*,*,#9852,.F.);
#13580=ORIENTED_EDGE('',*,*,#9853,.T.);
#13581=ORIENTED_EDGE('',*,*,#9850,.T.);
#13582=ORIENTED_EDGE('',*,*,#9854,.T.);
#13583=ORIENTED_EDGE('',*,*,#9855,.F.);
#13584=ORIENTED_EDGE('',*,*,#9856,.F.);
#13585=ORIENTED_EDGE('',*,*,#9857,.F.);
#13586=ORIENTED_EDGE('',*,*,#9858,.F.);
#13587=ORIENTED_EDGE('',*,*,#9857,.T.);
#13588=ORIENTED_EDGE('',*,*,#9859,.T.);
#13589=ORIENTED_EDGE('',*,*,#9860,.T.);
#13590=ORIENTED_EDGE('',*,*,#9861,.F.);
#13591=ORIENTED_EDGE('',*,*,#9862,.F.);
#13592=ORIENTED_EDGE('',*,*,#9856,.T.);
#13593=ORIENTED_EDGE('',*,*,#9863,.T.);
#13594=ORIENTED_EDGE('',*,*,#9864,.T.);
#13595=ORIENTED_EDGE('',*,*,#9859,.F.);
#13596=ORIENTED_EDGE('',*,*,#9848,.F.);
#13597=ORIENTED_EDGE('',*,*,#9851,.F.);
#13598=ORIENTED_EDGE('',*,*,#9853,.F.);
#13599=ORIENTED_EDGE('',*,*,#9865,.T.);
#13600=ORIENTED_EDGE('',*,*,#9863,.F.);
#13601=ORIENTED_EDGE('',*,*,#9855,.T.);
#13602=ORIENTED_EDGE('',*,*,#9866,.F.);
#13603=ORIENTED_EDGE('',*,*,#9860,.F.);
#13604=ORIENTED_EDGE('',*,*,#9864,.F.);
#13605=ORIENTED_EDGE('',*,*,#9865,.F.);
#13606=ORIENTED_EDGE('',*,*,#9858,.T.);
#13607=ORIENTED_EDGE('',*,*,#9867,.F.);
#13608=ORIENTED_EDGE('',*,*,#9868,.T.);
#13609=ORIENTED_EDGE('',*,*,#9869,.T.);
#13610=ORIENTED_EDGE('',*,*,#9862,.T.);
#13611=ORIENTED_EDGE('',*,*,#9870,.F.);
#13612=ORIENTED_EDGE('',*,*,#9871,.T.);
#13613=ORIENTED_EDGE('',*,*,#9867,.T.);
#13614=ORIENTED_EDGE('',*,*,#9861,.T.);
#13615=ORIENTED_EDGE('',*,*,#9872,.F.);
#13616=ORIENTED_EDGE('',*,*,#9873,.T.);
#13617=ORIENTED_EDGE('',*,*,#9870,.T.);
#13618=ORIENTED_EDGE('',*,*,#9874,.T.);
#13619=ORIENTED_EDGE('',*,*,#9875,.F.);
#13620=ORIENTED_EDGE('',*,*,#9876,.F.);
#13621=ORIENTED_EDGE('',*,*,#9877,.F.);
#13622=ORIENTED_EDGE('',*,*,#9878,.F.);
#13623=ORIENTED_EDGE('',*,*,#9877,.T.);
#13624=ORIENTED_EDGE('',*,*,#9879,.T.);
#13625=ORIENTED_EDGE('',*,*,#9880,.T.);
#13626=ORIENTED_EDGE('',*,*,#9881,.F.);
#13627=ORIENTED_EDGE('',*,*,#9882,.F.);
#13628=ORIENTED_EDGE('',*,*,#9876,.T.);
#13629=ORIENTED_EDGE('',*,*,#9883,.T.);
#13630=ORIENTED_EDGE('',*,*,#9884,.T.);
#13631=ORIENTED_EDGE('',*,*,#9879,.F.);
#13632=ORIENTED_EDGE('',*,*,#9868,.F.);
#13633=ORIENTED_EDGE('',*,*,#9871,.F.);
#13634=ORIENTED_EDGE('',*,*,#9873,.F.);
#13635=ORIENTED_EDGE('',*,*,#9885,.T.);
#13636=ORIENTED_EDGE('',*,*,#9883,.F.);
#13637=ORIENTED_EDGE('',*,*,#9875,.T.);
#13638=ORIENTED_EDGE('',*,*,#9886,.F.);
#13639=ORIENTED_EDGE('',*,*,#9880,.F.);
#13640=ORIENTED_EDGE('',*,*,#9884,.F.);
#13641=ORIENTED_EDGE('',*,*,#9885,.F.);
#13642=ORIENTED_EDGE('',*,*,#9878,.T.);
#13643=ORIENTED_EDGE('',*,*,#9887,.F.);
#13644=ORIENTED_EDGE('',*,*,#9888,.T.);
#13645=ORIENTED_EDGE('',*,*,#9889,.T.);
#13646=ORIENTED_EDGE('',*,*,#9882,.T.);
#13647=ORIENTED_EDGE('',*,*,#9890,.F.);
#13648=ORIENTED_EDGE('',*,*,#9891,.T.);
#13649=ORIENTED_EDGE('',*,*,#9887,.T.);
#13650=ORIENTED_EDGE('',*,*,#9881,.T.);
#13651=ORIENTED_EDGE('',*,*,#9892,.F.);
#13652=ORIENTED_EDGE('',*,*,#9893,.T.);
#13653=ORIENTED_EDGE('',*,*,#9890,.T.);
#13654=ORIENTED_EDGE('',*,*,#9894,.T.);
#13655=ORIENTED_EDGE('',*,*,#9895,.F.);
#13656=ORIENTED_EDGE('',*,*,#9896,.F.);
#13657=ORIENTED_EDGE('',*,*,#9897,.F.);
#13658=ORIENTED_EDGE('',*,*,#9898,.F.);
#13659=ORIENTED_EDGE('',*,*,#9897,.T.);
#13660=ORIENTED_EDGE('',*,*,#9899,.T.);
#13661=ORIENTED_EDGE('',*,*,#9900,.T.);
#13662=ORIENTED_EDGE('',*,*,#9901,.F.);
#13663=ORIENTED_EDGE('',*,*,#9902,.F.);
#13664=ORIENTED_EDGE('',*,*,#9896,.T.);
#13665=ORIENTED_EDGE('',*,*,#9903,.T.);
#13666=ORIENTED_EDGE('',*,*,#9904,.T.);
#13667=ORIENTED_EDGE('',*,*,#9899,.F.);
#13668=ORIENTED_EDGE('',*,*,#9888,.F.);
#13669=ORIENTED_EDGE('',*,*,#9891,.F.);
#13670=ORIENTED_EDGE('',*,*,#9893,.F.);
#13671=ORIENTED_EDGE('',*,*,#9905,.T.);
#13672=ORIENTED_EDGE('',*,*,#9903,.F.);
#13673=ORIENTED_EDGE('',*,*,#9895,.T.);
#13674=ORIENTED_EDGE('',*,*,#9906,.F.);
#13675=ORIENTED_EDGE('',*,*,#9900,.F.);
#13676=ORIENTED_EDGE('',*,*,#9904,.F.);
#13677=ORIENTED_EDGE('',*,*,#9905,.F.);
#13678=ORIENTED_EDGE('',*,*,#9898,.T.);
#13679=ORIENTED_EDGE('',*,*,#9907,.F.);
#13680=ORIENTED_EDGE('',*,*,#9908,.T.);
#13681=ORIENTED_EDGE('',*,*,#9909,.T.);
#13682=ORIENTED_EDGE('',*,*,#9902,.T.);
#13683=ORIENTED_EDGE('',*,*,#9910,.F.);
#13684=ORIENTED_EDGE('',*,*,#9911,.T.);
#13685=ORIENTED_EDGE('',*,*,#9907,.T.);
#13686=ORIENTED_EDGE('',*,*,#9901,.T.);
#13687=ORIENTED_EDGE('',*,*,#9912,.F.);
#13688=ORIENTED_EDGE('',*,*,#9913,.T.);
#13689=ORIENTED_EDGE('',*,*,#9910,.T.);
#13690=ORIENTED_EDGE('',*,*,#9914,.T.);
#13691=ORIENTED_EDGE('',*,*,#9915,.F.);
#13692=ORIENTED_EDGE('',*,*,#9916,.F.);
#13693=ORIENTED_EDGE('',*,*,#9917,.F.);
#13694=ORIENTED_EDGE('',*,*,#9918,.F.);
#13695=ORIENTED_EDGE('',*,*,#9917,.T.);
#13696=ORIENTED_EDGE('',*,*,#9919,.T.);
#13697=ORIENTED_EDGE('',*,*,#9920,.T.);
#13698=ORIENTED_EDGE('',*,*,#9921,.F.);
#13699=ORIENTED_EDGE('',*,*,#9922,.F.);
#13700=ORIENTED_EDGE('',*,*,#9916,.T.);
#13701=ORIENTED_EDGE('',*,*,#9923,.T.);
#13702=ORIENTED_EDGE('',*,*,#9924,.T.);
#13703=ORIENTED_EDGE('',*,*,#9919,.F.);
#13704=ORIENTED_EDGE('',*,*,#9908,.F.);
#13705=ORIENTED_EDGE('',*,*,#9911,.F.);
#13706=ORIENTED_EDGE('',*,*,#9913,.F.);
#13707=ORIENTED_EDGE('',*,*,#9925,.T.);
#13708=ORIENTED_EDGE('',*,*,#9923,.F.);
#13709=ORIENTED_EDGE('',*,*,#9915,.T.);
#13710=ORIENTED_EDGE('',*,*,#9926,.F.);
#13711=ORIENTED_EDGE('',*,*,#9920,.F.);
#13712=ORIENTED_EDGE('',*,*,#9924,.F.);
#13713=ORIENTED_EDGE('',*,*,#9925,.F.);
#13714=ORIENTED_EDGE('',*,*,#9918,.T.);
#13715=ORIENTED_EDGE('',*,*,#9927,.F.);
#13716=ORIENTED_EDGE('',*,*,#9928,.T.);
#13717=ORIENTED_EDGE('',*,*,#9929,.T.);
#13718=ORIENTED_EDGE('',*,*,#9922,.T.);
#13719=ORIENTED_EDGE('',*,*,#9930,.F.);
#13720=ORIENTED_EDGE('',*,*,#9931,.T.);
#13721=ORIENTED_EDGE('',*,*,#9927,.T.);
#13722=ORIENTED_EDGE('',*,*,#9921,.T.);
#13723=ORIENTED_EDGE('',*,*,#9932,.F.);
#13724=ORIENTED_EDGE('',*,*,#9933,.T.);
#13725=ORIENTED_EDGE('',*,*,#9930,.T.);
#13726=ORIENTED_EDGE('',*,*,#9933,.F.);
#13727=ORIENTED_EDGE('',*,*,#9934,.T.);
#13728=ORIENTED_EDGE('',*,*,#9935,.F.);
#13729=ORIENTED_EDGE('',*,*,#9936,.T.);
#13730=ORIENTED_EDGE('',*,*,#9928,.F.);
#13731=ORIENTED_EDGE('',*,*,#9931,.F.);
#13732=ORIENTED_EDGE('',*,*,#9937,.T.);
#13733=ORIENTED_EDGE('',*,*,#9936,.F.);
#13734=ORIENTED_EDGE('',*,*,#9938,.F.);
#13735=ORIENTED_EDGE('',*,*,#9939,.F.);
#13736=ORIENTED_EDGE('',*,*,#9938,.T.);
#13737=ORIENTED_EDGE('',*,*,#9935,.T.);
#13738=ORIENTED_EDGE('',*,*,#9940,.T.);
#13739=ORIENTED_EDGE('',*,*,#9941,.F.);
#13740=ORIENTED_EDGE('',*,*,#9942,.F.);
#13741=ORIENTED_EDGE('',*,*,#9943,.F.);
#13742=ORIENTED_EDGE('',*,*,#9666,.F.);
#13743=ORIENTED_EDGE('',*,*,#9939,.T.);
#13744=ORIENTED_EDGE('',*,*,#9941,.T.);
#13745=ORIENTED_EDGE('',*,*,#9944,.T.);
#13746=ORIENTED_EDGE('',*,*,#9945,.F.);
#13747=ORIENTED_EDGE('',*,*,#9944,.F.);
#13748=ORIENTED_EDGE('',*,*,#9940,.F.);
#13749=ORIENTED_EDGE('',*,*,#9934,.F.);
#13750=ORIENTED_EDGE('',*,*,#9659,.T.);
#13751=ORIENTED_EDGE('',*,*,#9946,.T.);
#13752=ORIENTED_EDGE('',*,*,#9942,.T.);
#13753=ORIENTED_EDGE('',*,*,#9947,.F.);
#13754=ORIENTED_EDGE('',*,*,#9658,.T.);
#13755=ORIENTED_EDGE('',*,*,#9667,.T.);
#13756=ORIENTED_EDGE('',*,*,#9943,.T.);
#13757=ORIENTED_EDGE('',*,*,#9946,.F.);
#13758=ORIENTED_EDGE('',*,*,#9948,.F.);
#13759=ORIENTED_EDGE('',*,*,#9332,.F.);
#13760=ORIENTED_EDGE('',*,*,#9949,.T.);
#13761=ORIENTED_EDGE('',*,*,#9948,.T.);
#13762=ORIENTED_EDGE('',*,*,#9949,.F.);
#13763=ORIENTED_EDGE('',*,*,#9929,.F.);
#13764=ORIENTED_EDGE('',*,*,#9937,.F.);
#13765=ORIENTED_EDGE('',*,*,#9665,.F.);
#13766=ORIENTED_EDGE('',*,*,#9646,.F.);
#13767=ORIENTED_EDGE('',*,*,#9664,.F.);
#13768=ORIENTED_EDGE('',*,*,#9672,.F.);
#13769=ORIENTED_EDGE('',*,*,#9687,.F.);
#13770=ORIENTED_EDGE('',*,*,#9692,.F.);
#13771=ORIENTED_EDGE('',*,*,#9707,.F.);
#13772=ORIENTED_EDGE('',*,*,#9712,.F.);
#13773=ORIENTED_EDGE('',*,*,#9727,.F.);
#13774=ORIENTED_EDGE('',*,*,#9732,.F.);
#13775=ORIENTED_EDGE('',*,*,#9747,.F.);
#13776=ORIENTED_EDGE('',*,*,#9752,.F.);
#13777=ORIENTED_EDGE('',*,*,#9767,.F.);
#13778=ORIENTED_EDGE('',*,*,#9772,.F.);
#13779=ORIENTED_EDGE('',*,*,#9787,.F.);
#13780=ORIENTED_EDGE('',*,*,#9793,.F.);
#13781=ORIENTED_EDGE('',*,*,#9950,.T.);
#13782=ORIENTED_EDGE('',*,*,#9635,.T.);
#13783=ORIENTED_EDGE('',*,*,#9645,.T.);
#13784=ORIENTED_EDGE('',*,*,#9636,.T.);
#13785=ORIENTED_EDGE('',*,*,#9950,.F.);
#13786=ORIENTED_EDGE('',*,*,#9792,.F.);
#13787=ORIENTED_EDGE('',*,*,#9809,.F.);
#13788=ORIENTED_EDGE('',*,*,#9814,.F.);
#13789=ORIENTED_EDGE('',*,*,#9829,.F.);
#13790=ORIENTED_EDGE('',*,*,#9834,.F.);
#13791=ORIENTED_EDGE('',*,*,#9849,.F.);
#13792=ORIENTED_EDGE('',*,*,#9854,.F.);
#13793=ORIENTED_EDGE('',*,*,#9869,.F.);
#13794=ORIENTED_EDGE('',*,*,#9874,.F.);
#13795=ORIENTED_EDGE('',*,*,#9889,.F.);
#13796=ORIENTED_EDGE('',*,*,#9894,.F.);
#13797=ORIENTED_EDGE('',*,*,#9909,.F.);
#13798=ORIENTED_EDGE('',*,*,#9914,.F.);
#13799=ORIENTED_EDGE('',*,*,#9135,.F.);
#13800=ORIENTED_EDGE('',*,*,#9951,.T.);
#13801=ORIENTED_EDGE('',*,*,#9806,.T.);
#13802=ORIENTED_EDGE('',*,*,#9790,.T.);
#13803=ORIENTED_EDGE('',*,*,#9784,.T.);
#13804=ORIENTED_EDGE('',*,*,#9770,.T.);
#13805=ORIENTED_EDGE('',*,*,#9764,.T.);
#13806=ORIENTED_EDGE('',*,*,#9750,.T.);
#13807=ORIENTED_EDGE('',*,*,#9744,.T.);
#13808=ORIENTED_EDGE('',*,*,#9730,.T.);
#13809=ORIENTED_EDGE('',*,*,#9724,.T.);
#13810=ORIENTED_EDGE('',*,*,#9710,.T.);
#13811=ORIENTED_EDGE('',*,*,#9704,.T.);
#13812=ORIENTED_EDGE('',*,*,#9690,.T.);
#13813=ORIENTED_EDGE('',*,*,#9684,.T.);
#13814=ORIENTED_EDGE('',*,*,#9670,.T.);
#13815=ORIENTED_EDGE('',*,*,#9661,.T.);
#13816=ORIENTED_EDGE('',*,*,#9947,.T.);
#13817=ORIENTED_EDGE('',*,*,#9945,.T.);
#13818=ORIENTED_EDGE('',*,*,#9932,.T.);
#13819=ORIENTED_EDGE('',*,*,#9926,.T.);
#13820=ORIENTED_EDGE('',*,*,#9912,.T.);
#13821=ORIENTED_EDGE('',*,*,#9906,.T.);
#13822=ORIENTED_EDGE('',*,*,#9892,.T.);
#13823=ORIENTED_EDGE('',*,*,#9886,.T.);
#13824=ORIENTED_EDGE('',*,*,#9872,.T.);
#13825=ORIENTED_EDGE('',*,*,#9866,.T.);
#13826=ORIENTED_EDGE('',*,*,#9852,.T.);
#13827=ORIENTED_EDGE('',*,*,#9846,.T.);
#13828=ORIENTED_EDGE('',*,*,#9832,.T.);
#13829=ORIENTED_EDGE('',*,*,#9826,.T.);
#13830=ORIENTED_EDGE('',*,*,#9812,.T.);
#13831=ORIENTED_EDGE('',*,*,#9805,.T.);
#13832=ORIENTED_EDGE('',*,*,#9951,.F.);
#13833=ORIENTED_EDGE('',*,*,#9325,.T.);
#13834=ORIENTED_EDGE('',*,*,#9627,.T.);
#13835=ORIENTED_EDGE('',*,*,#9952,.F.);
#13836=ORIENTED_EDGE('',*,*,#9633,.T.);
#13837=ORIENTED_EDGE('',*,*,#9953,.F.);
#13838=ORIENTED_EDGE('',*,*,#9954,.T.);
#13839=ORIENTED_EDGE('',*,*,#9624,.T.);
#13840=ORIENTED_EDGE('',*,*,#9952,.T.);
#13841=ORIENTED_EDGE('',*,*,#9625,.T.);
#13842=ORIENTED_EDGE('',*,*,#9954,.F.);
#13843=ORIENTED_EDGE('',*,*,#9953,.T.);
#18310=CYLINDRICAL_SURFACE('',#20143,6.933);
#18311=CYLINDRICAL_SURFACE('',#20153,6.933);
#18312=CYLINDRICAL_SURFACE('',#20154,6.933);
#18313=CYLINDRICAL_SURFACE('',#20155,6.933);
#18314=CYLINDRICAL_SURFACE('',#20156,6.933);
#18315=CYLINDRICAL_SURFACE('',#20157,6.933);
#18316=CYLINDRICAL_SURFACE('',#20158,6.933);
#18317=CYLINDRICAL_SURFACE('',#20159,6.933);
#18318=CYLINDRICAL_SURFACE('',#20160,6.933);
#18319=CYLINDRICAL_SURFACE('',#20161,6.933);
#18320=CYLINDRICAL_SURFACE('',#20162,6.933);
#18321=CYLINDRICAL_SURFACE('',#20163,6.933);
#18322=CYLINDRICAL_SURFACE('',#20164,6.933);
#18323=CYLINDRICAL_SURFACE('',#20165,6.933);
#18324=CYLINDRICAL_SURFACE('',#20166,6.933);
#18325=CYLINDRICAL_SURFACE('',#20167,6.933);
#18326=CYLINDRICAL_SURFACE('',#20168,6.933);
#18327=CYLINDRICAL_SURFACE('',#20169,6.933);
#18328=CYLINDRICAL_SURFACE('',#20170,6.933);
#18329=CYLINDRICAL_SURFACE('',#20171,6.933);
#18330=CYLINDRICAL_SURFACE('',#20172,6.933);
#18331=CYLINDRICAL_SURFACE('',#20173,6.933);
#18332=CYLINDRICAL_SURFACE('',#20174,6.933);
#18333=CYLINDRICAL_SURFACE('',#20175,6.933);
#18334=CYLINDRICAL_SURFACE('',#20176,6.933);
#18335=CYLINDRICAL_SURFACE('',#20177,6.933);
#18336=CYLINDRICAL_SURFACE('',#20178,6.933);
#18337=CYLINDRICAL_SURFACE('',#20179,6.933);
#18338=CYLINDRICAL_SURFACE('',#20180,6.933);
#18339=CYLINDRICAL_SURFACE('',#20181,6.933);
#18340=CYLINDRICAL_SURFACE('',#20182,6.933);
#18341=CYLINDRICAL_SURFACE('',#20183,6.933);
#18342=CYLINDRICAL_SURFACE('',#20184,6.933);
#18343=CYLINDRICAL_SURFACE('',#20185,6.933);
#18344=CYLINDRICAL_SURFACE('',#20186,6.933);
#18345=CYLINDRICAL_SURFACE('',#20187,6.933);
#18346=CYLINDRICAL_SURFACE('',#20188,6.933);
#18347=CYLINDRICAL_SURFACE('',#20189,6.933);
#18348=CYLINDRICAL_SURFACE('',#20190,6.933);
#18349=CYLINDRICAL_SURFACE('',#20191,6.933);
#18350=CYLINDRICAL_SURFACE('',#20192,6.933);
#18351=CYLINDRICAL_SURFACE('',#20193,6.933);
#18352=CYLINDRICAL_SURFACE('',#20194,6.933);
#18353=CYLINDRICAL_SURFACE('',#20195,6.933);
#18354=CYLINDRICAL_SURFACE('',#20196,6.933);
#18355=CYLINDRICAL_SURFACE('',#20197,6.933);
#18356=CYLINDRICAL_SURFACE('',#20198,6.933);
#18357=CYLINDRICAL_SURFACE('',#20199,6.933);
#18358=CYLINDRICAL_SURFACE('',#20200,6.933);
#18359=CYLINDRICAL_SURFACE('',#20201,6.933);
#18360=CYLINDRICAL_SURFACE('',#20202,6.933);
#18361=CYLINDRICAL_SURFACE('',#20203,6.933);
#18362=CYLINDRICAL_SURFACE('',#20204,6.933);
#18363=CYLINDRICAL_SURFACE('',#20205,6.933);
#18364=CYLINDRICAL_SURFACE('',#20206,6.933);
#18365=CYLINDRICAL_SURFACE('',#20207,6.933);
#18366=CYLINDRICAL_SURFACE('',#20208,6.933);
#18367=CYLINDRICAL_SURFACE('',#20209,6.933);
#18368=CYLINDRICAL_SURFACE('',#20210,6.933);
#18369=CYLINDRICAL_SURFACE('',#20211,6.933);
#18370=CYLINDRICAL_SURFACE('',#20212,6.933);
#18371=CYLINDRICAL_SURFACE('',#20213,6.933);
#18372=CYLINDRICAL_SURFACE('',#20214,6.933);
#18373=CYLINDRICAL_SURFACE('',#20218,6.933);
#18374=CYLINDRICAL_SURFACE('',#20219,6.933);
#18375=CYLINDRICAL_SURFACE('',#20220,6.933);
#18376=CYLINDRICAL_SURFACE('',#20221,6.933);
#18377=CYLINDRICAL_SURFACE('',#20222,6.933);
#18378=CYLINDRICAL_SURFACE('',#20223,6.933);
#18379=CYLINDRICAL_SURFACE('',#20224,6.933);
#18380=CYLINDRICAL_SURFACE('',#20225,6.933);
#18381=CYLINDRICAL_SURFACE('',#20226,6.933);
#18382=CYLINDRICAL_SURFACE('',#20227,6.933);
#18383=CYLINDRICAL_SURFACE('',#20228,6.933);
#18384=CYLINDRICAL_SURFACE('',#20229,6.933);
#18385=CYLINDRICAL_SURFACE('',#20230,6.933);
#18386=CYLINDRICAL_SURFACE('',#20231,6.933);
#18387=CYLINDRICAL_SURFACE('',#20232,6.933);
#18388=CYLINDRICAL_SURFACE('',#20233,6.21925);
#18389=CYLINDRICAL_SURFACE('',#20235,6.21925);
#18390=CYLINDRICAL_SURFACE('',#20236,6.21925);
#18391=CYLINDRICAL_SURFACE('',#20237,6.21925);
#18392=CYLINDRICAL_SURFACE('',#20238,6.21925);
#18393=CYLINDRICAL_SURFACE('',#20239,6.21925);
#18394=CYLINDRICAL_SURFACE('',#20240,6.21925);
#18395=CYLINDRICAL_SURFACE('',#20241,6.21925);
#18396=CYLINDRICAL_SURFACE('',#20242,6.21925);
#18397=CYLINDRICAL_SURFACE('',#20243,6.21925);
#18398=CYLINDRICAL_SURFACE('',#20244,6.21925);
#18399=CYLINDRICAL_SURFACE('',#20245,6.21925);
#18400=CYLINDRICAL_SURFACE('',#20246,6.21925);
#18401=CYLINDRICAL_SURFACE('',#20247,6.21925);
#18402=CYLINDRICAL_SURFACE('',#20248,6.21925);
#18403=CYLINDRICAL_SURFACE('',#20249,6.21925);
#18404=CYLINDRICAL_SURFACE('',#20250,6.21925);
#18405=CYLINDRICAL_SURFACE('',#20252,6.21925);
#18406=CYLINDRICAL_SURFACE('',#20254,6.21925);
#18407=CYLINDRICAL_SURFACE('',#20255,6.21925);
#18408=CYLINDRICAL_SURFACE('',#20256,6.21925);
#18409=CYLINDRICAL_SURFACE('',#20257,6.21925);
#18410=CYLINDRICAL_SURFACE('',#20258,6.21925);
#18411=CYLINDRICAL_SURFACE('',#20259,6.21925);
#18412=CYLINDRICAL_SURFACE('',#20260,6.21925);
#18413=CYLINDRICAL_SURFACE('',#20261,6.21925);
#18414=CYLINDRICAL_SURFACE('',#20262,6.21925);
#18415=CYLINDRICAL_SURFACE('',#20263,6.21925);
#18416=CYLINDRICAL_SURFACE('',#20264,6.21925);
#18417=CYLINDRICAL_SURFACE('',#20265,6.21925);
#18418=CYLINDRICAL_SURFACE('',#20266,6.21925);
#18419=CYLINDRICAL_SURFACE('',#20267,6.21925);
#18420=CYLINDRICAL_SURFACE('',#20268,6.21925);
#18421=CYLINDRICAL_SURFACE('',#20269,6.21925);
#18422=CYLINDRICAL_SURFACE('',#20270,6.21925);
#18423=CYLINDRICAL_SURFACE('',#20271,6.21925);
#18424=CYLINDRICAL_SURFACE('',#20272,6.21925);
#18425=CYLINDRICAL_SURFACE('',#20273,6.21925);
#18426=CYLINDRICAL_SURFACE('',#20274,6.21925);
#18427=CYLINDRICAL_SURFACE('',#20275,6.21925);
#18428=CYLINDRICAL_SURFACE('',#20276,6.21925);
#18429=CYLINDRICAL_SURFACE('',#20277,6.21925);
#18430=CYLINDRICAL_SURFACE('',#20278,6.21925);
#18431=CYLINDRICAL_SURFACE('',#20279,6.21925);
#18432=CYLINDRICAL_SURFACE('',#20280,6.21925);
#18433=CYLINDRICAL_SURFACE('',#20281,6.21925);
#18434=CYLINDRICAL_SURFACE('',#20282,6.21925);
#18435=CYLINDRICAL_SURFACE('',#20283,6.21925);
#18436=CYLINDRICAL_SURFACE('',#20284,6.21925);
#18437=CYLINDRICAL_SURFACE('',#20285,6.21925);
#18438=CYLINDRICAL_SURFACE('',#20286,6.21925);
#18439=CYLINDRICAL_SURFACE('',#20287,6.21925);
#18440=CYLINDRICAL_SURFACE('',#20288,6.21925);
#18441=CYLINDRICAL_SURFACE('',#20289,6.21925);
#18442=CYLINDRICAL_SURFACE('',#20290,6.21925);
#18443=CYLINDRICAL_SURFACE('',#20291,6.21925);
#18444=CYLINDRICAL_SURFACE('',#20292,6.21925);
#18445=CYLINDRICAL_SURFACE('',#20293,6.21925);
#18446=CYLINDRICAL_SURFACE('',#20294,6.21925);
#18447=CYLINDRICAL_SURFACE('',#20295,6.21925);
#18448=CYLINDRICAL_SURFACE('',#20296,6.21925);
#18449=CYLINDRICAL_SURFACE('',#20297,6.21925);
#18450=CYLINDRICAL_SURFACE('',#20298,6.21925);
#18451=CYLINDRICAL_SURFACE('',#20299,6.21925);
#18452=CYLINDRICAL_SURFACE('',#20300,6.21925);
#18453=CYLINDRICAL_SURFACE('',#20301,6.21925);
#18454=CYLINDRICAL_SURFACE('',#20302,6.21925);
#18455=CYLINDRICAL_SURFACE('',#20303,6.21925);
#18456=CYLINDRICAL_SURFACE('',#20304,6.21925);
#18457=CYLINDRICAL_SURFACE('',#20305,6.21925);
#18458=CYLINDRICAL_SURFACE('',#20306,6.21925);
#18459=CYLINDRICAL_SURFACE('',#20307,6.21925);
#18460=CYLINDRICAL_SURFACE('',#20308,6.21925);
#18461=CYLINDRICAL_SURFACE('',#20309,6.21925);
#18462=CYLINDRICAL_SURFACE('',#20310,6.21925);
#18463=CYLINDRICAL_SURFACE('',#20311,6.21925);
#18464=CYLINDRICAL_SURFACE('',#20312,6.21925);
#18465=CYLINDRICAL_SURFACE('',#20313,6.21925);
#18466=CYLINDRICAL_SURFACE('',#20314,6.21925);
#18467=CYLINDRICAL_SURFACE('',#20324,6.21925);
#18468=CYLINDRICAL_SURFACE('',#20330,6.21925);
#18469=CYLINDRICAL_SURFACE('',#20331,6.933);
#18470=CYLINDRICAL_SURFACE('',#20336,7.8125);
#18471=CYLINDRICAL_SURFACE('',#20346,10.625);
#18472=CYLINDRICAL_SURFACE('',#20353,7.8125);
#18473=CYLINDRICAL_SURFACE('',#20360,10.625);
#18474=CYLINDRICAL_SURFACE('',#20367,7.8125);
#18475=CYLINDRICAL_SURFACE('',#20374,10.625);
#18476=CYLINDRICAL_SURFACE('',#20381,7.8125);
#18477=CYLINDRICAL_SURFACE('',#20388,10.625);
#18478=CYLINDRICAL_SURFACE('',#20395,7.8125);
#18479=CYLINDRICAL_SURFACE('',#20402,10.625);
#18480=CYLINDRICAL_SURFACE('',#20409,7.8125);
#18481=CYLINDRICAL_SURFACE('',#20416,10.625);
#18482=CYLINDRICAL_SURFACE('',#20423,7.8125);
#18483=CYLINDRICAL_SURFACE('',#20430,10.625);
#18484=CYLINDRICAL_SURFACE('',#20438,7.8125);
#18485=CYLINDRICAL_SURFACE('',#20446,10.625);
#18486=CYLINDRICAL_SURFACE('',#20453,7.8125);
#18487=CYLINDRICAL_SURFACE('',#20460,10.625);
#18488=CYLINDRICAL_SURFACE('',#20467,7.8125);
#18489=CYLINDRICAL_SURFACE('',#20474,10.625);
#18490=CYLINDRICAL_SURFACE('',#20481,7.8125);
#18491=CYLINDRICAL_SURFACE('',#20488,10.625);
#18492=CYLINDRICAL_SURFACE('',#20495,7.8125);
#18493=CYLINDRICAL_SURFACE('',#20502,10.625);
#18494=CYLINDRICAL_SURFACE('',#20509,7.8125);
#18495=CYLINDRICAL_SURFACE('',#20516,10.625);
#18496=CYLINDRICAL_SURFACE('',#20523,7.8125);
#18497=CYLINDRICAL_SURFACE('',#20530,10.625);
#18498=CYLINDRICAL_SURFACE('',#20537,7.8125);
#18499=CYLINDRICAL_SURFACE('',#20544,10.625);
#18500=CYLINDRICAL_SURFACE('',#20550,6.933);
#18822=ADVANCED_FACE('',(#1126,#1082),#18310,.T.);
#18823=ADVANCED_FACE('',(#1127),#18311,.T.);
#18824=ADVANCED_FACE('',(#1128),#18312,.T.);
#18825=ADVANCED_FACE('',(#1129),#18313,.T.);
#18826=ADVANCED_FACE('',(#1130),#18314,.T.);
#18827=ADVANCED_FACE('',(#1131),#18315,.T.);
#18828=ADVANCED_FACE('',(#1132),#18316,.T.);
#18829=ADVANCED_FACE('',(#1133),#18317,.T.);
#18830=ADVANCED_FACE('',(#1134),#18318,.T.);
#18831=ADVANCED_FACE('',(#1135),#18319,.T.);
#18832=ADVANCED_FACE('',(#1136),#18320,.T.);
#18833=ADVANCED_FACE('',(#1137),#18321,.T.);
#18834=ADVANCED_FACE('',(#1138),#18322,.T.);
#18835=ADVANCED_FACE('',(#1139),#18323,.T.);
#18836=ADVANCED_FACE('',(#1140),#18324,.T.);
#18837=ADVANCED_FACE('',(#1141),#18325,.T.);
#18838=ADVANCED_FACE('',(#1142),#18326,.T.);
#18839=ADVANCED_FACE('',(#1143),#18327,.T.);
#18840=ADVANCED_FACE('',(#1144),#18328,.T.);
#18841=ADVANCED_FACE('',(#1145),#18329,.T.);
#18842=ADVANCED_FACE('',(#1146),#18330,.T.);
#18843=ADVANCED_FACE('',(#1147),#18331,.T.);
#18844=ADVANCED_FACE('',(#1148),#18332,.T.);
#18845=ADVANCED_FACE('',(#1149),#18333,.T.);
#18846=ADVANCED_FACE('',(#1150),#18334,.T.);
#18847=ADVANCED_FACE('',(#1151),#18335,.T.);
#18848=ADVANCED_FACE('',(#1152),#18336,.T.);
#18849=ADVANCED_FACE('',(#1153),#18337,.T.);
#18850=ADVANCED_FACE('',(#1154),#18338,.T.);
#18851=ADVANCED_FACE('',(#1155),#18339,.T.);
#18852=ADVANCED_FACE('',(#1156),#18340,.T.);
#18853=ADVANCED_FACE('',(#1157),#18341,.T.);
#18854=ADVANCED_FACE('',(#1158),#18342,.T.);
#18855=ADVANCED_FACE('',(#1159),#18343,.T.);
#18856=ADVANCED_FACE('',(#1160),#18344,.T.);
#18857=ADVANCED_FACE('',(#1161),#18345,.T.);
#18858=ADVANCED_FACE('',(#1162),#18346,.T.);
#18859=ADVANCED_FACE('',(#1163),#18347,.T.);
#18860=ADVANCED_FACE('',(#1164),#18348,.T.);
#18861=ADVANCED_FACE('',(#1165),#18349,.T.);
#18862=ADVANCED_FACE('',(#1166),#18350,.T.);
#18863=ADVANCED_FACE('',(#1167),#18351,.T.);
#18864=ADVANCED_FACE('',(#1168),#18352,.T.);
#18865=ADVANCED_FACE('',(#1169),#18353,.T.);
#18866=ADVANCED_FACE('',(#1170),#18354,.T.);
#18867=ADVANCED_FACE('',(#1171),#18355,.T.);
#18868=ADVANCED_FACE('',(#1172),#18356,.T.);
#18869=ADVANCED_FACE('',(#1173),#18357,.T.);
#18870=ADVANCED_FACE('',(#1174),#18358,.T.);
#18871=ADVANCED_FACE('',(#1175),#18359,.T.);
#18872=ADVANCED_FACE('',(#1176),#18360,.T.);
#18873=ADVANCED_FACE('',(#1177),#18361,.T.);
#18874=ADVANCED_FACE('',(#1178),#18362,.T.);
#18875=ADVANCED_FACE('',(#1179),#18363,.T.);
#18876=ADVANCED_FACE('',(#1180),#18364,.T.);
#18877=ADVANCED_FACE('',(#1181),#18365,.T.);
#18878=ADVANCED_FACE('',(#1182),#18366,.T.);
#18879=ADVANCED_FACE('',(#1183),#18367,.T.);
#18880=ADVANCED_FACE('',(#1184),#18368,.T.);
#18881=ADVANCED_FACE('',(#1185),#18369,.T.);
#18882=ADVANCED_FACE('',(#1186),#18370,.T.);
#18883=ADVANCED_FACE('',(#1187),#18371,.T.);
#18884=ADVANCED_FACE('',(#1188),#18372,.T.);
#18885=ADVANCED_FACE('',(#1189),#18373,.T.);
#18886=ADVANCED_FACE('',(#1190),#18374,.T.);
#18887=ADVANCED_FACE('',(#1191),#18375,.T.);
#18888=ADVANCED_FACE('',(#1192),#18376,.T.);
#18889=ADVANCED_FACE('',(#1193),#18377,.T.);
#18890=ADVANCED_FACE('',(#1194),#18378,.T.);
#18891=ADVANCED_FACE('',(#1195),#18379,.T.);
#18892=ADVANCED_FACE('',(#1196),#18380,.T.);
#18893=ADVANCED_FACE('',(#1197),#18381,.T.);
#18894=ADVANCED_FACE('',(#1198),#18382,.T.);
#18895=ADVANCED_FACE('',(#1199),#18383,.T.);
#18896=ADVANCED_FACE('',(#1200),#18384,.T.);
#18897=ADVANCED_FACE('',(#1201),#18385,.T.);
#18898=ADVANCED_FACE('',(#1202),#18386,.T.);
#18899=ADVANCED_FACE('',(#1203),#18387,.T.);
#18900=ADVANCED_FACE('',(#1204),#18388,.T.);
#18901=ADVANCED_FACE('',(#1205),#18389,.T.);
#18902=ADVANCED_FACE('',(#1206),#18390,.T.);
#18903=ADVANCED_FACE('',(#1207),#18391,.T.);
#18904=ADVANCED_FACE('',(#1208),#18392,.T.);
#18905=ADVANCED_FACE('',(#1209),#18393,.T.);
#18906=ADVANCED_FACE('',(#1210),#18394,.T.);
#18907=ADVANCED_FACE('',(#1211),#18395,.T.);
#18908=ADVANCED_FACE('',(#1212),#18396,.T.);
#18909=ADVANCED_FACE('',(#1213),#18397,.T.);
#18910=ADVANCED_FACE('',(#1214),#18398,.T.);
#18911=ADVANCED_FACE('',(#1215),#18399,.T.);
#18912=ADVANCED_FACE('',(#1216),#18400,.T.);
#18913=ADVANCED_FACE('',(#1217),#18401,.T.);
#18914=ADVANCED_FACE('',(#1218),#18402,.T.);
#18915=ADVANCED_FACE('',(#1219),#18403,.T.);
#18916=ADVANCED_FACE('',(#1220),#18404,.T.);
#18917=ADVANCED_FACE('',(#1221),#18405,.T.);
#18918=ADVANCED_FACE('',(#1222),#18406,.T.);
#18919=ADVANCED_FACE('',(#1223),#18407,.T.);
#18920=ADVANCED_FACE('',(#1224),#18408,.T.);
#18921=ADVANCED_FACE('',(#1225),#18409,.T.);
#18922=ADVANCED_FACE('',(#1226),#18410,.T.);
#18923=ADVANCED_FACE('',(#1227),#18411,.T.);
#18924=ADVANCED_FACE('',(#1228),#18412,.T.);
#18925=ADVANCED_FACE('',(#1229),#18413,.T.);
#18926=ADVANCED_FACE('',(#1230),#18414,.T.);
#18927=ADVANCED_FACE('',(#1231),#18415,.T.);
#18928=ADVANCED_FACE('',(#1232),#18416,.T.);
#18929=ADVANCED_FACE('',(#1233),#18417,.T.);
#18930=ADVANCED_FACE('',(#1234),#18418,.T.);
#18931=ADVANCED_FACE('',(#1235),#18419,.T.);
#18932=ADVANCED_FACE('',(#1236),#18420,.T.);
#18933=ADVANCED_FACE('',(#1237),#18421,.T.);
#18934=ADVANCED_FACE('',(#1238),#18422,.T.);
#18935=ADVANCED_FACE('',(#1239),#18423,.T.);
#18936=ADVANCED_FACE('',(#1240),#18424,.T.);
#18937=ADVANCED_FACE('',(#1241),#18425,.T.);
#18938=ADVANCED_FACE('',(#1242),#18426,.T.);
#18939=ADVANCED_FACE('',(#1243),#18427,.T.);
#18940=ADVANCED_FACE('',(#1244),#18428,.T.);
#18941=ADVANCED_FACE('',(#1245),#18429,.T.);
#18942=ADVANCED_FACE('',(#1246),#18430,.T.);
#18943=ADVANCED_FACE('',(#1247),#18431,.T.);
#18944=ADVANCED_FACE('',(#1248),#18432,.T.);
#18945=ADVANCED_FACE('',(#1249),#18433,.T.);
#18946=ADVANCED_FACE('',(#1250),#18434,.T.);
#18947=ADVANCED_FACE('',(#1251),#18435,.T.);
#18948=ADVANCED_FACE('',(#1252),#18436,.T.);
#18949=ADVANCED_FACE('',(#1253),#18437,.T.);
#18950=ADVANCED_FACE('',(#1254),#18438,.T.);
#18951=ADVANCED_FACE('',(#1255),#18439,.T.);
#18952=ADVANCED_FACE('',(#1256),#18440,.T.);
#18953=ADVANCED_FACE('',(#1257),#18441,.T.);
#18954=ADVANCED_FACE('',(#1258),#18442,.T.);
#18955=ADVANCED_FACE('',(#1259),#18443,.T.);
#18956=ADVANCED_FACE('',(#1260),#18444,.T.);
#18957=ADVANCED_FACE('',(#1261),#18445,.T.);
#18958=ADVANCED_FACE('',(#1262),#18446,.T.);
#18959=ADVANCED_FACE('',(#1263),#18447,.T.);
#18960=ADVANCED_FACE('',(#1264),#18448,.T.);
#18961=ADVANCED_FACE('',(#1265),#18449,.T.);
#18962=ADVANCED_FACE('',(#1266),#18450,.T.);
#18963=ADVANCED_FACE('',(#1267),#18451,.T.);
#18964=ADVANCED_FACE('',(#1268),#18452,.T.);
#18965=ADVANCED_FACE('',(#1269),#18453,.T.);
#18966=ADVANCED_FACE('',(#1270),#18454,.T.);
#18967=ADVANCED_FACE('',(#1271),#18455,.T.);
#18968=ADVANCED_FACE('',(#1272),#18456,.T.);
#18969=ADVANCED_FACE('',(#1273),#18457,.T.);
#18970=ADVANCED_FACE('',(#1274),#18458,.T.);
#18971=ADVANCED_FACE('',(#1275),#18459,.T.);
#18972=ADVANCED_FACE('',(#1276),#18460,.T.);
#18973=ADVANCED_FACE('',(#1277),#18461,.T.);
#18974=ADVANCED_FACE('',(#1278),#18462,.T.);
#18975=ADVANCED_FACE('',(#1279),#18463,.T.);
#18976=ADVANCED_FACE('',(#1280),#18464,.T.);
#18977=ADVANCED_FACE('',(#1281),#18465,.T.);
#18978=ADVANCED_FACE('',(#1282),#18466,.T.);
#18979=ADVANCED_FACE('',(#1283),#853,.F.);
#18980=ADVANCED_FACE('',(#1284),#854,.F.);
#18981=ADVANCED_FACE('',(#1285),#855,.F.);
#18982=ADVANCED_FACE('',(#1286),#856,.F.);
#18983=ADVANCED_FACE('',(#1287),#857,.F.);
#18984=ADVANCED_FACE('',(#1288),#834,.F.);
#18985=ADVANCED_FACE('',(#1289),#858,.T.);
#18986=ADVANCED_FACE('',(#1290),#18467,.T.);
#18987=ADVANCED_FACE('',(#1291),#835,.F.);
#18988=ADVANCED_FACE('',(#1292),#859,.F.);
#18989=ADVANCED_FACE('',(#1293),#836,.F.);
#18990=ADVANCED_FACE('',(#1294),#860,.T.);
#18991=ADVANCED_FACE('',(#1295),#18468,.T.);
#18992=ADVANCED_FACE('',(#1296),#837,.F.);
#18993=ADVANCED_FACE('',(#1297),#18469,.T.);
#18994=ADVANCED_FACE('',(#1298),#861,.T.);
#18995=ADVANCED_FACE('',(#1299),#500,.F.);
#18996=ADVANCED_FACE('',(#1300),#18470,.T.);
#18997=ADVANCED_FACE('',(#1301),#501,.F.);
#18998=ADVANCED_FACE('',(#1302),#862,.F.);
#18999=ADVANCED_FACE('',(#1303),#380,.T.);
#19000=ADVANCED_FACE('',(#1304),#381,.T.);
#19001=ADVANCED_FACE('',(#1305),#18471,.T.);
#19002=ADVANCED_FACE('',(#1306),#382,.T.);
#19003=ADVANCED_FACE('',(#1307),#863,.T.);
#19004=ADVANCED_FACE('',(#1308),#502,.F.);
#19005=ADVANCED_FACE('',(#1309),#18472,.T.);
#19006=ADVANCED_FACE('',(#1310),#503,.F.);
#19007=ADVANCED_FACE('',(#1311),#864,.F.);
#19008=ADVANCED_FACE('',(#1312),#383,.T.);
#19009=ADVANCED_FACE('',(#1313),#18473,.T.);
#19010=ADVANCED_FACE('',(#1314),#384,.T.);
#19011=ADVANCED_FACE('',(#1315),#865,.T.);
#19012=ADVANCED_FACE('',(#1316),#504,.F.);
#19013=ADVANCED_FACE('',(#1317),#18474,.T.);
#19014=ADVANCED_FACE('',(#1318),#505,.F.);
#19015=ADVANCED_FACE('',(#1319),#866,.F.);
#19016=ADVANCED_FACE('',(#1320),#385,.T.);
#19017=ADVANCED_FACE('',(#1321),#18475,.T.);
#19018=ADVANCED_FACE('',(#1322),#386,.T.);
#19019=ADVANCED_FACE('',(#1323),#867,.T.);
#19020=ADVANCED_FACE('',(#1324),#506,.F.);
#19021=ADVANCED_FACE('',(#1325),#18476,.T.);
#19022=ADVANCED_FACE('',(#1326),#507,.F.);
#19023=ADVANCED_FACE('',(#1327),#868,.F.);
#19024=ADVANCED_FACE('',(#1328),#387,.T.);
#19025=ADVANCED_FACE('',(#1329),#18477,.T.);
#19026=ADVANCED_FACE('',(#1330),#388,.T.);
#19027=ADVANCED_FACE('',(#1331),#869,.T.);
#19028=ADVANCED_FACE('',(#1332),#508,.F.);
#19029=ADVANCED_FACE('',(#1333),#18478,.T.);
#19030=ADVANCED_FACE('',(#1334),#509,.F.);
#19031=ADVANCED_FACE('',(#1335),#870,.F.);
#19032=ADVANCED_FACE('',(#1336),#389,.T.);
#19033=ADVANCED_FACE('',(#1337),#18479,.T.);
#19034=ADVANCED_FACE('',(#1338),#390,.T.);
#19035=ADVANCED_FACE('',(#1339),#871,.T.);
#19036=ADVANCED_FACE('',(#1340),#510,.F.);
#19037=ADVANCED_FACE('',(#1341),#18480,.T.);
#19038=ADVANCED_FACE('',(#1342),#511,.F.);
#19039=ADVANCED_FACE('',(#1343),#872,.F.);
#19040=ADVANCED_FACE('',(#1344),#391,.T.);
#19041=ADVANCED_FACE('',(#1345),#18481,.T.);
#19042=ADVANCED_FACE('',(#1346),#392,.T.);
#19043=ADVANCED_FACE('',(#1347),#873,.T.);
#19044=ADVANCED_FACE('',(#1348),#512,.F.);
#19045=ADVANCED_FACE('',(#1349),#18482,.T.);
#19046=ADVANCED_FACE('',(#1350),#513,.F.);
#19047=ADVANCED_FACE('',(#1351),#874,.F.);
#19048=ADVANCED_FACE('',(#1352),#393,.T.);
#19049=ADVANCED_FACE('',(#1353),#18483,.T.);
#19050=ADVANCED_FACE('',(#1354),#394,.T.);
#19051=ADVANCED_FACE('',(#1355),#875,.T.);
#19052=ADVANCED_FACE('',(#1356),#514,.F.);
#19053=ADVANCED_FACE('',(#1357),#18484,.T.);
#19054=ADVANCED_FACE('',(#1358),#515,.F.);
#19055=ADVANCED_FACE('',(#1359),#876,.F.);
#19056=ADVANCED_FACE('',(#1360),#395,.T.);
#19057=ADVANCED_FACE('',(#1361),#18485,.T.);
#19058=ADVANCED_FACE('',(#1362),#396,.T.);
#19059=ADVANCED_FACE('',(#1363),#877,.T.);
#19060=ADVANCED_FACE('',(#1364),#516,.F.);
#19061=ADVANCED_FACE('',(#1365),#18486,.T.);
#19062=ADVANCED_FACE('',(#1366),#517,.F.);
#19063=ADVANCED_FACE('',(#1367),#878,.F.);
#19064=ADVANCED_FACE('',(#1368),#397,.T.);
#19065=ADVANCED_FACE('',(#1369),#18487,.T.);
#19066=ADVANCED_FACE('',(#1370),#398,.T.);
#19067=ADVANCED_FACE('',(#1371),#879,.T.);
#19068=ADVANCED_FACE('',(#1372),#518,.F.);
#19069=ADVANCED_FACE('',(#1373),#18488,.T.);
#19070=ADVANCED_FACE('',(#1374),#519,.F.);
#19071=ADVANCED_FACE('',(#1375),#880,.F.);
#19072=ADVANCED_FACE('',(#1376),#399,.T.);
#19073=ADVANCED_FACE('',(#1377),#18489,.T.);
#19074=ADVANCED_FACE('',(#1378),#400,.T.);
#19075=ADVANCED_FACE('',(#1379),#881,.T.);
#19076=ADVANCED_FACE('',(#1380),#520,.F.);
#19077=ADVANCED_FACE('',(#1381),#18490,.T.);
#19078=ADVANCED_FACE('',(#1382),#521,.F.);
#19079=ADVANCED_FACE('',(#1383),#882,.F.);
#19080=ADVANCED_FACE('',(#1384),#401,.T.);
#19081=ADVANCED_FACE('',(#1385),#18491,.T.);
#19082=ADVANCED_FACE('',(#1386),#402,.T.);
#19083=ADVANCED_FACE('',(#1387),#883,.T.);
#19084=ADVANCED_FACE('',(#1388),#522,.F.);
#19085=ADVANCED_FACE('',(#1389),#18492,.T.);
#19086=ADVANCED_FACE('',(#1390),#523,.F.);
#19087=ADVANCED_FACE('',(#1391),#884,.F.);
#19088=ADVANCED_FACE('',(#1392),#403,.T.);
#19089=ADVANCED_FACE('',(#1393),#18493,.T.);
#19090=ADVANCED_FACE('',(#1394),#404,.T.);
#19091=ADVANCED_FACE('',(#1395),#885,.T.);
#19092=ADVANCED_FACE('',(#1396),#524,.F.);
#19093=ADVANCED_FACE('',(#1397),#18494,.T.);
#19094=ADVANCED_FACE('',(#1398),#525,.F.);
#19095=ADVANCED_FACE('',(#1399),#886,.F.);
#19096=ADVANCED_FACE('',(#1400),#405,.T.);
#19097=ADVANCED_FACE('',(#1401),#18495,.T.);
#19098=ADVANCED_FACE('',(#1402),#406,.T.);
#19099=ADVANCED_FACE('',(#1403),#887,.T.);
#19100=ADVANCED_FACE('',(#1404),#526,.F.);
#19101=ADVANCED_FACE('',(#1405),#18496,.T.);
#19102=ADVANCED_FACE('',(#1406),#527,.F.);
#19103=ADVANCED_FACE('',(#1407),#888,.F.);
#19104=ADVANCED_FACE('',(#1408),#407,.T.);
#19105=ADVANCED_FACE('',(#1409),#18497,.T.);
#19106=ADVANCED_FACE('',(#1410),#408,.T.);
#19107=ADVANCED_FACE('',(#1411),#528,.F.);
#19108=ADVANCED_FACE('',(#1412),#889,.T.);
#19109=ADVANCED_FACE('',(#1413),#18498,.T.);
#19110=ADVANCED_FACE('',(#1414),#529,.F.);
#19111=ADVANCED_FACE('',(#1415),#890,.F.);
#19112=ADVANCED_FACE('',(#1416),#409,.T.);
#19113=ADVANCED_FACE('',(#1417),#18499,.T.);
#19114=ADVANCED_FACE('',(#1418),#891,.T.);
#19115=ADVANCED_FACE('',(#1419),#410,.T.);
#19116=ADVANCED_FACE('',(#1420),#411,.T.);
#19117=ADVANCED_FACE('',(#1421),#412,.T.);
#19118=ADVANCED_FACE('',(#1422),#18500,.T.);
#19119=ADVANCED_FACE('',(#1423),#413,.T.);
#19120=ADVANCED_FACE('',(#1424),#892,.T.);
#20008=CLOSED_SHELL('',(#18822,#18823,#18824,#18825,#18826,#18827,#18828,
#18829,#18830,#18831,#18832,#18833,#18834,#18835,#18836,#18837,#18838,#18839,
#18840,#18841,#18842,#18843,#18844,#18845,#18846,#18847,#18848,#18849,#18850,
#18851,#18852,#18853,#18854,#18855,#18856,#18857,#18858,#18859,#18860,#18861,
#18862,#18863,#18864,#18865,#18866,#18867,#18868,#18869,#18870,#18871,#18872,
#18873,#18874,#18875,#18876,#18877,#18878,#18879,#18880,#18881,#18882,#18883,
#18884,#18885,#18886,#18887,#18888,#18889,#18890,#18891,#18892,#18893,#18894,
#18895,#18896,#18897,#18898,#18899,#18900,#18901,#18902,#18903,#18904,#18905,
#18906,#18907,#18908,#18909,#18910,#18911,#18912,#18913,#18914,#18915,#18916,
#18917,#18918,#18919,#18920,#18921,#18922,#18923,#18924,#18925,#18926,#18927,
#18928,#18929,#18930,#18931,#18932,#18933,#18934,#18935,#18936,#18937,#18938,
#18939,#18940,#18941,#18942,#18943,#18944,#18945,#18946,#18947,#18948,#18949,
#18950,#18951,#18952,#18953,#18954,#18955,#18956,#18957,#18958,#18959,#18960,
#18961,#18962,#18963,#18964,#18965,#18966,#18967,#18968,#18969,#18970,#18971,
#18972,#18973,#18974,#18975,#18976,#18977,#18978,#18979,#18980,#18981,#18982,
#18983,#18984,#18985,#18986,#18987,#18988,#18989,#18990,#18991,#18992,#18993,
#18994,#18995,#18996,#18997,#18998,#18999,#19000,#19001,#19002,#19003,#19004,
#19005,#19006,#19007,#19008,#19009,#19010,#19011,#19012,#19013,#19014,#19015,
#19016,#19017,#19018,#19019,#19020,#19021,#19022,#19023,#19024,#19025,#19026,
#19027,#19028,#19029,#19030,#19031,#19032,#19033,#19034,#19035,#19036,#19037,
#19038,#19039,#19040,#19041,#19042,#19043,#19044,#19045,#19046,#19047,#19048,
#19049,#19050,#19051,#19052,#19053,#19054,#19055,#19056,#19057,#19058,#19059,
#19060,#19061,#19062,#19063,#19064,#19065,#19066,#19067,#19068,#19069,#19070,
#19071,#19072,#19073,#19074,#19075,#19076,#19077,#19078,#19079,#19080,#19081,
#19082,#19083,#19084,#19085,#19086,#19087,#19088,#19089,#19090,#19091,#19092,
#19093,#19094,#19095,#19096,#19097,#19098,#19099,#19100,#19101,#19102,#19103,
#19104,#19105,#19106,#19107,#19108,#19109,#19110,#19111,#19112,#19113,#19114,
#19115,#19116,#19117,#19118,#19119,#19120));
#20142=AXIS2_PLACEMENT_3D('',#27820,#22405,#22406);
#20143=AXIS2_PLACEMENT_3D('',#27821,#22407,#22408);
#20144=AXIS2_PLACEMENT_3D('',#27852,#22410,#22411);
#20145=AXIS2_PLACEMENT_3D('',#27856,#22413,#22414);
#20146=AXIS2_PLACEMENT_3D('',#27860,#22416,#22417);
#20147=AXIS2_PLACEMENT_3D('',#27863,#22419,#22420);
#20148=AXIS2_PLACEMENT_3D('',#27865,#22421,#22422);
#20149=AXIS2_PLACEMENT_3D('',#27868,#22424,#22425);
#20150=AXIS2_PLACEMENT_3D('',#27870,#22426,#22427);
#20151=AXIS2_PLACEMENT_3D('',#27897,#22429,#22430);
#20152=AXIS2_PLACEMENT_3D('',#27900,#22432,#22433);
#20153=AXIS2_PLACEMENT_3D('',#27901,#22434,#22435);
#20154=AXIS2_PLACEMENT_3D('',#27961,#22437,#22438);
#20155=AXIS2_PLACEMENT_3D('',#28021,#22440,#22441);
#20156=AXIS2_PLACEMENT_3D('',#28078,#22443,#22444);
#20157=AXIS2_PLACEMENT_3D('',#28138,#22446,#22447);
#20158=AXIS2_PLACEMENT_3D('',#28198,#22449,#22450);
#20159=AXIS2_PLACEMENT_3D('',#28258,#22452,#22453);
#20160=AXIS2_PLACEMENT_3D('',#28315,#22455,#22456);
#20161=AXIS2_PLACEMENT_3D('',#28372,#22458,#22459);
#20162=AXIS2_PLACEMENT_3D('',#28435,#22461,#22462);
#20163=AXIS2_PLACEMENT_3D('',#28489,#22464,#22465);
#20164=AXIS2_PLACEMENT_3D('',#28549,#22467,#22468);
#20165=AXIS2_PLACEMENT_3D('',#28609,#22470,#22471);
#20166=AXIS2_PLACEMENT_3D('',#28666,#22473,#22474);
#20167=AXIS2_PLACEMENT_3D('',#28723,#22476,#22477);
#20168=AXIS2_PLACEMENT_3D('',#28789,#22479,#22480);
#20169=AXIS2_PLACEMENT_3D('',#28849,#22482,#22483);
#20170=AXIS2_PLACEMENT_3D('',#28906,#22485,#22486);
#20171=AXIS2_PLACEMENT_3D('',#28963,#22488,#22489);
#20172=AXIS2_PLACEMENT_3D('',#29026,#22491,#22492);
#20173=AXIS2_PLACEMENT_3D('',#29080,#22494,#22495);
#20174=AXIS2_PLACEMENT_3D('',#29137,#22497,#22498);
#20175=AXIS2_PLACEMENT_3D('',#29197,#22500,#22501);
#20176=AXIS2_PLACEMENT_3D('',#29254,#22503,#22504);
#20177=AXIS2_PLACEMENT_3D('',#29311,#22506,#22507);
#20178=AXIS2_PLACEMENT_3D('',#29377,#22509,#22510);
#20179=AXIS2_PLACEMENT_3D('',#29437,#22512,#22513);
#20180=AXIS2_PLACEMENT_3D('',#29494,#22515,#22516);
#20181=AXIS2_PLACEMENT_3D('',#29551,#22518,#22519);
#20182=AXIS2_PLACEMENT_3D('',#29611,#22521,#22522);
#20183=AXIS2_PLACEMENT_3D('',#29665,#22524,#22525);
#20184=AXIS2_PLACEMENT_3D('',#29722,#22527,#22528);
#20185=AXIS2_PLACEMENT_3D('',#29785,#22530,#22531);
#20186=AXIS2_PLACEMENT_3D('',#29845,#22533,#22534);
#20187=AXIS2_PLACEMENT_3D('',#29899,#22536,#22537);
#20188=AXIS2_PLACEMENT_3D('',#29959,#22539,#22540);
#20189=AXIS2_PLACEMENT_3D('',#30019,#22542,#22543);
#20190=AXIS2_PLACEMENT_3D('',#30076,#22545,#22546);
#20191=AXIS2_PLACEMENT_3D('',#30136,#22548,#22549);
#20192=AXIS2_PLACEMENT_3D('',#30196,#22551,#22552);
#20193=AXIS2_PLACEMENT_3D('',#30253,#22554,#22555);
#20194=AXIS2_PLACEMENT_3D('',#30313,#22557,#22558);
#20195=AXIS2_PLACEMENT_3D('',#30373,#22560,#22561);
#20196=AXIS2_PLACEMENT_3D('',#30433,#22563,#22564);
#20197=AXIS2_PLACEMENT_3D('',#30487,#22566,#22567);
#20198=AXIS2_PLACEMENT_3D('',#30544,#22569,#22570);
#20199=AXIS2_PLACEMENT_3D('',#30607,#22572,#22573);
#20200=AXIS2_PLACEMENT_3D('',#30664,#22575,#22576);
#20201=AXIS2_PLACEMENT_3D('',#30724,#22578,#22579);
#20202=AXIS2_PLACEMENT_3D('',#30784,#22581,#22582);
#20203=AXIS2_PLACEMENT_3D('',#30841,#22584,#22585);
#20204=AXIS2_PLACEMENT_3D('',#30901,#22587,#22588);
#20205=AXIS2_PLACEMENT_3D('',#30964,#22590,#22591);
#20206=AXIS2_PLACEMENT_3D('',#31024,#22593,#22594);
#20207=AXIS2_PLACEMENT_3D('',#31078,#22596,#22597);
#20208=AXIS2_PLACEMENT_3D('',#31135,#22599,#22600);
#20209=AXIS2_PLACEMENT_3D('',#31195,#22602,#22603);
#20210=AXIS2_PLACEMENT_3D('',#31252,#22605,#22606);
#20211=AXIS2_PLACEMENT_3D('',#31309,#22608,#22609);
#20212=AXIS2_PLACEMENT_3D('',#31369,#22611,#22612);
#20213=AXIS2_PLACEMENT_3D('',#31426,#22614,#22615);
#20214=AXIS2_PLACEMENT_3D('',#31486,#22617,#22618);
#20215=AXIS2_PLACEMENT_3D('',#31505,#22620,#22621);
#20216=AXIS2_PLACEMENT_3D('',#31508,#22623,#22624);
#20217=AXIS2_PLACEMENT_3D('',#31510,#22625,#22626);
#20218=AXIS2_PLACEMENT_3D('',#31518,#22627,#22628);
#20219=AXIS2_PLACEMENT_3D('',#31608,#22630,#22631);
#20220=AXIS2_PLACEMENT_3D('',#31692,#22633,#22634);
#20221=AXIS2_PLACEMENT_3D('',#31782,#22636,#22637);
#20222=AXIS2_PLACEMENT_3D('',#31872,#22639,#22640);
#20223=AXIS2_PLACEMENT_3D('',#31956,#22642,#22643);
#20224=AXIS2_PLACEMENT_3D('',#32046,#22645,#22646);
#20225=AXIS2_PLACEMENT_3D('',#32130,#22648,#22649);
#20226=AXIS2_PLACEMENT_3D('',#32220,#22651,#22652);
#20227=AXIS2_PLACEMENT_3D('',#32310,#22654,#22655);
#20228=AXIS2_PLACEMENT_3D('',#32394,#22657,#22658);
#20229=AXIS2_PLACEMENT_3D('',#32484,#22660,#22661);
#20230=AXIS2_PLACEMENT_3D('',#32574,#22663,#22664);
#20231=AXIS2_PLACEMENT_3D('',#32658,#22666,#22667);
#20232=AXIS2_PLACEMENT_3D('',#32748,#22669,#22670);
#20233=AXIS2_PLACEMENT_3D('',#32832,#22672,#22673);
#20234=AXIS2_PLACEMENT_3D('',#32847,#22675,#22676);
#20235=AXIS2_PLACEMENT_3D('',#32854,#22677,#22678);
#20236=AXIS2_PLACEMENT_3D('',#32891,#22680,#22681);
#20237=AXIS2_PLACEMENT_3D('',#32928,#22683,#22684);
#20238=AXIS2_PLACEMENT_3D('',#32965,#22686,#22687);
#20239=AXIS2_PLACEMENT_3D('',#33002,#22689,#22690);
#20240=AXIS2_PLACEMENT_3D('',#33040,#22692,#22693);
#20241=AXIS2_PLACEMENT_3D('',#33077,#22695,#22696);
#20242=AXIS2_PLACEMENT_3D('',#33114,#22698,#22699);
#20243=AXIS2_PLACEMENT_3D('',#33152,#22701,#22702);
#20244=AXIS2_PLACEMENT_3D('',#33189,#22704,#22705);
#20245=AXIS2_PLACEMENT_3D('',#33226,#22707,#22708);
#20246=AXIS2_PLACEMENT_3D('',#33263,#22710,#22711);
#20247=AXIS2_PLACEMENT_3D('',#33300,#22713,#22714);
#20248=AXIS2_PLACEMENT_3D('',#33338,#22716,#22717);
#20249=AXIS2_PLACEMENT_3D('',#33375,#22719,#22720);
#20250=AXIS2_PLACEMENT_3D('',#33412,#22722,#22723);
#20251=AXIS2_PLACEMENT_3D('',#33424,#22725,#22726);
#20252=AXIS2_PLACEMENT_3D('',#33425,#22727,#22728);
#20253=AXIS2_PLACEMENT_3D('',#33442,#22730,#22731);
#20254=AXIS2_PLACEMENT_3D('',#33456,#22732,#22733);
#20255=AXIS2_PLACEMENT_3D('',#33484,#22735,#22736);
#20256=AXIS2_PLACEMENT_3D('',#33512,#22738,#22739);
#20257=AXIS2_PLACEMENT_3D('',#33553,#22741,#22742);
#20258=AXIS2_PLACEMENT_3D('',#33594,#22744,#22745);
#20259=AXIS2_PLACEMENT_3D('',#33622,#22747,#22748);
#20260=AXIS2_PLACEMENT_3D('',#33650,#22750,#22751);
#20261=AXIS2_PLACEMENT_3D('',#33691,#22753,#22754);
#20262=AXIS2_PLACEMENT_3D('',#33732,#22756,#22757);
#20263=AXIS2_PLACEMENT_3D('',#33761,#22759,#22760);
#20264=AXIS2_PLACEMENT_3D('',#33789,#22762,#22763);
#20265=AXIS2_PLACEMENT_3D('',#33817,#22765,#22766);
#20266=AXIS2_PLACEMENT_3D('',#33845,#22768,#22769);
#20267=AXIS2_PLACEMENT_3D('',#33886,#22771,#22772);
#20268=AXIS2_PLACEMENT_3D('',#33927,#22774,#22775);
#20269=AXIS2_PLACEMENT_3D('',#33955,#22777,#22778);
#20270=AXIS2_PLACEMENT_3D('',#33983,#22780,#22781);
#20271=AXIS2_PLACEMENT_3D('',#34024,#22783,#22784);
#20272=AXIS2_PLACEMENT_3D('',#34065,#22786,#22787);
#20273=AXIS2_PLACEMENT_3D('',#34094,#22789,#22790);
#20274=AXIS2_PLACEMENT_3D('',#34122,#22792,#22793);
#20275=AXIS2_PLACEMENT_3D('',#34150,#22795,#22796);
#20276=AXIS2_PLACEMENT_3D('',#34178,#22798,#22799);
#20277=AXIS2_PLACEMENT_3D('',#34219,#22801,#22802);
#20278=AXIS2_PLACEMENT_3D('',#34260,#22804,#22805);
#20279=AXIS2_PLACEMENT_3D('',#34288,#22807,#22808);
#20280=AXIS2_PLACEMENT_3D('',#34315,#22810,#22811);
#20281=AXIS2_PLACEMENT_3D('',#34357,#22813,#22814);
#20282=AXIS2_PLACEMENT_3D('',#34398,#22816,#22817);
#20283=AXIS2_PLACEMENT_3D('',#34427,#22819,#22820);
#20284=AXIS2_PLACEMENT_3D('',#34454,#22822,#22823);
#20285=AXIS2_PLACEMENT_3D('',#34495,#22825,#22826);
#20286=AXIS2_PLACEMENT_3D('',#34537,#22828,#22829);
#20287=AXIS2_PLACEMENT_3D('',#34565,#22831,#22832);
#20288=AXIS2_PLACEMENT_3D('',#34592,#22834,#22835);
#20289=AXIS2_PLACEMENT_3D('',#34633,#22837,#22838);
#20290=AXIS2_PLACEMENT_3D('',#34662,#22840,#22841);
#20291=AXIS2_PLACEMENT_3D('',#34704,#22843,#22844);
#20292=AXIS2_PLACEMENT_3D('',#34731,#22846,#22847);
#20293=AXIS2_PLACEMENT_3D('',#34772,#22849,#22850);
#20294=AXIS2_PLACEMENT_3D('',#34801,#22852,#22853);
#20295=AXIS2_PLACEMENT_3D('',#34842,#22855,#22856);
#20296=AXIS2_PLACEMENT_3D('',#34884,#22858,#22859);
#20297=AXIS2_PLACEMENT_3D('',#34912,#22861,#22862);
#20298=AXIS2_PLACEMENT_3D('',#34939,#22864,#22865);
#20299=AXIS2_PLACEMENT_3D('',#34980,#22867,#22868);
#20300=AXIS2_PLACEMENT_3D('',#35009,#22870,#22871);
#20301=AXIS2_PLACEMENT_3D('',#35038,#22873,#22874);
#20302=AXIS2_PLACEMENT_3D('',#35065,#22876,#22877);
#20303=AXIS2_PLACEMENT_3D('',#35106,#22879,#22880);
#20304=AXIS2_PLACEMENT_3D('',#35135,#22882,#22883);
#20305=AXIS2_PLACEMENT_3D('',#35176,#22885,#22886);
#20306=AXIS2_PLACEMENT_3D('',#35218,#22888,#22889);
#20307=AXIS2_PLACEMENT_3D('',#35246,#22891,#22892);
#20308=AXIS2_PLACEMENT_3D('',#35273,#22894,#22895);
#20309=AXIS2_PLACEMENT_3D('',#35314,#22897,#22898);
#20310=AXIS2_PLACEMENT_3D('',#35343,#22900,#22901);
#20311=AXIS2_PLACEMENT_3D('',#35372,#22903,#22904);
#20312=AXIS2_PLACEMENT_3D('',#35399,#22906,#22907);
#20313=AXIS2_PLACEMENT_3D('',#35427,#22909,#22910);
#20314=AXIS2_PLACEMENT_3D('',#35456,#22912,#22913);
#20315=AXIS2_PLACEMENT_3D('',#35497,#22915,#22916);
#20316=AXIS2_PLACEMENT_3D('',#35500,#22919,#22920);
#20317=AXIS2_PLACEMENT_3D('',#35502,#22922,#22923);
#20318=AXIS2_PLACEMENT_3D('',#35504,#22925,#22926);
#20319=AXIS2_PLACEMENT_3D('',#35505,#22927,#22928);
#20320=AXIS2_PLACEMENT_3D('',#35623,#22929,#22930);
#20321=AXIS2_PLACEMENT_3D('',#35625,#22931,#22932);
#20322=AXIS2_PLACEMENT_3D('',#37934,#22933,#22934);
#20323=AXIS2_PLACEMENT_3D('',#38051,#22935,#22936);
#20324=AXIS2_PLACEMENT_3D('',#38052,#22937,#22938);
#20325=AXIS2_PLACEMENT_3D('',#40130,#22939,#22940);
#20326=AXIS2_PLACEMENT_3D('',#40245,#22941,#22942);
#20327=AXIS2_PLACEMENT_3D('',#40247,#22943,#22944);
#20328=AXIS2_PLACEMENT_3D('',#41363,#22945,#22946);
#20329=AXIS2_PLACEMENT_3D('',#41480,#22947,#22948);
#20330=AXIS2_PLACEMENT_3D('',#41481,#22949,#22950);
#20331=AXIS2_PLACEMENT_3D('',#42360,#22951,#22952);
#20332=AXIS2_PLACEMENT_3D('',#42361,#22953,#22954);
#20333=AXIS2_PLACEMENT_3D('',#42362,#22955,#22956);
#20334=AXIS2_PLACEMENT_3D('',#42365,#22957,#22958);
#20335=AXIS2_PLACEMENT_3D('',#42397,#22959,#22960);
#20336=AXIS2_PLACEMENT_3D('',#42547,#22962,#22963);
#20337=AXIS2_PLACEMENT_3D('',#42550,#22965,#22966);
#20338=AXIS2_PLACEMENT_3D('',#42681,#22967,#22968);
#20339=AXIS2_PLACEMENT_3D('',#42682,#22969,#22970);
#20340=AXIS2_PLACEMENT_3D('',#42683,#22971,#22972);
#20341=AXIS2_PLACEMENT_3D('',#42685,#22973,#22974);
#20342=AXIS2_PLACEMENT_3D('',#42691,#22975,#22976);
#20343=AXIS2_PLACEMENT_3D('',#42692,#22977,#22978);
#20344=AXIS2_PLACEMENT_3D('',#42694,#22979,#22980);
#20345=AXIS2_PLACEMENT_3D('',#42700,#22981,#22982);
#20346=AXIS2_PLACEMENT_3D('',#42701,#22983,#22984);
#20347=AXIS2_PLACEMENT_3D('',#42703,#22985,#22986);
#20348=AXIS2_PLACEMENT_3D('',#42708,#22987,#22988);
#20349=AXIS2_PLACEMENT_3D('',#42710,#22989,#22990);
#20350=AXIS2_PLACEMENT_3D('',#42715,#22991,#22992);
#20351=AXIS2_PLACEMENT_3D('',#42717,#22993,#22994);
#20352=AXIS2_PLACEMENT_3D('',#42749,#22995,#22996);
#20353=AXIS2_PLACEMENT_3D('',#42899,#22998,#22999);
#20354=AXIS2_PLACEMENT_3D('',#42902,#23001,#23002);
#20355=AXIS2_PLACEMENT_3D('',#43012,#23003,#23004);
#20356=AXIS2_PLACEMENT_3D('',#43013,#23005,#23006);
#20357=AXIS2_PLACEMENT_3D('',#43014,#23007,#23008);
#20358=AXIS2_PLACEMENT_3D('',#43016,#23009,#23010);
#20359=AXIS2_PLACEMENT_3D('',#43022,#23011,#23012);
#20360=AXIS2_PLACEMENT_3D('',#43023,#23013,#23014);
#20361=AXIS2_PLACEMENT_3D('',#43025,#23015,#23016);
#20362=AXIS2_PLACEMENT_3D('',#43030,#23017,#23018);
#20363=AXIS2_PLACEMENT_3D('',#43032,#23019,#23020);
#20364=AXIS2_PLACEMENT_3D('',#43037,#23021,#23022);
#20365=AXIS2_PLACEMENT_3D('',#43039,#23023,#23024);
#20366=AXIS2_PLACEMENT_3D('',#43071,#23025,#23026);
#20367=AXIS2_PLACEMENT_3D('',#43221,#23028,#23029);
#20368=AXIS2_PLACEMENT_3D('',#43224,#23031,#23032);
#20369=AXIS2_PLACEMENT_3D('',#43334,#23033,#23034);
#20370=AXIS2_PLACEMENT_3D('',#43335,#23035,#23036);
#20371=AXIS2_PLACEMENT_3D('',#43336,#23037,#23038);
#20372=AXIS2_PLACEMENT_3D('',#43338,#23039,#23040);
#20373=AXIS2_PLACEMENT_3D('',#43344,#23041,#23042);
#20374=AXIS2_PLACEMENT_3D('',#43345,#23043,#23044);
#20375=AXIS2_PLACEMENT_3D('',#43347,#23045,#23046);
#20376=AXIS2_PLACEMENT_3D('',#43352,#23047,#23048);
#20377=AXIS2_PLACEMENT_3D('',#43354,#23049,#23050);
#20378=AXIS2_PLACEMENT_3D('',#43359,#23051,#23052);
#20379=AXIS2_PLACEMENT_3D('',#43361,#23053,#23054);
#20380=AXIS2_PLACEMENT_3D('',#43393,#23055,#23056);
#20381=AXIS2_PLACEMENT_3D('',#43543,#23058,#23059);
#20382=AXIS2_PLACEMENT_3D('',#43546,#23061,#23062);
#20383=AXIS2_PLACEMENT_3D('',#43656,#23063,#23064);
#20384=AXIS2_PLACEMENT_3D('',#43657,#23065,#23066);
#20385=AXIS2_PLACEMENT_3D('',#43658,#23067,#23068);
#20386=AXIS2_PLACEMENT_3D('',#43660,#23069,#23070);
#20387=AXIS2_PLACEMENT_3D('',#43666,#23071,#23072);
#20388=AXIS2_PLACEMENT_3D('',#43667,#23073,#23074);
#20389=AXIS2_PLACEMENT_3D('',#43669,#23075,#23076);
#20390=AXIS2_PLACEMENT_3D('',#43674,#23077,#23078);
#20391=AXIS2_PLACEMENT_3D('',#43676,#23079,#23080);
#20392=AXIS2_PLACEMENT_3D('',#43681,#23081,#23082);
#20393=AXIS2_PLACEMENT_3D('',#43683,#23083,#23084);
#20394=AXIS2_PLACEMENT_3D('',#43715,#23085,#23086);
#20395=AXIS2_PLACEMENT_3D('',#43878,#23088,#23089);
#20396=AXIS2_PLACEMENT_3D('',#43881,#23091,#23092);
#20397=AXIS2_PLACEMENT_3D('',#43991,#23093,#23094);
#20398=AXIS2_PLACEMENT_3D('',#43992,#23095,#23096);
#20399=AXIS2_PLACEMENT_3D('',#43993,#23097,#23098);
#20400=AXIS2_PLACEMENT_3D('',#43995,#23099,#23100);
#20401=AXIS2_PLACEMENT_3D('',#44001,#23101,#23102);
#20402=AXIS2_PLACEMENT_3D('',#44002,#23103,#23104);
#20403=AXIS2_PLACEMENT_3D('',#44004,#23105,#23106);
#20404=AXIS2_PLACEMENT_3D('',#44009,#23107,#23108);
#20405=AXIS2_PLACEMENT_3D('',#44011,#23109,#23110);
#20406=AXIS2_PLACEMENT_3D('',#44016,#23111,#23112);
#20407=AXIS2_PLACEMENT_3D('',#44018,#23113,#23114);
#20408=AXIS2_PLACEMENT_3D('',#44050,#23115,#23116);
#20409=AXIS2_PLACEMENT_3D('',#44200,#23118,#23119);
#20410=AXIS2_PLACEMENT_3D('',#44203,#23121,#23122);
#20411=AXIS2_PLACEMENT_3D('',#44313,#23123,#23124);
#20412=AXIS2_PLACEMENT_3D('',#44314,#23125,#23126);
#20413=AXIS2_PLACEMENT_3D('',#44315,#23127,#23128);
#20414=AXIS2_PLACEMENT_3D('',#44317,#23129,#23130);
#20415=AXIS2_PLACEMENT_3D('',#44323,#23131,#23132);
#20416=AXIS2_PLACEMENT_3D('',#44324,#23133,#23134);
#20417=AXIS2_PLACEMENT_3D('',#44326,#23135,#23136);
#20418=AXIS2_PLACEMENT_3D('',#44331,#23137,#23138);
#20419=AXIS2_PLACEMENT_3D('',#44333,#23139,#23140);
#20420=AXIS2_PLACEMENT_3D('',#44338,#23141,#23142);
#20421=AXIS2_PLACEMENT_3D('',#44340,#23143,#23144);
#20422=AXIS2_PLACEMENT_3D('',#44372,#23145,#23146);
#20423=AXIS2_PLACEMENT_3D('',#44522,#23148,#23149);
#20424=AXIS2_PLACEMENT_3D('',#44525,#23151,#23152);
#20425=AXIS2_PLACEMENT_3D('',#44635,#23153,#23154);
#20426=AXIS2_PLACEMENT_3D('',#44636,#23155,#23156);
#20427=AXIS2_PLACEMENT_3D('',#44637,#23157,#23158);
#20428=AXIS2_PLACEMENT_3D('',#44639,#23159,#23160);
#20429=AXIS2_PLACEMENT_3D('',#44645,#23161,#23162);
#20430=AXIS2_PLACEMENT_3D('',#44646,#23163,#23164);
#20431=AXIS2_PLACEMENT_3D('',#44648,#23165,#23166);
#20432=AXIS2_PLACEMENT_3D('',#44653,#23167,#23168);
#20433=AXIS2_PLACEMENT_3D('',#44655,#23169,#23170);
#20434=AXIS2_PLACEMENT_3D('',#44660,#23171,#23172);
#20435=AXIS2_PLACEMENT_3D('',#44663,#23173,#23174);
#20436=AXIS2_PLACEMENT_3D('',#44664,#23175,#23176);
#20437=AXIS2_PLACEMENT_3D('',#44696,#23177,#23178);
#20438=AXIS2_PLACEMENT_3D('',#44848,#23180,#23181);
#20439=AXIS2_PLACEMENT_3D('',#44851,#23183,#23184);
#20440=AXIS2_PLACEMENT_3D('',#44961,#23185,#23186);
#20441=AXIS2_PLACEMENT_3D('',#44963,#23187,#23188);
#20442=AXIS2_PLACEMENT_3D('',#44964,#23189,#23190);
#20443=AXIS2_PLACEMENT_3D('',#44965,#23191,#23192);
#20444=AXIS2_PLACEMENT_3D('',#44967,#23193,#23194);
#20445=AXIS2_PLACEMENT_3D('',#44973,#23195,#23196);
#20446=AXIS2_PLACEMENT_3D('',#44974,#23197,#23198);
#20447=AXIS2_PLACEMENT_3D('',#44976,#23199,#23200);
#20448=AXIS2_PLACEMENT_3D('',#44981,#23201,#23202);
#20449=AXIS2_PLACEMENT_3D('',#44983,#23203,#23204);
#20450=AXIS2_PLACEMENT_3D('',#44988,#23205,#23206);
#20451=AXIS2_PLACEMENT_3D('',#44990,#23207,#23208);
#20452=AXIS2_PLACEMENT_3D('',#45022,#23209,#23210);
#20453=AXIS2_PLACEMENT_3D('',#45172,#23212,#23213);
#20454=AXIS2_PLACEMENT_3D('',#45175,#23215,#23216);
#20455=AXIS2_PLACEMENT_3D('',#45285,#23217,#23218);
#20456=AXIS2_PLACEMENT_3D('',#45286,#23219,#23220);
#20457=AXIS2_PLACEMENT_3D('',#45287,#23221,#23222);
#20458=AXIS2_PLACEMENT_3D('',#45289,#23223,#23224);
#20459=AXIS2_PLACEMENT_3D('',#45295,#23225,#23226);
#20460=AXIS2_PLACEMENT_3D('',#45296,#23227,#23228);
#20461=AXIS2_PLACEMENT_3D('',#45298,#23229,#23230);
#20462=AXIS2_PLACEMENT_3D('',#45303,#23231,#23232);
#20463=AXIS2_PLACEMENT_3D('',#45305,#23233,#23234);
#20464=AXIS2_PLACEMENT_3D('',#45310,#23235,#23236);
#20465=AXIS2_PLACEMENT_3D('',#45312,#23237,#23238);
#20466=AXIS2_PLACEMENT_3D('',#45344,#23239,#23240);
#20467=AXIS2_PLACEMENT_3D('',#45494,#23242,#23243);
#20468=AXIS2_PLACEMENT_3D('',#45497,#23245,#23246);
#20469=AXIS2_PLACEMENT_3D('',#45607,#23247,#23248);
#20470=AXIS2_PLACEMENT_3D('',#45608,#23249,#23250);
#20471=AXIS2_PLACEMENT_3D('',#45609,#23251,#23252);
#20472=AXIS2_PLACEMENT_3D('',#45611,#23253,#23254);
#20473=AXIS2_PLACEMENT_3D('',#45617,#23255,#23256);
#20474=AXIS2_PLACEMENT_3D('',#45618,#23257,#23258);
#20475=AXIS2_PLACEMENT_3D('',#45620,#23259,#23260);
#20476=AXIS2_PLACEMENT_3D('',#45625,#23261,#23262);
#20477=AXIS2_PLACEMENT_3D('',#45627,#23263,#23264);
#20478=AXIS2_PLACEMENT_3D('',#45632,#23265,#23266);
#20479=AXIS2_PLACEMENT_3D('',#45634,#23267,#23268);
#20480=AXIS2_PLACEMENT_3D('',#45666,#23269,#23270);
#20481=AXIS2_PLACEMENT_3D('',#45816,#23272,#23273);
#20482=AXIS2_PLACEMENT_3D('',#45819,#23275,#23276);
#20483=AXIS2_PLACEMENT_3D('',#45929,#23277,#23278);
#20484=AXIS2_PLACEMENT_3D('',#45930,#23279,#23280);
#20485=AXIS2_PLACEMENT_3D('',#45931,#23281,#23282);
#20486=AXIS2_PLACEMENT_3D('',#45933,#23283,#23284);
#20487=AXIS2_PLACEMENT_3D('',#45942,#23285,#23286);
#20488=AXIS2_PLACEMENT_3D('',#45943,#23287,#23288);
#20489=AXIS2_PLACEMENT_3D('',#45945,#23289,#23290);
#20490=AXIS2_PLACEMENT_3D('',#45950,#23291,#23292);
#20491=AXIS2_PLACEMENT_3D('',#45952,#23293,#23294);
#20492=AXIS2_PLACEMENT_3D('',#45960,#23295,#23296);
#20493=AXIS2_PLACEMENT_3D('',#45962,#23297,#23298);
#20494=AXIS2_PLACEMENT_3D('',#45994,#23299,#23300);
#20495=AXIS2_PLACEMENT_3D('',#46144,#23302,#23303);
#20496=AXIS2_PLACEMENT_3D('',#46147,#23305,#23306);
#20497=AXIS2_PLACEMENT_3D('',#46257,#23307,#23308);
#20498=AXIS2_PLACEMENT_3D('',#46258,#23309,#23310);
#20499=AXIS2_PLACEMENT_3D('',#46259,#23311,#23312);
#20500=AXIS2_PLACEMENT_3D('',#46261,#23313,#23314);
#20501=AXIS2_PLACEMENT_3D('',#46267,#23315,#23316);
#20502=AXIS2_PLACEMENT_3D('',#46268,#23317,#23318);
#20503=AXIS2_PLACEMENT_3D('',#46270,#23319,#23320);
#20504=AXIS2_PLACEMENT_3D('',#46275,#23321,#23322);
#20505=AXIS2_PLACEMENT_3D('',#46277,#23323,#23324);
#20506=AXIS2_PLACEMENT_3D('',#46282,#23325,#23326);
#20507=AXIS2_PLACEMENT_3D('',#46284,#23327,#23328);
#20508=AXIS2_PLACEMENT_3D('',#46316,#23329,#23330);
#20509=AXIS2_PLACEMENT_3D('',#46466,#23332,#23333);
#20510=AXIS2_PLACEMENT_3D('',#46469,#23335,#23336);
#20511=AXIS2_PLACEMENT_3D('',#46579,#23337,#23338);
#20512=AXIS2_PLACEMENT_3D('',#46580,#23339,#23340);
#20513=AXIS2_PLACEMENT_3D('',#46581,#23341,#23342);
#20514=AXIS2_PLACEMENT_3D('',#46583,#23343,#23344);
#20515=AXIS2_PLACEMENT_3D('',#46589,#23345,#23346);
#20516=AXIS2_PLACEMENT_3D('',#46590,#23347,#23348);
#20517=AXIS2_PLACEMENT_3D('',#46592,#23349,#23350);
#20518=AXIS2_PLACEMENT_3D('',#46597,#23351,#23352);
#20519=AXIS2_PLACEMENT_3D('',#46599,#23353,#23354);
#20520=AXIS2_PLACEMENT_3D('',#46604,#23355,#23356);
#20521=AXIS2_PLACEMENT_3D('',#46606,#23357,#23358);
#20522=AXIS2_PLACEMENT_3D('',#46638,#23359,#23360);
#20523=AXIS2_PLACEMENT_3D('',#46788,#23362,#23363);
#20524=AXIS2_PLACEMENT_3D('',#46791,#23365,#23366);
#20525=AXIS2_PLACEMENT_3D('',#46901,#23367,#23368);
#20526=AXIS2_PLACEMENT_3D('',#46902,#23369,#23370);
#20527=AXIS2_PLACEMENT_3D('',#46903,#23371,#23372);
#20528=AXIS2_PLACEMENT_3D('',#46905,#23373,#23374);
#20529=AXIS2_PLACEMENT_3D('',#46911,#23375,#23376);
#20530=AXIS2_PLACEMENT_3D('',#46912,#23377,#23378);
#20531=AXIS2_PLACEMENT_3D('',#46914,#23379,#23380);
#20532=AXIS2_PLACEMENT_3D('',#46919,#23381,#23382);
#20533=AXIS2_PLACEMENT_3D('',#46921,#23383,#23384);
#20534=AXIS2_PLACEMENT_3D('',#47067,#23386,#23387);
#20535=AXIS2_PLACEMENT_3D('',#47068,#23388,#23389);
#20536=AXIS2_PLACEMENT_3D('',#47070,#23390,#23391);
#20537=AXIS2_PLACEMENT_3D('',#47096,#23392,#23393);
#20538=AXIS2_PLACEMENT_3D('',#47098,#23394,#23395);
#20539=AXIS2_PLACEMENT_3D('',#47217,#23397,#23398);
#20540=AXIS2_PLACEMENT_3D('',#47218,#23399,#23400);
#20541=AXIS2_PLACEMENT_3D('',#47219,#23401,#23402);
#20542=AXIS2_PLACEMENT_3D('',#47220,#23403,#23404);
#20543=AXIS2_PLACEMENT_3D('',#47221,#23405,#23406);
#20544=AXIS2_PLACEMENT_3D('',#47222,#23407,#23408);
#20545=AXIS2_PLACEMENT_3D('',#47223,#23409,#23410);
#20546=AXIS2_PLACEMENT_3D('',#47225,#23411,#23412);
#20547=AXIS2_PLACEMENT_3D('',#47226,#23413,#23414);
#20548=AXIS2_PLACEMENT_3D('',#47228,#23416,#23417);
#20549=AXIS2_PLACEMENT_3D('',#47230,#23419,#23420);
#20550=AXIS2_PLACEMENT_3D('',#47232,#23422,#23423);
#20551=AXIS2_PLACEMENT_3D('',#47233,#23424,#23425);
#20552=AXIS2_PLACEMENT_3D('',#47234,#23426,#23427);
#20553=AXIS2_PLACEMENT_3D('',#47236,#23428,#23429);
#20554=AXIS2_PLACEMENT_3D('',#47238,#23431,#23432);
#22405=DIRECTION('axis',(0.,0.,1.));
#22406=DIRECTION('refdir',(1.,0.,0.));
#22407=DIRECTION('center_axis',(1.,0.,0.));
#22408=DIRECTION('ref_axis',(0.,1.,0.));
#22409=DIRECTION('',(-1.,0.,0.));
#22410=DIRECTION('center_axis',(-1.,0.,0.));
#22411=DIRECTION('ref_axis',(0.,1.,0.));
#22412=DIRECTION('',(-1.,0.,0.));
#22413=DIRECTION('center_axis',(1.,0.,0.));
#22414=DIRECTION('ref_axis',(0.,1.,0.));
#22415=DIRECTION('',(-1.,0.,0.));
#22416=DIRECTION('center_axis',(-1.,0.,0.));
#22417=DIRECTION('ref_axis',(0.,1.,0.));
#22418=DIRECTION('',(-1.,0.,0.));
#22419=DIRECTION('center_axis',(-1.,0.,0.));
#22420=DIRECTION('ref_axis',(0.,1.,0.));
#22421=DIRECTION('center_axis',(-1.,0.,0.));
#22422=DIRECTION('ref_axis',(0.,1.,0.));
#22423=DIRECTION('',(1.,0.,0.));
#22424=DIRECTION('center_axis',(1.,0.,0.));
#22425=DIRECTION('ref_axis',(0.,1.,0.));
#22426=DIRECTION('center_axis',(-1.,0.,0.));
#22427=DIRECTION('ref_axis',(0.,1.,0.));
#22428=DIRECTION('',(1.,0.,0.));
#22429=DIRECTION('center_axis',(1.,0.,0.));
#22430=DIRECTION('ref_axis',(0.,1.,0.));
#22431=DIRECTION('',(-1.,0.,0.));
#22432=DIRECTION('center_axis',(-1.,0.,0.));
#22433=DIRECTION('ref_axis',(0.,1.,0.));
#22434=DIRECTION('center_axis',(1.,0.,0.));
#22435=DIRECTION('ref_axis',(0.,1.,0.));
#22436=DIRECTION('',(-1.,0.,0.));
#22437=DIRECTION('center_axis',(1.,0.,0.));
#22438=DIRECTION('ref_axis',(0.,1.,0.));
#22439=DIRECTION('',(-1.,0.,0.));
#22440=DIRECTION('center_axis',(1.,0.,0.));
#22441=DIRECTION('ref_axis',(0.,1.,0.));
#22442=DIRECTION('',(-1.,0.,0.));
#22443=DIRECTION('center_axis',(1.,0.,0.));
#22444=DIRECTION('ref_axis',(0.,1.,0.));
#22445=DIRECTION('',(-1.,0.,0.));
#22446=DIRECTION('center_axis',(1.,0.,0.));
#22447=DIRECTION('ref_axis',(0.,1.,0.));
#22448=DIRECTION('',(-1.,0.,0.));
#22449=DIRECTION('center_axis',(1.,0.,0.));
#22450=DIRECTION('ref_axis',(0.,1.,0.));
#22451=DIRECTION('',(-1.,0.,0.));
#22452=DIRECTION('center_axis',(1.,0.,0.));
#22453=DIRECTION('ref_axis',(0.,1.,0.));
#22454=DIRECTION('',(-1.,0.,0.));
#22455=DIRECTION('center_axis',(1.,0.,0.));
#22456=DIRECTION('ref_axis',(0.,1.,0.));
#22457=DIRECTION('',(-1.,0.,0.));
#22458=DIRECTION('center_axis',(1.,0.,0.));
#22459=DIRECTION('ref_axis',(0.,1.,0.));
#22460=DIRECTION('',(-1.,0.,0.));
#22461=DIRECTION('center_axis',(1.,0.,0.));
#22462=DIRECTION('ref_axis',(0.,1.,0.));
#22463=DIRECTION('',(-1.,0.,0.));
#22464=DIRECTION('center_axis',(1.,0.,0.));
#22465=DIRECTION('ref_axis',(0.,1.,0.));
#22466=DIRECTION('',(-1.,0.,0.));
#22467=DIRECTION('center_axis',(1.,0.,0.));
#22468=DIRECTION('ref_axis',(0.,1.,0.));
#22469=DIRECTION('',(-1.,0.,0.));
#22470=DIRECTION('center_axis',(1.,0.,0.));
#22471=DIRECTION('ref_axis',(0.,1.,0.));
#22472=DIRECTION('',(-1.,0.,0.));
#22473=DIRECTION('center_axis',(1.,0.,0.));
#22474=DIRECTION('ref_axis',(0.,1.,0.));
#22475=DIRECTION('',(-1.,0.,0.));
#22476=DIRECTION('center_axis',(1.,0.,0.));
#22477=DIRECTION('ref_axis',(0.,1.,0.));
#22478=DIRECTION('',(-1.,0.,0.));
#22479=DIRECTION('center_axis',(1.,0.,0.));
#22480=DIRECTION('ref_axis',(0.,1.,0.));
#22481=DIRECTION('',(-1.,0.,0.));
#22482=DIRECTION('center_axis',(1.,0.,0.));
#22483=DIRECTION('ref_axis',(0.,1.,0.));
#22484=DIRECTION('',(-1.,0.,0.));
#22485=DIRECTION('center_axis',(1.,0.,0.));
#22486=DIRECTION('ref_axis',(0.,1.,0.));
#22487=DIRECTION('',(-1.,0.,0.));
#22488=DIRECTION('center_axis',(1.,0.,0.));
#22489=DIRECTION('ref_axis',(0.,1.,0.));
#22490=DIRECTION('',(-1.,0.,0.));
#22491=DIRECTION('center_axis',(1.,0.,0.));
#22492=DIRECTION('ref_axis',(0.,1.,0.));
#22493=DIRECTION('',(-1.,0.,0.));
#22494=DIRECTION('center_axis',(1.,0.,0.));
#22495=DIRECTION('ref_axis',(0.,1.,0.));
#22496=DIRECTION('',(-1.,0.,0.));
#22497=DIRECTION('center_axis',(1.,0.,0.));
#22498=DIRECTION('ref_axis',(0.,1.,0.));
#22499=DIRECTION('',(-1.,0.,0.));
#22500=DIRECTION('center_axis',(1.,0.,0.));
#22501=DIRECTION('ref_axis',(0.,1.,0.));
#22502=DIRECTION('',(-1.,0.,0.));
#22503=DIRECTION('center_axis',(1.,0.,0.));
#22504=DIRECTION('ref_axis',(0.,1.,0.));
#22505=DIRECTION('',(-1.,0.,0.));
#22506=DIRECTION('center_axis',(1.,0.,0.));
#22507=DIRECTION('ref_axis',(0.,1.,0.));
#22508=DIRECTION('',(-1.,0.,0.));
#22509=DIRECTION('center_axis',(1.,0.,0.));
#22510=DIRECTION('ref_axis',(0.,1.,0.));
#22511=DIRECTION('',(-1.,0.,0.));
#22512=DIRECTION('center_axis',(1.,0.,0.));
#22513=DIRECTION('ref_axis',(0.,1.,0.));
#22514=DIRECTION('',(-1.,0.,0.));
#22515=DIRECTION('center_axis',(1.,0.,0.));
#22516=DIRECTION('ref_axis',(0.,1.,0.));
#22517=DIRECTION('',(-1.,0.,0.));
#22518=DIRECTION('center_axis',(1.,0.,0.));
#22519=DIRECTION('ref_axis',(0.,1.,0.));
#22520=DIRECTION('',(-1.,0.,0.));
#22521=DIRECTION('center_axis',(1.,0.,0.));
#22522=DIRECTION('ref_axis',(0.,1.,0.));
#22523=DIRECTION('',(-1.,0.,0.));
#22524=DIRECTION('center_axis',(1.,0.,0.));
#22525=DIRECTION('ref_axis',(0.,1.,0.));
#22526=DIRECTION('',(-1.,0.,0.));
#22527=DIRECTION('center_axis',(1.,0.,0.));
#22528=DIRECTION('ref_axis',(0.,1.,0.));
#22529=DIRECTION('',(-1.,0.,0.));
#22530=DIRECTION('center_axis',(1.,0.,0.));
#22531=DIRECTION('ref_axis',(0.,1.,0.));
#22532=DIRECTION('',(-1.,0.,0.));
#22533=DIRECTION('center_axis',(1.,0.,0.));
#22534=DIRECTION('ref_axis',(0.,1.,0.));
#22535=DIRECTION('',(-1.,0.,0.));
#22536=DIRECTION('center_axis',(1.,0.,0.));
#22537=DIRECTION('ref_axis',(0.,1.,0.));
#22538=DIRECTION('',(-1.,0.,0.));
#22539=DIRECTION('center_axis',(1.,0.,0.));
#22540=DIRECTION('ref_axis',(0.,1.,0.));
#22541=DIRECTION('',(-1.,0.,0.));
#22542=DIRECTION('center_axis',(1.,0.,0.));
#22543=DIRECTION('ref_axis',(0.,1.,0.));
#22544=DIRECTION('',(-1.,0.,0.));
#22545=DIRECTION('center_axis',(1.,0.,0.));
#22546=DIRECTION('ref_axis',(0.,1.,0.));
#22547=DIRECTION('',(-1.,0.,0.));
#22548=DIRECTION('center_axis',(1.,0.,0.));
#22549=DIRECTION('ref_axis',(0.,1.,0.));
#22550=DIRECTION('',(-1.,0.,0.));
#22551=DIRECTION('center_axis',(1.,0.,0.));
#22552=DIRECTION('ref_axis',(0.,1.,0.));
#22553=DIRECTION('',(-1.,0.,0.));
#22554=DIRECTION('center_axis',(1.,0.,0.));
#22555=DIRECTION('ref_axis',(0.,1.,0.));
#22556=DIRECTION('',(-1.,0.,0.));
#22557=DIRECTION('center_axis',(1.,0.,0.));
#22558=DIRECTION('ref_axis',(0.,1.,0.));
#22559=DIRECTION('',(-1.,0.,0.));
#22560=DIRECTION('center_axis',(1.,0.,0.));
#22561=DIRECTION('ref_axis',(0.,1.,0.));
#22562=DIRECTION('',(-1.,0.,0.));
#22563=DIRECTION('center_axis',(1.,0.,0.));
#22564=DIRECTION('ref_axis',(0.,1.,0.));
#22565=DIRECTION('',(-1.,0.,0.));
#22566=DIRECTION('center_axis',(1.,0.,0.));
#22567=DIRECTION('ref_axis',(0.,1.,0.));
#22568=DIRECTION('',(-1.,0.,0.));
#22569=DIRECTION('center_axis',(1.,0.,0.));
#22570=DIRECTION('ref_axis',(0.,1.,0.));
#22571=DIRECTION('',(-1.,0.,0.));
#22572=DIRECTION('center_axis',(1.,0.,0.));
#22573=DIRECTION('ref_axis',(0.,1.,0.));
#22574=DIRECTION('',(-1.,0.,0.));
#22575=DIRECTION('center_axis',(1.,0.,0.));
#22576=DIRECTION('ref_axis',(0.,1.,0.));
#22577=DIRECTION('',(-1.,0.,0.));
#22578=DIRECTION('center_axis',(1.,0.,0.));
#22579=DIRECTION('ref_axis',(0.,1.,0.));
#22580=DIRECTION('',(-1.,0.,0.));
#22581=DIRECTION('center_axis',(1.,0.,0.));
#22582=DIRECTION('ref_axis',(0.,1.,0.));
#22583=DIRECTION('',(-1.,0.,0.));
#22584=DIRECTION('center_axis',(1.,0.,0.));
#22585=DIRECTION('ref_axis',(0.,1.,0.));
#22586=DIRECTION('',(-1.,0.,0.));
#22587=DIRECTION('center_axis',(1.,0.,0.));
#22588=DIRECTION('ref_axis',(0.,1.,0.));
#22589=DIRECTION('',(-1.,0.,0.));
#22590=DIRECTION('center_axis',(1.,0.,0.));
#22591=DIRECTION('ref_axis',(0.,1.,0.));
#22592=DIRECTION('',(-1.,0.,0.));
#22593=DIRECTION('center_axis',(1.,0.,0.));
#22594=DIRECTION('ref_axis',(0.,1.,0.));
#22595=DIRECTION('',(-1.,0.,0.));
#22596=DIRECTION('center_axis',(1.,0.,0.));
#22597=DIRECTION('ref_axis',(0.,1.,0.));
#22598=DIRECTION('',(-1.,0.,0.));
#22599=DIRECTION('center_axis',(1.,0.,0.));
#22600=DIRECTION('ref_axis',(0.,1.,0.));
#22601=DIRECTION('',(-1.,0.,0.));
#22602=DIRECTION('center_axis',(1.,0.,0.));
#22603=DIRECTION('ref_axis',(0.,1.,0.));
#22604=DIRECTION('',(-1.,0.,0.));
#22605=DIRECTION('center_axis',(1.,0.,0.));
#22606=DIRECTION('ref_axis',(0.,1.,0.));
#22607=DIRECTION('',(-1.,0.,0.));
#22608=DIRECTION('center_axis',(1.,0.,0.));
#22609=DIRECTION('ref_axis',(0.,1.,0.));
#22610=DIRECTION('',(-1.,0.,0.));
#22611=DIRECTION('center_axis',(1.,0.,0.));
#22612=DIRECTION('ref_axis',(0.,1.,0.));
#22613=DIRECTION('',(-1.,0.,0.));
#22614=DIRECTION('center_axis',(1.,0.,0.));
#22615=DIRECTION('ref_axis',(0.,1.,0.));
#22616=DIRECTION('',(-1.,0.,0.));
#22617=DIRECTION('center_axis',(1.,0.,0.));
#22618=DIRECTION('ref_axis',(0.,1.,0.));
#22619=DIRECTION('',(-1.,0.,0.));
#22620=DIRECTION('center_axis',(-1.,0.,0.));
#22621=DIRECTION('ref_axis',(0.,1.,0.));
#22622=DIRECTION('',(-1.,0.,0.));
#22623=DIRECTION('center_axis',(1.,0.,0.));
#22624=DIRECTION('ref_axis',(0.,1.,0.));
#22625=DIRECTION('center_axis',(-1.,0.,0.));
#22626=DIRECTION('ref_axis',(0.,1.,0.));
#22627=DIRECTION('center_axis',(1.,0.,0.));
#22628=DIRECTION('ref_axis',(0.,1.,0.));
#22629=DIRECTION('',(-1.,0.,0.));
#22630=DIRECTION('center_axis',(1.,0.,0.));
#22631=DIRECTION('ref_axis',(0.,1.,0.));
#22632=DIRECTION('',(-1.,0.,0.));
#22633=DIRECTION('center_axis',(1.,0.,0.));
#22634=DIRECTION('ref_axis',(0.,1.,0.));
#22635=DIRECTION('',(-1.,0.,0.));
#22636=DIRECTION('center_axis',(1.,0.,0.));
#22637=DIRECTION('ref_axis',(0.,1.,0.));
#22638=DIRECTION('',(-1.,0.,0.));
#22639=DIRECTION('center_axis',(1.,0.,0.));
#22640=DIRECTION('ref_axis',(0.,1.,0.));
#22641=DIRECTION('',(-1.,0.,0.));
#22642=DIRECTION('center_axis',(1.,0.,0.));
#22643=DIRECTION('ref_axis',(0.,1.,0.));
#22644=DIRECTION('',(-1.,0.,0.));
#22645=DIRECTION('center_axis',(1.,0.,0.));
#22646=DIRECTION('ref_axis',(0.,1.,0.));
#22647=DIRECTION('',(-1.,0.,0.));
#22648=DIRECTION('center_axis',(1.,0.,0.));
#22649=DIRECTION('ref_axis',(0.,1.,0.));
#22650=DIRECTION('',(-1.,0.,0.));
#22651=DIRECTION('center_axis',(1.,0.,0.));
#22652=DIRECTION('ref_axis',(0.,1.,0.));
#22653=DIRECTION('',(-1.,0.,0.));
#22654=DIRECTION('center_axis',(1.,0.,0.));
#22655=DIRECTION('ref_axis',(0.,1.,0.));
#22656=DIRECTION('',(-1.,0.,0.));
#22657=DIRECTION('center_axis',(1.,0.,0.));
#22658=DIRECTION('ref_axis',(0.,1.,0.));
#22659=DIRECTION('',(-1.,0.,0.));
#22660=DIRECTION('center_axis',(1.,0.,0.));
#22661=DIRECTION('ref_axis',(0.,1.,0.));
#22662=DIRECTION('',(-1.,0.,0.));
#22663=DIRECTION('center_axis',(1.,0.,0.));
#22664=DIRECTION('ref_axis',(0.,1.,0.));
#22665=DIRECTION('',(-1.,0.,0.));
#22666=DIRECTION('center_axis',(1.,0.,0.));
#22667=DIRECTION('ref_axis',(0.,1.,0.));
#22668=DIRECTION('',(-1.,0.,0.));
#22669=DIRECTION('center_axis',(1.,0.,0.));
#22670=DIRECTION('ref_axis',(0.,1.,0.));
#22671=DIRECTION('',(-1.,0.,0.));
#22672=DIRECTION('center_axis',(1.,0.,0.));
#22673=DIRECTION('ref_axis',(0.,-0.328007595378459,-0.944675085610942));
#22674=DIRECTION('',(1.,0.,0.));
#22675=DIRECTION('center_axis',(1.,0.,0.));
#22676=DIRECTION('ref_axis',(0.,1.,9.92840284004976E-14));
#22677=DIRECTION('center_axis',(1.,0.,0.));
#22678=DIRECTION('ref_axis',(0.,1.,9.92840284004976E-14));
#22679=DIRECTION('',(1.,0.,0.));
#22680=DIRECTION('center_axis',(1.,0.,0.));
#22681=DIRECTION('ref_axis',(0.,1.,9.92840284004976E-14));
#22682=DIRECTION('',(1.,0.,0.));
#22683=DIRECTION('center_axis',(1.,0.,0.));
#22684=DIRECTION('ref_axis',(0.,1.,9.92840284004976E-14));
#22685=DIRECTION('',(1.,0.,0.));
#22686=DIRECTION('center_axis',(1.,0.,0.));
#22687=DIRECTION('ref_axis',(0.,1.,9.92840284004976E-14));
#22688=DIRECTION('',(1.,0.,0.));
#22689=DIRECTION('center_axis',(1.,0.,0.));
#22690=DIRECTION('ref_axis',(0.,1.,9.92840284004976E-14));
#22691=DIRECTION('',(1.,0.,0.));
#22692=DIRECTION('center_axis',(1.,0.,0.));
#22693=DIRECTION('ref_axis',(0.,1.,9.92840284004976E-14));
#22694=DIRECTION('',(1.,0.,0.));
#22695=DIRECTION('center_axis',(1.,0.,0.));
#22696=DIRECTION('ref_axis',(0.,1.,9.92840284004976E-14));
#22697=DIRECTION('',(1.,0.,0.));
#22698=DIRECTION('center_axis',(1.,0.,0.));
#22699=DIRECTION('ref_axis',(0.,1.,9.92840284004976E-14));
#22700=DIRECTION('',(1.,0.,0.));
#22701=DIRECTION('center_axis',(1.,0.,0.));
#22702=DIRECTION('ref_axis',(0.,1.,9.92840284004976E-14));
#22703=DIRECTION('',(1.,0.,0.));
#22704=DIRECTION('center_axis',(1.,0.,0.));
#22705=DIRECTION('ref_axis',(0.,1.,9.92840284004976E-14));
#22706=DIRECTION('',(1.,0.,0.));
#22707=DIRECTION('center_axis',(1.,0.,0.));
#22708=DIRECTION('ref_axis',(0.,1.,9.92840284004976E-14));
#22709=DIRECTION('',(1.,0.,0.));
#22710=DIRECTION('center_axis',(1.,0.,0.));
#22711=DIRECTION('ref_axis',(0.,1.,9.92840284004976E-14));
#22712=DIRECTION('',(1.,0.,0.));
#22713=DIRECTION('center_axis',(1.,0.,0.));
#22714=DIRECTION('ref_axis',(0.,1.,9.92840284004976E-14));
#22715=DIRECTION('',(1.,0.,0.));
#22716=DIRECTION('center_axis',(1.,0.,0.));
#22717=DIRECTION('ref_axis',(0.,1.,9.92840284004976E-14));
#22718=DIRECTION('',(1.,0.,0.));
#22719=DIRECTION('center_axis',(1.,0.,0.));
#22720=DIRECTION('ref_axis',(0.,1.,9.92840284004976E-14));
#22721=DIRECTION('',(1.,0.,0.));
#22722=DIRECTION('center_axis',(1.,0.,0.));
#22723=DIRECTION('ref_axis',(0.,1.,-9.14588507257614E-13));
#22724=DIRECTION('',(1.,0.,0.));
#22725=DIRECTION('center_axis',(1.,0.,0.));
#22726=DIRECTION('ref_axis',(0.,1.,-9.14588507257614E-13));
#22727=DIRECTION('center_axis',(1.,0.,0.));
#22728=DIRECTION('ref_axis',(0.,1.,-9.14588507257614E-13));
#22729=DIRECTION('',(1.,0.,0.));
#22730=DIRECTION('center_axis',(1.,0.,0.));
#22731=DIRECTION('ref_axis',(0.,1.,-9.14588507257614E-13));
#22732=DIRECTION('center_axis',(1.,0.,0.));
#22733=DIRECTION('ref_axis',(0.,1.,-9.14588507257614E-13));
#22734=DIRECTION('',(1.,0.,0.));
#22735=DIRECTION('center_axis',(1.,0.,0.));
#22736=DIRECTION('ref_axis',(0.,1.,-9.14588507257614E-13));
#22737=DIRECTION('',(1.,0.,0.));
#22738=DIRECTION('center_axis',(1.,0.,0.));
#22739=DIRECTION('ref_axis',(0.,1.,-9.14588507257614E-13));
#22740=DIRECTION('',(1.,0.,0.));
#22741=DIRECTION('center_axis',(1.,0.,0.));
#22742=DIRECTION('ref_axis',(0.,1.,-9.14588507257614E-13));
#22743=DIRECTION('',(1.,0.,0.));
#22744=DIRECTION('center_axis',(1.,0.,0.));
#22745=DIRECTION('ref_axis',(0.,1.,-9.14588507257614E-13));
#22746=DIRECTION('',(1.,0.,0.));
#22747=DIRECTION('center_axis',(1.,0.,0.));
#22748=DIRECTION('ref_axis',(0.,1.,-9.14588507257614E-13));
#22749=DIRECTION('',(1.,0.,0.));
#22750=DIRECTION('center_axis',(1.,0.,0.));
#22751=DIRECTION('ref_axis',(0.,1.,-9.14588507257614E-13));
#22752=DIRECTION('',(1.,0.,0.));
#22753=DIRECTION('center_axis',(1.,0.,0.));
#22754=DIRECTION('ref_axis',(0.,1.,-9.14588507257614E-13));
#22755=DIRECTION('',(1.,0.,0.));
#22756=DIRECTION('center_axis',(1.,0.,0.));
#22757=DIRECTION('ref_axis',(0.,1.,-9.14588507257614E-13));
#22758=DIRECTION('',(1.,0.,0.));
#22759=DIRECTION('center_axis',(1.,0.,0.));
#22760=DIRECTION('ref_axis',(0.,1.,-9.14588507257614E-13));
#22761=DIRECTION('',(1.,0.,0.));
#22762=DIRECTION('center_axis',(1.,0.,0.));
#22763=DIRECTION('ref_axis',(0.,1.,-9.14588507257614E-13));
#22764=DIRECTION('',(1.,0.,0.));
#22765=DIRECTION('center_axis',(1.,0.,0.));
#22766=DIRECTION('ref_axis',(0.,1.,-9.14588507257614E-13));
#22767=DIRECTION('',(1.,0.,0.));
#22768=DIRECTION('center_axis',(1.,0.,0.));
#22769=DIRECTION('ref_axis',(0.,1.,-9.14588507257614E-13));
#22770=DIRECTION('',(1.,0.,0.));
#22771=DIRECTION('center_axis',(1.,0.,0.));
#22772=DIRECTION('ref_axis',(0.,1.,-9.14588507257614E-13));
#22773=DIRECTION('',(1.,0.,0.));
#22774=DIRECTION('center_axis',(1.,0.,0.));
#22775=DIRECTION('ref_axis',(0.,1.,-9.14588507257614E-13));
#22776=DIRECTION('',(1.,0.,0.));
#22777=DIRECTION('center_axis',(1.,0.,0.));
#22778=DIRECTION('ref_axis',(0.,1.,-9.14588507257614E-13));
#22779=DIRECTION('',(1.,0.,0.));
#22780=DIRECTION('center_axis',(1.,0.,0.));
#22781=DIRECTION('ref_axis',(0.,1.,-9.14588507257614E-13));
#22782=DIRECTION('',(1.,0.,0.));
#22783=DIRECTION('center_axis',(1.,0.,0.));
#22784=DIRECTION('ref_axis',(0.,1.,-9.14588507257614E-13));
#22785=DIRECTION('',(1.,0.,0.));
#22786=DIRECTION('center_axis',(1.,0.,0.));
#22787=DIRECTION('ref_axis',(0.,1.,-9.14588507257614E-13));
#22788=DIRECTION('',(1.,0.,0.));
#22789=DIRECTION('center_axis',(1.,0.,0.));
#22790=DIRECTION('ref_axis',(0.,1.,-9.14588507257614E-13));
#22791=DIRECTION('',(1.,0.,0.));
#22792=DIRECTION('center_axis',(1.,0.,0.));
#22793=DIRECTION('ref_axis',(0.,1.,-9.14588507257614E-13));
#22794=DIRECTION('',(1.,0.,0.));
#22795=DIRECTION('center_axis',(1.,0.,0.));
#22796=DIRECTION('ref_axis',(0.,1.,-9.14588507257614E-13));
#22797=DIRECTION('',(1.,0.,0.));
#22798=DIRECTION('center_axis',(1.,0.,0.));
#22799=DIRECTION('ref_axis',(0.,1.,-9.14588507257614E-13));
#22800=DIRECTION('',(1.,0.,0.));
#22801=DIRECTION('center_axis',(1.,0.,0.));
#22802=DIRECTION('ref_axis',(0.,1.,-9.14588507257614E-13));
#22803=DIRECTION('',(1.,0.,0.));
#22804=DIRECTION('center_axis',(1.,0.,0.));
#22805=DIRECTION('ref_axis',(0.,1.,-9.14588507257614E-13));
#22806=DIRECTION('',(1.,0.,0.));
#22807=DIRECTION('center_axis',(1.,0.,0.));
#22808=DIRECTION('ref_axis',(0.,1.,-9.14588507257614E-13));
#22809=DIRECTION('',(1.,0.,0.));
#22810=DIRECTION('center_axis',(1.,0.,0.));
#22811=DIRECTION('ref_axis',(0.,1.,-9.14588507257614E-13));
#22812=DIRECTION('',(1.,0.,0.));
#22813=DIRECTION('center_axis',(1.,0.,0.));
#22814=DIRECTION('ref_axis',(0.,1.,-9.14588507257614E-13));
#22815=DIRECTION('',(1.,0.,0.));
#22816=DIRECTION('center_axis',(1.,0.,0.));
#22817=DIRECTION('ref_axis',(0.,1.,-9.14588507257614E-13));
#22818=DIRECTION('',(1.,0.,0.));
#22819=DIRECTION('center_axis',(1.,0.,0.));
#22820=DIRECTION('ref_axis',(0.,1.,-9.14588507257614E-13));
#22821=DIRECTION('',(1.,0.,0.));
#22822=DIRECTION('center_axis',(1.,0.,0.));
#22823=DIRECTION('ref_axis',(0.,1.,-9.14588507257614E-13));
#22824=DIRECTION('',(1.,0.,0.));
#22825=DIRECTION('center_axis',(1.,0.,0.));
#22826=DIRECTION('ref_axis',(0.,1.,-9.14588507257614E-13));
#22827=DIRECTION('',(1.,0.,0.));
#22828=DIRECTION('center_axis',(1.,0.,0.));
#22829=DIRECTION('ref_axis',(0.,1.,-9.14588507257614E-13));
#22830=DIRECTION('',(1.,0.,0.));
#22831=DIRECTION('center_axis',(1.,0.,0.));
#22832=DIRECTION('ref_axis',(0.,1.,-9.14588507257614E-13));
#22833=DIRECTION('',(1.,0.,0.));
#22834=DIRECTION('center_axis',(1.,0.,0.));
#22835=DIRECTION('ref_axis',(0.,1.,-9.14588507257614E-13));
#22836=DIRECTION('',(1.,0.,0.));
#22837=DIRECTION('center_axis',(1.,0.,0.));
#22838=DIRECTION('ref_axis',(0.,1.,-9.14588507257614E-13));
#22839=DIRECTION('',(1.,0.,0.));
#22840=DIRECTION('center_axis',(1.,0.,0.));
#22841=DIRECTION('ref_axis',(0.,1.,-9.14588507257614E-13));
#22842=DIRECTION('',(1.,0.,0.));
#22843=DIRECTION('center_axis',(1.,0.,0.));
#22844=DIRECTION('ref_axis',(0.,1.,-9.14588507257614E-13));
#22845=DIRECTION('',(1.,0.,0.));
#22846=DIRECTION('center_axis',(1.,0.,0.));
#22847=DIRECTION('ref_axis',(0.,1.,-9.14588507257614E-13));
#22848=DIRECTION('',(1.,0.,0.));
#22849=DIRECTION('center_axis',(1.,0.,0.));
#22850=DIRECTION('ref_axis',(0.,1.,-9.14588507257614E-13));
#22851=DIRECTION('',(1.,0.,0.));
#22852=DIRECTION('center_axis',(1.,0.,0.));
#22853=DIRECTION('ref_axis',(0.,1.,-9.14588507257614E-13));
#22854=DIRECTION('',(1.,0.,0.));
#22855=DIRECTION('center_axis',(1.,0.,0.));
#22856=DIRECTION('ref_axis',(0.,1.,-9.14588507257614E-13));
#22857=DIRECTION('',(1.,0.,0.));
#22858=DIRECTION('center_axis',(1.,0.,0.));
#22859=DIRECTION('ref_axis',(0.,1.,-9.14588507257614E-13));
#22860=DIRECTION('',(1.,0.,0.));
#22861=DIRECTION('center_axis',(1.,0.,0.));
#22862=DIRECTION('ref_axis',(0.,1.,-9.14588507257614E-13));
#22863=DIRECTION('',(1.,0.,0.));
#22864=DIRECTION('center_axis',(1.,0.,0.));
#22865=DIRECTION('ref_axis',(0.,1.,-9.14588507257614E-13));
#22866=DIRECTION('',(1.,0.,0.));
#22867=DIRECTION('center_axis',(1.,0.,0.));
#22868=DIRECTION('ref_axis',(0.,1.,-9.14588507257614E-13));
#22869=DIRECTION('',(1.,0.,0.));
#22870=DIRECTION('center_axis',(1.,0.,0.));
#22871=DIRECTION('ref_axis',(0.,1.,-9.14588507257614E-13));
#22872=DIRECTION('',(1.,0.,0.));
#22873=DIRECTION('center_axis',(1.,0.,0.));
#22874=DIRECTION('ref_axis',(0.,1.,-9.14588507257614E-13));
#22875=DIRECTION('',(1.,0.,0.));
#22876=DIRECTION('center_axis',(1.,0.,0.));
#22877=DIRECTION('ref_axis',(0.,1.,-9.14588507257614E-13));
#22878=DIRECTION('',(1.,0.,0.));
#22879=DIRECTION('center_axis',(1.,0.,0.));
#22880=DIRECTION('ref_axis',(0.,1.,-9.14588507257614E-13));
#22881=DIRECTION('',(1.,0.,0.));
#22882=DIRECTION('center_axis',(1.,0.,0.));
#22883=DIRECTION('ref_axis',(0.,1.,-9.14588507257614E-13));
#22884=DIRECTION('',(1.,0.,0.));
#22885=DIRECTION('center_axis',(1.,0.,0.));
#22886=DIRECTION('ref_axis',(0.,1.,-9.14588507257614E-13));
#22887=DIRECTION('',(1.,0.,0.));
#22888=DIRECTION('center_axis',(1.,0.,0.));
#22889=DIRECTION('ref_axis',(0.,1.,-9.14588507257614E-13));
#22890=DIRECTION('',(1.,0.,0.));
#22891=DIRECTION('center_axis',(1.,0.,0.));
#22892=DIRECTION('ref_axis',(0.,1.,-9.14588507257614E-13));
#22893=DIRECTION('',(1.,0.,0.));
#22894=DIRECTION('center_axis',(1.,0.,0.));
#22895=DIRECTION('ref_axis',(0.,1.,-9.14588507257614E-13));
#22896=DIRECTION('',(1.,0.,0.));
#22897=DIRECTION('center_axis',(1.,0.,0.));
#22898=DIRECTION('ref_axis',(0.,1.,-9.14588507257614E-13));
#22899=DIRECTION('',(1.,0.,0.));
#22900=DIRECTION('center_axis',(1.,0.,0.));
#22901=DIRECTION('ref_axis',(0.,1.,-9.14588507257614E-13));
#22902=DIRECTION('',(1.,0.,0.));
#22903=DIRECTION('center_axis',(1.,0.,0.));
#22904=DIRECTION('ref_axis',(0.,1.,-9.14588507257614E-13));
#22905=DIRECTION('',(1.,0.,0.));
#22906=DIRECTION('center_axis',(1.,0.,0.));
#22907=DIRECTION('ref_axis',(0.,1.,-9.14588507257614E-13));
#22908=DIRECTION('',(1.,0.,0.));
#22909=DIRECTION('center_axis',(1.,0.,0.));
#22910=DIRECTION('ref_axis',(0.,1.,-9.14588507257614E-13));
#22911=DIRECTION('',(1.,0.,0.));
#22912=DIRECTION('center_axis',(1.,0.,0.));
#22913=DIRECTION('ref_axis',(0.,1.,-9.14588507257614E-13));
#22914=DIRECTION('',(1.,0.,0.));
#22915=DIRECTION('center_axis',(0.,0.,1.));
#22916=DIRECTION('ref_axis',(1.,0.,0.));
#22917=DIRECTION('',(0.,1.,0.));
#22918=DIRECTION('',(0.,-1.,0.));
#22919=DIRECTION('center_axis',(-1.,0.,0.));
#22920=DIRECTION('ref_axis',(0.,-1.,0.));
#22921=DIRECTION('',(0.,1.,0.));
#22922=DIRECTION('center_axis',(0.,0.,-1.));
#22923=DIRECTION('ref_axis',(-1.,0.,0.));
#22924=DIRECTION('',(0.,-1.,0.));
#22925=DIRECTION('center_axis',(1.,0.,0.));
#22926=DIRECTION('ref_axis',(0.,1.,0.));
#22927=DIRECTION('center_axis',(1.,0.,0.));
#22928=DIRECTION('ref_axis',(0.,0.,-1.));
#22929=DIRECTION('center_axis',(-1.,0.,0.));
#22930=DIRECTION('ref_axis',(0.,1.,0.));
#22931=DIRECTION('center_axis',(-1.,0.,0.));
#22932=DIRECTION('ref_axis',(0.,1.,0.));
#22933=DIRECTION('center_axis',(1.,0.,0.));
#22934=DIRECTION('ref_axis',(0.,0.,-1.));
#22935=DIRECTION('center_axis',(-1.,0.,0.));
#22936=DIRECTION('ref_axis',(0.,1.,-9.14588507257614E-13));
#22937=DIRECTION('center_axis',(1.,0.,0.));
#22938=DIRECTION('ref_axis',(0.,-0.298235389366233,0.95449235331121));
#22939=DIRECTION('center_axis',(1.,0.,0.));
#22940=DIRECTION('ref_axis',(0.,0.,-1.));
#22941=DIRECTION('center_axis',(1.,0.,0.));
#22942=DIRECTION('ref_axis',(0.,1.,0.));
#22943=DIRECTION('center_axis',(1.,0.,0.));
#22944=DIRECTION('ref_axis',(0.,1.,0.));
#22945=DIRECTION('center_axis',(1.,0.,0.));
#22946=DIRECTION('ref_axis',(0.,0.,-1.));
#22947=DIRECTION('center_axis',(-1.,0.,0.));
#22948=DIRECTION('ref_axis',(0.,1.,9.92840284004976E-14));
#22949=DIRECTION('center_axis',(1.,0.,0.));
#22950=DIRECTION('ref_axis',(0.,0.815561733925156,0.578670077122528));
#22951=DIRECTION('center_axis',(1.,0.,0.));
#22952=DIRECTION('ref_axis',(0.,1.,0.));
#22953=DIRECTION('center_axis',(1.,0.,0.));
#22954=DIRECTION('ref_axis',(0.,1.,0.));
#22955=DIRECTION('center_axis',(1.,0.,0.));
#22956=DIRECTION('ref_axis',(0.,-0.406736643075801,-0.913545457642601));
#22957=DIRECTION('center_axis',(1.,0.,0.));
#22958=DIRECTION('ref_axis',(0.,0.,-1.));
#22959=DIRECTION('center_axis',(1.,0.,0.));
#22960=DIRECTION('ref_axis',(0.,0.954766869449684,-0.297355385021442));
#22961=DIRECTION('',(1.,0.,0.));
#22962=DIRECTION('center_axis',(1.,0.,0.));
#22963=DIRECTION('ref_axis',(0.,0.954766869449684,-0.297355385021442));
#22964=DIRECTION('',(1.,0.,0.));
#22965=DIRECTION('center_axis',(-1.,0.,0.));
#22966=DIRECTION('ref_axis',(0.,0.954766869449684,-0.297355385021442));
#22967=DIRECTION('center_axis',(1.,0.,0.));
#22968=DIRECTION('ref_axis',(0.,-0.406736643075801,-0.913545457642601));
#22969=DIRECTION('center_axis',(1.,0.,0.));
#22970=DIRECTION('ref_axis',(0.,0.,-1.));
#22971=DIRECTION('center_axis',(1.,0.,0.));
#22972=DIRECTION('ref_axis',(0.,1.,0.));
#22973=DIRECTION('center_axis',(1.,0.,0.));
#22974=DIRECTION('ref_axis',(0.,0.,-1.));
#22975=DIRECTION('center_axis',(1.,0.,0.));
#22976=DIRECTION('ref_axis',(0.,0.,-1.));
#22977=DIRECTION('center_axis',(1.,0.,0.));
#22978=DIRECTION('ref_axis',(0.,1.,0.));
#22979=DIRECTION('center_axis',(1.,0.,0.));
#22980=DIRECTION('ref_axis',(0.,0.,-1.));
#22981=DIRECTION('center_axis',(1.,0.,0.));
#22982=DIRECTION('ref_axis',(0.,0.,-1.));
#22983=DIRECTION('center_axis',(1.,0.,0.));
#22984=DIRECTION('ref_axis',(0.,1.,0.));
#22985=DIRECTION('center_axis',(1.,0.,0.));
#22986=DIRECTION('ref_axis',(0.,0.,-1.));
#22987=DIRECTION('center_axis',(-1.,0.,0.));
#22988=DIRECTION('ref_axis',(0.,1.,0.));
#22989=DIRECTION('center_axis',(1.,0.,0.));
#22990=DIRECTION('ref_axis',(0.,0.,-1.));
#22991=DIRECTION('center_axis',(1.,0.,0.));
#22992=DIRECTION('ref_axis',(0.,-0.743144825477395,-0.669130606358858));
#22993=DIRECTION('center_axis',(1.,0.,0.));
#22994=DIRECTION('ref_axis',(0.,0.,-1.));
#22995=DIRECTION('center_axis',(1.,0.,0.));
#22996=DIRECTION('ref_axis',(0.,0.751277605589271,-0.65998633269186));
#22997=DIRECTION('',(1.,0.,0.));
#22998=DIRECTION('center_axis',(1.,0.,0.));
#22999=DIRECTION('ref_axis',(0.,0.751277605589271,-0.65998633269186));
#23000=DIRECTION('',(1.,0.,0.));
#23001=DIRECTION('center_axis',(-1.,0.,0.));
#23002=DIRECTION('ref_axis',(0.,0.751277605589271,-0.65998633269186));
#23003=DIRECTION('center_axis',(1.,0.,0.));
#23004=DIRECTION('ref_axis',(0.,-0.743144825477395,-0.669130606358858));
#23005=DIRECTION('center_axis',(1.,0.,0.));
#23006=DIRECTION('ref_axis',(0.,0.,-1.));
#23007=DIRECTION('center_axis',(1.,0.,0.));
#23008=DIRECTION('ref_axis',(0.,1.,0.));
#23009=DIRECTION('center_axis',(1.,0.,0.));
#23010=DIRECTION('ref_axis',(0.,0.,-1.));
#23011=DIRECTION('center_axis',(1.,0.,0.));
#23012=DIRECTION('ref_axis',(0.,0.,-1.));
#23013=DIRECTION('center_axis',(1.,0.,0.));
#23014=DIRECTION('ref_axis',(0.,1.,0.));
#23015=DIRECTION('center_axis',(1.,0.,0.));
#23016=DIRECTION('ref_axis',(0.,0.,-1.));
#23017=DIRECTION('center_axis',(-1.,0.,0.));
#23018=DIRECTION('ref_axis',(0.,1.,0.));
#23019=DIRECTION('center_axis',(1.,0.,0.));
#23020=DIRECTION('ref_axis',(0.,0.,-1.));
#23021=DIRECTION('center_axis',(1.,0.,0.));
#23022=DIRECTION('ref_axis',(0.,-0.951056516295154,-0.309016994374947));
#23023=DIRECTION('center_axis',(1.,0.,0.));
#23024=DIRECTION('ref_axis',(0.,0.,-1.));
#23025=DIRECTION('center_axis',(1.,0.,0.));
#23026=DIRECTION('ref_axis',(0.,0.417885618579693,-0.908499647652253));
#23027=DIRECTION('',(1.,0.,0.));
#23028=DIRECTION('center_axis',(1.,0.,0.));
#23029=DIRECTION('ref_axis',(0.,0.417885618579693,-0.908499647652253));
#23030=DIRECTION('',(1.,0.,0.));
#23031=DIRECTION('center_axis',(-1.,0.,0.));
#23032=DIRECTION('ref_axis',(0.,0.417885618579693,-0.908499647652253));
#23033=DIRECTION('center_axis',(1.,0.,0.));
#23034=DIRECTION('ref_axis',(0.,-0.951056516295154,-0.309016994374947));
#23035=DIRECTION('center_axis',(1.,0.,0.));
#23036=DIRECTION('ref_axis',(0.,0.,-1.));
#23037=DIRECTION('center_axis',(1.,0.,0.));
#23038=DIRECTION('ref_axis',(0.,1.,0.));
#23039=DIRECTION('center_axis',(1.,0.,0.));
#23040=DIRECTION('ref_axis',(0.,0.,-1.));
#23041=DIRECTION('center_axis',(1.,0.,0.));
#23042=DIRECTION('ref_axis',(0.,0.,-1.));
#23043=DIRECTION('center_axis',(1.,0.,0.));
#23044=DIRECTION('ref_axis',(0.,1.,0.));
#23045=DIRECTION('center_axis',(1.,0.,0.));
#23046=DIRECTION('ref_axis',(0.,0.,-1.));
#23047=DIRECTION('center_axis',(-1.,0.,0.));
#23048=DIRECTION('ref_axis',(0.,1.,0.));
#23049=DIRECTION('center_axis',(1.,0.,0.));
#23050=DIRECTION('ref_axis',(0.,0.,-1.));
#23051=DIRECTION('center_axis',(1.,0.,0.));
#23052=DIRECTION('ref_axis',(0.,-0.994521895368273,0.104528463267654));
#23053=DIRECTION('center_axis',(1.,0.,0.));
#23054=DIRECTION('ref_axis',(0.,0.,-1.));
#23055=DIRECTION('center_axis',(1.,0.,0.));
#23056=DIRECTION('ref_axis',(0.,0.0122374117460222,-0.999925120073377));
#23057=DIRECTION('',(1.,0.,0.));
#23058=DIRECTION('center_axis',(1.,0.,0.));
#23059=DIRECTION('ref_axis',(0.,0.0122374117460222,-0.999925120073377));
#23060=DIRECTION('',(1.,0.,0.));
#23061=DIRECTION('center_axis',(-1.,0.,0.));
#23062=DIRECTION('ref_axis',(0.,0.0122374117460222,-0.999925120073377));
#23063=DIRECTION('center_axis',(1.,0.,0.));
#23064=DIRECTION('ref_axis',(0.,-0.994521895368273,0.104528463267654));
#23065=DIRECTION('center_axis',(1.,0.,0.));
#23066=DIRECTION('ref_axis',(0.,0.,-1.));
#23067=DIRECTION('center_axis',(1.,0.,0.));
#23068=DIRECTION('ref_axis',(0.,1.,0.));
#23069=DIRECTION('center_axis',(1.,0.,0.));
#23070=DIRECTION('ref_axis',(0.,0.,-1.));
#23071=DIRECTION('center_axis',(1.,0.,0.));
#23072=DIRECTION('ref_axis',(0.,0.,-1.));
#23073=DIRECTION('center_axis',(1.,0.,0.));
#23074=DIRECTION('ref_axis',(0.,1.,0.));
#23075=DIRECTION('center_axis',(1.,0.,0.));
#23076=DIRECTION('ref_axis',(0.,0.,-1.));
#23077=DIRECTION('center_axis',(-1.,0.,0.));
#23078=DIRECTION('ref_axis',(0.,1.,0.));
#23079=DIRECTION('center_axis',(1.,0.,0.));
#23080=DIRECTION('ref_axis',(0.,0.,-1.));
#23081=DIRECTION('center_axis',(1.,0.,0.));
#23082=DIRECTION('ref_axis',(0.,-0.866025403784438,0.5));
#23083=DIRECTION('center_axis',(1.,0.,0.));
#23084=DIRECTION('ref_axis',(0.,0.,-1.));
#23085=DIRECTION('center_axis',(1.,0.,0.));
#23086=DIRECTION('ref_axis',(0.,-0.395526754751931,-0.91845445519928));
#23087=DIRECTION('',(1.,0.,0.));
#23088=DIRECTION('center_axis',(1.,0.,0.));
#23089=DIRECTION('ref_axis',(0.,-0.395526754751931,-0.91845445519928));
#23090=DIRECTION('',(1.,0.,0.));
#23091=DIRECTION('center_axis',(-1.,0.,0.));
#23092=DIRECTION('ref_axis',(0.,-0.395526754751931,-0.91845445519928));
#23093=DIRECTION('center_axis',(1.,0.,0.));
#23094=DIRECTION('ref_axis',(0.,-0.866025403784438,0.5));
#23095=DIRECTION('center_axis',(1.,0.,0.));
#23096=DIRECTION('ref_axis',(0.,0.,-1.));
#23097=DIRECTION('center_axis',(1.,0.,0.));
#23098=DIRECTION('ref_axis',(0.,1.,0.));
#23099=DIRECTION('center_axis',(1.,0.,0.));
#23100=DIRECTION('ref_axis',(0.,0.,-1.));
#23101=DIRECTION('center_axis',(1.,0.,0.));
#23102=DIRECTION('ref_axis',(0.,0.,-1.));
#23103=DIRECTION('center_axis',(1.,0.,0.));
#23104=DIRECTION('ref_axis',(0.,1.,0.));
#23105=DIRECTION('center_axis',(1.,0.,0.));
#23106=DIRECTION('ref_axis',(0.,0.,-1.));
#23107=DIRECTION('center_axis',(-1.,0.,0.));
#23108=DIRECTION('ref_axis',(0.,1.,0.));
#23109=DIRECTION('center_axis',(1.,0.,0.));
#23110=DIRECTION('ref_axis',(0.,0.,-1.));
#23111=DIRECTION('center_axis',(1.,0.,0.));
#23112=DIRECTION('ref_axis',(0.,-0.587785252292473,0.809016994374947));
#23113=DIRECTION('center_axis',(1.,0.,0.));
#23114=DIRECTION('ref_axis',(0.,0.,-1.));
#23115=DIRECTION('center_axis',(1.,0.,0.));
#23116=DIRECTION('ref_axis',(0.,-0.734900752105513,-0.678174671124446));
#23117=DIRECTION('',(1.,0.,0.));
#23118=DIRECTION('center_axis',(1.,0.,0.));
#23119=DIRECTION('ref_axis',(0.,-0.734900752105513,-0.678174671124446));
#23120=DIRECTION('',(1.,0.,0.));
#23121=DIRECTION('center_axis',(-1.,0.,0.));
#23122=DIRECTION('ref_axis',(0.,-0.734900752105513,-0.678174671124446));
#23123=DIRECTION('center_axis',(1.,0.,0.));
#23124=DIRECTION('ref_axis',(0.,-0.587785252292473,0.809016994374947));
#23125=DIRECTION('center_axis',(1.,0.,0.));
#23126=DIRECTION('ref_axis',(0.,0.,-1.));
#23127=DIRECTION('center_axis',(1.,0.,0.));
#23128=DIRECTION('ref_axis',(0.,1.,0.));
#23129=DIRECTION('center_axis',(1.,0.,0.));
#23130=DIRECTION('ref_axis',(0.,0.,-1.));
#23131=DIRECTION('center_axis',(1.,0.,0.));
#23132=DIRECTION('ref_axis',(0.,0.,-1.));
#23133=DIRECTION('center_axis',(1.,0.,0.));
#23134=DIRECTION('ref_axis',(0.,1.,0.));
#23135=DIRECTION('center_axis',(1.,0.,0.));
#23136=DIRECTION('ref_axis',(0.,0.,-1.));
#23137=DIRECTION('center_axis',(-1.,0.,0.));
#23138=DIRECTION('ref_axis',(0.,1.,0.));
#23139=DIRECTION('center_axis',(1.,0.,0.));
#23140=DIRECTION('ref_axis',(0.,0.,-1.));
#23141=DIRECTION('center_axis',(1.,0.,0.));
#23142=DIRECTION('ref_axis',(0.,-0.207911690817759,0.978147600733806));
#23143=DIRECTION('center_axis',(1.,0.,0.));
#23144=DIRECTION('ref_axis',(0.,0.,-1.));
#23145=DIRECTION('center_axis',(1.,0.,0.));
#23146=DIRECTION('ref_axis',(0.,-0.947203733056315,-0.320632325388725));
#23147=DIRECTION('',(1.,0.,0.));
#23148=DIRECTION('center_axis',(1.,0.,0.));
#23149=DIRECTION('ref_axis',(0.,-0.947203733056315,-0.320632325388725));
#23150=DIRECTION('',(1.,0.,0.));
#23151=DIRECTION('center_axis',(-1.,0.,0.));
#23152=DIRECTION('ref_axis',(0.,-0.947203733056315,-0.320632325388725));
#23153=DIRECTION('center_axis',(1.,0.,0.));
#23154=DIRECTION('ref_axis',(0.,-0.207911690817759,0.978147600733806));
#23155=DIRECTION('center_axis',(1.,0.,0.));
#23156=DIRECTION('ref_axis',(0.,0.,-1.));
#23157=DIRECTION('center_axis',(1.,0.,0.));
#23158=DIRECTION('ref_axis',(0.,1.,0.));
#23159=DIRECTION('center_axis',(1.,0.,0.));
#23160=DIRECTION('ref_axis',(0.,0.,-1.));
#23161=DIRECTION('center_axis',(1.,0.,0.));
#23162=DIRECTION('ref_axis',(0.,0.,-1.));
#23163=DIRECTION('center_axis',(1.,0.,0.));
#23164=DIRECTION('ref_axis',(0.,1.,0.));
#23165=DIRECTION('center_axis',(1.,0.,0.));
#23166=DIRECTION('ref_axis',(0.,0.,-1.));
#23167=DIRECTION('center_axis',(-1.,0.,0.));
#23168=DIRECTION('ref_axis',(0.,1.,0.));
#23169=DIRECTION('center_axis',(1.,0.,0.));
#23170=DIRECTION('ref_axis',(0.,0.,-1.));
#23171=DIRECTION('center_axis',(1.,0.,0.));
#23172=DIRECTION('ref_axis',(0.,0.20791169081776,0.978147600733805));
#23173=DIRECTION('center_axis',(1.,0.,0.));
#23174=DIRECTION('ref_axis',(0.,0.,-1.));
#23175=DIRECTION('center_axis',(1.,0.,0.));
#23176=DIRECTION('ref_axis',(0.,0.,-1.));
#23177=DIRECTION('center_axis',(1.,0.,0.));
#23178=DIRECTION('ref_axis',(0.,-0.995726583485909,0.0923502622599377));
#23179=DIRECTION('',(1.,0.,0.));
#23180=DIRECTION('center_axis',(1.,0.,0.));
#23181=DIRECTION('ref_axis',(0.,-0.995726583485909,0.0923502622599377));
#23182=DIRECTION('',(1.,0.,0.));
#23183=DIRECTION('center_axis',(-1.,0.,0.));
#23184=DIRECTION('ref_axis',(0.,-0.995726583485909,0.0923502622599377));
#23185=DIRECTION('center_axis',(1.,0.,0.));
#23186=DIRECTION('ref_axis',(0.,0.20791169081776,0.978147600733805));
#23187=DIRECTION('center_axis',(1.,0.,0.));
#23188=DIRECTION('ref_axis',(0.,0.,-1.));
#23189=DIRECTION('center_axis',(1.,0.,0.));
#23190=DIRECTION('ref_axis',(0.,0.,-1.));
#23191=DIRECTION('center_axis',(1.,0.,0.));
#23192=DIRECTION('ref_axis',(0.,1.,0.));
#23193=DIRECTION('center_axis',(1.,0.,0.));
#23194=DIRECTION('ref_axis',(0.,0.,-1.));
#23195=DIRECTION('center_axis',(1.,0.,0.));
#23196=DIRECTION('ref_axis',(0.,0.,-1.));
#23197=DIRECTION('center_axis',(1.,0.,0.));
#23198=DIRECTION('ref_axis',(0.,1.,0.));
#23199=DIRECTION('center_axis',(1.,0.,0.));
#23200=DIRECTION('ref_axis',(0.,0.,-1.));
#23201=DIRECTION('center_axis',(-1.,0.,0.));
#23202=DIRECTION('ref_axis',(0.,1.,0.));
#23203=DIRECTION('center_axis',(1.,0.,0.));
#23204=DIRECTION('ref_axis',(0.,0.,-1.));
#23205=DIRECTION('center_axis',(1.,0.,0.));
#23206=DIRECTION('ref_axis',(0.,0.587785252292473,0.809016994374947));
#23207=DIRECTION('center_axis',(1.,0.,0.));
#23208=DIRECTION('ref_axis',(0.,0.,-1.));
#23209=DIRECTION('center_axis',(1.,0.,0.));
#23210=DIRECTION('ref_axis',(0.,-0.872079261738761,0.489364650588063));
#23211=DIRECTION('',(1.,0.,0.));
#23212=DIRECTION('center_axis',(1.,0.,0.));
#23213=DIRECTION('ref_axis',(0.,-0.872079261738761,0.489364650588063));
#23214=DIRECTION('',(1.,0.,0.));
#23215=DIRECTION('center_axis',(-1.,0.,0.));
#23216=DIRECTION('ref_axis',(0.,-0.872079261738761,0.489364650588063));
#23217=DIRECTION('center_axis',(1.,0.,0.));
#23218=DIRECTION('ref_axis',(0.,0.587785252292473,0.809016994374947));
#23219=DIRECTION('center_axis',(1.,0.,0.));
#23220=DIRECTION('ref_axis',(0.,0.,-1.));
#23221=DIRECTION('center_axis',(1.,0.,0.));
#23222=DIRECTION('ref_axis',(0.,1.,0.));
#23223=DIRECTION('center_axis',(1.,0.,0.));
#23224=DIRECTION('ref_axis',(0.,0.,-1.));
#23225=DIRECTION('center_axis',(1.,0.,0.));
#23226=DIRECTION('ref_axis',(0.,0.,-1.));
#23227=DIRECTION('center_axis',(1.,0.,0.));
#23228=DIRECTION('ref_axis',(0.,1.,0.));
#23229=DIRECTION('center_axis',(1.,0.,0.));
#23230=DIRECTION('ref_axis',(0.,0.,-1.));
#23231=DIRECTION('center_axis',(-1.,0.,0.));
#23232=DIRECTION('ref_axis',(0.,1.,0.));
#23233=DIRECTION('center_axis',(1.,0.,0.));
#23234=DIRECTION('ref_axis',(0.,0.,-1.));
#23235=DIRECTION('center_axis',(1.,0.,0.));
#23236=DIRECTION('ref_axis',(0.,0.866025403784439,0.5));
#23237=DIRECTION('center_axis',(1.,0.,0.));
#23238=DIRECTION('ref_axis',(0.,0.,-1.));
#23239=DIRECTION('center_axis',(1.,0.,0.));
#23240=DIRECTION('ref_axis',(0.,-0.597641513045608,0.801763445091229));
#23241=DIRECTION('',(1.,0.,0.));
#23242=DIRECTION('center_axis',(1.,0.,0.));
#23243=DIRECTION('ref_axis',(0.,-0.597641513045608,0.801763445091229));
#23244=DIRECTION('',(1.,0.,0.));
#23245=DIRECTION('center_axis',(-1.,0.,0.));
#23246=DIRECTION('ref_axis',(0.,-0.597641513045608,0.801763445091229));
#23247=DIRECTION('center_axis',(1.,0.,0.));
#23248=DIRECTION('ref_axis',(0.,0.866025403784439,0.5));
#23249=DIRECTION('center_axis',(1.,0.,0.));
#23250=DIRECTION('ref_axis',(0.,0.,-1.));
#23251=DIRECTION('center_axis',(1.,0.,0.));
#23252=DIRECTION('ref_axis',(0.,1.,0.));
#23253=DIRECTION('center_axis',(1.,0.,0.));
#23254=DIRECTION('ref_axis',(0.,0.,-1.));
#23255=DIRECTION('center_axis',(1.,0.,0.));
#23256=DIRECTION('ref_axis',(0.,0.,-1.));
#23257=DIRECTION('center_axis',(1.,0.,0.));
#23258=DIRECTION('ref_axis',(0.,1.,0.));
#23259=DIRECTION('center_axis',(1.,0.,0.));
#23260=DIRECTION('ref_axis',(0.,0.,-1.));
#23261=DIRECTION('center_axis',(-1.,0.,0.));
#23262=DIRECTION('ref_axis',(0.,1.,0.));
#23263=DIRECTION('center_axis',(1.,0.,0.));
#23264=DIRECTION('ref_axis',(0.,0.,-1.));
#23265=DIRECTION('center_axis',(1.,0.,0.));
#23266=DIRECTION('ref_axis',(0.,0.994521895368273,0.104528463267653));
#23267=DIRECTION('center_axis',(1.,0.,0.));
#23268=DIRECTION('ref_axis',(0.,0.,-1.));
#23269=DIRECTION('center_axis',(1.,0.,0.));
#23270=DIRECTION('ref_axis',(0.,-0.219866117344171,0.975530056145888));
#23271=DIRECTION('',(1.,0.,0.));
#23272=DIRECTION('center_axis',(1.,0.,0.));
#23273=DIRECTION('ref_axis',(0.,-0.219866117344171,0.975530056145888));
#23274=DIRECTION('',(1.,0.,0.));
#23275=DIRECTION('center_axis',(-1.,0.,0.));
#23276=DIRECTION('ref_axis',(0.,-0.219866117344171,0.975530056145888));
#23277=DIRECTION('center_axis',(1.,0.,0.));
#23278=DIRECTION('ref_axis',(0.,0.994521895368273,0.104528463267653));
#23279=DIRECTION('center_axis',(1.,0.,0.));
#23280=DIRECTION('ref_axis',(0.,0.,-1.));
#23281=DIRECTION('center_axis',(1.,0.,0.));
#23282=DIRECTION('ref_axis',(0.,1.,0.));
#23283=DIRECTION('center_axis',(1.,0.,0.));
#23284=DIRECTION('ref_axis',(0.,0.,-1.));
#23285=DIRECTION('center_axis',(1.,0.,0.));
#23286=DIRECTION('ref_axis',(0.,0.,-1.));
#23287=DIRECTION('center_axis',(1.,0.,0.));
#23288=DIRECTION('ref_axis',(0.,1.,0.));
#23289=DIRECTION('center_axis',(1.,0.,0.));
#23290=DIRECTION('ref_axis',(0.,0.,-1.));
#23291=DIRECTION('center_axis',(-1.,0.,0.));
#23292=DIRECTION('ref_axis',(0.,1.,0.));
#23293=DIRECTION('center_axis',(1.,0.,0.));
#23294=DIRECTION('ref_axis',(0.,0.,-1.));
#23295=DIRECTION('center_axis',(1.,0.,0.));
#23296=DIRECTION('ref_axis',(0.,0.951056516295154,-0.309016994374948));
#23297=DIRECTION('center_axis',(1.,0.,0.));
#23298=DIRECTION('ref_axis',(0.,0.,-1.));
#23299=DIRECTION('center_axis',(1.,0.,0.));
#23300=DIRECTION('ref_axis',(0.,0.195926127467043,0.980618658080585));
#23301=DIRECTION('',(1.,0.,0.));
#23302=DIRECTION('center_axis',(1.,0.,0.));
#23303=DIRECTION('ref_axis',(0.,0.195926127467043,0.980618658080585));
#23304=DIRECTION('',(1.,0.,0.));
#23305=DIRECTION('center_axis',(-1.,0.,0.));
#23306=DIRECTION('ref_axis',(0.,0.195926127467043,0.980618658080585));
#23307=DIRECTION('center_axis',(1.,0.,0.));
#23308=DIRECTION('ref_axis',(0.,0.951056516295154,-0.309016994374948));
#23309=DIRECTION('center_axis',(1.,0.,0.));
#23310=DIRECTION('ref_axis',(0.,0.,-1.));
#23311=DIRECTION('center_axis',(1.,0.,0.));
#23312=DIRECTION('ref_axis',(0.,1.,0.));
#23313=DIRECTION('center_axis',(1.,0.,0.));
#23314=DIRECTION('ref_axis',(0.,0.,-1.));
#23315=DIRECTION('center_axis',(1.,0.,0.));
#23316=DIRECTION('ref_axis',(0.,0.,-1.));
#23317=DIRECTION('center_axis',(1.,0.,0.));
#23318=DIRECTION('ref_axis',(0.,1.,0.));
#23319=DIRECTION('center_axis',(1.,0.,0.));
#23320=DIRECTION('ref_axis',(0.,0.,-1.));
#23321=DIRECTION('center_axis',(-1.,0.,0.));
#23322=DIRECTION('ref_axis',(0.,1.,0.));
#23323=DIRECTION('center_axis',(1.,0.,0.));
#23324=DIRECTION('ref_axis',(0.,0.,-1.));
#23325=DIRECTION('center_axis',(1.,0.,0.));
#23326=DIRECTION('ref_axis',(0.,0.743144825477394,-0.669130606358858));
#23327=DIRECTION('center_axis',(1.,0.,0.));
#23328=DIRECTION('ref_axis',(0.,0.,-1.));
#23329=DIRECTION('center_axis',(1.,0.,0.));
#23330=DIRECTION('ref_axis',(0.,0.577840964906216,0.816149385392315));
#23331=DIRECTION('',(1.,0.,0.));
#23332=DIRECTION('center_axis',(1.,0.,0.));
#23333=DIRECTION('ref_axis',(0.,0.577840964906216,0.816149385392315));
#23334=DIRECTION('',(1.,0.,0.));
#23335=DIRECTION('center_axis',(-1.,0.,0.));
#23336=DIRECTION('ref_axis',(0.,0.577840964906216,0.816149385392315));
#23337=DIRECTION('center_axis',(1.,0.,0.));
#23338=DIRECTION('ref_axis',(0.,0.743144825477394,-0.669130606358858));
#23339=DIRECTION('center_axis',(1.,0.,0.));
#23340=DIRECTION('ref_axis',(0.,0.,-1.));
#23341=DIRECTION('center_axis',(1.,0.,0.));
#23342=DIRECTION('ref_axis',(0.,1.,0.));
#23343=DIRECTION('center_axis',(1.,0.,0.));
#23344=DIRECTION('ref_axis',(0.,0.,-1.));
#23345=DIRECTION('center_axis',(1.,0.,0.));
#23346=DIRECTION('ref_axis',(0.,0.,-1.));
#23347=DIRECTION('center_axis',(1.,0.,0.));
#23348=DIRECTION('ref_axis',(0.,1.,0.));
#23349=DIRECTION('center_axis',(1.,0.,0.));
#23350=DIRECTION('ref_axis',(0.,0.,-1.));
#23351=DIRECTION('center_axis',(-1.,0.,0.));
#23352=DIRECTION('ref_axis',(0.,1.,0.));
#23353=DIRECTION('center_axis',(1.,0.,0.));
#23354=DIRECTION('ref_axis',(0.,0.,-1.));
#23355=DIRECTION('center_axis',(1.,0.,0.));
#23356=DIRECTION('ref_axis',(0.,0.4067366430758,-0.913545457642601));
#23357=DIRECTION('center_axis',(1.,0.,0.));
#23358=DIRECTION('ref_axis',(0.,0.,-1.));
#23359=DIRECTION('center_axis',(1.,0.,0.));
#23360=DIRECTION('ref_axis',(0.,0.859841849992738,0.510560469485315));
#23361=DIRECTION('',(1.,0.,0.));
#23362=DIRECTION('center_axis',(1.,0.,0.));
#23363=DIRECTION('ref_axis',(0.,0.859841849992738,0.510560469485315));
#23364=DIRECTION('',(1.,0.,0.));
#23365=DIRECTION('center_axis',(-1.,0.,0.));
#23366=DIRECTION('ref_axis',(0.,0.859841849992738,0.510560469485315));
#23367=DIRECTION('center_axis',(1.,0.,0.));
#23368=DIRECTION('ref_axis',(0.,0.4067366430758,-0.913545457642601));
#23369=DIRECTION('center_axis',(1.,0.,0.));
#23370=DIRECTION('ref_axis',(0.,0.,-1.));
#23371=DIRECTION('center_axis',(1.,0.,0.));
#23372=DIRECTION('ref_axis',(0.,1.,0.));
#23373=DIRECTION('center_axis',(1.,0.,0.));
#23374=DIRECTION('ref_axis',(0.,0.,-1.));
#23375=DIRECTION('center_axis',(1.,0.,0.));
#23376=DIRECTION('ref_axis',(0.,0.,-1.));
#23377=DIRECTION('center_axis',(1.,0.,0.));
#23378=DIRECTION('ref_axis',(0.,1.,0.));
#23379=DIRECTION('center_axis',(1.,0.,0.));
#23380=DIRECTION('ref_axis',(0.,0.,-1.));
#23381=DIRECTION('center_axis',(-1.,0.,0.));
#23382=DIRECTION('ref_axis',(0.,1.,0.));
#23383=DIRECTION('center_axis',(1.,0.,0.));
#23384=DIRECTION('ref_axis',(0.,0.,-1.));
#23385=DIRECTION('',(1.,0.,0.));
#23386=DIRECTION('center_axis',(1.,0.,0.));
#23387=DIRECTION('ref_axis',(0.,0.,-1.));
#23388=DIRECTION('center_axis',(1.,0.,0.));
#23389=DIRECTION('ref_axis',(0.,0.,-1.));
#23390=DIRECTION('center_axis',(1.,0.,0.));
#23391=DIRECTION('ref_axis',(0.,0.993168267797538,0.116691010108051));
#23392=DIRECTION('center_axis',(1.,0.,0.));
#23393=DIRECTION('ref_axis',(0.,0.993168267797538,0.116691010108051));
#23394=DIRECTION('center_axis',(-1.,0.,0.));
#23395=DIRECTION('ref_axis',(0.,0.993168267797538,0.116691010108051));
#23396=DIRECTION('',(1.,0.,0.));
#23397=DIRECTION('center_axis',(1.,0.,0.));
#23398=DIRECTION('ref_axis',(0.,0.,-1.));
#23399=DIRECTION('center_axis',(1.,0.,0.));
#23400=DIRECTION('ref_axis',(0.,0.,-1.));
#23401=DIRECTION('center_axis',(-1.,0.,0.));
#23402=DIRECTION('ref_axis',(0.,1.,0.));
#23403=DIRECTION('center_axis',(1.,0.,0.));
#23404=DIRECTION('ref_axis',(0.,0.,-1.));
#23405=DIRECTION('center_axis',(1.,0.,0.));
#23406=DIRECTION('ref_axis',(0.,0.,-1.));
#23407=DIRECTION('center_axis',(1.,0.,0.));
#23408=DIRECTION('ref_axis',(0.,1.,0.));
#23409=DIRECTION('center_axis',(-1.,0.,0.));
#23410=DIRECTION('ref_axis',(0.,0.,1.));
#23411=DIRECTION('center_axis',(1.,0.,0.));
#23412=DIRECTION('ref_axis',(0.,0.,-1.));
#23413=DIRECTION('center_axis',(1.,0.,0.));
#23414=DIRECTION('ref_axis',(0.,1.,0.));
#23415=DIRECTION('',(-0.707106781186546,0.707106781186549,8.65956056235495E-17));
#23416=DIRECTION('center_axis',(1.,0.,0.));
#23417=DIRECTION('ref_axis',(0.,1.,0.));
#23418=DIRECTION('',(-0.157990501106675,0.987440631916705,1.20926600922483E-16));
#23419=DIRECTION('center_axis',(-1.,0.,0.));
#23420=DIRECTION('ref_axis',(0.,1.,0.));
#23421=DIRECTION('',(-0.157990501106672,-0.987440631916706,-1.20926600922483E-16));
#23422=DIRECTION('center_axis',(1.,0.,0.));
#23423=DIRECTION('ref_axis',(0.,1.,0.));
#23424=DIRECTION('center_axis',(-1.,0.,0.));
#23425=DIRECTION('ref_axis',(0.,1.,0.));
#23426=DIRECTION('center_axis',(-1.,0.,0.));
#23427=DIRECTION('ref_axis',(0.,1.,0.));
#23428=DIRECTION('center_axis',(1.,0.,0.));
#23429=DIRECTION('ref_axis',(0.,0.,-1.));
#23430=DIRECTION('',(-0.707106781186546,-0.707106781186549,-8.65956056235495E-17));
#23431=DIRECTION('center_axis',(1.,0.,0.));
#23432=DIRECTION('ref_axis',(0.,0.,-1.));
#27820=CARTESIAN_POINT('',(0.,0.,0.));
#27821=CARTESIAN_POINT('Origin',(29.75,0.,0.));
#27822=CARTESIAN_POINT('',(32.1628916636063,-6.92198924261957,-0.00637899664044927));
#27823=CARTESIAN_POINT('',(31.9835483363939,-6.9206415740836,-0.000329640349373658));
#27824=CARTESIAN_POINT('',(29.75,-6.933,-8.4904762584886E-16));
#27825=CARTESIAN_POINT('',(31.067,-4.95966987665981,-4.85170944379072));
#27826=CARTESIAN_POINT('Ctrl Pts',(32.1628916636063,-6.92198924261957,-0.00637899664044927));
#27827=CARTESIAN_POINT('Ctrl Pts',(32.1234269345577,-6.91442709372537,1.37132673071421));
#27828=CARTESIAN_POINT('Ctrl Pts',(32.0839622055092,-6.51430118721618,2.75348702170588));
#27829=CARTESIAN_POINT('Ctrl Pts',(32.0444974764607,-5.74807259775006,3.89182548507003));
#27830=CARTESIAN_POINT('Ctrl Pts',(32.0114122090537,-5.10570463048956,4.84615187646083));
#27831=CARTESIAN_POINT('Ctrl Pts',(31.9783269416467,-4.20602826637418,5.62911267424726));
#27832=CARTESIAN_POINT('Ctrl Pts',(31.9452416742396,-3.17855940282965,6.157422342539));
#27833=CARTESIAN_POINT('Ctrl Pts',(31.9121564068326,-2.15109053928511,6.68573201083074));
#27834=CARTESIAN_POINT('Ctrl Pts',(31.8790711394256,-0.995829176311432,
6.95939054962779));
#27835=CARTESIAN_POINT('Ctrl Pts',(31.8459858720186,0.153365723954005,6.93401243877144));
#27836=CARTESIAN_POINT('Ctrl Pts',(31.8129006046115,1.30256062421944,6.90863432791508));
#27837=CARTESIAN_POINT('Ctrl Pts',(31.7798153372045,2.44568906177664,6.58421956740534));
#27838=CARTESIAN_POINT('Ctrl Pts',(31.7467300697975,3.44866898595544,6.0108050971193));
#27839=CARTESIAN_POINT('Ctrl Pts',(31.7136448023905,4.45164891013425,5.43739062683326));
#27840=CARTESIAN_POINT('Ctrl Pts',(31.6805595349835,5.31448032093466,4.61497644677094));
#27841=CARTESIAN_POINT('Ctrl Pts',(31.6474742675765,5.91376424879513,3.63312504742053));
#27842=CARTESIAN_POINT('Ctrl Pts',(31.5813037327624,7.11233210451607,1.66942224871972));
#27843=CARTESIAN_POINT('Ctrl Pts',(31.5151331979484,7.25671002847726,-0.932029427133405));
#27844=CARTESIAN_POINT('Ctrl Pts',(31.4489626631344,6.26478062010639,-2.99981867537784));
#27845=CARTESIAN_POINT('Ctrl Pts',(31.3827921283203,5.27285121173552,-5.06760792362229));
#27846=CARTESIAN_POINT('Ctrl Pts',(31.3166215935063,3.14461447103258,-6.60173474425803));
#27847=CARTESIAN_POINT('Ctrl Pts',(31.2504510586922,0.869393195229573,-6.8908669450609));
#27848=CARTESIAN_POINT('Ctrl Pts',(31.1893007057948,-1.23321311324388,-7.15806345726668));
#27849=CARTESIAN_POINT('Ctrl Pts',(31.1281503528974,-3.46134732907935,-6.3620081845267));
#27850=CARTESIAN_POINT('Ctrl Pts',(31.067,-4.95966987665981,-4.85170944379072));
#27851=CARTESIAN_POINT('',(31.067,-6.933,-8.4904762584886E-16));
#27852=CARTESIAN_POINT('Origin',(31.067,0.,0.));
#27853=CARTESIAN_POINT('',(0.,-6.933,-8.4904762584886E-16));
#27854=CARTESIAN_POINT('',(29.75,-6.933,-8.4904762584886E-16));
#27855=CARTESIAN_POINT('',(0.,-6.60730572926666,-2.1));
#27856=CARTESIAN_POINT('Origin',(0.,0.,0.));
#27857=CARTESIAN_POINT('',(-16.,-6.60730572926666,-2.1));
#27858=CARTESIAN_POINT('',(29.75,-6.60730572926666,-2.1));
#27859=CARTESIAN_POINT('',(-16.,-6.933,-8.4904762584886E-16));
#27860=CARTESIAN_POINT('Origin',(-16.,0.,0.));
#27861=CARTESIAN_POINT('',(-49.48928,-6.933,8.4904762584886E-16));
#27862=CARTESIAN_POINT('',(29.75,-6.933,-8.4904762584886E-16));
#27863=CARTESIAN_POINT('Origin',(-49.48928,0.,0.));
#27864=CARTESIAN_POINT('',(-16.,-6.60730572926666,2.1));
#27865=CARTESIAN_POINT('Origin',(-16.,0.,0.));
#27866=CARTESIAN_POINT('',(0.,-6.60730572926666,2.1));
#27867=CARTESIAN_POINT('',(29.75,-6.60730572926666,2.1));
#27868=CARTESIAN_POINT('Origin',(0.,0.,0.));
#27869=CARTESIAN_POINT('',(31.067,0.728796816009639,-6.89458803707475));
#27870=CARTESIAN_POINT('Origin',(31.067,0.,0.));
#27871=CARTESIAN_POINT('Ctrl Pts',(31.067,0.728796816009639,-6.89458803707475));
#27872=CARTESIAN_POINT('Ctrl Pts',(31.100085267407,1.87539916180616,-6.77338570644206));
#27873=CARTESIAN_POINT('Ctrl Pts',(31.133170534814,2.9888184467541,-6.36193732933414));
#27874=CARTESIAN_POINT('Ctrl Pts',(31.166255802221,3.93811726940023,-5.70670201568804));
#27875=CARTESIAN_POINT('Ctrl Pts',(31.199341069628,4.88741609204636,-5.05146670204194));
#27876=CARTESIAN_POINT('Ctrl Pts',(31.2324263370351,5.67259445239068,-4.15244445185767));
#27877=CARTESIAN_POINT('Ctrl Pts',(31.2655116044421,6.19093045690171,-3.12438071542469));
#27878=CARTESIAN_POINT('Ctrl Pts',(31.2985968718491,6.70926646141273,-2.09631697899172));
#27879=CARTESIAN_POINT('Ctrl Pts',(31.3316821392561,6.96076011009046,-0.93921175631004));
#27880=CARTESIAN_POINT('Ctrl Pts',(31.3647674066631,6.92655811692062,0.214382199295643));
#27881=CARTESIAN_POINT('Ctrl Pts',(31.3978526740702,6.89235612375078,1.36797615490133));
#27882=CARTESIAN_POINT('Ctrl Pts',(31.4309379414772,6.57245848873336,2.51805884343103));
#27883=CARTESIAN_POINT('Ctrl Pts',(31.4640232088842,5.9879843556759,3.50963197083578));
#27884=CARTESIAN_POINT('Ctrl Pts',(31.5301937436983,4.81903608956097,5.49277822564526));
#27885=CARTESIAN_POINT('Ctrl Pts',(31.5963642785123,2.59178183128585,6.84188623595496));
#27886=CARTESIAN_POINT('Ctrl Pts',(31.6625348133263,0.300319744218148,6.93899847482886));
#27887=CARTESIAN_POINT('Ctrl Pts',(31.7287053481403,-1.99114234284955,7.03611071370276));
#27888=CARTESIAN_POINT('Ctrl Pts',(31.7948758829544,-4.34681225870981,5.88122718114086));
#27889=CARTESIAN_POINT('Ctrl Pts',(31.8610464177684,-5.67194850391824,4.00941248465481));
#27890=CARTESIAN_POINT('Ctrl Pts',(31.9018803906436,-6.48969280120721,2.85431179280679));
#27891=CARTESIAN_POINT('Ctrl Pts',(31.9427143635188,-6.91499447673405,1.42619300013786));
#27892=CARTESIAN_POINT('Ctrl Pts',(31.9835483363939,-6.9206415740836,-0.000329640349373658));
#27893=CARTESIAN_POINT('',(-16.,6.60730572926666,-2.1));
#27894=CARTESIAN_POINT('',(0.,6.60730572926666,-2.1));
#27895=CARTESIAN_POINT('',(29.75,6.60730572926666,-2.1));
#27896=CARTESIAN_POINT('',(0.,6.60730572926666,2.1));
#27897=CARTESIAN_POINT('Origin',(0.,0.,0.));
#27898=CARTESIAN_POINT('',(-16.,6.60730572926666,2.1));
#27899=CARTESIAN_POINT('',(29.75,6.60730572926666,2.1));
#27900=CARTESIAN_POINT('Origin',(-16.,0.,0.));
#27901=CARTESIAN_POINT('Origin',(29.75,0.,0.));
#27902=CARTESIAN_POINT('',(33.4128916636063,-6.93491738431276,-0.000440937362671394));
#27903=CARTESIAN_POINT('',(33.2335483363939,-6.94245604902185,-0.00577606699965401));
#27904=CARTESIAN_POINT('',(29.75,-6.933,-8.4904762584886E-16));
#27905=CARTESIAN_POINT('Ctrl Pts',(33.4128916636063,-6.94109895177657,-0.00186250112332087));
#27906=CARTESIAN_POINT('Ctrl Pts',(33.3868687441823,-6.93819580024513,0.904044259585895));
#27907=CARTESIAN_POINT('Ctrl Pts',(33.3608458247584,-6.75124710452186,1.81227878197669));
#27908=CARTESIAN_POINT('Ctrl Pts',(33.3348229053344,-6.40214532506429,2.65136988785769));
#27909=CARTESIAN_POINT('Ctrl Pts',(33.3017376379274,-5.95830097626352,3.718181538182));
#27910=CARTESIAN_POINT('Ctrl Pts',(33.2686523705204,-5.25234729975987,4.67322760256061));
#27911=CARTESIAN_POINT('Ctrl Pts',(33.2355671031134,-4.35830135115629,5.39541883541299));
#27912=CARTESIAN_POINT('Ctrl Pts',(33.2024818357063,-3.46425540255271,6.11761006826537));
#27913=CARTESIAN_POINT('Ctrl Pts',(33.1693965682993,-2.38211718184919,6.60694646959151));
#27914=CARTESIAN_POINT('Ctrl Pts',(33.1363113008923,-1.24582538897172,6.81653407868776));
#27915=CARTESIAN_POINT('Ctrl Pts',(33.1032260334853,-0.109533596094221,
7.026121687784));
#27916=CARTESIAN_POINT('Ctrl Pts',(33.0701407660783,1.08091176895724,6.95596050465035));
#27917=CARTESIAN_POINT('Ctrl Pts',(33.0370554986712,2.17244432217632,6.59294758082586));
#27918=CARTESIAN_POINT('Ctrl Pts',(32.9708849638572,4.35550942861445,5.86692173317689));
#27919=CARTESIAN_POINT('Ctrl Pts',(32.9047144290432,6.14292328772306,3.96948892276462));
#27920=CARTESIAN_POINT('Ctrl Pts',(32.8385438942291,6.72047556257529,1.75078263924961));
#27921=CARTESIAN_POINT('Ctrl Pts',(32.7723733594151,7.29802783742751,-0.467923644265391));
#27922=CARTESIAN_POINT('Ctrl Pts',(32.706202824601,6.66571852802333,-3.00790340088312));
#27923=CARTESIAN_POINT('Ctrl Pts',(32.640032289787,5.11290677397241,-4.6996294346094));
#27924=CARTESIAN_POINT('Ctrl Pts',(32.573861754973,3.5600950199215,-6.39135546833568));
#27925=CARTESIAN_POINT('Ctrl Pts',(32.507691220159,1.08678082122384,-7.23482777917051));
#27926=CARTESIAN_POINT('Ctrl Pts',(32.4415206853449,-1.17608958629167,-6.84435685493866));
#27927=CARTESIAN_POINT('Ctrl Pts',(32.3753501505309,-3.43895999380719,-6.45388593070681));
#27928=CARTESIAN_POINT('Ctrl Pts',(32.3091796157168,-5.49138661014055,-4.82947177140826));
#27929=CARTESIAN_POINT('Ctrl Pts',(32.2430090809028,-6.38984874475651,-2.72020711315945));
#27930=CARTESIAN_POINT('Ctrl Pts',(32.2163032751373,-6.75245961562451,-1.86892772680491));
#27931=CARTESIAN_POINT('Ctrl Pts',(32.1895974693718,-6.92710655330198,-0.938673286853879));
#27932=CARTESIAN_POINT('Ctrl Pts',(32.1628916636063,-6.92198924261957,-0.00637899664044927));
#27933=CARTESIAN_POINT('Ctrl Pts',(31.9835483363939,-6.9206415740836,-0.000329640349373658));
#27934=CARTESIAN_POINT('Ctrl Pts',(32.0088848983328,-6.92414547100318,-0.885454860675154));
#27935=CARTESIAN_POINT('Ctrl Pts',(32.0342214602717,-6.76608556809867,-1.76996557463074));
#27936=CARTESIAN_POINT('Ctrl Pts',(32.0595580222106,-6.4399614979216,-2.58826217872326));
#27937=CARTESIAN_POINT('Ctrl Pts',(32.0926432896176,-6.01409858504077,-3.65681923196416));
#27938=CARTESIAN_POINT('Ctrl Pts',(32.1257285570246,-5.30165357208037,-4.61246834672295));
#27939=CARTESIAN_POINT('Ctrl Pts',(32.1588138244316,-4.40922992098058,-5.34619371087281));
#27940=CARTESIAN_POINT('Ctrl Pts',(32.1918990918386,-3.51680626988078,-6.07991907502267));
#27941=CARTESIAN_POINT('Ctrl Pts',(32.2249843592456,-2.44440398064157,-6.59172068856359));
#27942=CARTESIAN_POINT('Ctrl Pts',(32.2580696266526,-1.31579639281641,-6.80975252112529));
#27943=CARTESIAN_POINT('Ctrl Pts',(32.2911548940597,-0.187188804991247,
-7.02778435368699));
#27944=CARTESIAN_POINT('Ctrl Pts',(32.3242401614667,0.997624081419872,-6.95204640526946));
#27945=CARTESIAN_POINT('Ctrl Pts',(32.3573254288737,2.09923002332463,-6.60381125494117));
#27946=CARTESIAN_POINT('Ctrl Pts',(32.3904106962807,3.20083596522939,-6.25557610461289));
#27947=CARTESIAN_POINT('Ctrl Pts',(32.4234959636878,4.21923496262778,-5.63484375237386));
#27948=CARTESIAN_POINT('Ctrl Pts',(32.4565812310948,5.01276264886046,-4.80196364224421));
#27949=CARTESIAN_POINT('Ctrl Pts',(32.5227517659088,6.59981802132581,-3.13620342198489));
#27950=CARTESIAN_POINT('Ctrl Pts',(32.5889223007228,7.28738814912826,-0.621852170163068));
#27951=CARTESIAN_POINT('Ctrl Pts',(32.6550928355369,6.75595288246311,1.60835144458171));
#27952=CARTESIAN_POINT('Ctrl Pts',(32.7212633703509,6.22451761579797,3.83855505932649));
#27953=CARTESIAN_POINT('Ctrl Pts',(32.787433905165,4.47407695466521,5.78461103699422));
#27954=CARTESIAN_POINT('Ctrl Pts',(32.853604439979,2.30893373876081,6.549597885576));
#27955=CARTESIAN_POINT('Ctrl Pts',(32.919774974793,0.143790522856417,7.31458473415778));
#27956=CARTESIAN_POINT('Ctrl Pts',(32.9859455096071,-2.43605524781962,6.89850245365361));
#27957=CARTESIAN_POINT('Ctrl Pts',(33.0521160444211,-4.25094412584906,5.49161238079396));
#27958=CARTESIAN_POINT('Ctrl Pts',(33.1125934750787,-5.90968568779572,4.20576669338399));
#27959=CARTESIAN_POINT('Ctrl Pts',(33.1730709057363,-6.92943684460085,2.09227087465205));
#27960=CARTESIAN_POINT('Ctrl Pts',(33.2335483363939,-6.94245604902185,-0.00577606699965401));
#27961=CARTESIAN_POINT('Origin',(29.75,0.,0.));
#27962=CARTESIAN_POINT('',(34.6628916636063,-6.933,1.97064586870965E-14));
#27963=CARTESIAN_POINT('',(34.4835483363939,-6.93389555109049,0.00595474732503822));
#27964=CARTESIAN_POINT('',(29.75,-6.933,-8.4904762584886E-16));
#27965=CARTESIAN_POINT('Ctrl Pts',(34.6628916636063,-6.933,-4.9960036108132E-15));
#27966=CARTESIAN_POINT('Ctrl Pts',(34.6056674683212,-6.933,1.99420935701628));
#27967=CARTESIAN_POINT('Ctrl Pts',(34.5484432730361,-6.02307502629249,3.97063309653046));
#27968=CARTESIAN_POINT('Ctrl Pts',(34.491219077751,-4.50798484753983,5.26731066241125));
#27969=CARTESIAN_POINT('Ctrl Pts',(34.4339948824659,-2.99289466878718,6.56398822829205));
#27970=CARTESIAN_POINT('Ctrl Pts',(34.3767706871808,-0.899664345628758,
7.15779044292411));
#27971=CARTESIAN_POINT('Ctrl Pts',(34.3195464918957,1.07062371681849,6.84983604599305));
#27972=CARTESIAN_POINT('Ctrl Pts',(34.2623222966106,3.04091177926574,6.541881649062));
#27973=CARTESIAN_POINT('Ctrl Pts',(34.2050981013255,4.85311303639886,5.33766370386397));
#27974=CARTESIAN_POINT('Ctrl Pts',(34.1478739060404,5.90026971493765,3.64050907030729));
#27975=CARTESIAN_POINT('Ctrl Pts',(34.0906497107553,6.94742639347644,1.9433544367506));
#27976=CARTESIAN_POINT('Ctrl Pts',(34.0334255154702,7.2108600852751,-0.216464293124));
#27977=CARTESIAN_POINT('Ctrl Pts',(33.9762013201851,6.6023393500608,-2.11556236179385));
#27978=CARTESIAN_POINT('Ctrl Pts',(33.9189771249,5.99381861484649,-4.0146604304637));
#27979=CARTESIAN_POINT('Ctrl Pts',(33.8617529296149,4.52419779647289,-5.61916312790447));
#27980=CARTESIAN_POINT('Ctrl Pts',(33.8045287343298,2.68569473000394,-6.39167683923625));
#27981=CARTESIAN_POINT('Ctrl Pts',(33.7473045390447,0.847191663535,-7.16419055056802));
#27982=CARTESIAN_POINT('Ctrl Pts',(33.6900803437597,-1.32739978994181,-7.09093574623785));
#27983=CARTESIAN_POINT('Ctrl Pts',(33.6328561484746,-3.10974706736201,-6.19644754492712));
#27984=CARTESIAN_POINT('Ctrl Pts',(33.5756319531895,-4.89209434478221,-5.3019593436164));
#27985=CARTESIAN_POINT('Ctrl Pts',(33.5184077579044,-6.25040525058661,-3.6021929658266));
#27986=CARTESIAN_POINT('Ctrl Pts',(33.4611835626193,-6.72974280712766,-1.66644854403415));
#27987=CARTESIAN_POINT('Ctrl Pts',(33.4450862629483,-6.86458158035574,-1.12191912096727));
#27988=CARTESIAN_POINT('Ctrl Pts',(33.4289889632773,-6.933,-0.560975745778045));
#27989=CARTESIAN_POINT('Ctrl Pts',(33.4128916636063,-6.933,-1.9151347174784E-14));
#27990=CARTESIAN_POINT('Ctrl Pts',(33.2335483363939,-6.94245604902185,-0.00577606699965401));
#27991=CARTESIAN_POINT('Ctrl Pts',(33.2392414405504,-6.9436816250094,-0.203277839711076));
#27992=CARTESIAN_POINT('Ctrl Pts',(33.2449345447068,-6.93598595639073,-0.400642710826199));
#27993=CARTESIAN_POINT('Ctrl Pts',(33.2506276488632,-6.91906227514061,-0.597167371676744));
#27994=CARTESIAN_POINT('Ctrl Pts',(33.3167981836772,-6.72235956101991,-2.88135918607271));
#27995=CARTESIAN_POINT('Ctrl Pts',(33.3829687184913,-5.27902214739564,-5.05204494964951));
#27996=CARTESIAN_POINT('Ctrl Pts',(33.4491392533053,-3.24890903512377,-6.13441620840687));
#27997=CARTESIAN_POINT('Ctrl Pts',(33.4822245207123,-2.23385247898783,-6.67560183778555));
#27998=CARTESIAN_POINT('Ctrl Pts',(33.5153097881194,-1.07210199819001,-6.94470884095935));
#27999=CARTESIAN_POINT('Ctrl Pts',(33.5483950555264,0.0832496906585477,
-6.92894560771863));
#28000=CARTESIAN_POINT('Ctrl Pts',(33.5814803229334,1.2386013795071,-6.91318237447791));
#28001=CARTESIAN_POINT('Ctrl Pts',(33.6145655903404,2.38755427640638,-6.61254890482264));
#28002=CARTESIAN_POINT('Ctrl Pts',(33.6476508577474,3.39019622543778,-6.05077719223303));
#28003=CARTESIAN_POINT('Ctrl Pts',(33.6807361251545,4.39283817446916,-5.48900547964343));
#28004=CARTESIAN_POINT('Ctrl Pts',(33.7138213925615,5.24916917563268,-4.6660955241195));
#28005=CARTESIAN_POINT('Ctrl Pts',(33.7469066599685,5.86588595288536,-3.68898482420616));
#28006=CARTESIAN_POINT('Ctrl Pts',(33.7799919273755,6.48260273013804,-2.71187412429283));
#28007=CARTESIAN_POINT('Ctrl Pts',(33.8130771947825,6.85970528347988,-1.58056267999009));
#28008=CARTESIAN_POINT('Ctrl Pts',(33.8461624621895,6.92817161952915,-0.432288782485585));
#28009=CARTESIAN_POINT('Ctrl Pts',(33.9123329970036,7.06510429162769,1.86425901252342));
#28010=CARTESIAN_POINT('Ctrl Pts',(33.9785035318176,5.96749209455592,4.22865662033947));
#28011=CARTESIAN_POINT('Ctrl Pts',(34.0446740666317,4.12212534563731,5.58911513351279));
#28012=CARTESIAN_POINT('Ctrl Pts',(34.1108446014457,2.2767585967187,6.94957364668611));
#28013=CARTESIAN_POINT('Ctrl Pts',(34.1770151362597,-0.316362704046755,
7.30609306521667));
#28014=CARTESIAN_POINT('Ctrl Pts',(34.2431856710738,-2.46387742523262,6.49288633327678));
#28015=CARTESIAN_POINT('Ctrl Pts',(34.3093562058878,-4.61139214641846,5.67967960133689));
#28016=CARTESIAN_POINT('Ctrl Pts',(34.3755267407019,-6.31330028802472,3.69674671892656));
#28017=CARTESIAN_POINT('Ctrl Pts',(34.4416972755159,-6.79143541399258,1.45074781472781));
#28018=CARTESIAN_POINT('Ctrl Pts',(34.4556476291419,-6.89223789514245,0.977236771704476));
#28019=CARTESIAN_POINT('Ctrl Pts',(34.4695979827679,-6.93864750106136,0.492033268463616));
#28020=CARTESIAN_POINT('Ctrl Pts',(34.4835483363939,-6.93389555109049,0.00595474732503822));
#28021=CARTESIAN_POINT('Origin',(29.75,0.,0.));
#28022=CARTESIAN_POINT('',(35.9128916636063,-6.92960145208156,-0.00126819834722902));
#28023=CARTESIAN_POINT('',(35.7335483363939,-6.92339125407611,-0.000268698171690447));
#28024=CARTESIAN_POINT('',(29.75,-6.933,-8.4904762584886E-16));
#28025=CARTESIAN_POINT('Ctrl Pts',(35.9128916636063,-6.92960145208156,-0.00126819834722902));
#28026=CARTESIAN_POINT('Ctrl Pts',(35.8806670960245,-6.9318585040595,1.1242479907601));
#28027=CARTESIAN_POINT('Ctrl Pts',(35.8484425284426,-6.6641919565166,2.25237223453277));
#28028=CARTESIAN_POINT('Ctrl Pts',(35.8162179608608,-6.13825503570355,3.2416449596582));
#28029=CARTESIAN_POINT('Ctrl Pts',(35.7500474260468,-5.05828624356125,5.27303623069012));
#28030=CARTESIAN_POINT('Ctrl Pts',(35.6838768912328,-2.88931292936768,6.71895604486874));
#28031=CARTESIAN_POINT('Ctrl Pts',(35.6177063564187,-0.605354648845225,
6.91835745444872));
#28032=CARTESIAN_POINT('Ctrl Pts',(35.5515358216047,1.67860363167723,7.11775886402871));
#28033=CARTESIAN_POINT('Ctrl Pts',(35.4853652867906,4.07754687852859,6.07064186901007));
#28034=CARTESIAN_POINT('Ctrl Pts',(35.4191947519766,5.48658138221935,4.25742756644304));
#28035=CARTESIAN_POINT('Ctrl Pts',(35.3530242171625,6.89561588591012,2.444213263876));
#28036=CARTESIAN_POINT('Ctrl Pts',(35.2868536823485,7.31474164644029,-0.135098346239444));
#28037=CARTESIAN_POINT('Ctrl Pts',(35.2206831475345,6.55232099334528,-2.30116369306058));
#28038=CARTESIAN_POINT('Ctrl Pts',(35.1545126127204,5.78990034025028,-4.46722903988171));
#28039=CARTESIAN_POINT('Ctrl Pts',(35.0883420779064,3.84593327353012,-6.22004812340854));
#28040=CARTESIAN_POINT('Ctrl Pts',(35.0221715430924,1.6163501133428,-6.75407554214492));
#28041=CARTESIAN_POINT('Ctrl Pts',(34.9560010082783,-0.613233046844523,
-7.2881029608813));
#28042=CARTESIAN_POINT('Ctrl Pts',(34.8898304734643,-3.128432300499,-6.60333871482723));
#28043=CARTESIAN_POINT('Ctrl Pts',(34.8236599386502,-4.79603498530099,-5.01841462544935));
#28044=CARTESIAN_POINT('Ctrl Pts',(34.7905746712432,-5.62983632770198,-4.22595258076041));
#28045=CARTESIAN_POINT('Ctrl Pts',(34.7574894038362,-6.25173852788985,-3.20845057524052));
#28046=CARTESIAN_POINT('Ctrl Pts',(34.7244041364292,-6.60130234039749,-2.10713804160215));
#28047=CARTESIAN_POINT('Ctrl Pts',(34.7038999788215,-6.81793989745299,-1.42461414094293));
#28048=CARTESIAN_POINT('Ctrl Pts',(34.6833958212139,-6.92997944340521,-0.709900820990376));
#28049=CARTESIAN_POINT('Ctrl Pts',(34.6628916636063,-6.93227389215358,0.00361668279959731));
#28050=CARTESIAN_POINT('Ctrl Pts',(34.4835483363939,-6.93389555109049,0.00595474732503822));
#28051=CARTESIAN_POINT('Ctrl Pts',(34.535768517582,-6.91610763724059,-1.81357679473825));
#28052=CARTESIAN_POINT('Ctrl Pts',(34.58798869877,-6.18143378983398,-3.64536926224785));
#28053=CARTESIAN_POINT('Ctrl Pts',(34.640208879958,-4.89936216432684,-4.92202954051599));
#28054=CARTESIAN_POINT('Ctrl Pts',(34.706379414772,-3.27479167836381,-6.53974306557382));
#28055=CARTESIAN_POINT('Ctrl Pts',(34.7725499495861,-0.771288596108303,
-7.26610518970229));
#28056=CARTESIAN_POINT('Ctrl Pts',(34.8387204844001,1.47793304890319,-6.78248854273389));
#28057=CARTESIAN_POINT('Ctrl Pts',(34.8718057518071,2.60254387140893,-6.54068021924969));
#28058=CARTESIAN_POINT('Ctrl Pts',(34.9048910192141,3.66358433460367,-5.99637720299127));
#28059=CARTESIAN_POINT('Ctrl Pts',(34.9379762866212,4.53587037073918,-5.2386165409355));
#28060=CARTESIAN_POINT('Ctrl Pts',(34.9710615540282,5.40815640687468,-4.48085587887973));
#28061=CARTESIAN_POINT('Ctrl Pts',(35.0041468214352,6.09168801595097,-3.50963757102659));
#28062=CARTESIAN_POINT('Ctrl Pts',(35.0372320888422,6.49491391291778,-2.43339928941026));
#28063=CARTESIAN_POINT('Ctrl Pts',(35.0703173562492,6.8981398098846,-1.35716100779393));
#28064=CARTESIAN_POINT('Ctrl Pts',(35.1034026236563,7.02105999474195,-0.175902752414387));
#28065=CARTESIAN_POINT('Ctrl Pts',(35.1364878910633,6.8614340140831,0.968476425158562));
#28066=CARTESIAN_POINT('Ctrl Pts',(35.1695731584703,6.70180803342424,2.11285560273151));
#28067=CARTESIAN_POINT('Ctrl Pts',(35.2026584258773,6.2596358872492,3.22035570249786));
#28068=CARTESIAN_POINT('Ctrl Pts',(35.2357436932843,5.57077791340997,4.14160239190325));
#28069=CARTESIAN_POINT('Ctrl Pts',(35.3019142280984,4.19306196573149,5.98409577071403));
#28070=CARTESIAN_POINT('Ctrl Pts',(35.3680847629124,1.82860270739628,7.08157550808095));
#28071=CARTESIAN_POINT('Ctrl Pts',(35.4342552977264,-0.459001209328522,
6.92960619427528));
#28072=CARTESIAN_POINT('Ctrl Pts',(35.5004258325405,-2.74660512605329,6.77763688046961));
#28073=CARTESIAN_POINT('Ctrl Pts',(35.5665963673545,-4.95735370116766,5.37621851549137));
#28074=CARTESIAN_POINT('Ctrl Pts',(35.6327669021686,-6.07274754602132,3.36897640009331));
#28075=CARTESIAN_POINT('Ctrl Pts',(35.666360713577,-6.63901666528224,2.34992897565731));
#28076=CARTESIAN_POINT('Ctrl Pts',(35.6999545249855,-6.92296421607281,1.17473386069699));
#28077=CARTESIAN_POINT('Ctrl Pts',(35.7335483363939,-6.92339125407611,-0.000268698171690447));
#28078=CARTESIAN_POINT('Origin',(29.75,0.,0.));
#28079=CARTESIAN_POINT('',(37.1628916636063,-6.93290463700014,-0.000100259380880677));
#28080=CARTESIAN_POINT('',(36.9835483363939,-6.93502389967407,-0.00589331438187145));
#28081=CARTESIAN_POINT('',(29.75,-6.933,-8.4904762584886E-16));
#28082=CARTESIAN_POINT('Ctrl Pts',(37.1628916636063,-6.92971491769494,-0.00345375376834933));
#28083=CARTESIAN_POINT('Ctrl Pts',(37.111023638242,-6.91260075130355,1.80429354156629));
#28084=CARTESIAN_POINT('Ctrl Pts',(37.0591556128777,-6.19436612714247,3.61861004078152));
#28085=CARTESIAN_POINT('Ctrl Pts',(37.0072875875135,-4.92782277232531,4.89353520916524));
#28086=CARTESIAN_POINT('Ctrl Pts',(36.9411170526994,-3.31203249373178,6.52001857049164));
#28087=CARTESIAN_POINT('Ctrl Pts',(36.8749465178854,-0.803851543980656,
7.26862462506543));
#28088=CARTESIAN_POINT('Ctrl Pts',(36.8087759830714,1.44271150104494,6.79314715502428));
#28089=CARTESIAN_POINT('Ctrl Pts',(36.7426054482574,3.68927454607051,6.31766968498313));
#28090=CARTESIAN_POINT('Ctrl Pts',(36.6764349134433,5.67421968637056,4.61810869032707));
#28091=CARTESIAN_POINT('Ctrl Pts',(36.6102643786292,6.48996666690957,2.47155768847992));
#28092=CARTESIAN_POINT('Ctrl Pts',(36.5440938438152,7.30571364744857,0.325006686632785));
#28093=CARTESIAN_POINT('Ctrl Pts',(36.4779233090012,6.95226246822655,-2.26853432240543));
#28094=CARTESIAN_POINT('Ctrl Pts',(36.4117527741872,5.59398829109631,-4.115509581796));
#28095=CARTESIAN_POINT('Ctrl Pts',(36.3455822393731,4.23571411396608,-5.96248484118655));
#28096=CARTESIAN_POINT('Ctrl Pts',(36.2794117045591,1.87261693892766,-7.06289435092948));
#28097=CARTESIAN_POINT('Ctrl Pts',(36.213241169745,-0.424091389993473,-6.92867833148972));
#28098=CARTESIAN_POINT('Ctrl Pts',(36.180155902338,-1.57244555445406,-6.86157032176984));
#28099=CARTESIAN_POINT('Ctrl Pts',(36.147070634931,-2.70420250738532,-6.48580592975427));
#28100=CARTESIAN_POINT('Ctrl Pts',(36.113985367524,-3.68204209515384,-5.87024610598754));
#28101=CARTESIAN_POINT('Ctrl Pts',(36.0809001001169,-4.65988168292234,-5.25468628222081));
#28102=CARTESIAN_POINT('Ctrl Pts',(36.0478148327099,-5.4838039055281,-4.39933102670292));
#28103=CARTESIAN_POINT('Ctrl Pts',(36.0147295653029,-6.04676165595723,-3.39735371629919));
#28104=CARTESIAN_POINT('Ctrl Pts',(35.9816442978959,-6.60971940638636,-2.39537640589547));
#28105=CARTESIAN_POINT('Ctrl Pts',(35.9485590304889,-6.91171268463887,-1.24677704060591));
#28106=CARTESIAN_POINT('Ctrl Pts',(35.9154737630819,-6.92884269098595,-0.0914456080964819));
#28107=CARTESIAN_POINT('Ctrl Pts',(35.9146130632567,-6.92928832115987,-0.0613901290286256));
#28108=CARTESIAN_POINT('Ctrl Pts',(35.9137523634315,-6.92954116751024,-0.0313300939727322));
#28109=CARTESIAN_POINT('Ctrl Pts',(35.9128916636063,-6.92960145208156,-0.00126819834722902));
#28110=CARTESIAN_POINT('Ctrl Pts',(35.7335483363939,-6.92339125407611,-0.000268698171690447));
#28111=CARTESIAN_POINT('Ctrl Pts',(35.7661250597995,-6.92380536305433,-1.1396968177055));
#28112=CARTESIAN_POINT('Ctrl Pts',(35.7987017832051,-6.65760683712713,-2.27894386431991));
#28113=CARTESIAN_POINT('Ctrl Pts',(35.8312785066107,-6.12370236615607,-3.27544410392846));
#28114=CARTESIAN_POINT('Ctrl Pts',(35.8974490414247,-5.03922422684416,-5.29955662673429));
#28115=CARTESIAN_POINT('Ctrl Pts',(35.9636195762388,-2.85022883362737,-6.73471580652803));
#28116=CARTESIAN_POINT('Ctrl Pts',(36.0297901110528,-0.565224684335127,
-6.92175159729262));
#28117=CARTESIAN_POINT('Ctrl Pts',(36.0959606458668,1.7197794649571,-7.10878738805721));
#28118=CARTESIAN_POINT('Ctrl Pts',(36.1621311806808,4.10079237032479,-6.04769978979263));
#28119=CARTESIAN_POINT('Ctrl Pts',(36.2283017154949,5.50660409421191,-4.22655276524806));
#28120=CARTESIAN_POINT('Ctrl Pts',(36.2613869829019,6.20950995615547,-3.31597925297579));
#28121=CARTESIAN_POINT('Ctrl Pts',(36.2944722503089,6.66861552272889,-2.21539088413354));
#28122=CARTESIAN_POINT('Ctrl Pts',(36.3275575177159,6.84577375546842,-1.07359444140203));
#28123=CARTESIAN_POINT('Ctrl Pts',(36.360642785123,7.02293198820795,0.068202001329485));
#28124=CARTESIAN_POINT('Ctrl Pts',(36.39372805253,6.91814288711357,1.25120651795023));
#28125=CARTESIAN_POINT('Ctrl Pts',(36.426813319937,6.5314703880391,2.33350238220899));
#28126=CARTESIAN_POINT('Ctrl Pts',(36.459898587344,6.14479788896462,3.41579824646776));
#28127=CARTESIAN_POINT('Ctrl Pts',(36.492983854751,5.47624199191003,4.39738545836455));
#28128=CARTESIAN_POINT('Ctrl Pts',(36.5260691221581,4.61568011269898,5.16843500806403));
#28129=CARTESIAN_POINT('Ctrl Pts',(36.5591543895651,3.75511823348794,5.93948455776351));
#28130=CARTESIAN_POINT('Ctrl Pts',(36.5922396569721,2.70255037212044,6.49999644526569));
#28131=CARTESIAN_POINT('Ctrl Pts',(36.6253249243791,1.58178036580302,6.759024175329));
#28132=CARTESIAN_POINT('Ctrl Pts',(36.6914954591931,-0.659759646831825,
7.27707963545561));
#28133=CARTESIAN_POINT('Ctrl Pts',(36.7576659940072,-3.17410823926632,6.58919846582668));
#28134=CARTESIAN_POINT('Ctrl Pts',(36.8238365288212,-4.82329809281977,4.99659080039366));
#28135=CARTESIAN_POINT('Ctrl Pts',(36.8770737980121,-6.15014794263986,3.71526394942559));
#28136=CARTESIAN_POINT('Ctrl Pts',(36.930311067203,-6.91698486849107,1.84831216335871));
#28137=CARTESIAN_POINT('Ctrl Pts',(36.9835483363939,-6.93502389967407,-0.00589331438187144));
#28138=CARTESIAN_POINT('Origin',(29.75,0.,0.));
#28139=CARTESIAN_POINT('',(38.4128916636063,-6.93577359535222,0.000670304473996572));
#28140=CARTESIAN_POINT('',(38.2335483363939,-6.94167024712608,0.00637861567201024));
#28141=CARTESIAN_POINT('',(29.75,-6.933,-8.4904762584886E-16));
#28142=CARTESIAN_POINT('Ctrl Pts',(38.4128916636063,-6.933,2.77555756156289E-16));
#28143=CARTESIAN_POINT('Ctrl Pts',(38.3556674683212,-6.933,1.99420935701628));
#28144=CARTESIAN_POINT('Ctrl Pts',(38.2984432730361,-6.02307502629249,3.97063309653045));
#28145=CARTESIAN_POINT('Ctrl Pts',(38.241219077751,-4.50798484753985,5.26731066241124));
#28146=CARTESIAN_POINT('Ctrl Pts',(38.1839948824659,-2.9928946687872,6.56398822829204));
#28147=CARTESIAN_POINT('Ctrl Pts',(38.1267706871808,-0.899664345628795,
7.1577904429241));
#28148=CARTESIAN_POINT('Ctrl Pts',(38.0695464918957,1.07062371681845,6.84983604599306));
#28149=CARTESIAN_POINT('Ctrl Pts',(38.0123222966106,3.04091177926569,6.54188164906202));
#28150=CARTESIAN_POINT('Ctrl Pts',(37.9550981013255,4.85311303639881,5.33766370386401));
#28151=CARTESIAN_POINT('Ctrl Pts',(37.8978739060404,5.90026971493761,3.64050907030734));
#28152=CARTESIAN_POINT('Ctrl Pts',(37.8406497107553,6.94742639347642,1.94335443675068));
#28153=CARTESIAN_POINT('Ctrl Pts',(37.7834255154702,7.2108600852751,-0.216464293123911));
#28154=CARTESIAN_POINT('Ctrl Pts',(37.7262013201851,6.60233935006083,-2.11556236179376));
#28155=CARTESIAN_POINT('Ctrl Pts',(37.6689771249,5.99381861484655,-4.01466043046361));
#28156=CARTESIAN_POINT('Ctrl Pts',(37.611752929615,4.52419779647298,-5.6191631279044));
#28157=CARTESIAN_POINT('Ctrl Pts',(37.5545287343298,2.68569473000405,-6.3916768392362));
#28158=CARTESIAN_POINT('Ctrl Pts',(37.4973045390448,0.847191663535129,-7.164190550568));
#28159=CARTESIAN_POINT('Ctrl Pts',(37.4400803437597,-1.32739978994167,-7.09093574623788));
#28160=CARTESIAN_POINT('Ctrl Pts',(37.3828561484746,-3.10974706736188,-6.19644754492719));
#28161=CARTESIAN_POINT('Ctrl Pts',(37.3256319531895,-4.89209434478209,-5.3019593436165));
#28162=CARTESIAN_POINT('Ctrl Pts',(37.2684077579044,-6.25040525058653,-3.60219296582674));
#28163=CARTESIAN_POINT('Ctrl Pts',(37.2111835626193,-6.72974280712762,-1.66644854403432));
#28164=CARTESIAN_POINT('Ctrl Pts',(37.1950862629483,-6.86458158035574,-1.12191912096732));
#28165=CARTESIAN_POINT('Ctrl Pts',(37.1789889632773,-6.93300000000001,-0.56097574577799));
#28166=CARTESIAN_POINT('Ctrl Pts',(37.1628916636063,-6.933,1.46271883494364E-13));
#28167=CARTESIAN_POINT('Ctrl Pts',(36.9835483363939,-6.93502389967407,-0.00589331438187144));
#28168=CARTESIAN_POINT('Ctrl Pts',(36.996481602017,-6.93940623530886,-0.45634714734448));
#28169=CARTESIAN_POINT('Ctrl Pts',(37.0094148676402,-6.89959597956175,-0.906048718048468));
#28170=CARTESIAN_POINT('Ctrl Pts',(37.0223481332633,-6.81288640392014,-1.34641880273624));
#28171=CARTESIAN_POINT('Ctrl Pts',(37.0885186680774,-6.36925374679465,-3.59948657919598));
#28172=CARTESIAN_POINT('Ctrl Pts',(37.1546892028914,-4.69795731787126,-5.60828797087832));
#28173=CARTESIAN_POINT('Ctrl Pts',(37.2208597377055,-2.56316717324256,-6.45433488339996));
#28174=CARTESIAN_POINT('Ctrl Pts',(37.2870302725195,-0.428377028613836,
-7.3003817959216));
#28175=CARTESIAN_POINT('Ctrl Pts',(37.3532008073335,2.1699068317202,-6.98367422928253));
#28176=CARTESIAN_POINT('Ctrl Pts',(37.4193713421476,4.03592169067489,-5.65167764699365));
#28177=CARTESIAN_POINT('Ctrl Pts',(37.4855418769616,5.90193654962956,-4.31968106470479));
#28178=CARTESIAN_POINT('Ctrl Pts',(37.5517124117756,7.03568240720489,-1.97239546676614));
#28179=CARTESIAN_POINT('Ctrl Pts',(37.6178829465897,6.93398675840259,0.325982457550818));
#28180=CARTESIAN_POINT('Ctrl Pts',(37.6509682139967,6.88313893400144,1.47517141970932));
#28181=CARTESIAN_POINT('Ctrl Pts',(37.6840534814037,6.52343073300587,2.61213346346238));
#28182=CARTESIAN_POINT('Ctrl Pts',(37.7171387488107,5.92177261965832,3.59858755296438));
#28183=CARTESIAN_POINT('Ctrl Pts',(37.7502240162178,5.32011450631077,4.58504164246637));
#28184=CARTESIAN_POINT('Ctrl Pts',(37.7833092836248,4.47650648061124,5.42098777771728));
#28185=CARTESIAN_POINT('Ctrl Pts',(37.8163945510318,3.48259747344794,5.99807082616737));
#28186=CARTESIAN_POINT('Ctrl Pts',(37.8494798184388,2.48868846628466,6.57515387461745));
#28187=CARTESIAN_POINT('Ctrl Pts',(37.8825650858458,1.34447847765756,6.89337383626672));
#28188=CARTESIAN_POINT('Ctrl Pts',(37.9156503532529,0.18950522617225,6.92685434411176));
#28189=CARTESIAN_POINT('Ctrl Pts',(37.9487356206599,-0.965468025313094,
6.96033485195681));
#28190=CARTESIAN_POINT('Ctrl Pts',(37.9818208880669,-2.13120453965668,6.70907590599762));
#28191=CARTESIAN_POINT('Ctrl Pts',(38.0149061554739,-3.15444121278794,6.18352145329789));
#28192=CARTESIAN_POINT('Ctrl Pts',(38.0810766902879,-5.2009145590504,5.13241254789846));
#28193=CARTESIAN_POINT('Ctrl Pts',(38.147247225102,-6.6773885404635,2.98412161553692));
#28194=CARTESIAN_POINT('Ctrl Pts',(38.213417759916,-6.90909644225956,0.703214384342509));
#28195=CARTESIAN_POINT('Ctrl Pts',(38.2201279520753,-6.93259337409259,0.471913158474033));
#28196=CARTESIAN_POINT('Ctrl Pts',(38.2268381442346,-6.94328976360018,0.239248173925071));
#28197=CARTESIAN_POINT('Ctrl Pts',(38.2335483363939,-6.94167024712608,0.00637861567201024));
#28198=CARTESIAN_POINT('Origin',(29.75,0.,0.));
#28199=CARTESIAN_POINT('',(39.6628916636063,-6.92332261655204,0.00297343908938319));
#28200=CARTESIAN_POINT('',(39.4835483363939,-6.92769178317914,-6.1482564198808E-5));
#28201=CARTESIAN_POINT('',(29.75,-6.933,-8.4904762584886E-16));
#28202=CARTESIAN_POINT('Ctrl Pts',(39.6628916636063,-6.92332261655204,0.00297343908938319));
#28203=CARTESIAN_POINT('Ctrl Pts',(39.6379072574912,-6.92850463656999,0.8768019092153));
#28204=CARTESIAN_POINT('Ctrl Pts',(39.612922851376,-6.77585609379785,1.74910600870471));
#28205=CARTESIAN_POINT('Ctrl Pts',(39.5879384452609,-6.45736297806441,2.55552893049358));
#28206=CARTESIAN_POINT('Ctrl Pts',(39.5217679104469,-5.61384243546796,4.69131858165475));
#28207=CARTESIAN_POINT('Ctrl Pts',(39.4555973756329,-3.60701984478563,6.36499055491544));
#28208=CARTESIAN_POINT('Ctrl Pts',(39.3894268408188,-1.35447852944345,6.81128861951564));
#28209=CARTESIAN_POINT('Ctrl Pts',(39.3232563060048,0.898062785898749,7.25758668411585));
#28210=CARTESIAN_POINT('Ctrl Pts',(39.2570857711907,3.39632282590077,6.47651084005551));
#28211=CARTESIAN_POINT('Ctrl Pts',(39.1909152363767,4.9908806162241,4.82920643515976));
#28212=CARTESIAN_POINT('Ctrl Pts',(39.1247447015627,6.58543840654742,3.18190203026401));
#28213=CARTESIAN_POINT('Ctrl Pts',(39.0585741667487,7.27629394719206,0.668369064532852));
#28214=CARTESIAN_POINT('Ctrl Pts',(38.9924036319346,6.76089092856649,-1.57378231670003));
#28215=CARTESIAN_POINT('Ctrl Pts',(38.9593183645276,6.5031894192537,-2.69485800731648));
#28216=CARTESIAN_POINT('Ctrl Pts',(38.9262330971205,5.94392327012335,-3.74808830180835));
#28217=CARTESIAN_POINT('Ctrl Pts',(38.8931478297135,5.17389243420951,-4.60956184626221));
#28218=CARTESIAN_POINT('Ctrl Pts',(38.8600625623065,4.40386159829564,-5.47103539071609));
#28219=CARTESIAN_POINT('Ctrl Pts',(38.8269772948995,3.42306607559827,-6.14075218513195));
#28220=CARTESIAN_POINT('Ctrl Pts',(38.7938920274925,2.34122846057253,-6.52870493231168));
#28221=CARTESIAN_POINT('Ctrl Pts',(38.7608067600855,1.25939084554681,-6.9166576794914));
#28222=CARTESIAN_POINT('Ctrl Pts',(38.7277214926785,0.0765111381927339,
-7.02284637943501));
#28223=CARTESIAN_POINT('Ctrl Pts',(38.6946362252715,-1.06549411019643,-6.84703918759221));
#28224=CARTESIAN_POINT('Ctrl Pts',(38.6615509578644,-2.20749935858561,-6.67123199574941));
#28225=CARTESIAN_POINT('Ctrl Pts',(38.6284656904574,-3.30863014800987,-6.21342891212019));
#28226=CARTESIAN_POINT('Ctrl Pts',(38.5953804230504,-4.22003466628295,-5.51160088755531));
#28227=CARTESIAN_POINT('Ctrl Pts',(38.534550836569,-5.89571584732849,-4.22124080099123));
#28228=CARTESIAN_POINT('Ctrl Pts',(38.4737212500876,-6.93005765768905,-2.10599335907293));
#28229=CARTESIAN_POINT('Ctrl Pts',(38.4128916636063,-6.94291148540326,0.00239534328771114));
#28230=CARTESIAN_POINT('Ctrl Pts',(38.2335483363939,-6.94167024712608,0.00637861567201024));
#28231=CARTESIAN_POINT('Ctrl Pts',(38.2930086790487,-6.92731939066792,-2.05712469375046));
#28232=CARTESIAN_POINT('Ctrl Pts',(38.3524690217034,-5.94591333167301,-4.1366913009233));
#28233=CARTESIAN_POINT('Ctrl Pts',(38.4119293643581,-4.33465654613917,-5.42577343538037));
#28234=CARTESIAN_POINT('Ctrl Pts',(38.4780998991722,-2.54156692604374,-6.86033049388152));
#28235=CARTESIAN_POINT('Ctrl Pts',(38.5442704339862,0.031554136326008,-7.31592108085652));
#28236=CARTESIAN_POINT('Ctrl Pts',(38.6104409688002,2.20819358647839,-6.58423464266746));
#28237=CARTESIAN_POINT('Ctrl Pts',(38.6766115036143,4.38483303663073,-5.8525482044784));
#28238=CARTESIAN_POINT('Ctrl Pts',(38.7427820384283,6.16499087456564,-3.93358474112524));
#28239=CARTESIAN_POINT('Ctrl Pts',(38.8089525732423,6.73052165696255,-1.71178338114024));
#28240=CARTESIAN_POINT('Ctrl Pts',(38.8751231080564,7.29605243935946,0.510017978844769));
#28241=CARTESIAN_POINT('Ctrl Pts',(38.9412936428704,6.64695616621838,3.03465723546165));
#28242=CARTESIAN_POINT('Ctrl Pts',(39.0074641776845,5.08579358974434,4.72452542493378));
#28243=CARTESIAN_POINT('Ctrl Pts',(39.0405494450915,4.3052123015073,5.56945951966986));
#28244=CARTESIAN_POINT('Ctrl Pts',(39.0736347124985,3.29661443743698,6.20570084761976));
#28245=CARTESIAN_POINT('Ctrl Pts',(39.1067199799055,2.20035984233609,6.57081729311669));
#28246=CARTESIAN_POINT('Ctrl Pts',(39.1398052473125,1.10410524723521,6.93593373861362));
#28247=CARTESIAN_POINT('Ctrl Pts',(39.1728905147195,-0.0798060788962004,
7.0299253016576));
#28248=CARTESIAN_POINT('Ctrl Pts',(39.2059757821266,-1.21143464275791,6.82918479059629));
#28249=CARTESIAN_POINT('Ctrl Pts',(39.2390610495336,-2.34306320661961,6.62844427953498));
#28250=CARTESIAN_POINT('Ctrl Pts',(39.2721463169406,-3.42240900821157,6.13297169436833));
#28251=CARTESIAN_POINT('Ctrl Pts',(39.3052315843476,-4.32619084933698,5.41306715923603));
#28252=CARTESIAN_POINT('Ctrl Pts',(39.3383168517546,-5.22997269046238,4.69316262410372));
#28253=CARTESIAN_POINT('Ctrl Pts',(39.3714021191617,-5.95819057112127,3.74882613900572));
#28254=CARTESIAN_POINT('Ctrl Pts',(39.4044873865687,-6.40052273738413,2.68695843223506));
#28255=CARTESIAN_POINT('Ctrl Pts',(39.4308410365104,-6.7528568117702,1.84114118420078));
#28256=CARTESIAN_POINT('Ctrl Pts',(39.4571946864522,-6.92380449431593,0.920753703537604));
#28257=CARTESIAN_POINT('Ctrl Pts',(39.4835483363939,-6.92013724019376,-0.000148983254069613));
#28258=CARTESIAN_POINT('Origin',(29.75,0.,0.));
#28259=CARTESIAN_POINT('',(40.9128916636063,-6.92852880502623,-0.00501897357509773));
#28260=CARTESIAN_POINT('',(40.7335483363939,-6.93300654955486,-1.27468492755348E-5));
#28261=CARTESIAN_POINT('',(29.75,-6.933,-8.4904762584886E-16));
#28262=CARTESIAN_POINT('Ctrl Pts',(40.9128916636063,-6.92852880502623,-0.00501897357509773));
#28263=CARTESIAN_POINT('Ctrl Pts',(40.8682637997087,-6.91735475736882,1.55301169949673));
#28264=CARTESIAN_POINT('Ctrl Pts',(40.8236359358112,-6.3969852050255,3.11776396156197));
#28265=CARTESIAN_POINT('Ctrl Pts',(40.7790080719136,-5.43089818827215,4.32823400634588));
#28266=CARTESIAN_POINT('Ctrl Pts',(40.7128375370996,-3.9984636285045,6.12301966813749));
#28267=CARTESIAN_POINT('Ctrl Pts',(40.6466670022855,-1.58614038791887,7.1389326981632));
#28268=CARTESIAN_POINT('Ctrl Pts',(40.5804964674715,0.6950393921076,6.90992361478826));
#28269=CARTESIAN_POINT('Ctrl Pts',(40.5143259326574,2.97621917213404,6.68091453141333));
#28270=CARTESIAN_POINT('Ctrl Pts',(40.4481553978434,5.1262554916013,5.20698333463781));
#28271=CARTESIAN_POINT('Ctrl Pts',(40.3819848630294,6.1797849470107,3.16175504064282));
#28272=CARTESIAN_POINT('Ctrl Pts',(40.3488995956224,6.7065496747154,2.13914089364533));
#28273=CARTESIAN_POINT('Ctrl Pts',(40.3158143282154,6.95918768640563,0.973702472342916));
#28274=CARTESIAN_POINT('Ctrl Pts',(40.2827290608083,6.92707370902873,-0.181309583225821));
#28275=CARTESIAN_POINT('Ctrl Pts',(40.2496437934013,6.89495973165184,-1.33632163879456));
#28276=CARTESIAN_POINT('Ctrl Pts',(40.2165585259943,6.57809376520782,-2.48090732862967));
#28277=CARTESIAN_POINT('Ctrl Pts',(40.1834732585873,6.00218706448473,-3.47549841615815));
#28278=CARTESIAN_POINT('Ctrl Pts',(40.1503879911802,5.42628036376162,-4.47008950368665));
#28279=CARTESIAN_POINT('Ctrl Pts',(40.1173027237732,4.59133292875946,-5.31468598890848));
#28280=CARTESIAN_POINT('Ctrl Pts',(40.0842174563662,3.6055913817208,-5.91751080466672));
#28281=CARTESIAN_POINT('Ctrl Pts',(40.0511321889592,2.61984983468214,-6.52033562042496));
#28282=CARTESIAN_POINT('Ctrl Pts',(40.0180469215522,1.48331417560702,-6.88138876671957));
#28283=CARTESIAN_POINT('Ctrl Pts',(39.9849616541452,0.334186178414354,-6.93359621888145));
#28284=CARTESIAN_POINT('Ctrl Pts',(39.9187911193311,-1.96406981597094,-7.03801112320521));
#28285=CARTESIAN_POINT('Ctrl Pts',(39.8526205845171,-4.3126951628264,-5.90704325099806));
#28286=CARTESIAN_POINT('Ctrl Pts',(39.786450049703,-5.64689858899888,-4.04260565036367));
#28287=CARTESIAN_POINT('Ctrl Pts',(39.7452639210041,-6.47733881704471,-2.88213494861335));
#28288=CARTESIAN_POINT('Ctrl Pts',(39.7040777923052,-6.91478019443497,-1.43750954319842));
#28289=CARTESIAN_POINT('Ctrl Pts',(39.6628916636063,-6.92332261655204,0.00297343908938319));
#28290=CARTESIAN_POINT('Ctrl Pts',(39.4835483363939,-6.933,-5.33212363151847E-12));
#28291=CARTESIAN_POINT('Ctrl Pts',(39.540772531679,-6.93299999999847,-1.99420935702161));
#28292=CARTESIAN_POINT('Ctrl Pts',(39.5979967269641,-6.02307502628944,-3.97063309653508));
#28293=CARTESIAN_POINT('Ctrl Pts',(39.6552209222492,-4.50798484753579,-5.26731066241471));
#28294=CARTESIAN_POINT('Ctrl Pts',(39.7124451175343,-2.99289466878215,-6.56398822829434));
#28295=CARTESIAN_POINT('Ctrl Pts',(39.7696693128194,-0.899664345623291,
-7.15779044292479));
#28296=CARTESIAN_POINT('Ctrl Pts',(39.8268935081045,1.07062371682372,-6.84983604599224));
#28297=CARTESIAN_POINT('Ctrl Pts',(39.8841177033896,3.04091177927072,-6.54188164905968));
#28298=CARTESIAN_POINT('Ctrl Pts',(39.9413418986747,4.85311303640291,-5.33766370386027));
#28299=CARTESIAN_POINT('Ctrl Pts',(39.9985660939598,5.90026971494041,-3.64050907030281));
#28300=CARTESIAN_POINT('Ctrl Pts',(40.0557902892449,6.94742639347791,-1.94335443674534));
#28301=CARTESIAN_POINT('Ctrl Pts',(40.11301448453,7.21086008527493,0.216464293129457));
#28302=CARTESIAN_POINT('Ctrl Pts',(40.1702386798151,6.6023393500592,2.11556236179884));
#28303=CARTESIAN_POINT('Ctrl Pts',(40.2274628751002,5.99381861484346,4.01466043046822));
#28304=CARTESIAN_POINT('Ctrl Pts',(40.2846870703853,4.52419779646866,5.61916312790788));
#28305=CARTESIAN_POINT('Ctrl Pts',(40.3419112656703,2.68569472999914,6.39167683923827));
#28306=CARTESIAN_POINT('Ctrl Pts',(40.3991354609554,0.84719166352962,7.16419055056865));
#28307=CARTESIAN_POINT('Ctrl Pts',(40.4563596562405,-1.32739978994712,7.09093574623685));
#28308=CARTESIAN_POINT('Ctrl Pts',(40.5135838515256,-3.10974706736665,6.1964475449248));
#28309=CARTESIAN_POINT('Ctrl Pts',(40.5708080468107,-4.89209434478617,5.30195934361274));
#28310=CARTESIAN_POINT('Ctrl Pts',(40.6280322420958,-6.2504052505893,3.60219296582193));
#28311=CARTESIAN_POINT('Ctrl Pts',(40.6852564373809,-6.7297428071289,1.66644854402914));
#28312=CARTESIAN_POINT('Ctrl Pts',(40.7013537370519,-6.86458158035659,1.12191912096209));
#28313=CARTESIAN_POINT('Ctrl Pts',(40.7174510367229,-6.93300000000043,0.560975745772757));
#28314=CARTESIAN_POINT('Ctrl Pts',(40.7335483363939,-6.933,-5.33018074122538E-12));
#28315=CARTESIAN_POINT('Origin',(29.75,0.,0.));
#28316=CARTESIAN_POINT('',(42.1628916636063,-6.94425388693856,-0.00173762222092533));
#28317=CARTESIAN_POINT('',(41.983548336394,-6.93579090859155,-0.000199833497099776));
#28318=CARTESIAN_POINT('',(29.75,-6.933,-8.4904762584886E-16));
#28319=CARTESIAN_POINT('Ctrl Pts',(42.1628916636063,-6.94425388693856,-0.00173762222092533));
#28320=CARTESIAN_POINT('Ctrl Pts',(42.0986203419263,-6.93743152686536,2.22904201996126));
#28321=CARTESIAN_POINT('Ctrl Pts',(42.0343490202463,-5.76506820550086,4.46620311375873));
#28322=CARTESIAN_POINT('Ctrl Pts',(41.9700776985663,-3.92913448030361,5.72643225354837));
#28323=CARTESIAN_POINT('Ctrl Pts',(41.9039071637522,-2.03894903983166,7.0239010777201));
#28324=CARTESIAN_POINT('Ctrl Pts',(41.8377366289382,0.55460315267518,7.28584834836761));
#28325=CARTESIAN_POINT('Ctrl Pts',(41.7715660941241,2.67938377070186,6.40369733338716));
#28326=CARTESIAN_POINT('Ctrl Pts',(41.7384808267171,3.7417740797152,5.96262182589693));
#28327=CARTESIAN_POINT('Ctrl Pts',(41.7053955593101,4.68697149510849,5.23552174699971));
#28328=CARTESIAN_POINT('Ctrl Pts',(41.6723102919031,5.4079448361866,4.33259229377163));
#28329=CARTESIAN_POINT('Ctrl Pts',(41.6392250244961,6.1289181772647,3.42966284054355));
#28330=CARTESIAN_POINT('Ctrl Pts',(41.606139757089,6.62566744402761,2.35090401298461));
#28331=CARTESIAN_POINT('Ctrl Pts',(41.573054489682,6.82774670134459,1.2195137473861));
#28332=CARTESIAN_POINT('Ctrl Pts',(41.539969222275,7.02982595866158,0.0881234817875855));
#28333=CARTESIAN_POINT('Ctrl Pts',(41.506883954868,6.93723520653264,-1.09589822185049));
#28334=CARTESIAN_POINT('Ctrl Pts',(41.473798687461,6.57341605062311,-2.19258403731697));
#28335=CARTESIAN_POINT('Ctrl Pts',(41.440713420054,6.20959689471358,-3.28926985278344));
#28336=CARTESIAN_POINT('Ctrl Pts',(41.407628152647,5.57454933502346,-4.29861978007831));
#28337=CARTESIAN_POINT('Ctrl Pts',(41.3745428852399,4.73053937671899,-5.08020020605896));
#28338=CARTESIAN_POINT('Ctrl Pts',(41.3083723504259,3.04251946011003,-6.64336105802027));
#28339=CARTESIAN_POINT('Ctrl Pts',(41.2422018156119,0.518649949043639,-7.29544390472471));
#28340=CARTESIAN_POINT('Ctrl Pts',(41.1760312807978,-1.70381896380896,-6.73254224326552));
#28341=CARTESIAN_POINT('Ctrl Pts',(41.1098607459838,-3.92628787666155,-6.16964058180633));
#28342=CARTESIAN_POINT('Ctrl Pts',(41.0436902111697,-5.84735619130035,-4.3917544121835));
#28343=CARTESIAN_POINT('Ctrl Pts',(40.9775196763557,-6.58161740914491,-2.21598218059335));
#28344=CARTESIAN_POINT('Ctrl Pts',(40.9559770054392,-6.8206656173423,-1.50763147274297));
#28345=CARTESIAN_POINT('Ctrl Pts',(40.9344343345228,-6.93392271839034,-0.75710834412651));
#28346=CARTESIAN_POINT('Ctrl Pts',(40.9128916636063,-6.92852880502623,-0.00501897357509773));
#28347=CARTESIAN_POINT('Ctrl Pts',(40.7335483363939,-6.93403978357422,-0.00202363712922985));
#28348=CARTESIAN_POINT('Ctrl Pts',(40.7537217634838,-6.93745058116421,-0.706445496939072));
#28349=CARTESIAN_POINT('Ctrl Pts',(40.7738951905736,-6.83493540187031,-1.410290980689));
#28350=CARTESIAN_POINT('Ctrl Pts',(40.7940686176635,-6.62303379288307,-2.07890844114385));
#28351=CARTESIAN_POINT('Ctrl Pts',(40.8602391524775,-5.92797872206192,-4.2720298551332));
#28352=CARTESIAN_POINT('Ctrl Pts',(40.9264096872915,-4.05604043060457,-6.08613469797778));
#28353=CARTESIAN_POINT('Ctrl Pts',(40.9925802221056,-1.84572944398094,-6.69502852409246));
#28354=CARTESIAN_POINT('Ctrl Pts',(41.0587507569196,0.364581542642692,-7.30392235020714));
#28355=CARTESIAN_POINT('Ctrl Pts',(41.1249212917337,2.91326522443259,-6.70760515959187));
#28356=CARTESIAN_POINT('Ctrl Pts',(41.1910918265477,4.62679641577792,-5.17890139624333));
#28357=CARTESIAN_POINT('Ctrl Pts',(41.2572623613617,6.34032760712328,-3.65019763289477));
#28358=CARTESIAN_POINT('Ctrl Pts',(41.3234328961758,7.21870630802407,-1.18910729681289));
#28359=CARTESIAN_POINT('Ctrl Pts',(41.3896034309898,6.86030974856457,1.07908058031658));
#28360=CARTESIAN_POINT('Ctrl Pts',(41.4557739658038,6.50191318910508,3.34726845744604));
#28361=CARTESIAN_POINT('Ctrl Pts',(41.5219445006179,4.90674136928536,5.42255387562307));
#28362=CARTESIAN_POINT('Ctrl Pts',(41.5881150354319,2.81038650873806,6.35073631875021));
#28363=CARTESIAN_POINT('Ctrl Pts',(41.6542855702459,0.714031648190772,7.27891876187734));
#28364=CARTESIAN_POINT('Ctrl Pts',(41.72045610506,-1.88350625308409,7.05999822995456));
#28365=CARTESIAN_POINT('Ctrl Pts',(41.786626639874,-3.81008929259621,5.80255603254067));
#28366=CARTESIAN_POINT('Ctrl Pts',(41.8197119072811,-4.77338081235228,5.17383493383372));
#28367=CARTESIAN_POINT('Ctrl Pts',(41.8527971746881,-5.56893361666766,4.28548341875398));
#28368=CARTESIAN_POINT('Ctrl Pts',(41.8858824420951,-6.11177954673742,3.26548221666705));
#28369=CARTESIAN_POINT('Ctrl Pts',(41.9184377401947,-6.64593001492546,2.26181968653242));
#28370=CARTESIAN_POINT('Ctrl Pts',(41.9509930382943,-6.93540463039963,1.13069129491634));
#28371=CARTESIAN_POINT('Ctrl Pts',(41.983548336394,-6.93579090859155,-0.000199833497099776));
#28372=CARTESIAN_POINT('Origin',(29.75,0.,0.));
#28373=CARTESIAN_POINT('',(43.4128916636063,-6.93181729306353,0.00373977463357647));
#28374=CARTESIAN_POINT('',(43.2335483363939,-6.93333665186083,0.000459679647765049));
#28375=CARTESIAN_POINT('',(29.75,-6.933,-8.4904762584886E-16));
#28376=CARTESIAN_POINT('Ctrl Pts',(43.4128916636063,-6.93014855072287,0.00901641594148822));
#28377=CARTESIAN_POINT('Ctrl Pts',(43.3951474189579,-6.93567118806017,0.627760842080671));
#28378=CARTESIAN_POINT('Ctrl Pts',(43.3774031743095,-6.85978677319659,1.24489869731294));
#28379=CARTESIAN_POINT('Ctrl Pts',(43.3596589296611,-6.6972076135722,1.83780692661128));
#28380=CARTESIAN_POINT('Ctrl Pts',(43.293488394847,-6.09092934390644,4.04883677914626));
#28381=CARTESIAN_POINT('Ctrl Pts',(43.227317860033,-4.27904055528442,5.92292011921481));
#28382=CARTESIAN_POINT('Ctrl Pts',(43.1611473252189,-2.08674303097735,6.62056949597221));
#28383=CARTESIAN_POINT('Ctrl Pts',(43.1280620578119,-0.990594268823833,
6.96939418435091));
#28384=CARTESIAN_POINT('Ctrl Pts',(43.0949767904049,0.200656677250987,7.02411038190183));
#28385=CARTESIAN_POINT('Ctrl Pts',(43.0618915229979,1.33413363877489,6.79980225956431));
#28386=CARTESIAN_POINT('Ctrl Pts',(43.0288062555909,2.46761060029882,6.57549413722679));
#28387=CARTESIAN_POINT('Ctrl Pts',(42.9957209881839,3.54331357727186,6.07216169500083));
#28388=CARTESIAN_POINT('Ctrl Pts',(42.9626357207769,4.42791770297886,5.33843456580973));
#28389=CARTESIAN_POINT('Ctrl Pts',(42.9295504533698,5.31252182868585,4.60470743661862));
#28390=CARTESIAN_POINT('Ctrl Pts',(42.8964651859628,6.00602710312679,3.64058562046237));
#28391=CARTESIAN_POINT('Ctrl Pts',(42.8633799185557,6.43599643445051,2.56810693527878));
#28392=CARTESIAN_POINT('Ctrl Pts',(42.8302946511487,6.86596576577423,1.49562825009519));
#28393=CARTESIAN_POINT('Ctrl Pts',(42.7972093837417,7.03239915398073,0.314792695884272));
#28394=CARTESIAN_POINT('Ctrl Pts',(42.7641241163347,6.89221272945286,-0.826946564354824));
#28395=CARTESIAN_POINT('Ctrl Pts',(42.6979535815207,6.61183988039712,-3.11042508483302));
#28396=CARTESIAN_POINT('Ctrl Pts',(42.6317830467066,5.10498778040392,-5.23751842942387));
#28397=CARTESIAN_POINT('Ctrl Pts',(42.5656125118926,3.04413503102753,-6.24206424443556));
#28398=CARTESIAN_POINT('Ctrl Pts',(42.4994419770785,0.983282281651154,-7.24661005944724));
#28399=CARTESIAN_POINT('Ctrl Pts',(42.4332714422645,-1.63157111710844,-7.12860834487975));
#28400=CARTESIAN_POINT('Ctrl Pts',(42.3671009074505,-3.5967532801185,-5.94067593687986));
#28401=CARTESIAN_POINT('Ctrl Pts',(42.3009303726365,-5.5619354431286,-4.75274352887994));
#28402=CARTESIAN_POINT('Ctrl Pts',(42.2347598378224,-6.87744637038917,-2.49488042744759));
#28403=CARTESIAN_POINT('Ctrl Pts',(42.1685893030084,-6.94179248980091,-0.199453687883419));
#28404=CARTESIAN_POINT('Ctrl Pts',(42.1666900898743,-6.94363933893783,-0.13357081986297));
#28405=CARTESIAN_POINT('Ctrl Pts',(42.1647908767403,-6.94445548720937,-0.067657007178727));
#28406=CARTESIAN_POINT('Ctrl Pts',(42.1628916636063,-6.94425388693856,-0.00173762222092533));
#28407=CARTESIAN_POINT('Ctrl Pts',(41.983548336394,-6.93579090859155,-0.000199833497099776));
#28408=CARTESIAN_POINT('Ctrl Pts',(41.9840783057013,-6.93579719683334,-0.0186096660913617));
#28409=CARTESIAN_POINT('Ctrl Pts',(41.9846082750087,-6.93572687451181,-0.0370194358091072));
#28410=CARTESIAN_POINT('Ctrl Pts',(41.9851382443161,-6.93557975002843,-0.0554285917301944));
#28411=CARTESIAN_POINT('Ctrl Pts',(42.0182235117232,-6.92639496742555,-1.20468730894637));
#28412=CARTESIAN_POINT('Ctrl Pts',(42.0513087791302,-6.61788634639566,-2.35155385428462));
#28413=CARTESIAN_POINT('Ctrl Pts',(42.0843940465372,-6.05880726310654,-3.36274856089688));
#28414=CARTESIAN_POINT('Ctrl Pts',(42.1174793139442,-5.49972817981741,-4.37394326750917));
#28415=CARTESIAN_POINT('Ctrl Pts',(42.1505645813512,-4.69007863426907,-5.24946613539546));
#28416=CARTESIAN_POINT('Ctrl Pts',(42.1836498487583,-3.71686142459988,-5.8627108131522));
#28417=CARTESIAN_POINT('Ctrl Pts',(42.2498203835723,-1.77042700526154,-7.08920016866564));
#28418=CARTESIAN_POINT('Ctrl Pts',(42.3159909183863,0.830278070560082,-7.26657676366079));
#28419=CARTESIAN_POINT('Ctrl Pts',(42.3821614532004,2.91153018628898,-6.30500722387515));
#28420=CARTESIAN_POINT('Ctrl Pts',(42.4483319880144,4.99278230201796,-5.34343768408949));
#28421=CARTESIAN_POINT('Ctrl Pts',(42.5145025228284,6.55458145765417,-3.24292200952291));
#28422=CARTESIAN_POINT('Ctrl Pts',(42.5806730576425,6.87668020567494,-0.969295669001434));
#28423=CARTESIAN_POINT('Ctrl Pts',(42.6468435924565,7.1987789536957,1.30433067151996));
#28424=CARTESIAN_POINT('Ctrl Pts',(42.7130141272706,6.28117729410115,3.75106767799625));
#28425=CARTESIAN_POINT('Ctrl Pts',(42.7791846620846,4.54343198507275,5.2521891190326));
#28426=CARTESIAN_POINT('Ctrl Pts',(42.8453551968986,2.80568667604431,6.75331056006899));
#28427=CARTESIAN_POINT('Ctrl Pts',(42.9115257317127,0.247797717581995,7.30881643566538));
#28428=CARTESIAN_POINT('Ctrl Pts',(42.9776962665267,-1.95249909982447,6.66467338914477));
#28429=CARTESIAN_POINT('Ctrl Pts',(43.0438668013407,-4.15279591723087,6.02053034262418));
#28430=CARTESIAN_POINT('Ctrl Pts',(43.1100373361548,-5.99550059358143,4.17673837398668));
#28431=CARTESIAN_POINT('Ctrl Pts',(43.1762078709688,-6.6554146239929,1.9727881566635));
#28432=CARTESIAN_POINT('Ctrl Pts',(43.1953213594438,-6.84603208311179,1.33617282331664));
#28433=CARTESIAN_POINT('Ctrl Pts',(43.2144348479189,-6.93796286882622,0.669507523321825));
#28434=CARTESIAN_POINT('Ctrl Pts',(43.2335483363939,-6.93462080470656,0.00221311993343605));
#28435=CARTESIAN_POINT('Origin',(29.75,0.,0.));
#28436=CARTESIAN_POINT('',(44.6628916636063,-6.9275833124368,-0.00244717393932553));
#28437=CARTESIAN_POINT('',(44.4835483363939,-6.92717195859874,0.000292485364254664));
#28438=CARTESIAN_POINT('',(29.75,-6.933,-8.4904762584886E-16));
#28439=CARTESIAN_POINT('Ctrl Pts',(44.6628916636063,-6.933,-1.39055433834301E-13));
#28440=CARTESIAN_POINT('Ctrl Pts',(44.6056674683212,-6.93300000000004,1.99420935701617));
#28441=CARTESIAN_POINT('Ctrl Pts',(44.5484432730361,-6.02307502629254,3.97063309653039));
#28442=CARTESIAN_POINT('Ctrl Pts',(44.491219077751,-4.50798484753988,5.26731066241122));
#28443=CARTESIAN_POINT('Ctrl Pts',(44.4339948824659,-2.99289466878721,6.56398822829204));
#28444=CARTESIAN_POINT('Ctrl Pts',(44.3767706871808,-0.899664345628768,
7.15779044292411));
#28445=CARTESIAN_POINT('Ctrl Pts',(44.3195464918957,1.0706237168185,6.84983604599305));
#28446=CARTESIAN_POINT('Ctrl Pts',(44.2623222966106,3.04091177926578,6.54188164906199));
#28447=CARTESIAN_POINT('Ctrl Pts',(44.2050981013255,4.85311303639891,5.33766370386393));
#28448=CARTESIAN_POINT('Ctrl Pts',(44.1478739060404,5.90026971493769,3.64050907030721));
#28449=CARTESIAN_POINT('Ctrl Pts',(44.0906497107553,6.94742639347648,1.9433544367505));
#28450=CARTESIAN_POINT('Ctrl Pts',(44.0334255154702,7.2108600852751,-0.216464293124145));
#28451=CARTESIAN_POINT('Ctrl Pts',(43.9762013201851,6.60233935006075,-2.115562361794));
#28452=CARTESIAN_POINT('Ctrl Pts',(43.9189771249,5.99381861484639,-4.01466043046386));
#28453=CARTESIAN_POINT('Ctrl Pts',(43.8617529296149,4.52419779647272,-5.61916312790462));
#28454=CARTESIAN_POINT('Ctrl Pts',(43.8045287343298,2.68569473000373,-6.39167683923634));
#28455=CARTESIAN_POINT('Ctrl Pts',(43.7473045390448,0.847191663534734,-7.16419055056806));
#28456=CARTESIAN_POINT('Ctrl Pts',(43.6900803437597,-1.3273997899421,-7.0909357462378));
#28457=CARTESIAN_POINT('Ctrl Pts',(43.6328561484746,-3.10974706736229,-6.19644754492699));
#28458=CARTESIAN_POINT('Ctrl Pts',(43.5756319531895,-4.89209434478247,-5.30195934361617));
#28459=CARTESIAN_POINT('Ctrl Pts',(43.5184077579044,-6.2504052505868,-3.60219296582628));
#28460=CARTESIAN_POINT('Ctrl Pts',(43.4611835626193,-6.72974280712775,-1.66644854403378));
#28461=CARTESIAN_POINT('Ctrl Pts',(43.4450862629483,-6.86458158035576,-1.12191912096703));
#28462=CARTESIAN_POINT('Ctrl Pts',(43.4289889632773,-6.93299999999999,-0.560975745777965));
#28463=CARTESIAN_POINT('Ctrl Pts',(43.4128916636063,-6.933,-9.18709552877317E-14));
#28464=CARTESIAN_POINT('Ctrl Pts',(43.2335483363939,-6.933,-5.62244695245795E-12));
#28465=CARTESIAN_POINT('Ctrl Pts',(43.290772531679,-6.93299999999838,-1.99420935702193));
#28466=CARTESIAN_POINT('Ctrl Pts',(43.3479967269641,-6.02307502628924,-3.97063309653539));
#28467=CARTESIAN_POINT('Ctrl Pts',(43.4052209222492,-4.5079848475355,-5.26731066241496));
#28468=CARTESIAN_POINT('Ctrl Pts',(43.4624451175343,-2.99289466878176,-6.56398822829453));
#28469=CARTESIAN_POINT('Ctrl Pts',(43.5196693128194,-0.89966434562282,-7.15779044292486));
#28470=CARTESIAN_POINT('Ctrl Pts',(43.5768935081045,1.0706237168242,-6.84983604599216));
#28471=CARTESIAN_POINT('Ctrl Pts',(43.6341177033896,3.04091177927121,-6.54188164905946));
#28472=CARTESIAN_POINT('Ctrl Pts',(43.6913418986747,4.85311303640335,-5.33766370385989));
#28473=CARTESIAN_POINT('Ctrl Pts',(43.7485660939598,5.90026971494072,-3.64050907030231));
#28474=CARTESIAN_POINT('Ctrl Pts',(43.8057902892449,6.94742639347808,-1.94335443674474));
#28475=CARTESIAN_POINT('Ctrl Pts',(43.86301448453,7.21086008527492,0.216464293130101));
#28476=CARTESIAN_POINT('Ctrl Pts',(43.9202386798151,6.60233935005901,2.11556236179944));
#28477=CARTESIAN_POINT('Ctrl Pts',(43.9774628751002,5.99381861484309,4.0146604304688));
#28478=CARTESIAN_POINT('Ctrl Pts',(44.0346870703853,4.52419779646809,5.61916312790834));
#28479=CARTESIAN_POINT('Ctrl Pts',(44.0919112656704,2.68569472999846,6.39167683923855));
#28480=CARTESIAN_POINT('Ctrl Pts',(44.1491354609555,0.847191663528831,7.16419055056876));
#28481=CARTESIAN_POINT('Ctrl Pts',(44.2063596562406,-1.32739978994794,7.09093574623671));
#28482=CARTESIAN_POINT('Ctrl Pts',(44.2635838515257,-3.10974706736739,6.19644754492442));
#28483=CARTESIAN_POINT('Ctrl Pts',(44.3208080468107,-4.89209434478684,5.30195934361214));
#28484=CARTESIAN_POINT('Ctrl Pts',(44.3780322420958,-6.25040525058977,3.60219296582113));
#28485=CARTESIAN_POINT('Ctrl Pts',(44.4352564373809,-6.72974280712912,1.66644854402824));
#28486=CARTESIAN_POINT('Ctrl Pts',(44.4513537370519,-6.86458158035669,1.12191912096138));
#28487=CARTESIAN_POINT('Ctrl Pts',(44.4674510367229,-6.93300000000046,0.560975745772253));
#28488=CARTESIAN_POINT('Ctrl Pts',(44.4835483363939,-6.933,-5.62078161792101E-12));
#28489=CARTESIAN_POINT('Origin',(29.75,0.,0.));
#28490=CARTESIAN_POINT('',(45.9128916636063,-6.93405647677003,-0.000332869569125593));
#28491=CARTESIAN_POINT('',(45.7335483363939,-6.94075830301621,-0.00694975155396205));
#28492=CARTESIAN_POINT('',(29.75,-6.933,-8.4904762584886E-16));
#28493=CARTESIAN_POINT('Ctrl Pts',(45.9128916636063,-6.94022992359918,-0.00227796920823947));
#28494=CARTESIAN_POINT('Ctrl Pts',(45.8889457708,-6.93676910672981,0.831764088413885));
#28495=CARTESIAN_POINT('Ctrl Pts',(45.8649998779937,-6.7789353365392,1.66778218659105));
#28496=CARTESIAN_POINT('Ctrl Pts',(45.8410539851874,-6.48203451786819,2.44958197340933));
#28497=CARTESIAN_POINT('Ctrl Pts',(45.8079687177804,-6.07181623707313,3.52976951182737));
#28498=CARTESIAN_POINT('Ctrl Pts',(45.7748834503734,-5.39611816499337,4.50645398362649));
#28499=CARTESIAN_POINT('Ctrl Pts',(45.7417981829664,-4.52512595472309,5.25628898479498));
#28500=CARTESIAN_POINT('Ctrl Pts',(45.7087129155594,-3.65413374445282,6.00612398596347));
#28501=CARTESIAN_POINT('Ctrl Pts',(45.6756276481523,-2.58784739599202,6.52910951650133));
#28502=CARTESIAN_POINT('Ctrl Pts',(45.6425423807453,-1.45867703652056,6.77417778320101));
#28503=CARTESIAN_POINT('Ctrl Pts',(45.6094571133383,-0.329506677049107,
7.01924604990069));
#28504=CARTESIAN_POINT('Ctrl Pts',(45.5763718459313,0.862547693433012,6.9863970527622));
#28505=CARTESIAN_POINT('Ctrl Pts',(45.5432865785243,1.9649124195632,6.65774407076276));
#28506=CARTESIAN_POINT('Ctrl Pts',(45.4771160437103,4.16964187182359,6.00043810676387));
#28507=CARTESIAN_POINT('Ctrl Pts',(45.4109455088962,6.01561274667627,4.15991620332117));
#28508=CARTESIAN_POINT('Ctrl Pts',(45.3447749740822,6.66235862434885,1.96038304403867));
#28509=CARTESIAN_POINT('Ctrl Pts',(45.2786044392681,7.30910450202143,-0.239150115243826));
#28510=CARTESIAN_POINT('Ctrl Pts',(45.2124339044541,6.75662538251391,-2.79769453036612));
#28511=CARTESIAN_POINT('Ctrl Pts',(45.1462633696401,5.25756100615865,-4.53721467550155));
#28512=CARTESIAN_POINT('Ctrl Pts',(45.080092834826,3.75849662980338,-6.27673482063697));
#28513=CARTESIAN_POINT('Ctrl Pts',(45.013922300012,1.31284699660037,-7.19723069578553));
#28514=CARTESIAN_POINT('Ctrl Pts',(44.947751765198,-0.961158843812644,-6.87782221506396));
#28515=CARTESIAN_POINT('Ctrl Pts',(44.8815812303839,-3.23516468422572,-6.55841373434238));
#28516=CARTESIAN_POINT('Ctrl Pts',(44.8154106955699,-5.3375267318488,-4.9991008977506));
#28517=CARTESIAN_POINT('Ctrl Pts',(44.7492401607558,-6.30155803282916,-2.91898792009768));
#28518=CARTESIAN_POINT('Ctrl Pts',(44.7204573283726,-6.72089197695158,-2.01418122113218));
#28519=CARTESIAN_POINT('Ctrl Pts',(44.6916744959895,-6.92484549387806,-1.01083536103422));
#28520=CARTESIAN_POINT('Ctrl Pts',(44.6628916636063,-6.92069769006582,-0.0055579894376756));
#28521=CARTESIAN_POINT('Ctrl Pts',(44.4835483363939,-6.91974231982792,0.000665348317145921));
#28522=CARTESIAN_POINT('Ctrl Pts',(44.5109619249504,-6.92284490954652,-0.957366321970913));
#28523=CARTESIAN_POINT('Ctrl Pts',(44.538375513507,-6.73728033370965,-1.91504791652457));
#28524=CARTESIAN_POINT('Ctrl Pts',(44.5657891020636,-6.35676001150659,-2.78891360290006));
#28525=CARTESIAN_POINT('Ctrl Pts',(44.5988743694706,-5.89751270836997,-3.84357595955975));
#28526=CARTESIAN_POINT('Ctrl Pts',(44.6319596368777,-5.15429468801847,-4.77615284809136));
#28527=CARTESIAN_POINT('Ctrl Pts',(44.6650449042847,-4.23912218741068,-5.48152044742052));
#28528=CARTESIAN_POINT('Ctrl Pts',(44.6981301716917,-3.32394968680288,-6.18688804674967));
#28529=CARTESIAN_POINT('Ctrl Pts',(44.7312154390987,-2.23682270593883,-6.66504635687637));
#28530=CARTESIAN_POINT('Ctrl Pts',(44.7643007065057,-1.10213028992486,-6.84767461418953));
#28531=CARTESIAN_POINT('Ctrl Pts',(44.7973859739127,0.0325621260890784,
-7.03030287150269));
#28532=CARTESIAN_POINT('Ctrl Pts',(44.8304712413197,1.214819977253,-6.91740107600231));
#28533=CARTESIAN_POINT('Ctrl Pts',(44.8635565087267,2.30509895463997,-6.53481003125602));
#28534=CARTESIAN_POINT('Ctrl Pts',(44.8966417761338,3.39537793202696,-6.15221898650973));
#28535=CARTESIAN_POINT('Ctrl Pts',(44.9297270435408,4.39367803563707,-5.49993869251753));
#28536=CARTESIAN_POINT('Ctrl Pts',(44.9628123109478,5.16065519039781,-4.64263663602381));
#28537=CARTESIAN_POINT('Ctrl Pts',(45.0289828457619,6.69460949991927,-2.92803252303641));
#28538=CARTESIAN_POINT('Ctrl Pts',(45.0951533805759,7.30327201404325,-0.393341360043043));
#28539=CARTESIAN_POINT('Ctrl Pts',(45.1613239153899,6.70230282379522,1.81913742662187));
#28540=CARTESIAN_POINT('Ctrl Pts',(45.2274944502039,6.10133363354718,4.03161621328681));
#28541=CARTESIAN_POINT('Ctrl Pts',(45.293664985018,4.2907327389271,5.92188262362324));
#28542=CARTESIAN_POINT('Ctrl Pts',(45.3598355198321,2.10267690769521,6.61868677056951));
#28543=CARTESIAN_POINT('Ctrl Pts',(45.4260060546461,-0.0853789235366806,
7.31549091751577));
#28544=CARTESIAN_POINT('Ctrl Pts',(45.4921765894601,-2.65088969138045,6.81883280107182));
#28545=CARTESIAN_POINT('Ctrl Pts',(45.5583471242741,-4.42082201083547,5.35580035975756));
#28546=CARTESIAN_POINT('Ctrl Pts',(45.616747528314,-5.98291853718214,4.06456573491428));
#28547=CARTESIAN_POINT('Ctrl Pts',(45.675147932354,-6.92530945898835,2.02058625327023));
#28548=CARTESIAN_POINT('Ctrl Pts',(45.7335483363939,-6.94075830301621,-0.00694975155396205));
#28549=CARTESIAN_POINT('Origin',(29.75,0.,0.));
#28550=CARTESIAN_POINT('',(47.1628916636063,-6.933,-3.32511795875234E-13));
#28551=CARTESIAN_POINT('',(46.9835483363939,-6.93618751727322,0.00576443580885351));
#28552=CARTESIAN_POINT('',(29.75,-6.933,-8.4904762584886E-16));
#28553=CARTESIAN_POINT('Ctrl Pts',(47.1628916636063,-6.933,-1.35447209004269E-13));
#28554=CARTESIAN_POINT('Ctrl Pts',(47.1056674683212,-6.93300000000004,1.99420935701617));
#28555=CARTESIAN_POINT('Ctrl Pts',(47.0484432730361,-6.02307502629254,3.97063309653039));
#28556=CARTESIAN_POINT('Ctrl Pts',(46.991219077751,-4.50798484753988,5.26731066241122));
#28557=CARTESIAN_POINT('Ctrl Pts',(46.9339948824659,-2.99289466878721,6.56398822829204));
#28558=CARTESIAN_POINT('Ctrl Pts',(46.8767706871808,-0.899664345628765,
7.15779044292411));
#28559=CARTESIAN_POINT('Ctrl Pts',(46.8195464918957,1.07062371681851,6.84983604599305));
#28560=CARTESIAN_POINT('Ctrl Pts',(46.7623222966106,3.04091177926578,6.54188164906199));
#28561=CARTESIAN_POINT('Ctrl Pts',(46.7050981013255,4.85311303639891,5.33766370386392));
#28562=CARTESIAN_POINT('Ctrl Pts',(46.6478739060404,5.90026971493769,3.64050907030721));
#28563=CARTESIAN_POINT('Ctrl Pts',(46.5906497107553,6.94742639347648,1.94335443675049));
#28564=CARTESIAN_POINT('Ctrl Pts',(46.5334255154702,7.2108600852751,-0.216464293124149));
#28565=CARTESIAN_POINT('Ctrl Pts',(46.4762013201851,6.60233935006075,-2.11556236179401));
#28566=CARTESIAN_POINT('Ctrl Pts',(46.4189771249,5.99381861484639,-4.01466043046386));
#28567=CARTESIAN_POINT('Ctrl Pts',(46.3617529296149,4.52419779647272,-5.61916312790462));
#28568=CARTESIAN_POINT('Ctrl Pts',(46.3045287343298,2.68569473000372,-6.39167683923634));
#28569=CARTESIAN_POINT('Ctrl Pts',(46.2473045390448,0.847191663534731,-7.16419055056806));
#28570=CARTESIAN_POINT('Ctrl Pts',(46.1900803437597,-1.32739978994211,-7.0909357462378));
#28571=CARTESIAN_POINT('Ctrl Pts',(46.1328561484746,-3.10974706736229,-6.19644754492698));
#28572=CARTESIAN_POINT('Ctrl Pts',(46.0756319531895,-4.89209434478247,-5.30195934361617));
#28573=CARTESIAN_POINT('Ctrl Pts',(46.0184077579044,-6.25040525058681,-3.60219296582627));
#28574=CARTESIAN_POINT('Ctrl Pts',(45.9611835626193,-6.72974280712775,-1.66644854403378));
#28575=CARTESIAN_POINT('Ctrl Pts',(45.9450862629483,-6.86458158035576,-1.12191912096703));
#28576=CARTESIAN_POINT('Ctrl Pts',(45.9289889632773,-6.93299999999999,-0.560975745777962));
#28577=CARTESIAN_POINT('Ctrl Pts',(45.9128916636063,-6.933,-8.82627304576999E-14));
#28578=CARTESIAN_POINT('Ctrl Pts',(45.7335483363939,-6.94075830301621,-0.00694975155396205));
#28579=CARTESIAN_POINT('Ctrl Pts',(45.741318467168,-6.94281376034358,-0.276711924704654));
#28580=CARTESIAN_POINT('Ctrl Pts',(45.7490885979422,-6.92846039015388,-0.546183013675027));
#28581=CARTESIAN_POINT('Ctrl Pts',(45.7568587287163,-6.89697457304899,-0.813551385903551));
#28582=CARTESIAN_POINT('Ctrl Pts',(45.8230292635303,-6.62884094474111,-3.09046392406575));
#28583=CARTESIAN_POINT('Ctrl Pts',(45.8891997983443,-5.11821981705906,-5.21488223420553));
#28584=CARTESIAN_POINT('Ctrl Pts',(45.9553703331584,-3.05520819225478,-6.23314846849565));
#28585=CARTESIAN_POINT('Ctrl Pts',(45.9884556005654,-2.02370237985268,-6.74228158564068));
#28586=CARTESIAN_POINT('Ctrl Pts',(46.0215408679724,-0.854098943170027,
-6.97487668382332));
#28587=CARTESIAN_POINT('Ctrl Pts',(46.0546261353794,0.300191666840078,-6.92294072619767));
#28588=CARTESIAN_POINT('Ctrl Pts',(46.0877114027864,1.45448227685025,-6.87100476857203));
#28589=CARTESIAN_POINT('Ctrl Pts',(46.1207966701934,2.59346006018791,-6.53453775513806));
#28590=CARTESIAN_POINT('Ctrl Pts',(46.1538819376005,3.57801869911607,-5.94164295347351));
#28591=CARTESIAN_POINT('Ctrl Pts',(46.1869672050075,4.56257733804423,-5.34874815180897));
#28592=CARTESIAN_POINT('Ctrl Pts',(46.2200524724145,5.39271683256293,-4.49942556191382));
#28593=CARTESIAN_POINT('Ctrl Pts',(46.2531377398216,5.9785317786885,-3.50348128388014));
#28594=CARTESIAN_POINT('Ctrl Pts',(46.2862230072286,6.56434672481405,-2.50753700584648));
#28595=CARTESIAN_POINT('Ctrl Pts',(46.3193082746355,6.9058371225465,-1.36497103967435));
#28596=CARTESIAN_POINT('Ctrl Pts',(46.3523935420426,6.93831117486302,-0.215116175824418));
#28597=CARTESIAN_POINT('Ctrl Pts',(46.4185640768566,7.00325927949605,2.08459355187545));
#28598=CARTESIAN_POINT('Ctrl Pts',(46.4847346116707,5.83214200246525,4.41345887028628));
#28599=CARTESIAN_POINT('Ctrl Pts',(46.5509051464847,3.94507643800014,5.7154611377496));
#28600=CARTESIAN_POINT('Ctrl Pts',(46.6170756812988,2.05801087353504,7.01746340521292));
#28601=CARTESIAN_POINT('Ctrl Pts',(46.6832462161128,-0.545002978364427,
7.29260262172879));
#28602=CARTESIAN_POINT('Ctrl Pts',(46.7494167509268,-2.66599822587748,6.41254381697971));
#28603=CARTESIAN_POINT('Ctrl Pts',(46.8155872857408,-4.78699347339055,5.53248501223062));
#28604=CARTESIAN_POINT('Ctrl Pts',(46.8817578205549,-6.42597011651721,3.49722818621661));
#28605=CARTESIAN_POINT('Ctrl Pts',(46.9479283553689,-6.83353573651531,1.23735770205496));
#28606=CARTESIAN_POINT('Ctrl Pts',(46.9598016823773,-6.90666737882698,0.831857257932137));
#28607=CARTESIAN_POINT('Ctrl Pts',(46.9716750093856,-6.94015126573288,0.419124925177673));
#28608=CARTESIAN_POINT('Ctrl Pts',(46.9835483363939,-6.93618751727322,0.00576443580885351));
#28609=CARTESIAN_POINT('Origin',(29.75,0.,0.));
#28610=CARTESIAN_POINT('',(48.4128916636063,-6.933,-3.80251385934116E-13));
#28611=CARTESIAN_POINT('',(48.2335483363939,-6.92348246561576,0.00082620762749036));
#28612=CARTESIAN_POINT('',(29.75,-6.933,-8.4904762584886E-16));
#28613=CARTESIAN_POINT('Ctrl Pts',(48.4128916636063,-6.930055142889,-0.000658831376577074));
#28614=CARTESIAN_POINT('Ctrl Pts',(48.3827441226422,-6.93264111678612,1.05251277108305));
#28615=CARTESIAN_POINT('Ctrl Pts',(48.352596581678,-6.69957236130202,2.10736732158826));
#28616=CARTESIAN_POINT('Ctrl Pts',(48.3224490407138,-6.23675887648899,3.04783130190406));
#28617=CARTESIAN_POINT('Ctrl Pts',(48.2562785058998,-5.2209342078818,5.11204624483563));
#28618=CARTESIAN_POINT('Ctrl Pts',(48.1901079710858,-3.0983046766226,6.6251798215178));
#28619=CARTESIAN_POINT('Ctrl Pts',(48.1239374362717,-0.821710974525657,
6.89600719207382));
#28620=CARTESIAN_POINT('Ctrl Pts',(48.0577669014577,1.45488272757128,7.16683456262985));
#28621=CARTESIAN_POINT('Ctrl Pts',(47.9915963666437,3.88544060050593,6.19535572705974));
#28622=CARTESIAN_POINT('Ctrl Pts',(47.9254258318296,5.35056611389629,4.42715563380048));
#28623=CARTESIAN_POINT('Ctrl Pts',(47.8592552970156,6.81569162728666,2.6589555405412));
#28624=CARTESIAN_POINT('Ctrl Pts',(47.7930847622015,7.3153847811327,0.0940341895926755));
#28625=CARTESIAN_POINT('Ctrl Pts',(47.7269142273875,6.62116992097035,-2.09484453425644));
#28626=CARTESIAN_POINT('Ctrl Pts',(47.6607436925735,5.92695506080801,-4.28372325810549));
#28627=CARTESIAN_POINT('Ctrl Pts',(47.5945731577595,4.03883218663742,-6.09655935485521));
#28628=CARTESIAN_POINT('Ctrl Pts',(47.5284026229454,1.8270659854587,-6.7001458195751));
#28629=CARTESIAN_POINT('Ctrl Pts',(47.4622320881314,-0.384700215720024,
-7.30373228429499));
#28630=CARTESIAN_POINT('Ctrl Pts',(47.3960615533173,-2.92010974390683,-6.69806911698503));
#28631=CARTESIAN_POINT('Ctrl Pts',(47.3298910185033,-4.63652755541892,-5.1661445156104));
#28632=CARTESIAN_POINT('Ctrl Pts',(47.2968057510963,-5.494736461175,-4.40018221492305));
#28633=CARTESIAN_POINT('Ctrl Pts',(47.2637204836893,-6.14819743776237,-3.40265455571952));
#28634=CARTESIAN_POINT('Ctrl Pts',(47.2306352162822,-6.53207817870433,-2.3128290041811));
#28635=CARTESIAN_POINT('Ctrl Pts',(47.2080540320569,-6.79408246070457,-1.56900695039511));
#28636=CARTESIAN_POINT('Ctrl Pts',(47.1854728478316,-6.93050914286102,-0.782190098558359));
#28637=CARTESIAN_POINT('Ctrl Pts',(47.1628916636063,-6.93309008421871,0.00326550207437409));
#28638=CARTESIAN_POINT('Ctrl Pts',(46.9835483363939,-6.93618751727322,0.00576443580885351));
#28639=CARTESIAN_POINT('Ctrl Pts',(47.0378455441996,-6.9180611341918,-1.88454991114452));
#28640=CARTESIAN_POINT('Ctrl Pts',(47.0921427520053,-6.11680353603182,-3.78800070978208));
#28641=CARTESIAN_POINT('Ctrl Pts',(47.146439959811,-4.74282239922126,-5.07304246071674));
#28642=CARTESIAN_POINT('Ctrl Pts',(47.2126104946251,-3.06838884505966,-6.63908799701747));
#28643=CARTESIAN_POINT('Ctrl Pts',(47.2787810294391,-0.543367139866965,
-7.28669492730971));
#28644=CARTESIAN_POINT('Ctrl Pts',(47.3449515642531,1.68960656755196,-6.73287951586954));
#28645=CARTESIAN_POINT('Ctrl Pts',(47.3780368316602,2.80609342126142,-6.45597181014945));
#28646=CARTESIAN_POINT('Ctrl Pts',(47.4111220990672,3.84956827552745,-5.87870851899626));
#28647=CARTESIAN_POINT('Ctrl Pts',(47.4442073664742,4.69769668825529,-5.09400325485192));
#28648=CARTESIAN_POINT('Ctrl Pts',(47.4772926338812,5.54582510098315,-4.30929799070757));
#28649=CARTESIAN_POINT('Ctrl Pts',(47.5103779012883,6.19860707217283,-3.31715075357204));
#28650=CARTESIAN_POINT('Ctrl Pts',(47.5434631686953,6.5679320432874,-2.22881301874882));
#28651=CARTESIAN_POINT('Ctrl Pts',(47.5765484361023,6.93725701440196,-1.14047528392563));
#28652=CARTESIAN_POINT('Ctrl Pts',(47.6096337035093,7.02312498544144,0.0440529485851764));
#28653=CARTESIAN_POINT('Ctrl Pts',(47.6427189709163,6.82774025790008,1.1828720581437));
#28654=CARTESIAN_POINT('Ctrl Pts',(47.6758042383233,6.63235553035873,2.32169116770218));
#28655=CARTESIAN_POINT('Ctrl Pts',(47.7088895057303,6.15571810423654,3.41480115430832));
#28656=CARTESIAN_POINT('Ctrl Pts',(47.7419747731374,5.43834849684116,4.31402394003972));
#28657=CARTESIAN_POINT('Ctrl Pts',(47.8081453079514,4.00360928205037,6.11246951150258));
#28658=CARTESIAN_POINT('Ctrl Pts',(47.8743158427655,1.60594134216666,7.13536627946652));
#28659=CARTESIAN_POINT('Ctrl Pts',(47.9404863775795,-0.675781576911461,
6.91183357576677));
#28660=CARTESIAN_POINT('Ctrl Pts',(48.0066569123935,-2.95750449598962,6.68830087206702));
#28661=CARTESIAN_POINT('Ctrl Pts',(48.0728274472075,-5.12328239426221,5.21833869670365));
#28662=CARTESIAN_POINT('Ctrl Pts',(48.1389979820216,-6.17527098918003,3.17715170479127));
#28663=CARTESIAN_POINT('Ctrl Pts',(48.1705147668124,-6.67632932642266,2.20494177294425));
#28664=CARTESIAN_POINT('Ctrl Pts',(48.2020315516031,-6.92471540330101,1.10314479520007));
#28665=CARTESIAN_POINT('Ctrl Pts',(48.2335483363939,-6.92348246561576,0.00082620762749036));
#28666=CARTESIAN_POINT('Origin',(29.75,0.,0.));
#28667=CARTESIAN_POINT('',(49.6628916636063,-6.93186465004489,-0.000678253275532354));
#28668=CARTESIAN_POINT('',(49.4835483363939,-6.93271820397492,-0.00595368521987888));
#28669=CARTESIAN_POINT('',(29.75,-6.933,-8.4904762584886E-16));
#28670=CARTESIAN_POINT('Ctrl Pts',(49.6628916636063,-6.933,-4.27990975992998E-13));
#28671=CARTESIAN_POINT('Ctrl Pts',(49.6056674683212,-6.93300000000012,1.99420935701588));
#28672=CARTESIAN_POINT('Ctrl Pts',(49.5484432730361,-6.02307502629271,3.97063309653014));
#28673=CARTESIAN_POINT('Ctrl Pts',(49.491219077751,-4.5079848475401,5.26731066241103));
#28674=CARTESIAN_POINT('Ctrl Pts',(49.4339948824659,-2.99289466878749,6.56398822829192));
#28675=CARTESIAN_POINT('Ctrl Pts',(49.3767706871808,-0.899664345629066,
7.15779044292407));
#28676=CARTESIAN_POINT('Ctrl Pts',(49.3195464918957,1.07062371681822,6.8498360459931));
#28677=CARTESIAN_POINT('Ctrl Pts',(49.2623222966106,3.0409117792655,6.54188164906212));
#28678=CARTESIAN_POINT('Ctrl Pts',(49.2050981013255,4.85311303639869,5.33766370386413));
#28679=CARTESIAN_POINT('Ctrl Pts',(49.1478739060404,5.90026971493754,3.64050907030746));
#28680=CARTESIAN_POINT('Ctrl Pts',(49.0906497107553,6.9474263934764,1.94335443675079));
#28681=CARTESIAN_POINT('Ctrl Pts',(49.0334255154702,7.21086008527511,-0.216464293123844));
#28682=CARTESIAN_POINT('Ctrl Pts',(48.9762013201851,6.60233935006084,-2.11556236179373));
#28683=CARTESIAN_POINT('Ctrl Pts',(48.9189771249,5.99381861484656,-4.01466043046361));
#28684=CARTESIAN_POINT('Ctrl Pts',(48.8617529296149,4.52419779647296,-5.61916312790443));
#28685=CARTESIAN_POINT('Ctrl Pts',(48.8045287343298,2.68569473000399,-6.39167683923622));
#28686=CARTESIAN_POINT('Ctrl Pts',(48.7473045390448,0.847191663535033,-7.16419055056802));
#28687=CARTESIAN_POINT('Ctrl Pts',(48.6900803437597,-1.32739978994181,-7.09093574623786));
#28688=CARTESIAN_POINT('Ctrl Pts',(48.6328561484746,-3.10974706736203,-6.19644754492712));
#28689=CARTESIAN_POINT('Ctrl Pts',(48.5756319531895,-4.89209434478225,-5.30195934361637));
#28690=CARTESIAN_POINT('Ctrl Pts',(48.5184077579044,-6.25040525058665,-3.60219296582654));
#28691=CARTESIAN_POINT('Ctrl Pts',(48.4611835626193,-6.72974280712768,-1.66644854403406));
#28692=CARTESIAN_POINT('Ctrl Pts',(48.4450862629483,-6.86458158035571,-1.12191912096732));
#28693=CARTESIAN_POINT('Ctrl Pts',(48.4289889632773,-6.93299999999997,-0.560975745778254));
#28694=CARTESIAN_POINT('Ctrl Pts',(48.4128916636063,-6.933,-3.80251385934116E-13));
#28695=CARTESIAN_POINT('Ctrl Pts',(48.2335483363939,-6.92348246561576,0.00082620762749036));
#28696=CARTESIAN_POINT('Ctrl Pts',(48.2682020864172,-6.92212680974468,-1.21120963401434));
#28697=CARTESIAN_POINT('Ctrl Pts',(48.3028558364405,-6.61898846170223,-2.42387608794565));
#28698=CARTESIAN_POINT('Ctrl Pts',(48.3375095864637,-6.01812611974246,-3.46560568327387));
#28699=CARTESIAN_POINT('Ctrl Pts',(48.4036801212778,-4.87079336382414,-5.4547642709652));
#28700=CARTESIAN_POINT('Ctrl Pts',(48.4698506560917,-2.63792856042451,-6.82066963788656));
#28701=CARTESIAN_POINT('Ctrl Pts',(48.5360211909058,-0.348187949984992,
-6.93605718476102));
#28702=CARTESIAN_POINT('Ctrl Pts',(48.6021917257198,1.94155266045456,-7.05144473163549));
#28703=CARTESIAN_POINT('Ctrl Pts',(48.6683622605339,4.288169077934,-5.91631445846307));
#28704=CARTESIAN_POINT('Ctrl Pts',(48.734532795348,5.63626081271754,-4.05203664585539));
#28705=CARTESIAN_POINT('Ctrl Pts',(48.767618062755,6.31030668010929,-3.11989773955158));
#28706=CARTESIAN_POINT('Ctrl Pts',(48.800703330162,6.73472137682705,-2.00547194838899));
#28707=CARTESIAN_POINT('Ctrl Pts',(48.833788597569,6.87603656298273,-0.858687673028613));
#28708=CARTESIAN_POINT('Ctrl Pts',(48.866873864976,7.0173517491384,0.288096602331795));
#28709=CARTESIAN_POINT('Ctrl Pts',(48.899959132383,6.87556742473195,1.46723936189003));
#28710=CARTESIAN_POINT('Ctrl Pts',(48.93304439979,6.4551917161997,2.53689548560685));
#28711=CARTESIAN_POINT('Ctrl Pts',(48.9661296671971,6.03481600766747,3.60655160932363));
#28712=CARTESIAN_POINT('Ctrl Pts',(48.9992149346041,5.33584891500949,4.56672109719906));
#28713=CARTESIAN_POINT('Ctrl Pts',(49.0323002020111,4.45156314573267,5.31044338025002));
#28714=CARTESIAN_POINT('Ctrl Pts',(49.0653854694181,3.5672773764558,6.05416566330103));
#28715=CARTESIAN_POINT('Ctrl Pts',(49.0984707368251,2.49767293056012,6.58144074152752));
#28716=CARTESIAN_POINT('Ctrl Pts',(49.1315560042321,1.36934097820534,6.80524372919427));
#28717=CARTESIAN_POINT('Ctrl Pts',(49.1977265390462,-0.887322926504155,
7.25284970452777));
#28718=CARTESIAN_POINT('Ctrl Pts',(49.2638970738602,-3.37889685704989,6.48656731762235));
#28719=CARTESIAN_POINT('Ctrl Pts',(49.3300676086743,-4.97740422569037,4.84309521823281));
#28720=CARTESIAN_POINT('Ctrl Pts',(49.3812278512475,-6.2133021214013,3.57243250554062));
#28721=CARTESIAN_POINT('Ctrl Pts',(49.4323880938207,-6.91534942433851,1.77740994335895));
#28722=CARTESIAN_POINT('Ctrl Pts',(49.4835483363939,-6.93271820397492,-0.00595368521987888));
#28723=CARTESIAN_POINT('Origin',(29.75,0.,0.));
#28724=CARTESIAN_POINT('',(50.9128916636063,-6.94407271247953,0.00085298068625117));
#28725=CARTESIAN_POINT('',(50.7335483363939,-6.94318480280473,0.00509973895979926));
#28726=CARTESIAN_POINT('',(29.75,-6.933,-8.4904762584886E-16));
#28727=CARTESIAN_POINT('Ctrl Pts',(50.9128916636063,-6.94407271247953,0.00085298068625117));
#28728=CARTESIAN_POINT('Ctrl Pts',(50.9096277418913,-6.94453748549343,0.113946146647875));
#28729=CARTESIAN_POINT('Ctrl Pts',(50.9063638201763,-6.9420222511174,0.227031117887721));
#28730=CARTESIAN_POINT('Ctrl Pts',(50.9030998984613,-6.93646428876074,0.339981307628455));
#28731=CARTESIAN_POINT('Ctrl Pts',(50.8369293636473,-6.82378593010814,2.62985683624597));
#28732=CARTESIAN_POINT('Ctrl Pts',(50.7707588288332,-5.46052333404185,4.86433614825873));
#28733=CARTESIAN_POINT('Ctrl Pts',(50.7045882940192,-3.47272360578677,6.0140215748597));
#28734=CARTESIAN_POINT('Ctrl Pts',(50.6384177592051,-1.48492387753177,7.16370700146062));
#28735=CARTESIAN_POINT('Ctrl Pts',(50.5722472243911,1.12741298291193,7.22859854264998));
#28736=CARTESIAN_POINT('Ctrl Pts',(50.5060766895771,3.16984320685072,6.17902571519562));
#28737=CARTESIAN_POINT('Ctrl Pts',(50.439906154763,5.21227343078961,5.12945288774122));
#28738=CARTESIAN_POINT('Ctrl Pts',(50.373735619949,6.68479701822344,2.96541569164298));
#28739=CARTESIAN_POINT('Ctrl Pts',(50.307565085135,6.9110291867925,0.683958842396304));
#28740=CARTESIAN_POINT('Ctrl Pts',(50.2413945503209,7.13726135536154,-1.59749800685027));
#28741=CARTESIAN_POINT('Ctrl Pts',(50.1752240155069,6.11720210506592,-3.99637450924526));
#28742=CARTESIAN_POINT('Ctrl Pts',(50.1090534806928,4.32045530461438,-5.43324055137998));
#28743=CARTESIAN_POINT('Ctrl Pts',(50.0759682132858,3.42208190438857,-6.15167357244737));
#28744=CARTESIAN_POINT('Ctrl Pts',(50.0428829458788,2.32953661662386,-6.62960397844963));
#28745=CARTESIAN_POINT('Ctrl Pts',(50.0097976784718,1.19094947366404,-6.82633596349212));
#28746=CARTESIAN_POINT('Ctrl Pts',(49.9767124110648,0.0523623307042911,
-7.0230679485346));
#28747=CARTESIAN_POINT('Ctrl Pts',(49.9436271436578,-1.13226666745058,-6.93860151261728));
#28748=CARTESIAN_POINT('Ctrl Pts',(49.9105418762507,-2.22104060749918,-6.57056446719955));
#28749=CARTESIAN_POINT('Ctrl Pts',(49.8774566088437,-3.30981454754782,-6.20252742178181));
#28750=CARTESIAN_POINT('Ctrl Pts',(49.8443713414367,-4.30273342949029,-5.55091976686365));
#28751=CARTESIAN_POINT('Ctrl Pts',(49.8112860740297,-5.08844160785031,-4.7037203720868));
#28752=CARTESIAN_POINT('Ctrl Pts',(49.7782008066227,-5.87414978621033,-3.85652097730995));
#28753=CARTESIAN_POINT('Ctrl Pts',(49.7451155392157,-6.45264726098789,-2.81372984267439));
#28754=CARTESIAN_POINT('Ctrl Pts',(49.7120302718086,-6.73087574473247,-1.69757139387494));
#28755=CARTESIAN_POINT('Ctrl Pts',(49.6956507357412,-6.868618427251,-1.14499440109481));
#28756=CARTESIAN_POINT('Ctrl Pts',(49.6792711996737,-6.9327667757156,-0.574435469491616));
#28757=CARTESIAN_POINT('Ctrl Pts',(49.6628916636063,-6.92759240687057,-0.00323047333067872));
#28758=CARTESIAN_POINT('Ctrl Pts',(49.4835483363939,-6.93271820397492,-0.00595368521987888));
#28759=CARTESIAN_POINT('Ctrl Pts',(49.4985586286347,-6.93781416218575,-0.529188288697132));
#28760=CARTESIAN_POINT('Ctrl Pts',(49.5135689208755,-6.88397152104115,-1.05141926610295));
#28761=CARTESIAN_POINT('Ctrl Pts',(49.5285792131163,-6.76738092568683,-1.55910876840476));
#28762=CARTESIAN_POINT('Ctrl Pts',(49.5947497479304,-6.25340945030763,-3.79717884377907));
#28763=CARTESIAN_POINT('Ctrl Pts',(49.6609202827444,-4.52002569281411,-5.75265718265399));
#28764=CARTESIAN_POINT('Ctrl Pts',(49.7270908175585,-2.35978801703893,-6.53143669185472));
#28765=CARTESIAN_POINT('Ctrl Pts',(49.7932613523725,-0.199550341263754,
-7.31021620105544));
#28766=CARTESIAN_POINT('Ctrl Pts',(49.8594318871866,2.38754125279309,-6.91229688058191));
#28767=CARTESIAN_POINT('Ctrl Pts',(49.9256024220006,4.21092850274789,-5.52251801839842));
#28768=CARTESIAN_POINT('Ctrl Pts',(49.9917729568146,6.03431575270265,-4.13273915621496));
#28769=CARTESIAN_POINT('Ctrl Pts',(50.0579434916286,7.09399865855549,-1.75110075232157));
#28770=CARTESIAN_POINT('Ctrl Pts',(50.1241140264427,6.92037756701128,0.542965245975702));
#28771=CARTESIAN_POINT('Ctrl Pts',(50.1571992938497,6.83356702123917,1.68999824512437));
#28772=CARTESIAN_POINT('Ctrl Pts',(50.1902845612568,6.4384304761178,2.815138142874));
#28773=CARTESIAN_POINT('Ctrl Pts',(50.2233698286638,5.80617594701643,3.78226707248107));
#28774=CARTESIAN_POINT('Ctrl Pts',(50.2564550960708,5.17392141791508,4.74939600208811));
#28775=CARTESIAN_POINT('Ctrl Pts',(50.2895403634778,4.30454890483377,5.55851396355256));
#28776=CARTESIAN_POINT('Ctrl Pts',(50.3226256308848,3.29305560594214,6.10418901853135));
#28777=CARTESIAN_POINT('Ctrl Pts',(50.3557108982918,2.28156230705047,6.64986407351015));
#28778=CARTESIAN_POINT('Ctrl Pts',(50.3887961656989,1.1279482223485,6.93209622200326));
#28779=CARTESIAN_POINT('Ctrl Pts',(50.4218814331059,-0.0275070301753554,
6.92939150997962));
#28780=CARTESIAN_POINT('Ctrl Pts',(50.4549667005129,-1.18296228269921,6.92668679795597));
#28781=CARTESIAN_POINT('Ctrl Pts',(50.4880519679199,-2.34025870304492,6.63904522541559));
#28782=CARTESIAN_POINT('Ctrl Pts',(50.521137235327,-3.34653541563076,6.08170515893852));
#28783=CARTESIAN_POINT('Ctrl Pts',(50.587307770141,-5.35908884080245,4.96702502598438));
#28784=CARTESIAN_POINT('Ctrl Pts',(50.653478304955,-6.76756343493463,2.77355091728346));
#28785=CARTESIAN_POINT('Ctrl Pts',(50.719648839769,-6.92772948095231,0.486506276972989));
#28786=CARTESIAN_POINT('Ctrl Pts',(50.7242820053106,-6.93894407680581,0.326370705310355));
#28787=CARTESIAN_POINT('Ctrl Pts',(50.7289151708523,-6.94403871679269,0.165776394880989));
#28788=CARTESIAN_POINT('Ctrl Pts',(50.7335483363939,-6.94318480280473,0.00509973895979926));
#28789=CARTESIAN_POINT('Origin',(29.75,0.,0.));
#28790=CARTESIAN_POINT('',(52.1628916636063,-6.92485909669474,0.00398171681318865));
#28791=CARTESIAN_POINT('',(51.9835483363939,-6.92875907966107,0.000287925818791141));
#28792=CARTESIAN_POINT('',(29.75,-6.933,-8.4904762584886E-16));
#28793=CARTESIAN_POINT('Ctrl Pts',(52.1628916636063,-6.92485909669474,0.00398171681318865));
#28794=CARTESIAN_POINT('Ctrl Pts',(52.1399842841088,-6.93057837326804,0.804739728972275));
#28795=CARTESIAN_POINT('Ctrl Pts',(52.1170769046114,-6.80294244975768,1.60389401713382));
#28796=CARTESIAN_POINT('Ctrl Pts',(52.0941695251139,-6.53422410442902,2.35205869360553));
#28797=CARTESIAN_POINT('Ctrl Pts',(52.0279989902999,-5.7580010263276,4.51321627064897));
#28798=CARTESIAN_POINT('Ctrl Pts',(51.9618284554859,-3.80457490977705,6.24891243983584));
#28799=CARTESIAN_POINT('Ctrl Pts',(51.8956579206719,-1.56711450642194,6.76553152892132));
#28800=CARTESIAN_POINT('Ctrl Pts',(51.8294873858578,0.67034589693314,7.28215061800679));
#28801=CARTESIAN_POINT('Ctrl Pts',(51.7633168510438,3.19184058709277,6.5796926269909));
#28802=CARTESIAN_POINT('Ctrl Pts',(51.6971463162297,4.83720281076991,4.98313085181089));
#28803=CARTESIAN_POINT('Ctrl Pts',(51.6309757814157,6.48256503444705,3.38656907663088));
#28804=CARTESIAN_POINT('Ctrl Pts',(51.5648052466017,7.25179479164169,0.895903517286758));
#28805=CARTESIAN_POINT('Ctrl Pts',(51.4986347117877,6.80685910234047,-1.36128839310964));
#28806=CARTESIAN_POINT('Ctrl Pts',(51.4655494443806,6.58439125768985,-2.48988434830787));
#28807=CARTESIAN_POINT('Ctrl Pts',(51.4324641769736,6.05838205141525,-3.56011189126916));
#28808=CARTESIAN_POINT('Ctrl Pts',(51.3993789095666,5.31570653195091,-4.44527697691168));
#28809=CARTESIAN_POINT('Ctrl Pts',(51.3662936421595,4.57303101248661,-5.33044206255415));
#28810=CARTESIAN_POINT('Ctrl Pts',(51.3332083747525,3.6136891798326,-6.03054469087787));
#28811=CARTESIAN_POINT('Ctrl Pts',(51.3001231073455,2.54453117246911,-6.45218566922238));
#28812=CARTESIAN_POINT('Ctrl Pts',(51.2670378399385,1.47537316510556,-6.87382664756691));
#28813=CARTESIAN_POINT('Ctrl Pts',(51.2339525725315,0.296398983032527,-7.01700597593221));
#28814=CARTESIAN_POINT('Ctrl Pts',(51.2008673051245,-0.850551686782959,
-6.87704770693045));
#28815=CARTESIAN_POINT('Ctrl Pts',(51.1677820377175,-1.99750235659838,-6.73708943792869));
#28816=CARTESIAN_POINT('Ctrl Pts',(51.1346967703104,-3.11242951415625,-6.31399357155991));
#28817=CARTESIAN_POINT('Ctrl Pts',(51.1016115029034,-4.04536526565498,-5.64105103644369));
#28818=CARTESIAN_POINT('Ctrl Pts',(51.0387048898043,-5.81920096248678,-4.36155296941387));
#28819=CARTESIAN_POINT('Ctrl Pts',(50.9757982767053,-6.93511499268184,-2.17882798488593));
#28820=CARTESIAN_POINT('Ctrl Pts',(50.9128916636063,-6.94407271247953,0.00085298068625117));
#28821=CARTESIAN_POINT('Ctrl Pts',(50.7335483363939,-6.94318480280473,0.00509973895979926));
#28822=CARTESIAN_POINT('Ctrl Pts',(50.7950857056663,-6.93184317904203,-2.12899597163449));
#28823=CARTESIAN_POINT('Ctrl Pts',(50.8566230749388,-5.87111952376545,-4.27761821756149));
#28824=CARTESIAN_POINT('Ctrl Pts',(50.9181604442112,-4.16261867540694,-5.55885514366222));
#28825=CARTESIAN_POINT('Ctrl Pts',(50.9843309790252,-2.32548432594074,-6.93655675206683));
#28826=CARTESIAN_POINT('Ctrl Pts',(51.0505015138392,0.260641870894862,-7.31134479695605));
#28827=CARTESIAN_POINT('Ctrl Pts',(51.1166720486532,2.41330049815419,-6.51185422523226));
#28828=CARTESIAN_POINT('Ctrl Pts',(51.1828425834673,4.56595912541357,-5.71236365350845));
#28829=CARTESIAN_POINT('Ctrl Pts',(51.2490131182814,6.28515018309664,-3.73859446517156));
#28830=CARTESIAN_POINT('Ctrl Pts',(51.3151836530954,6.78082632587978,-1.50017280906083));
#28831=CARTESIAN_POINT('Ctrl Pts',(51.3813541879094,7.27650246866292,0.738248847049866));
#28832=CARTESIAN_POINT('Ctrl Pts',(51.4475247227234,6.54866369654615,3.24132297093438));
#28833=CARTESIAN_POINT('Ctrl Pts',(51.5136952575375,4.93534739297613,4.88147344958201));
#28834=CARTESIAN_POINT('Ctrl Pts',(51.5467805249445,4.12868924119113,5.70154868890581));
#28835=CARTESIAN_POINT('Ctrl Pts',(51.5798657923515,3.10066170654277,6.30589301692042));
#28836=CARTESIAN_POINT('Ctrl Pts',(51.6129510597585,1.99351089896141,6.63650040541012));
#28837=CARTESIAN_POINT('Ctrl Pts',(51.6460363271656,0.886360091380012,6.96710779389984));
#28838=CARTESIAN_POINT('Ctrl Pts',(51.6791215945726,-0.299913989134387,
7.02397824286466));
#28839=CARTESIAN_POINT('Ctrl Pts',(51.7122068619796,-1.42470120777253,6.78789844254885));
#28840=CARTESIAN_POINT('Ctrl Pts',(51.7452921293866,-2.54948842641068,6.55181864223305));
#28841=CARTESIAN_POINT('Ctrl Pts',(51.7783773967936,-3.61278878317257,6.02278859263659));
#28842=CARTESIAN_POINT('Ctrl Pts',(51.8114626642007,-4.49358304177177,5.27493457608602));
#28843=CARTESIAN_POINT('Ctrl Pts',(51.8445479316077,-5.37437730037094,4.52708055953547));
#28844=CARTESIAN_POINT('Ctrl Pts',(51.8776331990147,-6.07266546080745,3.56040257603086));
#28845=CARTESIAN_POINT('Ctrl Pts',(51.9107184664217,-6.48152754865665,2.48520372692769));
#28846=CARTESIAN_POINT('Ctrl Pts',(51.9349950897458,-6.78153391632782,1.69626655023685));
#28847=CARTESIAN_POINT('Ctrl Pts',(51.9592717130699,-6.92571249345945,0.848901442148907));
#28848=CARTESIAN_POINT('Ctrl Pts',(51.9835483363939,-6.92116679875715,0.000803383211501455));
#28849=CARTESIAN_POINT('Origin',(29.75,0.,0.));
#28850=CARTESIAN_POINT('',(53.4128916636063,-6.92692581532746,-0.0043983532947317));
#28851=CARTESIAN_POINT('',(53.2335483363939,-6.933,-5.95370974743048E-12));
#28852=CARTESIAN_POINT('',(29.75,-6.933,-8.4904762584886E-16));
#28853=CARTESIAN_POINT('Ctrl Pts',(53.4128916636063,-6.92692581532746,-0.0043983532947317));
#28854=CARTESIAN_POINT('Ctrl Pts',(53.3703408263264,-6.91775456656079,1.48198715944652));
#28855=CARTESIAN_POINT('Ctrl Pts',(53.3277899890465,-6.44830631727461,2.97362567138676));
#28856=CARTESIAN_POINT('Ctrl Pts',(53.2852391517666,-5.56377625673586,4.15603880035411));
#28857=CARTESIAN_POINT('Ctrl Pts',(53.2190686169526,-4.18824921880831,5.99480189214149));
#28858=CARTESIAN_POINT('Ctrl Pts',(53.1528980821386,-1.80892314934302,7.0857602583535));
#28859=CARTESIAN_POINT('Ctrl Pts',(53.0867275473245,0.478309390730293,6.92830024216106));
#28860=CARTESIAN_POINT('Ctrl Pts',(53.0205570125105,2.76554193080364,6.77084022596862));
#28861=CARTESIAN_POINT('Ctrl Pts',(52.9543864776965,4.96068094148503,5.36496182737171));
#28862=CARTESIAN_POINT('Ctrl Pts',(52.8882159428824,6.07774144758688,3.3537286450479));
#28863=CARTESIAN_POINT('Ctrl Pts',(52.8551306754754,6.6362717006378,2.34811205388602));
#28864=CARTESIAN_POINT('Ctrl Pts',(52.8220454080684,6.92528232754384,1.19115676679243));
#28865=CARTESIAN_POINT('Ctrl Pts',(52.7889601406614,6.92935411498852,0.0357055230789582));
#28866=CARTESIAN_POINT('Ctrl Pts',(52.7558748732543,6.9334259024332,-1.11974572063455));
#28867=CARTESIAN_POINT('Ctrl Pts',(52.7227896058473,6.65255885041648,-2.27369292096794));
#28868=CARTESIAN_POINT('Ctrl Pts',(52.6897043384403,6.10808092604286,-3.28583112753789));
#28869=CARTESIAN_POINT('Ctrl Pts',(52.6566190710333,5.56360300166923,-4.29796933410788));
#28870=CARTESIAN_POINT('Ctrl Pts',(52.6235338036263,4.75551420493866,-5.16829854691442));
#28871=CARTESIAN_POINT('Ctrl Pts',(52.5904485362193,3.78913400442954,-5.80169689244124));
#28872=CARTESIAN_POINT('Ctrl Pts',(52.5573632688123,2.82275380392046,-6.43509523796805));
#28873=CARTESIAN_POINT('Ctrl Pts',(52.5242780014052,1.69808219963283,-6.83156271621516));
#28874=CARTESIAN_POINT('Ctrl Pts',(52.4911927339982,0.551152713248234,-6.91973031374846));
#28875=CARTESIAN_POINT('Ctrl Pts',(52.4250221991841,-1.74270625952099,-7.09606550881507));
#28876=CARTESIAN_POINT('Ctrl Pts',(52.3588516643701,-4.12559676067808,-6.0392011810264));
#28877=CARTESIAN_POINT('Ctrl Pts',(52.2926811295561,-5.51753199143044,-4.21745952468206));
#28878=CARTESIAN_POINT('Ctrl Pts',(52.2494179742395,-6.42759732863707,-3.02638116258884));
#28879=CARTESIAN_POINT('Ctrl Pts',(52.2061548189229,-6.91405760145096,-1.50833959671446));
#28880=CARTESIAN_POINT('Ctrl Pts',(52.1628916636063,-6.92485909669474,0.00398171681318865));
#28881=CARTESIAN_POINT('Ctrl Pts',(51.9835483363939,-6.933,-5.90610893524968E-12));
#28882=CARTESIAN_POINT('Ctrl Pts',(52.040772531679,-6.9329999999983,-1.99420935702222));
#28883=CARTESIAN_POINT('Ctrl Pts',(52.0979967269641,-6.02307502628908,-3.97063309653564));
#28884=CARTESIAN_POINT('Ctrl Pts',(52.1552209222492,-4.50798484753529,-5.26731066241515));
#28885=CARTESIAN_POINT('Ctrl Pts',(52.2124451175343,-2.99289466878149,-6.56398822829465));
#28886=CARTESIAN_POINT('Ctrl Pts',(52.2696693128194,-0.899664345622527,
-7.1577904429249));
#28887=CARTESIAN_POINT('Ctrl Pts',(52.3268935081045,1.07062371682448,-6.84983604599212));
#28888=CARTESIAN_POINT('Ctrl Pts',(52.3841177033896,3.04091177927148,-6.54188164905934));
#28889=CARTESIAN_POINT('Ctrl Pts',(52.4413418986747,4.85311303640357,-5.33766370385969));
#28890=CARTESIAN_POINT('Ctrl Pts',(52.4985660939598,5.90026971494087,-3.64050907030207));
#28891=CARTESIAN_POINT('Ctrl Pts',(52.5557902892449,6.94742639347817,-1.94335443674444));
#28892=CARTESIAN_POINT('Ctrl Pts',(52.61301448453,7.21086008527491,0.216464293130433));
#28893=CARTESIAN_POINT('Ctrl Pts',(52.6702386798151,6.6023393500589,2.11556236179976));
#28894=CARTESIAN_POINT('Ctrl Pts',(52.7274628751002,5.99381861484289,4.01466043046909));
#28895=CARTESIAN_POINT('Ctrl Pts',(52.7846870703853,4.52419779646782,5.61916312790856));
#28896=CARTESIAN_POINT('Ctrl Pts',(52.8419112656704,2.68569472999816,6.39167683923868));
#28897=CARTESIAN_POINT('Ctrl Pts',(52.8991354609555,0.847191663528488,7.1641905505688));
#28898=CARTESIAN_POINT('Ctrl Pts',(52.9563596562406,-1.32739978994829,7.09093574623664));
#28899=CARTESIAN_POINT('Ctrl Pts',(53.0135838515257,-3.10974706736769,6.19644754492427));
#28900=CARTESIAN_POINT('Ctrl Pts',(53.0708080468108,-4.89209434478709,5.3019593436119));
#28901=CARTESIAN_POINT('Ctrl Pts',(53.1280322420959,-6.25040525058995,3.60219296582083));
#28902=CARTESIAN_POINT('Ctrl Pts',(53.1852564373809,-6.7297428071292,1.66644854402792));
#28903=CARTESIAN_POINT('Ctrl Pts',(53.2013537370519,-6.86458158035674,1.12191912096105));
#28904=CARTESIAN_POINT('Ctrl Pts',(53.2174510367229,-6.93300000000048,0.56097574577192));
#28905=CARTESIAN_POINT('Ctrl Pts',(53.2335483363939,-6.933,-5.95370974743048E-12));
#28906=CARTESIAN_POINT('Origin',(29.75,0.,0.));
#28907=CARTESIAN_POINT('',(54.6628916636063,-6.94327184494755,-0.00291245565295251));
#28908=CARTESIAN_POINT('',(54.483548336394,-6.93556957250402,-0.00097039555626976));
#28909=CARTESIAN_POINT('',(29.75,-6.933,-8.4904762584886E-16));
#28910=CARTESIAN_POINT('Ctrl Pts',(54.6628916636063,-6.94327184494755,-0.00291245565295251));
#28911=CARTESIAN_POINT('Ctrl Pts',(54.600697368544,-6.93190021454453,2.15659674677899));
#28912=CARTESIAN_POINT('Ctrl Pts',(54.5385030734816,-5.84407642554417,4.32603973215319));
#28913=CARTESIAN_POINT('Ctrl Pts',(54.4763087784193,-4.10653465994407,5.60058007758731));
#28914=CARTESIAN_POINT('Ctrl Pts',(54.4101382436052,-2.25790742208785,6.95660503477874));
#28915=CARTESIAN_POINT('Ctrl Pts',(54.3439677087913,0.32616968197601,7.29964274132155));
#28916=CARTESIAN_POINT('Ctrl Pts',(54.2777971739772,2.47753336573461,6.48446338180748));
#28917=CARTESIAN_POINT('Ctrl Pts',(54.2447119065702,3.55321520761379,6.07687370205049));
#28918=CARTESIAN_POINT('Ctrl Pts',(54.2116266391631,4.5207186944167,5.37972975577934));
#28919=CARTESIAN_POINT('Ctrl Pts',(54.1785413717561,5.26961429958365,4.49982093742742));
#28920=CARTESIAN_POINT('Ctrl Pts',(54.1454561043491,6.01850990475068,3.6199121190754));
#28921=CARTESIAN_POINT('Ctrl Pts',(54.1123708369421,6.54879762828172,2.55723842864254));
#28922=CARTESIAN_POINT('Ctrl Pts',(54.0792855695351,6.78620805577826,1.43273131517245));
#28923=CARTESIAN_POINT('Ctrl Pts',(54.0462003021281,7.02361848327481,0.308224201702331));
#28924=CARTESIAN_POINT('Ctrl Pts',(54.013115034721,6.96815161473686,-0.878116334804946));
#28925=CARTESIAN_POINT('Ctrl Pts',(53.980029767314,6.63885438353871,-1.98565752572177));
#28926=CARTESIAN_POINT('Ctrl Pts',(53.946944499907,6.3095571523406,-3.0931987166385));
#28927=CARTESIAN_POINT('Ctrl Pts',(53.9138592325,5.70642955848233,-4.12194056196472));
#28928=CARTESIAN_POINT('Ctrl Pts',(53.880773965093,4.8873092910417,-4.92956842147746));
#28929=CARTESIAN_POINT('Ctrl Pts',(53.814603430279,3.24906875616034,-6.54482414050303));
#28930=CARTESIAN_POINT('Ctrl Pts',(53.7484328954649,0.746857526949387,-7.27562391627462));
#28931=CARTESIAN_POINT('Ctrl Pts',(53.6822623606508,-1.49214902185302,-6.78259650984583));
#28932=CARTESIAN_POINT('Ctrl Pts',(53.6160918258368,-3.73115557065537,-6.28956910341706));
#28933=CARTESIAN_POINT('Ctrl Pts',(53.5499212910228,-5.70695743904921,-4.57271451478797));
#28934=CARTESIAN_POINT('Ctrl Pts',(53.4837507562088,-6.50899437005123,-2.42100331179203));
#28935=CARTESIAN_POINT('Ctrl Pts',(53.4601310586746,-6.79528296927026,-1.65294592887326));
#28936=CARTESIAN_POINT('Ctrl Pts',(53.4365113611405,-6.93201671684027,-0.829481441534794));
#28937=CARTESIAN_POINT('Ctrl Pts',(53.4128916636063,-6.92692581532746,-0.0043983532947317));
#28938=CARTESIAN_POINT('Ctrl Pts',(53.2335483363939,-6.9329724241112,-0.00157606328284038));
#28939=CARTESIAN_POINT('Ctrl Pts',(53.2557987901015,-6.93641591712985,-0.778738933088749));
#28940=CARTESIAN_POINT('Ctrl Pts',(53.278049243809,-6.81138105671096,-1.55551720174311));
#28941=CARTESIAN_POINT('Ctrl Pts',(53.3002996975165,-6.55468300132901,-2.28529378426906));
#28942=CARTESIAN_POINT('Ctrl Pts',(53.3664702323305,-5.79128968658476,-4.45557342868741));
#28943=CARTESIAN_POINT('Ctrl Pts',(53.4326407671446,-3.863459532006,-6.21016746804625));
#28944=CARTESIAN_POINT('Ctrl Pts',(53.4988113019586,-1.63516466953287,-6.74954521596095));
#28945=CARTESIAN_POINT('Ctrl Pts',(53.5649818367726,0.593130192940265,-7.28892296387565));
#28946=CARTESIAN_POINT('Ctrl Pts',(53.6311523715867,3.1218897633078,-6.6130844203462));
#28947=CARTESIAN_POINT('Ctrl Pts',(53.6973229064007,4.78670810869231,-5.03146998671818));
#28948=CARTESIAN_POINT('Ctrl Pts',(53.7634934412148,6.45152645407682,-3.44985555309015));
#28949=CARTESIAN_POINT('Ctrl Pts',(53.8296639760288,7.25240357447835,-0.962465229363512));
#28950=CARTESIAN_POINT('Ctrl Pts',(53.8958345108428,6.82315289555494,1.29338675922819));
#28951=CARTESIAN_POINT('Ctrl Pts',(53.9620050456569,6.39390221663153,3.5492387478199));
#28952=CARTESIAN_POINT('Ctrl Pts',(54.0281755804709,4.73452373838319,5.57355240127669));
#28953=CARTESIAN_POINT('Ctrl Pts',(54.094346115285,2.61013036397045,6.43563078508));
#28954=CARTESIAN_POINT('Ctrl Pts',(54.160516650099,0.485736989557669,7.29770916888332));
#28955=CARTESIAN_POINT('Ctrl Pts',(54.226687184913,-2.10367128101945,6.99755228303315));
#28956=CARTESIAN_POINT('Ctrl Pts',(54.2928577197271,-3.98993172841131,5.6803945048691));
#28957=CARTESIAN_POINT('Ctrl Pts',(54.3259429871341,-4.93306195210724,5.02181561578707));
#28958=CARTESIAN_POINT('Ctrl Pts',(54.3590282545411,-5.70040522000687,4.10898650362653));
#28959=CARTESIAN_POINT('Ctrl Pts',(54.3921135219481,-6.21104285301366,3.07248596633321));
#28960=CARTESIAN_POINT('Ctrl Pts',(54.4225917934301,-6.68144414118274,2.11765781342223));
#28961=CARTESIAN_POINT('Ctrl Pts',(54.453070064912,-6.93400084389427,1.05788007359531));
#28962=CARTESIAN_POINT('Ctrl Pts',(54.483548336394,-6.93556957250402,-0.00097039555626976));
#28963=CARTESIAN_POINT('Origin',(29.75,0.,0.));
#28964=CARTESIAN_POINT('',(55.9128916636063,-6.93279366535694,0.00322938497813596));
#28965=CARTESIAN_POINT('',(55.7335483363939,-6.93303840625552,3.40981942736484E-5));
#28966=CARTESIAN_POINT('',(29.75,-6.933,-8.4904762584886E-16));
#28967=CARTESIAN_POINT('Ctrl Pts',(55.9128916636063,-6.93241833981259,0.00910368052880667));
#28968=CARTESIAN_POINT('Ctrl Pts',(55.8972244455755,-6.9374986604769,0.554924718265877));
#28969=CARTESIAN_POINT('Ctrl Pts',(55.8815572275448,-6.87855946148903,1.09943300383134));
#28970=CARTESIAN_POINT('Ctrl Pts',(55.8658900095141,-6.75147513749155,1.6271777980981));
#28971=CARTESIAN_POINT('Ctrl Pts',(55.7997194747001,-6.21473417499926,3.85610926592132));
#28972=CARTESIAN_POINT('Ctrl Pts',(55.7335489398861,-4.46242227668877,5.78601401976182));
#28973=CARTESIAN_POINT('Ctrl Pts',(55.667378405072,-2.29304736038406,6.55197456736258));
#28974=CARTESIAN_POINT('Ctrl Pts',(55.634293137665,-1.20835990223168,6.93495484116297));
#28975=CARTESIAN_POINT('Ctrl Pts',(55.6012078702579,-0.0194066895807528,
7.02694906340341));
#28976=CARTESIAN_POINT('Ctrl Pts',(55.5681226028509,1.12053871685304,6.83824658222559));
#28977=CARTESIAN_POINT('Ctrl Pts',(55.5350373354439,2.26048412328677,6.64954410104778));
#28978=CARTESIAN_POINT('Ctrl Pts',(55.5019520680369,3.35142172350335,6.18014491645175));
#28979=CARTESIAN_POINT('Ctrl Pts',(55.4688668006299,4.25856916975443,5.47447964871574));
#28980=CARTESIAN_POINT('Ctrl Pts',(55.4357815332229,5.16571661600551,4.76881438097973));
#28981=CARTESIAN_POINT('Ctrl Pts',(55.4026962658158,5.88907390829107,3.82688303010377));
#28982=CARTESIAN_POINT('Ctrl Pts',(55.3696109984088,6.35241778199036,2.76839514129382));
#28983=CARTESIAN_POINT('Ctrl Pts',(55.3365257310018,6.81576165568967,1.70990725248383));
#28984=CARTESIAN_POINT('Ctrl Pts',(55.3034404635948,7.0190921108027,0.534862825739778));
#28985=CARTESIAN_POINT('Ctrl Pts',(55.2703551961878,6.91472880905904,-0.610706497017424));
#28986=CARTESIAN_POINT('Ctrl Pts',(55.2041846613738,6.70600220557173,-2.90184514253183));
#28987=CARTESIAN_POINT('Ctrl Pts',(55.1380141265597,5.26650057465781,-5.07508337209913));
#28988=CARTESIAN_POINT('Ctrl Pts',(55.0718435917456,3.23811664294813,-6.14367355296912));
#28989=CARTESIAN_POINT('Ctrl Pts',(55.0056730569316,1.20973271123846,-7.21226373383911));
#28990=CARTESIAN_POINT('Ctrl Pts',(54.9395025221176,-1.40753352126693,-7.17620586601176));
#28991=CARTESIAN_POINT('Ctrl Pts',(54.8733319873035,-3.40895278540716,-6.05039714828136));
#28992=CARTESIAN_POINT('Ctrl Pts',(54.8071614524895,-5.4103720495474,-4.92458843055096));
#28993=CARTESIAN_POINT('Ctrl Pts',(54.7409909176755,-6.79594434532244,-2.70902886291751));
#28994=CARTESIAN_POINT('Ctrl Pts',(54.6748203828614,-6.93214180738565,-0.416742975180784));
#28995=CARTESIAN_POINT('Ctrl Pts',(54.6708441431097,-6.94032602055938,-0.278997703894782));
#28996=CARTESIAN_POINT('Ctrl Pts',(54.666867903358,-6.94399886225364,-0.140975381300478));
#28997=CARTESIAN_POINT('Ctrl Pts',(54.6628916636063,-6.94327184494755,-0.00291245565295251));
#28998=CARTESIAN_POINT('Ctrl Pts',(54.483548336394,-6.93556957250402,-0.00097039555626976));
#28999=CARTESIAN_POINT('Ctrl Pts',(54.486155332319,-6.93570375560872,-0.0915404549499743));
#29000=CARTESIAN_POINT('Ctrl Pts',(54.4887623282441,-6.93400159931765,-0.182103730019941));
#29001=CARTESIAN_POINT('Ctrl Pts',(54.4913693241692,-6.93044236180577,-0.272593960816664));
#29002=CARTESIAN_POINT('Ctrl Pts',(54.5244545915762,-6.88527223947709,-1.42100138824727));
#29003=CARTESIAN_POINT('Ctrl Pts',(54.5575398589832,-6.54099999670573,-2.55764428068227));
#29004=CARTESIAN_POINT('Ctrl Pts',(54.5906251263902,-5.95052884467048,-3.55083508544557));
#29005=CARTESIAN_POINT('Ctrl Pts',(54.6237103937972,-5.36005769263525,-4.54402589020884));
#29006=CARTESIAN_POINT('Ctrl Pts',(54.6567956612043,-4.52338763133613,-5.39376460730039));
#29007=CARTESIAN_POINT('Ctrl Pts',(54.6898809286113,-3.53144355466652,-5.97623153404674));
#29008=CARTESIAN_POINT('Ctrl Pts',(54.7560514634254,-1.54755540132733,-7.14116538753941));
#29009=CARTESIAN_POINT('Ctrl Pts',(54.8222219982394,1.05742881349393,-7.23701207965144));
#29010=CARTESIAN_POINT('Ctrl Pts',(54.8883925330534,3.10754793880998,-6.21073827550217));
#29011=CARTESIAN_POINT('Ctrl Pts',(54.9545630678674,5.15766706412604,-5.1844644713529));
#29012=CARTESIAN_POINT('Ctrl Pts',(55.0207336026815,6.65292109993693,-3.03607017094233));
#29013=CARTESIAN_POINT('Ctrl Pts',(55.0869041374955,6.90366166557409,-0.753472197462701));
#29014=CARTESIAN_POINT('Ctrl Pts',(55.1530746723096,7.15440223121126,1.52912577601692));
#29015=CARTESIAN_POINT('Ctrl Pts',(55.2192452071236,6.16062932667472,3.94592742256563));
#29016=CARTESIAN_POINT('Ctrl Pts',(55.2854157419376,4.37672763385377,5.39189391254384));
#29017=CARTESIAN_POINT('Ctrl Pts',(55.3515862767517,2.59282594103279,6.83786040252208));
#29018=CARTESIAN_POINT('Ctrl Pts',(55.4177568115657,0.0187954599274759,
7.31299173592979));
#29019=CARTESIAN_POINT('Ctrl Pts',(55.4839273463797,-2.16025041450548,6.60026077253155));
#29020=CARTESIAN_POINT('Ctrl Pts',(55.5500978811938,-4.3392962889384,5.88752980913332));
#29021=CARTESIAN_POINT('Ctrl Pts',(55.6162684160078,-6.1233575566989,3.98693654892914));
#29022=CARTESIAN_POINT('Ctrl Pts',(55.6824389508218,-6.71392967766051,1.76340160251706));
#29023=CARTESIAN_POINT('Ctrl Pts',(55.6994754126792,-6.86598012490355,1.19092371021159));
#29024=CARTESIAN_POINT('Ctrl Pts',(55.7165118745365,-6.93891754636801,0.597038925338642));
#29025=CARTESIAN_POINT('Ctrl Pts',(55.7335483363939,-6.93581065002168,0.00249537752124046));
#29026=CARTESIAN_POINT('Origin',(29.75,0.,0.));
#29027=CARTESIAN_POINT('',(57.1628916636063,-6.933,-6.1478599988618E-13));
#29028=CARTESIAN_POINT('',(56.9835483363939,-6.92793287508387,0.000631348358467133));
#29029=CARTESIAN_POINT('',(29.75,-6.933,-8.4904762584886E-16));
#29030=CARTESIAN_POINT('Ctrl Pts',(57.1628916636063,-6.933,-6.1478599988618E-13));
#29031=CARTESIAN_POINT('Ctrl Pts',(57.1056674683212,-6.93300000000018,1.99420935701573));
#29032=CARTESIAN_POINT('Ctrl Pts',(57.0484432730361,-6.02307502629278,3.97063309653004));
#29033=CARTESIAN_POINT('Ctrl Pts',(56.991219077751,-4.50798484754016,5.26731066241097));
#29034=CARTESIAN_POINT('Ctrl Pts',(56.9339948824659,-2.99289466878755,6.5639882282919));
#29035=CARTESIAN_POINT('Ctrl Pts',(56.8767706871808,-0.899664345629088,
7.15779044292408));
#29036=CARTESIAN_POINT('Ctrl Pts',(56.8195464918957,1.07062371681823,6.8498360459931));
#29037=CARTESIAN_POINT('Ctrl Pts',(56.7623222966106,3.04091177926555,6.54188164906211));
#29038=CARTESIAN_POINT('Ctrl Pts',(56.7050981013255,4.85311303639876,5.33766370386408));
#29039=CARTESIAN_POINT('Ctrl Pts',(56.6478739060404,5.9002697149376,3.64050907030736));
#29040=CARTESIAN_POINT('Ctrl Pts',(56.5906497107553,6.94742639347645,1.94335443675065));
#29041=CARTESIAN_POINT('Ctrl Pts',(56.5334255154702,7.21086008527512,-0.216464293124029));
#29042=CARTESIAN_POINT('Ctrl Pts',(56.4762013201851,6.60233935006077,-2.11556236179393));
#29043=CARTESIAN_POINT('Ctrl Pts',(56.4189771249,5.99381861484643,-4.01466043046382));
#29044=CARTESIAN_POINT('Ctrl Pts',(56.3617529296149,4.52419779647274,-5.61916312790461));
#29045=CARTESIAN_POINT('Ctrl Pts',(56.3045287343298,2.68569473000371,-6.39167683923634));
#29046=CARTESIAN_POINT('Ctrl Pts',(56.2473045390448,0.847191663534686,-7.16419055056807));
#29047=CARTESIAN_POINT('Ctrl Pts',(56.1900803437596,-1.32739978994219,-7.0909357462378));
#29048=CARTESIAN_POINT('Ctrl Pts',(56.1328561484746,-3.10974706736239,-6.19644754492693));
#29049=CARTESIAN_POINT('Ctrl Pts',(56.0756319531895,-4.89209434478259,-5.30195934361607));
#29050=CARTESIAN_POINT('Ctrl Pts',(56.0184077579044,-6.25040525058691,-3.60219296582612));
#29051=CARTESIAN_POINT('Ctrl Pts',(55.9611835626193,-6.7297428071278,-1.66644854403358));
#29052=CARTESIAN_POINT('Ctrl Pts',(55.9450862629483,-6.86458158035573,-1.12191912096708));
#29053=CARTESIAN_POINT('Ctrl Pts',(55.9289889632773,-6.93299999999995,-0.560975745778276));
#29054=CARTESIAN_POINT('Ctrl Pts',(55.9128916636063,-6.933,-6.65856259018938E-13));
#29055=CARTESIAN_POINT('Ctrl Pts',(55.7335483363939,-6.933,-5.85170800704304E-12));
#29056=CARTESIAN_POINT('Ctrl Pts',(55.790772531679,-6.93299999999832,-1.99420935702216));
#29057=CARTESIAN_POINT('Ctrl Pts',(55.8479967269641,-6.02307502628911,-3.97063309653559));
#29058=CARTESIAN_POINT('Ctrl Pts',(55.9052209222492,-4.50798484753533,-5.26731066241511));
#29059=CARTESIAN_POINT('Ctrl Pts',(55.9624451175343,-2.99289466878154,-6.56398822829463));
#29060=CARTESIAN_POINT('Ctrl Pts',(56.0196693128194,-0.899664345622583,
-7.15779044292489));
#29061=CARTESIAN_POINT('Ctrl Pts',(56.0768935081045,1.07062371682442,-6.84983604599213));
#29062=CARTESIAN_POINT('Ctrl Pts',(56.1341177033896,3.04091177927143,-6.54188164905936));
#29063=CARTESIAN_POINT('Ctrl Pts',(56.1913418986747,4.85311303640352,-5.33766370385973));
#29064=CARTESIAN_POINT('Ctrl Pts',(56.2485660939598,5.90026971494084,-3.64050907030211));
#29065=CARTESIAN_POINT('Ctrl Pts',(56.3057902892449,6.94742639347816,-1.94335443674449));
#29066=CARTESIAN_POINT('Ctrl Pts',(56.36301448453,7.21086008527492,0.216464293130376));
#29067=CARTESIAN_POINT('Ctrl Pts',(56.4202386798151,6.60233935005892,2.11556236179971));
#29068=CARTESIAN_POINT('Ctrl Pts',(56.4774628751002,5.99381861484291,4.01466043046907));
#29069=CARTESIAN_POINT('Ctrl Pts',(56.5346870703853,4.52419779646782,5.61916312790858));
#29070=CARTESIAN_POINT('Ctrl Pts',(56.5919112656704,2.68569472999811,6.3916768392387));
#29071=CARTESIAN_POINT('Ctrl Pts',(56.6491354609555,0.847191663528411,7.16419055056882));
#29072=CARTESIAN_POINT('Ctrl Pts',(56.7063596562406,-1.3273997899484,7.09093574623663));
#29073=CARTESIAN_POINT('Ctrl Pts',(56.7635838515257,-3.10974706736782,6.19644754492421));
#29074=CARTESIAN_POINT('Ctrl Pts',(56.8208080468108,-4.89209434478723,5.30195934361179));
#29075=CARTESIAN_POINT('Ctrl Pts',(56.8780322420959,-6.25040525059006,3.60219296582064));
#29076=CARTESIAN_POINT('Ctrl Pts',(56.935256437381,-6.72974280712926,1.66644854402768));
#29077=CARTESIAN_POINT('Ctrl Pts',(56.951353737052,-6.86458158035676,1.12191912096091));
#29078=CARTESIAN_POINT('Ctrl Pts',(56.9674510367229,-6.93300000000048,0.560975745771875));
#29079=CARTESIAN_POINT('Ctrl Pts',(56.9835483363939,-6.933,-5.89944759710193E-12));
#29080=CARTESIAN_POINT('Origin',(29.75,0.,0.));
#29081=CARTESIAN_POINT('',(58.4128916636063,-6.933,-4.64905891561784E-13));
#29082=CARTESIAN_POINT('',(58.2335483363939,-6.93876249354147,-0.00788840371280948));
#29083=CARTESIAN_POINT('',(29.75,-6.933,-8.4904762584886E-16));
#29084=CARTESIAN_POINT('Ctrl Pts',(58.4128916636063,-6.933,-4.64905891561784E-13));
#29085=CARTESIAN_POINT('Ctrl Pts',(58.3556674683212,-6.93300000000013,1.99420935701588));
#29086=CARTESIAN_POINT('Ctrl Pts',(58.2984432730361,-6.0230750262927,3.97063309653017));
#29087=CARTESIAN_POINT('Ctrl Pts',(58.241219077751,-4.50798484754005,5.26731066241107));
#29088=CARTESIAN_POINT('Ctrl Pts',(58.1839948824659,-2.9928946687874,6.56398822829196));
#29089=CARTESIAN_POINT('Ctrl Pts',(58.1267706871808,-0.899664345628934,
7.1577904429241));
#29090=CARTESIAN_POINT('Ctrl Pts',(58.0695464918957,1.07062371681838,6.84983604599307));
#29091=CARTESIAN_POINT('Ctrl Pts',(58.0123222966106,3.04091177926569,6.54188164906204));
#29092=CARTESIAN_POINT('Ctrl Pts',(57.9550981013255,4.85311303639887,5.33766370386397));
#29093=CARTESIAN_POINT('Ctrl Pts',(57.8978739060404,5.90026971493768,3.64050907030724));
#29094=CARTESIAN_POINT('Ctrl Pts',(57.8406497107553,6.94742639347649,1.9433544367505));
#29095=CARTESIAN_POINT('Ctrl Pts',(57.7834255154702,7.21086008527511,-0.216464293124184));
#29096=CARTESIAN_POINT('Ctrl Pts',(57.7262013201851,6.60233935006073,-2.11556236179407));
#29097=CARTESIAN_POINT('Ctrl Pts',(57.6689771249,5.99381861484634,-4.01466043046395));
#29098=CARTESIAN_POINT('Ctrl Pts',(57.6117529296149,4.52419779647262,-5.61916312790471));
#29099=CARTESIAN_POINT('Ctrl Pts',(57.5545287343298,2.68569473000357,-6.3916768392364));
#29100=CARTESIAN_POINT('Ctrl Pts',(57.4973045390447,0.847191663534532,-7.16419055056809));
#29101=CARTESIAN_POINT('Ctrl Pts',(57.4400803437596,-1.32739978994234,-7.09093574623777));
#29102=CARTESIAN_POINT('Ctrl Pts',(57.3828561484745,-3.10974706736252,-6.19644754492687));
#29103=CARTESIAN_POINT('Ctrl Pts',(57.3256319531895,-4.8920943447827,-5.30195934361597));
#29104=CARTESIAN_POINT('Ctrl Pts',(57.2684077579043,-6.25040525058699,-3.60219296582598));
#29105=CARTESIAN_POINT('Ctrl Pts',(57.2111835626193,-6.72974280712784,-1.66644854403343));
#29106=CARTESIAN_POINT('Ctrl Pts',(57.1950862629483,-6.86458158035575,-1.12191912096696));
#29107=CARTESIAN_POINT('Ctrl Pts',(57.1789889632773,-6.93299999999995,-0.560975745778193));
#29108=CARTESIAN_POINT('Ctrl Pts',(57.1628916636063,-6.933,-6.1478599988618E-13));
#29109=CARTESIAN_POINT('Ctrl Pts',(56.9835483363939,-6.91923797360895,0.00171470667456418));
#29110=CARTESIAN_POINT('Ctrl Pts',(57.0130389515682,-6.92101525208908,-1.02900630106465));
#29111=CARTESIAN_POINT('Ctrl Pts',(57.0425295667424,-6.70489479915974,-2.0598170771908));
#29112=CARTESIAN_POINT('Ctrl Pts',(57.0720201819166,-6.26630550510988,-2.98661216848789));
#29113=CARTESIAN_POINT('Ctrl Pts',(57.1051054493236,-5.77425595003048,-4.02637560665029));
#29114=CARTESIAN_POINT('Ctrl Pts',(57.1381907167306,-5.00219814537272,-4.93522071175101));
#29115=CARTESIAN_POINT('Ctrl Pts',(57.1712759841377,-4.06538541530075,-5.61158308860758));
#29116=CARTESIAN_POINT('Ctrl Pts',(57.2043612515447,-3.12857268522872,-6.2879454654642));
#29117=CARTESIAN_POINT('Ctrl Pts',(57.2374465189517,-2.02700502974241,-6.73182511407668));
#29118=CARTESIAN_POINT('Ctrl Pts',(57.2705317863588,-0.88714999921381,-6.87883010959571));
#29119=CARTESIAN_POINT('Ctrl Pts',(57.3036170537658,0.252705031314849,-7.02583510511475));
#29120=CARTESIAN_POINT('Ctrl Pts',(57.3367023211728,1.43084743688566,-6.87596544754036));
#29121=CARTESIAN_POINT('Ctrl Pts',(57.3697875885798,2.50861057196623,-6.45941919475009));
#29122=CARTESIAN_POINT('Ctrl Pts',(57.4028728559868,3.58637370704667,-6.04287294195987));
#29123=CARTESIAN_POINT('Ctrl Pts',(57.4359581233938,4.56375757163673,-5.35965009395384));
#29124=CARTESIAN_POINT('Ctrl Pts',(57.4690433908008,5.3035115407242,-4.47875007850801));
#29125=CARTESIAN_POINT('Ctrl Pts',(57.5352139256149,6.7830194788992,-2.71695004761632));
#29126=CARTESIAN_POINT('Ctrl Pts',(57.6013844604289,7.31200783506392,-0.164441346965323));
#29127=CARTESIAN_POINT('Ctrl Pts',(57.667554995243,6.64204806609351,2.02813254164841));
#29128=CARTESIAN_POINT('Ctrl Pts',(57.733725530057,5.97208829712309,4.2207064302622));
#29129=CARTESIAN_POINT('Ctrl Pts',(57.799896064871,4.10318040301745,6.0533455068388));
#29130=CARTESIAN_POINT('Ctrl Pts',(57.8660665996851,1.89437680725851,6.6812873951947));
#29131=CARTESIAN_POINT('Ctrl Pts',(57.9322371344991,-0.31442678850043,7.3092292835506));
#29132=CARTESIAN_POINT('Ctrl Pts',(57.9984076693131,-2.86312608591256,6.73247398368588));
#29133=CARTESIAN_POINT('Ctrl Pts',(58.0645782041272,-4.58637444068998,5.21473242217204));
#29134=CARTESIAN_POINT('Ctrl Pts',(58.1209015815494,-6.0531778714189,3.92285332464293));
#29135=CARTESIAN_POINT('Ctrl Pts',(58.1772249589717,-6.92192873783322,1.94921445473074));
#29136=CARTESIAN_POINT('Ctrl Pts',(58.2335483363939,-6.93876249354147,-0.00788840371280948));
#29137=CARTESIAN_POINT('Origin',(29.75,0.,0.));
#29138=CARTESIAN_POINT('',(59.6628916636063,-6.933,-3.15580894749701E-13));
#29139=CARTESIAN_POINT('',(59.483548336394,-6.93838776086578,0.00532365672661986));
#29140=CARTESIAN_POINT('',(29.75,-6.933,-8.4904762584886E-16));
#29141=CARTESIAN_POINT('Ctrl Pts',(59.6628916636063,-6.933,-1.18793863634892E-13));
#29142=CARTESIAN_POINT('Ctrl Pts',(59.6056674683212,-6.93300000000003,1.99420935701622));
#29143=CARTESIAN_POINT('Ctrl Pts',(59.5484432730361,-6.0230750262925,3.97063309653047));
#29144=CARTESIAN_POINT('Ctrl Pts',(59.491219077751,-4.50798484753979,5.26731066241129));
#29145=CARTESIAN_POINT('Ctrl Pts',(59.4339948824659,-2.99289466878708,6.56398822829211));
#29146=CARTESIAN_POINT('Ctrl Pts',(59.3767706871808,-0.899664345628577,
7.15779044292415));
#29147=CARTESIAN_POINT('Ctrl Pts',(59.3195464918957,1.07062371681872,6.84983604599302));
#29148=CARTESIAN_POINT('Ctrl Pts',(59.2623222966106,3.04091177926602,6.54188164906189));
#29149=CARTESIAN_POINT('Ctrl Pts',(59.2050981013255,4.85311303639914,5.33766370386373));
#29150=CARTESIAN_POINT('Ctrl Pts',(59.1478739060404,5.90026971493786,3.64050907030694));
#29151=CARTESIAN_POINT('Ctrl Pts',(59.0906497107553,6.94742639347658,1.94335443675015));
#29152=CARTESIAN_POINT('Ctrl Pts',(59.0334255154702,7.2108600852751,-0.216464293124544));
#29153=CARTESIAN_POINT('Ctrl Pts',(58.9762013201851,6.60233935006062,-2.1155623617944));
#29154=CARTESIAN_POINT('Ctrl Pts',(58.9189771249,5.99381861484614,-4.01466043046425));
#29155=CARTESIAN_POINT('Ctrl Pts',(58.8617529296149,4.52419779647234,-5.61916312790494));
#29156=CARTESIAN_POINT('Ctrl Pts',(58.8045287343298,2.68569473000325,-6.39167683923653));
#29157=CARTESIAN_POINT('Ctrl Pts',(58.7473045390447,0.847191663534174,-7.16419055056813));
#29158=CARTESIAN_POINT('Ctrl Pts',(58.6900803437596,-1.3273997899427,-7.0909357462377));
#29159=CARTESIAN_POINT('Ctrl Pts',(58.6328561484745,-3.10974706736283,-6.19644754492671));
#29160=CARTESIAN_POINT('Ctrl Pts',(58.5756319531895,-4.89209434478297,-5.30195934361572));
#29161=CARTESIAN_POINT('Ctrl Pts',(58.5184077579043,-6.25040525058717,-3.60219296582567));
#29162=CARTESIAN_POINT('Ctrl Pts',(58.4611835626192,-6.72974280712792,-1.66644854403309));
#29163=CARTESIAN_POINT('Ctrl Pts',(58.4450862629483,-6.86458158035579,-1.12191912096668));
#29164=CARTESIAN_POINT('Ctrl Pts',(58.4289889632773,-6.93299999999996,-0.560975745777977));
#29165=CARTESIAN_POINT('Ctrl Pts',(58.4128916636063,-6.933,-4.64905891561784E-13));
#29166=CARTESIAN_POINT('Ctrl Pts',(58.2335483363939,-6.93876249354147,-0.00788840371280948));
#29167=CARTESIAN_POINT('Ctrl Pts',(58.2433954937857,-6.94170558128835,-0.350053606884688));
#29168=CARTESIAN_POINT('Ctrl Pts',(58.2532426511775,-6.9186086245689,-0.691713363612853));
#29169=CARTESIAN_POINT('Ctrl Pts',(58.2630898085693,-6.86811497086886,-1.02913598018768));
#29170=CARTESIAN_POINT('Ctrl Pts',(58.3292603433833,-6.52880973412778,-3.2965349978707));
#29171=CARTESIAN_POINT('Ctrl Pts',(58.3954308781973,-4.95240184850311,-5.37260521007374));
#29172=CARTESIAN_POINT('Ctrl Pts',(58.4616014130114,-2.85851431917938,-6.32576736968542));
#29173=CARTESIAN_POINT('Ctrl Pts',(58.4946866804184,-1.81157055451755,-6.80234844949124));
#29174=CARTESIAN_POINT('Ctrl Pts',(58.5277719478254,-0.635256878931015,
-6.99820251614922));
#29175=CARTESIAN_POINT('Ctrl Pts',(58.5608572152324,0.516841190274217,-6.91014460914694));
#29176=CARTESIAN_POINT('Ctrl Pts',(58.5939424826395,1.66893925947945,-6.82208670214467));
#29177=CARTESIAN_POINT('Ctrl Pts',(58.6270277500465,2.79682172230348,-6.45011682148206));
#29178=CARTESIAN_POINT('Ctrl Pts',(58.6601130174535,3.76233056023795,-5.82668066340393));
#29179=CARTESIAN_POINT('Ctrl Pts',(58.6931982848605,4.72783939817248,-5.20324450532576));
#29180=CARTESIAN_POINT('Ctrl Pts',(58.7262835522675,5.53097461121756,-4.32834206983201));
#29181=CARTESIAN_POINT('Ctrl Pts',(58.7593688196746,6.08531354531465,-3.31454105276985));
#29182=CARTESIAN_POINT('Ctrl Pts',(58.7924540870816,6.63965247941167,-2.30074003570779));
#29183=CARTESIAN_POINT('Ctrl Pts',(58.8255393544886,6.94519513456072,-1.14804043707739));
#29184=CARTESIAN_POINT('Ctrl Pts',(58.8586246218956,6.94164474653778,0.00226742029728548));
#29185=CARTESIAN_POINT('Ctrl Pts',(58.9247951567097,6.9345439704919,2.30288313504689));
#29186=CARTESIAN_POINT('Ctrl Pts',(58.9909656915237,5.69107102175774,4.5939318847734));
#29187=CARTESIAN_POINT('Ctrl Pts',(59.0571362263377,3.76415786551684,5.83620079180433));
#29188=CARTESIAN_POINT('Ctrl Pts',(59.1233067611518,1.83724470927605,7.07846969883519));
#29189=CARTESIAN_POINT('Ctrl Pts',(59.1894772959658,-0.773108654471531,
7.27195876317054));
#29190=CARTESIAN_POINT('Ctrl Pts',(59.2556478307798,-2.86550398523472,6.32591113245124));
#29191=CARTESIAN_POINT('Ctrl Pts',(59.3218183655939,-4.95789931599796,5.37986350173191));
#29192=CARTESIAN_POINT('Ctrl Pts',(59.3879889004079,-6.53233661377687,3.29427917595797));
#29193=CARTESIAN_POINT('Ctrl Pts',(59.454159435222,-6.86893290788461,1.02275385701864));
#29194=CARTESIAN_POINT('Ctrl Pts',(59.4639557356126,-6.91876473131977,0.686463022557893));
#29195=CARTESIAN_POINT('Ctrl Pts',(59.4737520360033,-6.94146593200598,0.34609678994491));
#29196=CARTESIAN_POINT('Ctrl Pts',(59.483548336394,-6.93838776086578,0.00532365672661986));
#29197=CARTESIAN_POINT('Origin',(29.75,0.,0.));
#29198=CARTESIAN_POINT('',(60.9128916636063,-6.933,-1.66533453693773E-13));
#29199=CARTESIAN_POINT('',(60.7335483363939,-6.9239281092218,0.00189150495899608));
#29200=CARTESIAN_POINT('',(29.75,-6.933,-8.4904762584886E-16));
#29201=CARTESIAN_POINT('Ctrl Pts',(60.9128916636063,-6.93063399872081,-3.45088283915107E-5));
#29202=CARTESIAN_POINT('Ctrl Pts',(60.8848211492598,-6.93354690158584,0.980671123326722));
#29203=CARTESIAN_POINT('Ctrl Pts',(60.8567506349133,-6.73243917945665,1.96229231020105));
#29204=CARTESIAN_POINT('Ctrl Pts',(60.8286801205668,-6.32914499442313,2.85102798441176));
#29205=CARTESIAN_POINT('Ctrl Pts',(60.7625095857528,-5.3784608857645,4.94604178234169));
#29206=CARTESIAN_POINT('Ctrl Pts',(60.6963390509388,-3.30425725422927,6.52490486785065));
#29207=CARTESIAN_POINT('Ctrl Pts',(60.6301685161248,-1.03726127266794,6.86689254109988));
#29208=CARTESIAN_POINT('Ctrl Pts',(60.5639979813107,1.22973470889339,7.2088802143491));
#29209=CARTESIAN_POINT('Ctrl Pts',(60.4978274464967,3.6895230404809,6.31399247533858));
#29210=CARTESIAN_POINT('Ctrl Pts',(60.4316569116826,5.20930240162831,4.59254104319776));
#29211=CARTESIAN_POINT('Ctrl Pts',(60.3654863768686,6.72908176277572,2.87108961105695));
#29212=CARTESIAN_POINT('Ctrl Pts',(60.2993158420546,7.30885215348307,0.323074485785975));
#29213=CARTESIAN_POINT('Ctrl Pts',(60.2331453072406,6.68352405143822,-1.88647051366126));
#29214=CARTESIAN_POINT('Ctrl Pts',(60.1669747724266,6.05819594939336,-4.09601551310856));
#29215=CARTESIAN_POINT('Ctrl Pts',(60.1008042376125,4.22776935459611,-5.96709038673199));
#29216=CARTESIAN_POINT('Ctrl Pts',(60.0346337027984,2.03598966376562,-6.63964383139859));
#29217=CARTESIAN_POINT('Ctrl Pts',(59.9684631679844,-0.155790027064813,
-7.31219727606518));
#29218=CARTESIAN_POINT('Ctrl Pts',(59.9022926331704,-2.70892281392854,-6.78622929177505));
#29219=CARTESIAN_POINT('Ctrl Pts',(59.8361220983563,-4.4724720920668,-5.30880686350652));
#29220=CARTESIAN_POINT('Ctrl Pts',(59.8030368309493,-5.3542467311359,-4.57009564937227));
#29221=CARTESIAN_POINT('Ctrl Pts',(59.7699515635423,-6.03862549302366,-3.59352082424343));
#29222=CARTESIAN_POINT('Ctrl Pts',(59.7368662961352,-6.45644661012001,-2.51625128036857));
#29223=CARTESIAN_POINT('Ctrl Pts',(59.7122080852923,-6.7678456710154,-1.71337006980382));
#29224=CARTESIAN_POINT('Ctrl Pts',(59.6875498744493,-6.93118226952631,-0.854556837411979));
#29225=CARTESIAN_POINT('Ctrl Pts',(59.6628916636063,-6.93388706352457,0.00279784803854183));
#29226=CARTESIAN_POINT('Ctrl Pts',(59.483548336394,-6.93838776086578,0.00532365672661986));
#29227=CARTESIAN_POINT('Ctrl Pts',(59.5399225708173,-6.92067397764835,-1.9557048674237));
#29228=CARTESIAN_POINT('Ctrl Pts',(59.5962968052407,-6.04925198579133,-3.9302082888362));
#29229=CARTESIAN_POINT('Ctrl Pts',(59.6526710396641,-4.58163035911404,-5.21907916889889));
#29230=CARTESIAN_POINT('Ctrl Pts',(59.7188415744781,-2.85897622579923,-6.73192056377248));
#29231=CARTESIAN_POINT('Ctrl Pts',(59.7850121092921,-0.314912668733032,
-7.30013704141502));
#29232=CARTESIAN_POINT('Ctrl Pts',(59.8511826441062,1.89962274248406,-6.67666611150862));
#29233=CARTESIAN_POINT('Ctrl Pts',(59.8842679115132,3.00689044809264,-6.36493064655541));
#29234=CARTESIAN_POINT('Ctrl Pts',(59.9173531789202,4.03177611723897,-5.75527332971494));
#29235=CARTESIAN_POINT('Ctrl Pts',(59.9504384463273,4.85491496267529,-4.94439319234203));
#29236=CARTESIAN_POINT('Ctrl Pts',(59.9835237137343,5.67805380811161,-4.13351305496913));
#29237=CARTESIAN_POINT('Ctrl Pts',(60.0166089811413,6.29944582983796,-3.12141009706376));
#29238=CARTESIAN_POINT('Ctrl Pts',(60.0496942485483,6.63450760188871,-2.02204047394371));
#29239=CARTESIAN_POINT('Ctrl Pts',(60.0827795159553,6.96956937393944,-0.922670850823727));
#29240=CARTESIAN_POINT('Ctrl Pts',(60.1158647833623,7.01830089631462,0.263965437510784));
#29241=CARTESIAN_POINT('Ctrl Pts',(60.1489500507693,6.7873490757456,1.39610739531813));
#29242=CARTESIAN_POINT('Ctrl Pts',(60.1820353181763,6.55639725517657,2.52824935312553));
#29243=CARTESIAN_POINT('Ctrl Pts',(60.2151205855834,6.04576209166327,3.60589698040562));
#29244=CARTESIAN_POINT('Ctrl Pts',(60.2482058529904,5.30058452960073,4.48221380267472));
#29245=CARTESIAN_POINT('Ctrl Pts',(60.3143763878044,3.81022940547564,6.23484744721291));
#29246=CARTESIAN_POINT('Ctrl Pts',(60.3805469226185,1.38170468715351,7.18215787170724));
#29247=CARTESIAN_POINT('Ctrl Pts',(60.4467174574325,-0.891899061462053,
6.88728104428395));
#29248=CARTESIAN_POINT('Ctrl Pts',(60.5128879922466,-3.16550281007755,6.59240421686066));
#29249=CARTESIAN_POINT('Ctrl Pts',(60.5790585270606,-5.28418558898654,5.05534013751981));
#29250=CARTESIAN_POINT('Ctrl Pts',(60.6452290618746,-6.27173702357961,2.98221049762208));
#29251=CARTESIAN_POINT('Ctrl Pts',(60.6746688200477,-6.71110592848,2.05985985572997));
#29252=CARTESIAN_POINT('Ctrl Pts',(60.7041085782208,-6.92657579720744,1.03139902341889));
#29253=CARTESIAN_POINT('Ctrl Pts',(60.7335483363939,-6.9239281092218,0.00189150495899608));
#29254=CARTESIAN_POINT('Origin',(29.75,0.,0.));
#29255=CARTESIAN_POINT('',(62.1628916636063,-6.93103310215991,-0.000748976776520713));
#29256=CARTESIAN_POINT('',(61.9835483363939,-6.93044600006181,-0.00576111198420661));
#29257=CARTESIAN_POINT('',(29.75,-6.933,-8.4904762584886E-16));
#29258=CARTESIAN_POINT('Ctrl Pts',(62.1628916636063,-6.933,-1.69309011255336E-14));
#29259=CARTESIAN_POINT('Ctrl Pts',(62.1056674683212,-6.93300000000001,1.99420935701633));
#29260=CARTESIAN_POINT('Ctrl Pts',(62.0484432730361,-6.02307502629244,3.97063309653056));
#29261=CARTESIAN_POINT('Ctrl Pts',(61.991219077751,-4.50798484753971,5.26731066241136));
#29262=CARTESIAN_POINT('Ctrl Pts',(61.9339948824659,-2.99289466878698,6.56398822829216));
#29263=CARTESIAN_POINT('Ctrl Pts',(61.8767706871808,-0.899664345628471,
7.15779044292416));
#29264=CARTESIAN_POINT('Ctrl Pts',(61.8195464918957,1.07062371681882,6.849836045993));
#29265=CARTESIAN_POINT('Ctrl Pts',(61.7623222966106,3.04091177926611,6.54188164906185));
#29266=CARTESIAN_POINT('Ctrl Pts',(61.7050981013255,4.85311303639922,5.33766370386366));
#29267=CARTESIAN_POINT('Ctrl Pts',(61.6478739060404,5.90026971493791,3.64050907030685));
#29268=CARTESIAN_POINT('Ctrl Pts',(61.5906497107553,6.94742639347661,1.94335443675005));
#29269=CARTESIAN_POINT('Ctrl Pts',(61.5334255154702,7.2108600852751,-0.21646429312465));
#29270=CARTESIAN_POINT('Ctrl Pts',(61.4762013201851,6.60233935006059,-2.11556236179449));
#29271=CARTESIAN_POINT('Ctrl Pts',(61.4189771249,5.99381861484609,-4.01466043046434));
#29272=CARTESIAN_POINT('Ctrl Pts',(61.3617529296149,4.52419779647225,-5.619163127905));
#29273=CARTESIAN_POINT('Ctrl Pts',(61.3045287343298,2.68569473000316,-6.39167683923658));
#29274=CARTESIAN_POINT('Ctrl Pts',(61.2473045390447,0.847191663534068,-7.16419055056815));
#29275=CARTESIAN_POINT('Ctrl Pts',(61.1900803437596,-1.3273997899428,-7.09093574623768));
#29276=CARTESIAN_POINT('Ctrl Pts',(61.1328561484745,-3.10974706736292,-6.19644754492667));
#29277=CARTESIAN_POINT('Ctrl Pts',(61.0756319531895,-4.89209434478304,-5.30195934361565));
#29278=CARTESIAN_POINT('Ctrl Pts',(61.0184077579043,-6.25040525058722,-3.60219296582558));
#29279=CARTESIAN_POINT('Ctrl Pts',(60.9611835626192,-6.72974280712794,-1.66644854403299));
#29280=CARTESIAN_POINT('Ctrl Pts',(60.9450862629483,-6.86458158035582,-1.12191912096652));
#29281=CARTESIAN_POINT('Ctrl Pts',(60.9289889632773,-6.93299999999999,-0.560975745777744));
#29282=CARTESIAN_POINT('Ctrl Pts',(60.9128916636063,-6.933,-1.66533453693773E-13));
#29283=CARTESIAN_POINT('Ctrl Pts',(60.7335483363939,-6.9239281092218,0.00189150495899608));
#29284=CARTESIAN_POINT('Ctrl Pts',(60.7702791130349,-6.9206246977113,-1.28258272503899));
#29285=CARTESIAN_POINT('Ctrl Pts',(60.8070098896758,-6.57778798958841,-2.56868628191917));
#29286=CARTESIAN_POINT('Ctrl Pts',(60.8437406663167,-5.90664661057516,-3.65236780224111));
#29287=CARTESIAN_POINT('Ctrl Pts',(60.9099112011308,-4.69758467270039,-5.60462126175199));
#29288=CARTESIAN_POINT('Ctrl Pts',(60.9760817359448,-2.42304070667363,-6.89993298031901));
#29289=CARTESIAN_POINT('Ctrl Pts',(61.0422522707589,-0.130809673177829,
-6.94355909805576));
#29290=CARTESIAN_POINT('Ctrl Pts',(61.1084228055729,2.16142136031784,-6.98718521579251));
#29291=CARTESIAN_POINT('Ctrl Pts',(61.1745933403869,4.47133946128256,-5.77912573269915));
#29292=CARTESIAN_POINT('Ctrl Pts',(61.240763875201,5.76038884520191,-3.87354582784349));
#29293=CARTESIAN_POINT('Ctrl Pts',(61.273849142608,6.40491353716163,-2.9207558754156));
#29294=CARTESIAN_POINT('Ctrl Pts',(61.306934410015,6.79422104985998,-1.79358581754712));
#29295=CARTESIAN_POINT('Ctrl Pts',(61.340019677422,6.89955457142813,-0.642938606067334));
#29296=CARTESIAN_POINT('Ctrl Pts',(61.373104944829,7.00488809299628,0.507708605412388));
#29297=CARTESIAN_POINT('Ctrl Pts',(61.4061902122361,6.82624762343428,1.68183297050341));
#29298=CARTESIAN_POINT('Ctrl Pts',(61.4392754796431,6.37258105776411,2.73780011323174));
#29299=CARTESIAN_POINT('Ctrl Pts',(61.4723607470501,5.91891449209395,3.79376725596006));
#29300=CARTESIAN_POINT('Ctrl Pts',(61.5054460144571,5.19022183031563,4.73157717632567));
#29301=CARTESIAN_POINT('Ctrl Pts',(61.5385312818641,4.28307957908654,5.44724266528475));
#29302=CARTESIAN_POINT('Ctrl Pts',(61.5716165492711,3.3759373278574,6.16290815424387));
#29303=CARTESIAN_POINT('Ctrl Pts',(61.6047018166782,2.29034548717748,6.65642921179643));
#29304=CARTESIAN_POINT('Ctrl Pts',(61.6377870840852,1.15555838515488,6.84478792562842));
#29305=CARTESIAN_POINT('Ctrl Pts',(61.7039576188993,-1.11401581889026,7.22150535329239));
#29306=CARTESIAN_POINT('Ctrl Pts',(61.7701281537132,-3.58037106830612,6.37757340607417));
#29307=CARTESIAN_POINT('Ctrl Pts',(61.8362986885273,-5.12662795410679,4.68484897717745));
#29308=CARTESIAN_POINT('Ctrl Pts',(61.8853819044828,-6.27359254887378,3.42923937797663));
#29309=CARTESIAN_POINT('Ctrl Pts',(61.9344651204383,-6.91430020443789,1.70660679429336));
#29310=CARTESIAN_POINT('Ctrl Pts',(61.9835483363939,-6.93044600006181,-0.00576111198420661));
#29311=CARTESIAN_POINT('Origin',(29.75,0.,0.));
#29312=CARTESIAN_POINT('',(63.4128916636063,-6.94470568062749,-0.000764679492917131));
#29313=CARTESIAN_POINT('',(63.2335483363939,-6.94425137989254,0.00364565552205904));
#29314=CARTESIAN_POINT('',(29.75,-6.933,-8.4904762584886E-16));
#29315=CARTESIAN_POINT('Ctrl Pts',(63.4128916636063,-6.94470568062749,-0.000764679492917131));
#29316=CARTESIAN_POINT('Ctrl Pts',(63.411704768509,-6.94477403368304,0.0403562036678778));
#29317=CARTESIAN_POINT('Ctrl Pts',(63.4105178734116,-6.94444287705134,0.081477862393955));
#29318=CARTESIAN_POINT('Ctrl Pts',(63.4093309783143,-6.94370900561522,0.122594307078241));
#29319=CARTESIAN_POINT('Ctrl Pts',(63.3431604435003,-6.90279497241768,2.41487535244701));
#29320=CARTESIAN_POINT('Ctrl Pts',(63.2769899086863,-5.61017528801263,4.69095027501292));
#29321=CARTESIAN_POINT('Ctrl Pts',(63.2108193738722,-3.65935369701219,5.90232117604843));
#29322=CARTESIAN_POINT('Ctrl Pts',(63.1446488390582,-1.70853210601164,7.11369207708401));
#29323=CARTESIAN_POINT('Ctrl Pts',(63.0784783042442,0.900491391584395,7.26035895658904));
#29324=CARTESIAN_POINT('Ctrl Pts',(63.0123077694301,2.97478800230089,6.27526103731416));
#29325=CARTESIAN_POINT('Ctrl Pts',(62.9461372346161,5.0490846130174,5.29016311803928));
#29326=CARTESIAN_POINT('Ctrl Pts',(62.879966699802,6.58865433685436,3.17330039998448));
#29327=CARTESIAN_POINT('Ctrl Pts',(62.813796164988,6.88622097301192,0.900047126344276));
#29328=CARTESIAN_POINT('Ctrl Pts',(62.747625630174,7.18378760916946,-1.37320614729579));
#29329=CARTESIAN_POINT('Ctrl Pts',(62.68145509536,6.23935115764776,-3.80284997652125));
#29330=CARTESIAN_POINT('Ctrl Pts',(62.6152845605459,4.48848205404005,-5.29527768666486));
#29331=CARTESIAN_POINT('Ctrl Pts',(62.5821992931389,3.61304750223614,-6.04149154173671));
#29332=CARTESIAN_POINT('Ctrl Pts',(62.5491140257318,2.53600478741071,-6.55340136703808));
#29333=CARTESIAN_POINT('Ctrl Pts',(62.5160287583248,1.40413687274796,-6.78569252013943));
#29334=CARTESIAN_POINT('Ctrl Pts',(62.4829434909178,0.272268958085274,-7.01798367324077));
#29335=CARTESIAN_POINT('Ctrl Pts',(62.4498582235108,-0.914424156414728,
-6.97065615414214));
#29336=CARTESIAN_POINT('Ctrl Pts',(62.4167729561038,-2.01418943852191,-6.63689533618939));
#29337=CARTESIAN_POINT('Ctrl Pts',(62.3836876886968,-3.11395472062909,-6.30313451823664));
#29338=CARTESIAN_POINT('Ctrl Pts',(62.3506024212897,-4.12679217034345,-5.68294040142978));
#29339=CARTESIAN_POINT('Ctrl Pts',(62.3175171538827,-4.93864563719572,-4.86076152526476));
#29340=CARTESIAN_POINT('Ctrl Pts',(62.2844318864757,-5.75049910404804,-4.03858264909971));
#29341=CARTESIAN_POINT('Ctrl Pts',(62.2513466190687,-6.36136858803824,-3.01441901357648));
#29342=CARTESIAN_POINT('Ctrl Pts',(62.2182613516617,-6.67441389900069,-1.90752091290157));
#29343=CARTESIAN_POINT('Ctrl Pts',(62.1998047889765,-6.84904571726545,-1.29003960529028));
#29344=CARTESIAN_POINT('Ctrl Pts',(62.1813482262914,-6.93099619848535,-0.646811761486181));
#29345=CARTESIAN_POINT('Ctrl Pts',(62.1628916636063,-6.92559703060158,-0.00281898329623498));
#29346=CARTESIAN_POINT('Ctrl Pts',(61.9835483363939,-6.93044600006181,-0.00576111198420661));
#29347=CARTESIAN_POINT('Ctrl Pts',(62.0006356552524,-6.93606682894759,-0.601887014657739));
#29348=CARTESIAN_POINT('Ctrl Pts',(62.0177229741109,-6.86599438447961,-1.19676889799133));
#29349=CARTESIAN_POINT('Ctrl Pts',(62.0348102929694,-6.71523723016996,-1.77026938277931));
#29350=CARTESIAN_POINT('Ctrl Pts',(62.1009808277835,-6.13143109824698,-3.99114640326435));
#29351=CARTESIAN_POINT('Ctrl Pts',(62.1671513625975,-4.33766031221545,-5.89138353365921));
#29352=CARTESIAN_POINT('Ctrl Pts',(62.2333218974115,-2.15409411222323,-6.60213172397762));
#29353=CARTESIAN_POINT('Ctrl Pts',(62.2994924322255,0.0294720877690602,
-7.31287991429606));
#29354=CARTESIAN_POINT('Ctrl Pts',(62.3656629670396,2.60283370172207,-6.83413916453793));
#29355=CARTESIAN_POINT('Ctrl Pts',(62.4318335018536,4.38180475697552,-5.38794127571344));
#29356=CARTESIAN_POINT('Ctrl Pts',(62.4980040366677,6.16077581222893,-3.94174338688899));
#29357=CARTESIAN_POINT('Ctrl Pts',(62.5641745714817,7.14535630878282,-1.52808835899822));
#29358=CARTESIAN_POINT('Ctrl Pts',(62.6303451062957,6.8999800818199,0.759415432302316));
#29359=CARTESIAN_POINT('Ctrl Pts',(62.6634303737028,6.77729196833845,1.90316732795255));
#29360=CARTESIAN_POINT('Ctrl Pts',(62.6965156411098,6.3471146739778,3.01538141445524));
#29361=CARTESIAN_POINT('Ctrl Pts',(62.7296009085168,5.68488391631017,3.9622365140618));
#29362=CARTESIAN_POINT('Ctrl Pts',(62.7626861759238,5.02265315864249,4.90909161366842));
#29363=CARTESIAN_POINT('Ctrl Pts',(62.7957714433308,4.1283689376678,5.6905877263789));
#29364=CARTESIAN_POINT('Ctrl Pts',(62.8288567107379,3.10028353477502,6.20431952769911));
#29365=CARTESIAN_POINT('Ctrl Pts',(62.8619419781449,2.07219813188224,6.71805132901933));
#29366=CARTESIAN_POINT('Ctrl Pts',(62.8950272455519,0.910311547071365,6.96401881894927));
#29367=CARTESIAN_POINT('Ctrl Pts',(62.9281125129589,-0.244492304498008,
6.92513154014622));
#29368=CARTESIAN_POINT('Ctrl Pts',(62.9611977803659,-1.39929615606738,6.88624426134317));
#29369=CARTESIAN_POINT('Ctrl Pts',(62.994283047773,-2.54701727439525,6.56250221380711));
#29370=CARTESIAN_POINT('Ctrl Pts',(63.02736831518,-3.53534695572987,5.97392323611058));
#29371=CARTESIAN_POINT('Ctrl Pts',(63.093538849994,-5.51200631839906,4.79676528071754));
#29372=CARTESIAN_POINT('Ctrl Pts',(63.1597093848081,-6.8510999330953,2.56025960468261));
#29373=CARTESIAN_POINT('Ctrl Pts',(63.2258799196221,-6.93956701425102,0.269320948886368));
#29374=CARTESIAN_POINT('Ctrl Pts',(63.228436058546,-6.94298445904371,0.180822986962495));
#29375=CARTESIAN_POINT('Ctrl Pts',(63.23099219747,-6.94453566485637,0.092243797792992));
#29376=CARTESIAN_POINT('Ctrl Pts',(63.2335483363939,-6.94425137989254,0.00364565552205904));
#29377=CARTESIAN_POINT('Origin',(29.75,0.,0.));
#29378=CARTESIAN_POINT('',(64.6628916636063,-6.9266679019854,0.00480994512238903));
#29379=CARTESIAN_POINT('',(64.483548336394,-6.92953670012574,0.00054474835552538));
#29380=CARTESIAN_POINT('',(29.75,-6.933,-8.4904762584886E-16));
#29381=CARTESIAN_POINT('Ctrl Pts',(64.6628916636063,-6.9266679019854,0.00480994512238903));
#29382=CARTESIAN_POINT('Ctrl Pts',(64.6420613107265,-6.93261174586027,0.732499836952666));
#29383=CARTESIAN_POINT('Ctrl Pts',(64.6212309578468,-6.82760440508976,1.45863474940064));
#29384=CARTESIAN_POINT('Ctrl Pts',(64.600400604967,-6.60467572025062,2.14628128990626));
#29385=CARTESIAN_POINT('Ctrl Pts',(64.534230070153,-5.89651151456714,4.33068688355847));
#29386=CARTESIAN_POINT('Ctrl Pts',(64.4680595353389,-3.99839801476722,6.12670468035998));
#29387=CARTESIAN_POINT('Ctrl Pts',(64.4018890005249,-1.77821327916756,6.71313803514095));
#29388=CARTESIAN_POINT('Ctrl Pts',(64.3357184657109,0.441971456432111,7.29957138992192));
#29389=CARTESIAN_POINT('Ctrl Pts',(64.2695479308968,2.9842274278316,6.67642030268235));
#29390=CARTESIAN_POINT('Ctrl Pts',(64.2033773960828,4.67878012636471,5.13216724668294));
#29391=CARTESIAN_POINT('Ctrl Pts',(64.1372068612687,6.37333282489787,3.58791419068348));
#29392=CARTESIAN_POINT('Ctrl Pts',(64.0710363264547,7.22018225056462,1.12255916592427));
#29393=CARTESIAN_POINT('Ctrl Pts',(64.0048657916407,6.84615033414182,-1.14745916295991));
#29394=CARTESIAN_POINT('Ctrl Pts',(63.9717805242337,6.65913437593043,-2.28246832740194));
#29395=CARTESIAN_POINT('Ctrl Pts',(63.9386952568267,6.16689808219666,-3.3686433178752));
#29396=CARTESIAN_POINT('Ctrl Pts',(63.9056099894197,5.45230637984183,-4.27663167406574));
#29397=CARTESIAN_POINT('Ctrl Pts',(63.8725247220126,4.73771467748695,-5.18462003025633));
#29398=CARTESIAN_POINT('Ctrl Pts',(63.8394394546056,3.80076756651095,-5.9144217521642));
#29399=CARTESIAN_POINT('Ctrl Pts',(63.8063541871985,2.7453379186447,-6.36933736822265));
#29400=CARTESIAN_POINT('Ctrl Pts',(63.7732689197915,1.68990827077845,-6.8242529842811));
#29401=CARTESIAN_POINT('Ctrl Pts',(63.7401836523845,0.515996086021923,-7.00428249449014));
#29402=CARTESIAN_POINT('Ctrl Pts',(63.7070983849775,-0.634774945489243,
-6.90031043532577));
#29403=CARTESIAN_POINT('Ctrl Pts',(63.6740131175705,-1.78554597700034,-6.7963383761614));
#29404=CARTESIAN_POINT('Ctrl Pts',(63.6409278501635,-2.91317585526612,-6.40836474762363));
#29405=CARTESIAN_POINT('Ctrl Pts',(63.6078425827564,-3.86672771044496,-5.76496780056987));
#29406=CARTESIAN_POINT('Ctrl Pts',(63.5428589430397,-5.73962386829838,-4.50125501602957));
#29407=CARTESIAN_POINT('Ctrl Pts',(63.477875303323,-6.94096328557867,-2.25217229100375));
#29408=CARTESIAN_POINT('Ctrl Pts',(63.4128916636063,-6.94470568062749,-0.000764679492917131));
#29409=CARTESIAN_POINT('Ctrl Pts',(63.2335483363939,-6.94425137989254,0.00364565552205904));
#29410=CARTESIAN_POINT('Ctrl Pts',(63.297162732284,-6.93717640596789,-2.20128821749584));
#29411=CARTESIAN_POINT('Ctrl Pts',(63.3607771281741,-5.79327512818524,-4.41796084971756));
#29412=CARTESIAN_POINT('Ctrl Pts',(63.4243915240642,-3.98649763460576,-5.6864840942668));
#29413=CARTESIAN_POINT('Ctrl Pts',(63.4905620588782,-2.10712062618958,-7.00597884606616));
#29414=CARTESIAN_POINT('Ctrl Pts',(63.5567325936923,0.489473938257958,-7.29959671410731));
#29415=CARTESIAN_POINT('Ctrl Pts',(63.6229031285063,2.61604017008766,-6.43308624017697));
#29416=CARTESIAN_POINT('Ctrl Pts',(63.6890736633204,4.74260640191736,-5.56657576624663));
#29417=CARTESIAN_POINT('Ctrl Pts',(63.7552441981344,6.39914430112923,-3.53993695034479));
#29418=CARTESIAN_POINT('Ctrl Pts',(63.8214147329484,6.82447958873384,-1.28709069678286));
#29419=CARTESIAN_POINT('Ctrl Pts',(63.8875852677624,7.24981487633844,0.965755556779008));
#29420=CARTESIAN_POINT('Ctrl Pts',(63.9537558025765,6.44394755233585,3.44480924800095));
#29421=CARTESIAN_POINT('Ctrl Pts',(64.0199263373905,4.78006004588273,5.03363316959887));
#29422=CARTESIAN_POINT('Ctrl Pts',(64.0530116047975,3.94811629265612,5.82804513039787));
#29423=CARTESIAN_POINT('Ctrl Pts',(64.0860968722045,2.90166749381685,6.39989964879084));
#29424=CARTESIAN_POINT('Ctrl Pts',(64.1191821396116,1.78470649325174,6.69567368292629));
#29425=CARTESIAN_POINT('Ctrl Pts',(64.1522674070186,0.667745492686632,6.99144771706174));
#29426=CARTESIAN_POINT('Ctrl Pts',(64.1853526744256,-0.519727709604317,
7.01114126693967));
#29427=CARTESIAN_POINT('Ctrl Pts',(64.2184379418327,-1.63657026372325,6.73995375130146));
#29428=CARTESIAN_POINT('Ctrl Pts',(64.2515232092397,-2.75341281784225,6.46876623566324));
#29429=CARTESIAN_POINT('Ctrl Pts',(64.2846084766467,-3.79962472378922,5.90669765450884));
#29430=CARTESIAN_POINT('Ctrl Pts',(64.3176937440537,-4.6565674166262,5.13162773685908));
#29431=CARTESIAN_POINT('Ctrl Pts',(64.3507790114607,-5.51351010946303,4.35655781920945));
#29432=CARTESIAN_POINT('Ctrl Pts',(64.3838642788677,-6.18118358918994,3.36848656506454));
#29433=CARTESIAN_POINT('Ctrl Pts',(64.4169495462748,-6.55617454016449,2.281011251009));
#29434=CARTESIAN_POINT('Ctrl Pts',(64.4391491429812,-6.80778646694058,1.55133561915753));
#29435=CARTESIAN_POINT('Ctrl Pts',(64.4613487396876,-6.92762805264689,0.776906694603623));
#29436=CARTESIAN_POINT('Ctrl Pts',(64.483548336394,-6.92250999810812,0.0016499903344943));
#29437=CARTESIAN_POINT('Origin',(29.75,0.,0.));
#29438=CARTESIAN_POINT('',(65.9128916636062,-6.92558145942544,-0.00361457160125256));
#29439=CARTESIAN_POINT('',(65.7335483363939,-6.933,-5.0499882053856E-12));
#29440=CARTESIAN_POINT('',(29.75,-6.933,-8.4904762584886E-16));
#29441=CARTESIAN_POINT('Ctrl Pts',(65.9128916636062,-6.92558145942544,-0.00361457160125256));
#29442=CARTESIAN_POINT('Ctrl Pts',(65.8724178529441,-6.91851212277228,1.41090647206241));
#29443=CARTESIAN_POINT('Ctrl Pts',(65.8319440422819,-6.49691708916176,2.82927471017481));
#29444=CARTESIAN_POINT('Ctrl Pts',(65.7914702316197,-5.69119674035493,3.97976687862786));
#29445=CARTESIAN_POINT('Ctrl Pts',(65.7252996968056,-4.37392649772603,5.86070373237007));
#29446=CARTESIAN_POINT('Ctrl Pts',(65.6591291619916,-2.02993151309655,7.02563729856908));
#29447=CARTESIAN_POINT('Ctrl Pts',(65.5929586271776,0.261110209086824,6.93988080424563));
#29448=CARTESIAN_POINT('Ctrl Pts',(65.5267880923635,2.55215193127013,6.85412430992217));
#29449=CARTESIAN_POINT('Ctrl Pts',(65.4606175575495,4.79024039100734,5.51767775507631));
#29450=CARTESIAN_POINT('Ctrl Pts',(65.3944470227355,5.96973620774678,3.54241253078668));
#29451=CARTESIAN_POINT('Ctrl Pts',(65.3613617553284,6.55948411611648,2.55477991864189));
#29452=CARTESIAN_POINT('Ctrl Pts',(65.3282764879214,6.88458386373675,1.40744263913616));
#29453=CARTESIAN_POINT('Ctrl Pts',(65.2951912205144,6.92483742193198,0.252685605335446));
#29454=CARTESIAN_POINT('Ctrl Pts',(65.2621059531074,6.96509098012721,-0.902071428465336));
#29455=CARTESIAN_POINT('Ctrl Pts',(65.2290206857003,6.72049834889736,-2.06424821656111));
#29456=CARTESIAN_POINT('Ctrl Pts',(65.1959354182933,6.20798328677723,-3.09294072184353));
#29457=CARTESIAN_POINT('Ctrl Pts',(65.1628501508863,5.69546822465709,-4.12163322712596));
#29458=CARTESIAN_POINT('Ctrl Pts',(65.1297648834793,4.91503073164666,-5.01684144959503));
#29459=CARTESIAN_POINT('Ctrl Pts',(65.0966796160723,3.96895981333477,-5.6801920157194));
#29460=CARTESIAN_POINT('Ctrl Pts',(65.0635943486653,3.02288889502287,-6.34354258184377));
#29461=CARTESIAN_POINT('Ctrl Pts',(65.0305090812582,1.91118455140951,-6.77503549162344));
#29462=CARTESIAN_POINT('Ctrl Pts',(64.9974238138512,0.767578614783853,-6.89907674971449));
#29463=CARTESIAN_POINT('Ctrl Pts',(64.9312532790372,-1.5196332584674,-7.14715926589657));
#29464=CARTESIAN_POINT('Ctrl Pts',(64.8650827442231,-3.93445150376781,-6.16543517532421));
#29465=CARTESIAN_POINT('Ctrl Pts',(64.7989122094091,-5.38275317063448,-4.38817643478656));
#29466=CARTESIAN_POINT('Ctrl Pts',(64.7535720274748,-6.37513235052187,-3.17039521438781));
#29467=CARTESIAN_POINT('Ctrl Pts',(64.7082318455406,-6.91373029289969,-1.57910907333059));
#29468=CARTESIAN_POINT('Ctrl Pts',(64.6628916636063,-6.9266679019854,0.00480994512238903));
#29469=CARTESIAN_POINT('Ctrl Pts',(64.4835483363939,-6.933,-5.39651656694673E-12));
#29470=CARTESIAN_POINT('Ctrl Pts',(64.540772531679,-6.93299999999845,-1.99420935702167));
#29471=CARTESIAN_POINT('Ctrl Pts',(64.5979967269641,-6.0230750262894,-3.97063309653513));
#29472=CARTESIAN_POINT('Ctrl Pts',(64.6552209222492,-4.50798484753575,-5.26731066241475));
#29473=CARTESIAN_POINT('Ctrl Pts',(64.7124451175343,-2.99289466878209,-6.56398822829437));
#29474=CARTESIAN_POINT('Ctrl Pts',(64.7696693128194,-0.899664345623224,
-7.1577904429248));
#29475=CARTESIAN_POINT('Ctrl Pts',(64.8268935081045,1.07062371682378,-6.84983604599223));
#29476=CARTESIAN_POINT('Ctrl Pts',(64.8841177033896,3.04091177927078,-6.54188164905966));
#29477=CARTESIAN_POINT('Ctrl Pts',(64.9413418986747,4.85311303640296,-5.33766370386023));
#29478=CARTESIAN_POINT('Ctrl Pts',(64.9985660939598,5.90026971494045,-3.64050907030275));
#29479=CARTESIAN_POINT('Ctrl Pts',(65.0557902892449,6.94742639347793,-1.94335443674527));
#29480=CARTESIAN_POINT('Ctrl Pts',(65.11301448453,7.21086008527493,0.216464293129524));
#29481=CARTESIAN_POINT('Ctrl Pts',(65.1702386798151,6.60233935005918,2.1155623617989));
#29482=CARTESIAN_POINT('Ctrl Pts',(65.2274628751002,5.99381861484343,4.01466043046827));
#29483=CARTESIAN_POINT('Ctrl Pts',(65.2846870703853,4.5241977964686,5.61916312790792));
#29484=CARTESIAN_POINT('Ctrl Pts',(65.3419112656703,2.68569472999908,6.39167683923829));
#29485=CARTESIAN_POINT('Ctrl Pts',(65.3991354609554,0.847191663529553,7.16419055056866));
#29486=CARTESIAN_POINT('Ctrl Pts',(65.4563596562406,-1.32739978994719,7.09093574623684));
#29487=CARTESIAN_POINT('Ctrl Pts',(65.5135838515256,-3.1097470673667,6.19644754492477));
#29488=CARTESIAN_POINT('Ctrl Pts',(65.5708080468107,-4.89209434478622,5.30195934361269));
#29489=CARTESIAN_POINT('Ctrl Pts',(65.6280322420958,-6.25040525058933,3.60219296582188));
#29490=CARTESIAN_POINT('Ctrl Pts',(65.6852564373809,-6.72974280712892,1.66644854402908));
#29491=CARTESIAN_POINT('Ctrl Pts',(65.7013537370519,-6.86458158035656,1.1219191209622));
#29492=CARTESIAN_POINT('Ctrl Pts',(65.7174510367229,-6.93300000000039,0.560975745773053));
#29493=CARTESIAN_POINT('Ctrl Pts',(65.7335483363939,-6.933,-4.85292361851464E-12));
#29494=CARTESIAN_POINT('Origin',(29.75,0.,0.));
#29495=CARTESIAN_POINT('',(67.1628916636063,-6.94182785481333,-0.00394764471083664));
#29496=CARTESIAN_POINT('',(66.9835483363939,-6.933,-4.50639525695351E-12));
#29497=CARTESIAN_POINT('',(29.75,-6.933,-8.4904762584886E-16));
#29498=CARTESIAN_POINT('Ctrl Pts',(67.1628916636063,-6.94182785481333,-0.00394764471083664));
#29499=CARTESIAN_POINT('Ctrl Pts',(67.1027743951617,-6.92719609612228,2.08459150757714));
#29500=CARTESIAN_POINT('Ctrl Pts',(67.042657126717,-5.92001797146785,4.18526716644349));
#29501=CARTESIAN_POINT('Ctrl Pts',(66.9825398582723,-4.27990668625507,5.4692342224079));
#29502=CARTESIAN_POINT('Ctrl Pts',(66.9163693234583,-2.47465099675213,6.88248517300629));
#29503=CARTESIAN_POINT('Ctrl Pts',(66.8501987886443,0.0974162692902572,
7.30627680879808));
#29504=CARTESIAN_POINT('Ctrl Pts',(66.7840282538302,2.27325271597746,6.55886872652768));
#29505=CARTESIAN_POINT('Ctrl Pts',(66.7509429864232,3.36117093932118,6.18516468539243));
#29506=CARTESIAN_POINT('Ctrl Pts',(66.7178577190162,4.35003145782598,5.51866071474172));
#29507=CARTESIAN_POINT('Ctrl Pts',(66.6847724516092,5.12611472467068,4.66263564681462));
#29508=CARTESIAN_POINT('Ctrl Pts',(66.6516871842021,5.90219799151526,3.80661057888767));
#29509=CARTESIAN_POINT('Ctrl Pts',(66.6186019167951,6.46550400669962,2.76106441368453));
#29510=CARTESIAN_POINT('Ctrl Pts',(66.5855166493881,6.738012725561,1.64454349610523));
#29511=CARTESIAN_POINT('Ctrl Pts',(66.5524313819811,7.01052144442241,0.528022578525872));
#29512=CARTESIAN_POINT('Ctrl Pts',(66.519346114574,6.99223286696077,-0.659473091429799));
#29513=CARTESIAN_POINT('Ctrl Pts',(66.486260847167,6.69778057245195,-1.77678325488286));
#29514=CARTESIAN_POINT('Ctrl Pts',(66.45317557976,6.40332827794312,-2.89409341833599));
#29515=CARTESIAN_POINT('Ctrl Pts',(66.420090312353,5.8327122663871,-3.94121807528664));
#29516=CARTESIAN_POINT('Ctrl Pts',(66.387005044946,5.03928517632311,-4.77410115534899));
#29517=CARTESIAN_POINT('Ctrl Pts',(66.320834510132,3.45243099619514,-6.43986731547369));
#29518=CARTESIAN_POINT('Ctrl Pts',(66.2546639753179,0.974332502035366,-7.24866716804506));
#29519=CARTESIAN_POINT('Ctrl Pts',(66.1884934405039,-1.27901541039728,-6.82599763384204));
#29520=CARTESIAN_POINT('Ctrl Pts',(66.1223229056898,-3.5323633228298,-6.40332809963903));
#29521=CARTESIAN_POINT('Ctrl Pts',(66.0561523708758,-5.56096065353515,-4.74918917866183));
#29522=CARTESIAN_POINT('Ctrl Pts',(65.9899818360618,-6.42998656857364,-2.62364964753062));
#29523=CARTESIAN_POINT('Ctrl Pts',(65.9642851119099,-6.76746486283719,-1.79821574165669));
#29524=CARTESIAN_POINT('Ctrl Pts',(65.9385883877581,-6.93006976410791,-0.901690548913561));
#29525=CARTESIAN_POINT('Ctrl Pts',(65.9128916636062,-6.92558145942544,-0.00361457160125256));
#29526=CARTESIAN_POINT('Ctrl Pts',(65.7335483363939,-6.93201917574831,-0.00104661053196153));
#29527=CARTESIAN_POINT('Ctrl Pts',(65.7578758167191,-6.93536664097712,-0.850911801504528));
#29528=CARTESIAN_POINT('Ctrl Pts',(65.7822032970444,-6.78541196678331,-1.70071837762845));
#29529=CARTESIAN_POINT('Ctrl Pts',(65.8065307773696,-6.47990263081343,-2.48943745121956));
#29530=CARTESIAN_POINT('Ctrl Pts',(65.8727013121836,-5.64891989517595,-4.63474646883597));
#29531=CARTESIAN_POINT('Ctrl Pts',(65.9388718469976,-3.66708891267972,-6.32810859915136));
#29532=CARTESIAN_POINT('Ctrl Pts',(66.0050423818116,-1.42299593951584,-6.79744118581012));
#29533=CARTESIAN_POINT('Ctrl Pts',(66.0712129166256,0.821097033647975,-7.26677377246886));
#29534=CARTESIAN_POINT('Ctrl Pts',(66.1373834514397,3.32745199747944,-6.51207681547106));
#29535=CARTESIAN_POINT('Ctrl Pts',(66.2035539862538,4.94192445361747,-4.87910313893728));
#29536=CARTESIAN_POINT('Ctrl Pts',(66.2697245210678,6.55639690975559,-3.24612946240341));
#29537=CARTESIAN_POINT('Ctrl Pts',(66.3358950558818,7.27898685820016,-0.734879066333458));
#29538=CARTESIAN_POINT('Ctrl Pts',(66.4020655906958,6.77930311774462,1.50642423731264));
#29539=CARTESIAN_POINT('Ctrl Pts',(66.4682361255099,6.2796193772891,3.74772754095867));
#29540=CARTESIAN_POINT('Ctrl Pts',(66.534406660324,4.55766194793354,5.71908375218086));
#29541=CARTESIAN_POINT('Ctrl Pts',(66.600577195138,2.40731390636405,6.51421245228286));
#29542=CARTESIAN_POINT('Ctrl Pts',(66.666747729952,0.256965864794573,7.30934115238486));
#29543=CARTESIAN_POINT('Ctrl Pts',(66.7329182647661,-2.32177278898883,6.92824234136667));
#29544=CARTESIAN_POINT('Ctrl Pts',(66.7990887995801,-4.16586038519456,5.55266099999641));
#29545=CARTESIAN_POINT('Ctrl Pts',(66.8321740669871,-5.08790418329745,4.86487032931126));
#29546=CARTESIAN_POINT('Ctrl Pts',(66.8652593343941,-5.82628521700591,3.92845902603808));
#29547=CARTESIAN_POINT('Ctrl Pts',(66.8983446018012,-6.3042136615862,2.87647587172514));
#29548=CARTESIAN_POINT('Ctrl Pts',(66.9267458466654,-6.71447973606366,1.97342646332384));
#29549=CARTESIAN_POINT('Ctrl Pts',(66.9551470915296,-6.93281966865977,0.98521276627255));
#29550=CARTESIAN_POINT('Ctrl Pts',(66.9835483363939,-6.93511079172564,-0.00169474912669407));
#29551=CARTESIAN_POINT('Origin',(29.75,0.,0.));
#29552=CARTESIAN_POINT('',(68.4128916636063,-6.93357857970305,0.00297544388368854));
#29553=CARTESIAN_POINT('',(68.2335483363939,-6.933,-4.7509218781272E-12));
#29554=CARTESIAN_POINT('',(29.75,-6.933,-8.4904762584886E-16));
#29555=CARTESIAN_POINT('Ctrl Pts',(68.4128916636063,-6.93473393447276,0.0089170509982972));
#29556=CARTESIAN_POINT('Ctrl Pts',(68.3993014721933,-6.93916860973486,0.481932871115519));
#29557=CARTESIAN_POINT('Ctrl Pts',(68.3857112807802,-6.89496607960317,0.95394242452496));
#29558=CARTESIAN_POINT('Ctrl Pts',(68.3721210893672,-6.79911921480736,1.41495069786618));
#29559=CARTESIAN_POINT('Ctrl Pts',(68.3059505545531,-6.33244158599193,3.65959634512357));
#29560=CARTESIAN_POINT('Ctrl Pts',(68.239780019739,-4.6414273666631,5.643433719458));
#29561=CARTESIAN_POINT('Ctrl Pts',(68.173609484925,-2.49710289781263,6.47695380660065));
#29562=CARTESIAN_POINT('Ctrl Pts',(68.140524217518,-1.42494066338746,6.89371385017195));
#29563=CARTESIAN_POINT('Ctrl Pts',(68.107438950111,-0.239450866581887,7.02289457194535));
#29564=CARTESIAN_POINT('Ctrl Pts',(68.074353682704,0.905844897653366,6.86998260787669));
#29565=CARTESIAN_POINT('Ctrl Pts',(68.041268415297,2.05114066188868,6.71707064380802));
#29566=CARTESIAN_POINT('Ctrl Pts',(68.0081831478899,3.15624239355368,6.28206599389726));
#29567=CARTESIAN_POINT('Ctrl Pts',(67.9750978804829,4.08504323520468,5.60515498849634));
#29568=CARTESIAN_POINT('Ctrl Pts',(67.9420126130759,5.01384407685567,4.92824398309542));
#29569=CARTESIAN_POINT('Ctrl Pts',(67.9089273456688,5.76634402849265,4.00942662220434));
#29570=CARTESIAN_POINT('Ctrl Pts',(67.8758420782618,6.26260800157698,2.96596768737957));
#29571=CARTESIAN_POINT('Ctrl Pts',(67.8427568108548,6.75887197466129,1.92250875255486));
#29572=CARTESIAN_POINT('Ctrl Pts',(67.8096715434478,6.99889996919296,0.754408243796477));
#29573=CARTESIAN_POINT('Ctrl Pts',(67.7765862760408,6.93046212332443,-0.39386735146852));
#29574=CARTESIAN_POINT('Ctrl Pts',(67.7104157412267,6.79358643158735,-2.69041854199858));
#29575=CARTESIAN_POINT('Ctrl Pts',(67.6442452064128,5.42284737824935,-4.9076700785551));
#29576=CARTESIAN_POINT('Ctrl Pts',(67.5780746715987,3.42892195617063,-6.03925647982234));
#29577=CARTESIAN_POINT('Ctrl Pts',(67.5119041367847,1.43499653409197,-7.17084288108956));
#29578=CARTESIAN_POINT('Ctrl Pts',(67.4457336019706,-1.18211525672738,-7.21676414706757));
#29579=CARTESIAN_POINT('Ctrl Pts',(67.3795630671565,-3.21780841116017,-6.15418342104918));
#29580=CARTESIAN_POINT('Ctrl Pts',(67.3133925323425,-5.25350156559306,-5.09160269503072));
#29581=CARTESIAN_POINT('Ctrl Pts',(67.2472219975285,-6.7077760836393,-2.92051997701569));
#29582=CARTESIAN_POINT('Ctrl Pts',(67.1810514627145,-6.91569128618054,-0.633623485305609));
#29583=CARTESIAN_POINT('Ctrl Pts',(67.1749981963451,-6.93471132443119,-0.424418683463479));
#29584=CARTESIAN_POINT('Ctrl Pts',(67.1689449299757,-6.94330114086077,-0.214244688119485));
#29585=CARTESIAN_POINT('Ctrl Pts',(67.1628916636063,-6.94182785481333,-0.00394764471083664));
#29586=CARTESIAN_POINT('Ctrl Pts',(66.9835483363939,-6.933,-4.50639525695351E-12));
#29587=CARTESIAN_POINT('Ctrl Pts',(67.040772531679,-6.9329999999987,-1.99420935702078));
#29588=CARTESIAN_POINT('Ctrl Pts',(67.0979967269641,-6.02307502628991,-3.97063309653436));
#29589=CARTESIAN_POINT('Ctrl Pts',(67.1552209222492,-4.50798484753642,-5.26731066241417));
#29590=CARTESIAN_POINT('Ctrl Pts',(67.2124451175343,-2.99289466878293,-6.56398822829398));
#29591=CARTESIAN_POINT('Ctrl Pts',(67.2696693128194,-0.899664345624143,
-7.15779044292469));
#29592=CARTESIAN_POINT('Ctrl Pts',(67.3268935081045,1.0706237168229,-6.84983604599237));
#29593=CARTESIAN_POINT('Ctrl Pts',(67.3841177033896,3.04091177926994,-6.54188164906005));
#29594=CARTESIAN_POINT('Ctrl Pts',(67.4413418986747,4.85311303640228,-5.33766370386085));
#29595=CARTESIAN_POINT('Ctrl Pts',(67.4985660939598,5.90026971493998,-3.64050907030351));
#29596=CARTESIAN_POINT('Ctrl Pts',(67.5557902892448,6.94742639347768,-1.94335443674616));
#29597=CARTESIAN_POINT('Ctrl Pts',(67.6130144845299,7.21086008527496,0.216464293128598));
#29598=CARTESIAN_POINT('Ctrl Pts',(67.670238679815,6.60233935005945,2.11556236179805));
#29599=CARTESIAN_POINT('Ctrl Pts',(67.7274628751001,5.99381861484394,4.0146604304675));
#29600=CARTESIAN_POINT('Ctrl Pts',(67.7846870703852,4.52419779646933,5.61916312790734));
#29601=CARTESIAN_POINT('Ctrl Pts',(67.8419112656703,2.6856947299999,6.39167683923795));
#29602=CARTESIAN_POINT('Ctrl Pts',(67.8991354609554,0.847191663530473,7.16419055056855));
#29603=CARTESIAN_POINT('Ctrl Pts',(67.9563596562405,-1.32739978994628,7.09093574623701));
#29604=CARTESIAN_POINT('Ctrl Pts',(68.0135838515256,-3.10974706736591,6.19644754492517));
#29605=CARTESIAN_POINT('Ctrl Pts',(68.0708080468107,-4.89209434478554,5.30195934361332));
#29606=CARTESIAN_POINT('Ctrl Pts',(68.1280322420958,-6.25040525058887,3.60219296582268));
#29607=CARTESIAN_POINT('Ctrl Pts',(68.1852564373809,-6.7297428071287,1.66644854402994));
#29608=CARTESIAN_POINT('Ctrl Pts',(68.2013537370519,-6.86458158035646,1.12191912096289));
#29609=CARTESIAN_POINT('Ctrl Pts',(68.2174510367229,-6.93300000000037,0.560975745773549));
#29610=CARTESIAN_POINT('Ctrl Pts',(68.2335483363939,-6.933,-4.55399606913431E-12));
#29611=CARTESIAN_POINT('Origin',(29.75,0.,0.));
#29612=CARTESIAN_POINT('',(69.6628916636063,-6.92775586673719,-0.00132508185730362));
#29613=CARTESIAN_POINT('',(69.4835483363939,-6.92774438460107,0.00106183211813038));
#29614=CARTESIAN_POINT('',(29.75,-6.933,-8.4904762584886E-16));
#29615=CARTESIAN_POINT('Ctrl Pts',(69.6628916636063,-6.933,8.80129302771593E-13));
#29616=CARTESIAN_POINT('Ctrl Pts',(69.6056674683212,-6.93299999999975,1.99420935701716));
#29617=CARTESIAN_POINT('Ctrl Pts',(69.5484432730361,-6.02307502629199,3.97063309653121));
#29618=CARTESIAN_POINT('Ctrl Pts',(69.491219077751,-4.50798484753918,5.26731066241181));
#29619=CARTESIAN_POINT('Ctrl Pts',(69.4339948824659,-2.99289466878637,6.56398822829242));
#29620=CARTESIAN_POINT('Ctrl Pts',(69.3767706871808,-0.899664345627887,
7.15779044292421));
#29621=CARTESIAN_POINT('Ctrl Pts',(69.3195464918957,1.07062371681932,6.84983604599292));
#29622=CARTESIAN_POINT('Ctrl Pts',(69.2623222966106,3.04091177926652,6.54188164906164));
#29623=CARTESIAN_POINT('Ctrl Pts',(69.2050981013255,4.85311303639948,5.33766370386339));
#29624=CARTESIAN_POINT('Ctrl Pts',(69.1478739060404,5.90026971493807,3.64050907030659));
#29625=CARTESIAN_POINT('Ctrl Pts',(69.0906497107553,6.94742639347666,1.9433544367498));
#29626=CARTESIAN_POINT('Ctrl Pts',(69.0334255154702,7.21086008527507,-0.216464293124826));
#29627=CARTESIAN_POINT('Ctrl Pts',(68.9762013201851,6.60233935006056,-2.1155623617946));
#29628=CARTESIAN_POINT('Ctrl Pts',(68.9189771249,5.99381861484604,-4.01466043046437));
#29629=CARTESIAN_POINT('Ctrl Pts',(68.8617529296149,4.52419779647226,-5.61916312790497));
#29630=CARTESIAN_POINT('Ctrl Pts',(68.8045287343298,2.68569473000324,-6.39167683923654));
#29631=CARTESIAN_POINT('Ctrl Pts',(68.7473045390447,0.84719166353422,-7.16419055056811));
#29632=CARTESIAN_POINT('Ctrl Pts',(68.6900803437596,-1.32739978994257,-7.09093574623771));
#29633=CARTESIAN_POINT('Ctrl Pts',(68.6328561484745,-3.10974706736267,-6.19644754492679));
#29634=CARTESIAN_POINT('Ctrl Pts',(68.5756319531894,-4.89209434478277,-5.30195934361588));
#29635=CARTESIAN_POINT('Ctrl Pts',(68.5184077579043,-6.25040525058698,-3.60219296582595));
#29636=CARTESIAN_POINT('Ctrl Pts',(68.4611835626193,-6.72974280712783,-1.66644854403346));
#29637=CARTESIAN_POINT('Ctrl Pts',(68.4450862629483,-6.86458158035586,-1.12191912096655));
#29638=CARTESIAN_POINT('Ctrl Pts',(68.4289889632773,-6.93300000000006,-0.560975745777307));
#29639=CARTESIAN_POINT('Ctrl Pts',(68.4128916636063,-6.933,7.30526750203353E-13));
#29640=CARTESIAN_POINT('Ctrl Pts',(68.2335483363939,-6.933,-4.55399606913431E-12));
#29641=CARTESIAN_POINT('Ctrl Pts',(68.290772531679,-6.93299999999869,-1.99420935702096));
#29642=CARTESIAN_POINT('Ctrl Pts',(68.3479967269641,-6.02307502628976,-3.97063309653466));
#29643=CARTESIAN_POINT('Ctrl Pts',(68.4052209222492,-4.50798484753609,-5.26731066241446));
#29644=CARTESIAN_POINT('Ctrl Pts',(68.4624451175343,-2.99289466878242,-6.56398822829426));
#29645=CARTESIAN_POINT('Ctrl Pts',(68.5196693128194,-0.89966434562341,-7.15779044292481));
#29646=CARTESIAN_POINT('Ctrl Pts',(68.5768935081045,1.07062371682373,-6.84983604599224));
#29647=CARTESIAN_POINT('Ctrl Pts',(68.6341177033896,3.04091177927086,-6.54188164905966));
#29648=CARTESIAN_POINT('Ctrl Pts',(68.6913418986747,4.85311303640315,-5.3376637038601));
#29649=CARTESIAN_POINT('Ctrl Pts',(68.7485660939598,5.90026971494062,-3.64050907030246));
#29650=CARTESIAN_POINT('Ctrl Pts',(68.8057902892449,6.94742639347809,-1.94335443674482));
#29651=CARTESIAN_POINT('Ctrl Pts',(68.86301448453,7.21086008527495,0.216464293130162));
#29652=CARTESIAN_POINT('Ctrl Pts',(68.9202386798151,6.60233935005896,2.1155623617996));
#29653=CARTESIAN_POINT('Ctrl Pts',(68.9774628751002,5.99381861484296,4.01466043046903));
#29654=CARTESIAN_POINT('Ctrl Pts',(69.0346870703853,4.52419779646781,5.6191631279086));
#29655=CARTESIAN_POINT('Ctrl Pts',(69.0919112656704,2.68569472999804,6.39167683923873));
#29656=CARTESIAN_POINT('Ctrl Pts',(69.1491354609555,0.847191663528267,7.16419055056885));
#29657=CARTESIAN_POINT('Ctrl Pts',(69.2063596562406,-1.32739978994863,7.09093574623661));
#29658=CARTESIAN_POINT('Ctrl Pts',(69.2635838515257,-3.10974706736806,6.19644754492409));
#29659=CARTESIAN_POINT('Ctrl Pts',(69.3208080468108,-4.8920943447875,5.30195934361156));
#29660=CARTESIAN_POINT('Ctrl Pts',(69.3780322420959,-6.25040525059029,3.60219296582028));
#29661=CARTESIAN_POINT('Ctrl Pts',(69.435256437381,-6.72974280712937,1.66644854402722));
#29662=CARTESIAN_POINT('Ctrl Pts',(69.451353737052,-6.86458158035667,1.12191912096107));
#29663=CARTESIAN_POINT('Ctrl Pts',(69.4674510367229,-6.93300000000036,0.560975745772714));
#29664=CARTESIAN_POINT('Ctrl Pts',(69.4835483363939,-6.933,-4.40453229444415E-12));
#29665=CARTESIAN_POINT('Origin',(29.75,0.,0.));
#29666=CARTESIAN_POINT('',(70.9128916636062,-6.93600788003209,-0.00402363236026881));
#29667=CARTESIAN_POINT('',(70.7335483363939,-6.93748346162273,-0.00501519726878595));
#29668=CARTESIAN_POINT('',(29.75,-6.933,-8.4904762584886E-16));
#29669=CARTESIAN_POINT('Ctrl Pts',(70.9128916636062,-6.93600788003209,-0.00402363236026881));
#29670=CARTESIAN_POINT('Ctrl Pts',(70.8930998240354,-6.93185358698644,0.684973550004836));
#29671=CARTESIAN_POINT('Ctrl Pts',(70.8733079844645,-6.82435975372044,1.37546389076954));
#29672=CARTESIAN_POINT('Ctrl Pts',(70.8535161448936,-6.62104360085322,2.03665129400251));
#29673=CARTESIAN_POINT('Ctrl Pts',(70.8204308774865,-6.28116770090578,3.14193319383502));
#29674=CARTESIAN_POINT('Ctrl Pts',(70.7873456100795,-5.67352073095605,4.16532938092614));
#29675=CARTESIAN_POINT('Ctrl Pts',(70.7542603426724,-4.85002858812791,4.96638979919627));
#29676=CARTESIAN_POINT('Ctrl Pts',(70.6880898078583,-3.20304430247158,6.5685106357366));
#29677=CARTESIAN_POINT('Ctrl Pts',(70.6219192730444,-0.692679325301471,
7.28128839699305));
#29678=CARTESIAN_POINT('Ctrl Pts',(70.5557487382303,1.54387781336133,6.77133000678115));
#29679=CARTESIAN_POINT('Ctrl Pts',(70.4895782034163,3.7804349520242,6.26137161656925));
#29680=CARTESIAN_POINT('Ctrl Pts',(70.4234076686023,5.74318425217982,4.52867707488891));
#29681=CARTESIAN_POINT('Ctrl Pts',(70.3572371337882,6.52768685308951,2.37106409472671));
#29682=CARTESIAN_POINT('Ctrl Pts',(70.2910665989742,7.31218945399919,0.213451114564565));
#29683=CARTESIAN_POINT('Ctrl Pts',(70.2248960641602,6.91844535566313,-2.36908030407929));
#29684=CARTESIAN_POINT('Ctrl Pts',(70.1587255293462,5.53062392128402,-4.1977203057812));
#29685=CARTESIAN_POINT('Ctrl Pts',(70.0925549945321,4.1428024869049,-6.02636030748311));
#29686=CARTESIAN_POINT('Ctrl Pts',(70.026384459718,1.76090371648268,-7.10110889224293));
#29687=CARTESIAN_POINT('Ctrl Pts',(69.960213924904,-0.528348580108324,-6.92532263247645));
#29688=CARTESIAN_POINT('Ctrl Pts',(69.89404339009,-2.81760087669933,-6.74953637270997));
#29689=CARTESIAN_POINT('Ctrl Pts',(69.8278728552759,-5.0142066994592,-5.32321526841718));
#29690=CARTESIAN_POINT('Ctrl Pts',(69.7617023204619,-6.10668716247187,-3.30725649205025));
#29691=CARTESIAN_POINT('Ctrl Pts',(69.7287654348434,-6.65047759958824,-2.30379771972032));
#29692=CARTESIAN_POINT('Ctrl Pts',(69.6958285492248,-6.92070705183615,-1.15424877668268));
#29693=CARTESIAN_POINT('Ctrl Pts',(69.6628916636063,-6.91934367692504,-0.00345066477998368));
#29694=CARTESIAN_POINT('Ctrl Pts',(69.4835483363939,-6.91910824403556,0.00280665757405688));
#29695=CARTESIAN_POINT('Ctrl Pts',(69.5151159781859,-6.91929278287084,-1.10048129744765));
#29696=CARTESIAN_POINT('Ctrl Pts',(69.5466836199778,-6.67002846877592,-2.20446988795717));
#29697=CARTESIAN_POINT('Ctrl Pts',(69.5782512617697,-6.16970630690116,-3.18137335378403));
#29698=CARTESIAN_POINT('Ctrl Pts',(69.6113365291767,-5.64533097901331,-4.20524180144227));
#29699=CARTESIAN_POINT('Ctrl Pts',(69.6444217965837,-4.84517815766031,-5.08951207500788));
#29700=CARTESIAN_POINT('Ctrl Pts',(69.6775070639907,-3.88765338934523,-5.73617004499287));
#29701=CARTESIAN_POINT('Ctrl Pts',(69.7105923313977,-2.93012862103014,-6.38282801497786));
#29702=CARTESIAN_POINT('Ctrl Pts',(69.7436775988048,-1.81523190575297,-6.79187368138223));
#29703=CARTESIAN_POINT('Ctrl Pts',(69.7767628662118,-0.671317570116662,
-6.90316829378146));
#29704=CARTESIAN_POINT('Ctrl Pts',(69.8098481336188,0.472596765519775,-7.0144629061807));
#29705=CARTESIAN_POINT('Ctrl Pts',(69.8429334010258,1.64552872151536,-6.82800646457471));
#29706=CARTESIAN_POINT('Ctrl Pts',(69.8760186684328,2.70970252414811,-6.37785070657828));
#29707=CARTESIAN_POINT('Ctrl Pts',(69.9091039358398,3.77387632678074,-5.9276949485819));
#29708=CARTESIAN_POINT('Ctrl Pts',(69.9421892032469,4.72929197605057,-5.21383987419512));
#29709=CARTESIAN_POINT('Ctrl Pts',(69.9752744706539,5.44108660062344,-4.31016536153499));
#29710=CARTESIAN_POINT('Ctrl Pts',(70.0414450054679,6.86467584976921,-2.50281633621466));
#29711=CARTESIAN_POINT('Ctrl Pts',(70.1076155402819,7.3137810001271,0.0638104421991439));
#29712=CARTESIAN_POINT('Ctrl Pts',(70.173786075096,6.57541224839079,2.23462018433102));
#29713=CARTESIAN_POINT('Ctrl Pts',(70.23995660991,5.83704349665449,4.40542992646289));
#29714=CARTESIAN_POINT('Ctrl Pts',(70.3061271447241,3.91120084282398,6.18042263231284));
#29715=CARTESIAN_POINT('Ctrl Pts',(70.3722976795381,1.68399291891217,6.73820552039241));
#29716=CARTESIAN_POINT('Ctrl Pts',(70.4384682143522,-0.543215004999702,
7.29598840847199));
#29717=CARTESIAN_POINT('Ctrl Pts',(70.5046387491662,-3.0717881989929,6.63656147878113));
#29718=CARTESIAN_POINT('Ctrl Pts',(70.5708092839802,-4.74702605841882,5.06699124973978));
#29719=CARTESIAN_POINT('Ctrl Pts',(70.6250556347848,-6.12037963427992,3.780263592237));
#29720=CARTESIAN_POINT('Ctrl Pts',(70.6793019855893,-6.92023575397323,1.88185979080618));
#29721=CARTESIAN_POINT('Ctrl Pts',(70.7335483363939,-6.93748346162273,-0.00501519726878595));
#29722=CARTESIAN_POINT('Origin',(29.75,0.,0.));
#29723=CARTESIAN_POINT('',(72.1628916636062,-6.94192775449039,0.00618195413371575));
#29724=CARTESIAN_POINT('',(71.9835483363939,-6.9401949188535,0.00210382873980236));
#29725=CARTESIAN_POINT('',(29.75,-6.933,-8.4904762584886E-16));
#29726=CARTESIAN_POINT('Ctrl Pts',(72.1628916636062,-6.94192775449039,0.00618195413371575));
#29727=CARTESIAN_POINT('Ctrl Pts',(72.1565416336599,-6.94340649393155,0.226523173955462));
#29728=CARTESIAN_POINT('Ctrl Pts',(72.1501916037136,-6.93383229160786,0.446685249002146));
#29729=CARTESIAN_POINT('Ctrl Pts',(72.1438415737672,-6.91278923537634,0.665688012065615));
#29730=CARTESIAN_POINT('Ctrl Pts',(72.0776710389532,-6.69350990965197,2.94780795167749));
#29731=CARTESIAN_POINT('Ctrl Pts',(72.0115005041392,-5.22886240848834,5.10404170763851));
#29732=CARTESIAN_POINT('Ctrl Pts',(71.9453299693251,-3.18799897027634,6.16629140109333));
#29733=CARTESIAN_POINT('Ctrl Pts',(71.9122447019181,-2.16756725117023,6.69741624782081));
#29734=CARTESIAN_POINT('Ctrl Pts',(71.8791594345111,-1.00308154780201,6.95504507892165));
#29735=CARTESIAN_POINT('Ctrl Pts',(71.8460741671041,0.151959897059239,6.92780658346952));
#29736=CARTESIAN_POINT('Ctrl Pts',(71.8129888996971,1.30700134192036,6.90056808801738));
#29737=CARTESIAN_POINT('Ctrl Pts',(71.7799036322901,2.45259852827447,6.58846226601233));
#29738=CARTESIAN_POINT('Ctrl Pts',(71.7468183648831,3.4497814268547,6.01683565816965));
#29739=CARTESIAN_POINT('Ctrl Pts',(71.713733097476,4.44696432543494,5.44520905032697));
#29740=CARTESIAN_POINT('Ctrl Pts',(71.680647830069,5.29573293624125,4.61406165664668));
#29741=CARTESIAN_POINT('Ctrl Pts',(71.6475625626619,5.90256931486079,3.63083473489497));
#29742=CARTESIAN_POINT('Ctrl Pts',(71.6144772952549,6.50940569348037,2.64760781314321));
#29743=CARTESIAN_POINT('Ctrl Pts',(71.5813920278479,6.87430983991314,1.51230136332004));
#29744=CARTESIAN_POINT('Ctrl Pts',(71.5483067604409,6.93129030217091,0.363370212588453));
#29745=CARTESIAN_POINT('Ctrl Pts',(71.4821362256269,7.04525122668644,-1.93449208887466));
#29746=CARTESIAN_POINT('Ctrl Pts',(71.4159656908128,5.92751741450193,-4.28685319397145));
#29747=CARTESIAN_POINT('Ctrl Pts',(71.3497951559988,4.06794409821576,-5.62922334413628));
#29748=CARTESIAN_POINT('Ctrl Pts',(71.2836246211847,2.20837078192963,-6.97159349430107));
#29749=CARTESIAN_POINT('Ctrl Pts',(71.2174540863708,-0.393042038458098,
-7.30397268953411));
#29750=CARTESIAN_POINT('Ctrl Pts',(71.1512835515567,-2.53030427501,-6.46891859890768));
#29751=CARTESIAN_POINT('Ctrl Pts',(71.0851130167427,-4.66756651156202,-5.63386450828119));
#29752=CARTESIAN_POINT('Ctrl Pts',(71.0189424819285,-6.34067816427811,-3.63137713179512));
#29753=CARTESIAN_POINT('Ctrl Pts',(70.9527719471145,-6.8022422752566,-1.38099118953441));
#29754=CARTESIAN_POINT('Ctrl Pts',(70.9394785192785,-6.89496888262458,-0.928896564473384));
#29755=CARTESIAN_POINT('Ctrl Pts',(70.9261850914423,-6.9387981610777,-0.466796902638633));
#29756=CARTESIAN_POINT('Ctrl Pts',(70.9128916636062,-6.93600788003209,-0.00402363236026881));
#29757=CARTESIAN_POINT('Ctrl Pts',(70.7335483363939,-6.93748346162273,-0.00501519726878595));
#29758=CARTESIAN_POINT('Ctrl Pts',(70.7454725204034,-6.94127477360416,-0.419779402178013));
#29759=CARTESIAN_POINT('Ctrl Pts',(70.7573967044129,-6.90725137386348,-0.833986548478055));
#29760=CARTESIAN_POINT('Ctrl Pts',(70.7693208884224,-6.83319224883801,-1.24101743892661));
#29761=CARTESIAN_POINT('Ctrl Pts',(70.8354914232364,-6.42221805497271,-3.49974237015994));
#29762=CARTESIAN_POINT('Ctrl Pts',(70.9016619580505,-4.7783671423835,-5.53747870423487));
#29763=CARTESIAN_POINT('Ctrl Pts',(70.9678324928645,-2.65923204405885,-6.41583616523792));
#29764=CARTESIAN_POINT('Ctrl Pts',(71.0340030276785,-0.540096945734205,
-7.29419362624096));
#29765=CARTESIAN_POINT('Ctrl Pts',(71.1001735624925,2.05432233832609,-7.01317221417207));
#29766=CARTESIAN_POINT('Ctrl Pts',(71.1663440973065,3.94699624409178,-5.71043129652606));
#29767=CARTESIAN_POINT('Ctrl Pts',(71.1994293647136,4.89333319697466,-5.05906083770303));
#29768=CARTESIAN_POINT('Ctrl Pts',(71.2325146321206,5.66423380528383,-4.15226050248588));
#29769=CARTESIAN_POINT('Ctrl Pts',(71.2655998995276,6.18492037000725,-3.11976391325222));
#29770=CARTESIAN_POINT('Ctrl Pts',(71.2986851669347,6.70560693473067,-2.08726732401856));
#29771=CARTESIAN_POINT('Ctrl Pts',(71.3317704343417,6.9760794558682,-0.929074480768539));
#29772=CARTESIAN_POINT('Ctrl Pts',(71.3648557017487,6.9375587400496,0.218895786211316));
#29773=CARTESIAN_POINT('Ctrl Pts',(71.4310262365627,6.86051730841241,2.51483632017089));
#29774=CARTESIAN_POINT('Ctrl Pts',(71.4971967713767,5.5475029289509,4.76988654904982));
#29775=CARTESIAN_POINT('Ctrl Pts',(71.5633673061908,3.58085398574065,5.95204437955841));
#29776=CARTESIAN_POINT('Ctrl Pts',(71.6295378410048,1.61420504253036,7.13420221006703));
#29777=CARTESIAN_POINT('Ctrl Pts',(71.6957083758188,-1.00607846442871,7.24346764220525));
#29778=CARTESIAN_POINT('Ctrl Pts',(71.7618789106329,-3.06469476610544,6.23249313156326));
#29779=CARTESIAN_POINT('Ctrl Pts',(71.8280494454469,-5.12331106778224,5.22151862092123));
#29780=CARTESIAN_POINT('Ctrl Pts',(71.894219980261,-6.62026016417667,3.09030416749892));
#29781=CARTESIAN_POINT('Ctrl Pts',(71.960390515075,-6.89385797829254,0.80594375703103));
#29782=CARTESIAN_POINT('Ctrl Pts',(71.968109788848,-6.92577515165044,0.539456513818102));
#29783=CARTESIAN_POINT('Ctrl Pts',(71.9758290626209,-6.94104383768068,0.270885119828461));
#29784=CARTESIAN_POINT('Ctrl Pts',(71.9835483363939,-6.9401949188535,0.00210382873980236));
#29785=CARTESIAN_POINT('Origin',(29.75,0.,0.));
#29786=CARTESIAN_POINT('',(73.4128916636062,-6.92763786104848,9.47019909190297E-6));
#29787=CARTESIAN_POINT('',(73.2335483363939,-6.92837444992812,0.00246305386789827));
#29788=CARTESIAN_POINT('',(29.75,-6.933,-8.4904762584886E-16));
#29789=CARTESIAN_POINT('Ctrl Pts',(73.4128916636062,-6.92029165047812,2.2444507172259E-5));
#29790=CARTESIAN_POINT('Ctrl Pts',(73.3868981758774,-6.92413299961627,0.90830462489887));
#29791=CARTESIAN_POINT('Ctrl Pts',(73.3609046881487,-6.75800402829825,1.81602407914437));
#29792=CARTESIAN_POINT('Ctrl Pts',(73.3349112004199,-6.41502137678869,2.65215700470205));
#29793=CARTESIAN_POINT('Ctrl Pts',(73.3018259330129,-5.97846307958873,3.71641131788004));
#29794=CARTESIAN_POINT('Ctrl Pts',(73.2687406656059,-5.25538521396701,4.66468873262861));
#29795=CARTESIAN_POINT('Ctrl Pts',(73.2356553981989,-4.35552620310463,5.38949129071545));
#29796=CARTESIAN_POINT('Ctrl Pts',(73.2025701307919,-3.4556671922422,6.11429384880233));
#29797=CARTESIAN_POINT('Ctrl Pts',(73.1694848633848,-2.37902703613907,6.61562155022746));
#29798=CARTESIAN_POINT('Ctrl Pts',(73.1363995959778,-1.24850598774616,6.82250488956186));
#29799=CARTESIAN_POINT('Ctrl Pts',(73.1033143285708,-0.117984939353238,
7.02938822889626));
#29800=CARTESIAN_POINT('Ctrl Pts',(73.0702290611638,1.06641700132947,6.94182720613994));
#29801=CARTESIAN_POINT('Ctrl Pts',(73.0371437937568,2.16463905450583,6.58267021332574));
#29802=CARTESIAN_POINT('Ctrl Pts',(73.0040585263498,3.26286110768207,6.22351322051157));
#29803=CARTESIAN_POINT('Ctrl Pts',(72.9709732589427,4.27490327335198,5.59276025763959));
#29804=CARTESIAN_POINT('Ctrl Pts',(72.9378879915357,5.06006237968395,4.75207816740074));
#29805=CARTESIAN_POINT('Ctrl Pts',(72.8717174567216,6.63038059234808,3.07071398692286));
#29806=CARTESIAN_POINT('Ctrl Pts',(72.8055469219076,7.29316656766025,0.549633296977299));
#29807=CARTESIAN_POINT('Ctrl Pts',(72.7393763870936,6.73971393441234,-1.67520577327393));
#29808=CARTESIAN_POINT('Ctrl Pts',(72.6732058522796,6.18626130116446,-3.90004484352504));
#29809=CARTESIAN_POINT('Ctrl Pts',(72.6070353174655,4.41657005935665,-5.82864229408185));
#29810=CARTESIAN_POINT('Ctrl Pts',(72.5408647826515,2.24392949191622,-6.57214175759916));
#29811=CARTESIAN_POINT('Ctrl Pts',(72.4746942478375,0.0712889244756562,
-7.31564122111651));
#29812=CARTESIAN_POINT('Ctrl Pts',(72.4085237130234,-2.50430096859759,-6.87404269759419));
#29813=CARTESIAN_POINT('Ctrl Pts',(72.3423531782093,-4.3051403399917,-5.44924037420161));
#29814=CARTESIAN_POINT('Ctrl Pts',(72.2825326733416,-5.93316285311149,-4.16116865827016));
#29815=CARTESIAN_POINT('Ctrl Pts',(72.2227121684739,-6.92799727846338,-2.06954416437256));
#29816=CARTESIAN_POINT('Ctrl Pts',(72.1628916636062,-6.94192775449039,0.00618195413371575));
#29817=CARTESIAN_POINT('Ctrl Pts',(71.9835483363939,-6.9401949188535,0.00210382873980236));
#29818=CARTESIAN_POINT('Ctrl Pts',(72.0089143300279,-6.93740532099759,-0.881127511310418));
#29819=CARTESIAN_POINT('Ctrl Pts',(72.0342803236619,-6.76057480142328,-1.76662535962301));
#29820=CARTESIAN_POINT('Ctrl Pts',(72.059646317296,-6.42854092195365,-2.58788465809884));
#29821=CARTESIAN_POINT('Ctrl Pts',(72.092731584703,-5.99546387206851,-3.65906617349956));
#29822=CARTESIAN_POINT('Ctrl Pts',(72.1258168521101,-5.2983486858099,-4.62096250980574));
#29823=CARTESIAN_POINT('Ctrl Pts',(72.1589021195171,-4.41133942826932,-5.35195176352421));
#29824=CARTESIAN_POINT('Ctrl Pts',(72.1919873869242,-3.52433017072873,-6.08294101724269));
#29825=CARTESIAN_POINT('Ctrl Pts',(72.2250726543312,-2.44742684190618,-6.58302318837345));
#29826=CARTESIAN_POINT('Ctrl Pts',(72.2581579217382,-1.31336822550145,-6.80387094031927));
#29827=CARTESIAN_POINT('Ctrl Pts',(72.2912431891452,-0.179309609096652,
-7.0247186922651));
#29828=CARTESIAN_POINT('Ctrl Pts',(72.3243284565522,1.01190429489034,-6.96633202502595));
#29829=CARTESIAN_POINT('Ctrl Pts',(72.3574137239592,2.10704588485406,-6.61413975637045));
#29830=CARTESIAN_POINT('Ctrl Pts',(72.4235842587733,4.29732906478144,-5.90975521905948));
#29831=CARTESIAN_POINT('Ctrl Pts',(72.4897547935873,6.10332298861579,-4.0301482760832));
#29832=CARTESIAN_POINT('Ctrl Pts',(72.5559253284013,6.70278317878333,-1.81727631370743));
#29833=CARTESIAN_POINT('Ctrl Pts',(72.6220958632153,7.30224336895088,0.395595648668328));
#29834=CARTESIAN_POINT('Ctrl Pts',(72.6882663980294,6.69516982545161,2.94173263044357));
#29835=CARTESIAN_POINT('Ctrl Pts',(72.7544369328434,5.15921646832352,4.64875676238626));
#29836=CARTESIAN_POINT('Ctrl Pts',(72.8206074676575,3.62326311119548,6.3557808943289));
#29837=CARTESIAN_POINT('Ctrl Pts',(72.8867780024715,1.15842994043866,7.22369217643902));
#29838=CARTESIAN_POINT('Ctrl Pts',(72.9529485372855,-1.10822237865247,6.8556626234175));
#29839=CARTESIAN_POINT('Ctrl Pts',(73.0191190720996,-3.37487469774379,6.48763307039594));
#29840=CARTESIAN_POINT('Ctrl Pts',(73.0852896069136,-5.44334616516939,4.88366268224249));
#29841=CARTESIAN_POINT('Ctrl Pts',(73.1514601417277,-6.36261189066002,2.78338431219154));
#29842=CARTESIAN_POINT('Ctrl Pts',(73.1788228732831,-6.74274515307623,1.91488062859826));
#29843=CARTESIAN_POINT('Ctrl Pts',(73.2061856048385,-6.9263671749664,0.961509550380373));
#29844=CARTESIAN_POINT('Ctrl Pts',(73.2335483363939,-6.92150572898554,0.00612057123355675));
#29845=CARTESIAN_POINT('Origin',(29.75,0.,0.));
#29846=CARTESIAN_POINT('',(74.6628916636063,-6.93302851199415,-6.57016384422878E-5));
#29847=CARTESIAN_POINT('',(74.4835483363939,-6.93138337985325,-0.00328068813936701));
#29848=CARTESIAN_POINT('',(29.75,-6.933,-8.4904762584886E-16));
#29849=CARTESIAN_POINT('Ctrl Pts',(74.6628916636062,-6.933,1.47798440153224E-12));
#29850=CARTESIAN_POINT('Ctrl Pts',(74.6056674683211,-6.93299999999958,1.99420935701776));
#29851=CARTESIAN_POINT('Ctrl Pts',(74.548443273036,-6.02307502629165,3.97063309653173));
#29852=CARTESIAN_POINT('Ctrl Pts',(74.491219077751,-4.50798484753872,5.2673106624122));
#29853=CARTESIAN_POINT('Ctrl Pts',(74.4339948824659,-2.9928946687858,6.56398822829268));
#29854=CARTESIAN_POINT('Ctrl Pts',(74.3767706871808,-0.89966434562727,7.15779044292429));
#29855=CARTESIAN_POINT('Ctrl Pts',(74.3195464918957,1.07062371681991,6.84983604599283));
#29856=CARTESIAN_POINT('Ctrl Pts',(74.2623222966106,3.04091177926709,6.54188164906137));
#29857=CARTESIAN_POINT('Ctrl Pts',(74.2050981013255,4.85311303639994,5.33766370386297));
#29858=CARTESIAN_POINT('Ctrl Pts',(74.1478739060404,5.90026971493839,3.64050907030609));
#29859=CARTESIAN_POINT('Ctrl Pts',(74.0906497107553,6.94742639347683,1.9433544367492));
#29860=CARTESIAN_POINT('Ctrl Pts',(74.0334255154702,7.21086008527505,-0.216464293125449));
#29861=CARTESIAN_POINT('Ctrl Pts',(73.9762013201851,6.60233935006037,-2.11556236179517));
#29862=CARTESIAN_POINT('Ctrl Pts',(73.9189771249,5.99381861484569,-4.01466043046489));
#29863=CARTESIAN_POINT('Ctrl Pts',(73.8617529296149,4.52419779647178,-5.61916312790536));
#29864=CARTESIAN_POINT('Ctrl Pts',(73.8045287343298,2.68569473000269,-6.39167683923677));
#29865=CARTESIAN_POINT('Ctrl Pts',(73.7473045390447,0.847191663533602,-7.16419055056818));
#29866=CARTESIAN_POINT('Ctrl Pts',(73.6900803437596,-1.32739978994318,-7.09093574623759));
#29867=CARTESIAN_POINT('Ctrl Pts',(73.6328561484745,-3.1097470673632,-6.19644754492653));
#29868=CARTESIAN_POINT('Ctrl Pts',(73.5756319531894,-4.89209434478322,-5.30195934361546));
#29869=CARTESIAN_POINT('Ctrl Pts',(73.5184077579043,-6.25040525058729,-3.60219296582541));
#29870=CARTESIAN_POINT('Ctrl Pts',(73.4611835626192,-6.72974280712797,-1.66644854403288));
#29871=CARTESIAN_POINT('Ctrl Pts',(73.4450862629482,-6.86458158035597,-1.12191912096589));
#29872=CARTESIAN_POINT('Ctrl Pts',(73.4289889632772,-6.93300000000012,-0.560975745776578));
#29873=CARTESIAN_POINT('Ctrl Pts',(73.4128916636062,-6.933,1.52572399159112E-12));
#29874=CARTESIAN_POINT('Ctrl Pts',(73.2335483363939,-6.933,-4.15320555724463E-12));
#29875=CARTESIAN_POINT('Ctrl Pts',(73.290772531679,-6.93299999999881,-1.99420935702036));
#29876=CARTESIAN_POINT('Ctrl Pts',(73.3479967269641,-6.02307502629018,-3.97063309653393));
#29877=CARTESIAN_POINT('Ctrl Pts',(73.4052209222492,-4.50798484753684,-5.26731066241381));
#29878=CARTESIAN_POINT('Ctrl Pts',(73.4624451175343,-2.9928946687835,-6.5639882282937));
#29879=CARTESIAN_POINT('Ctrl Pts',(73.5196693128193,-0.89966434562485,-7.15779044292458));
#29880=CARTESIAN_POINT('Ctrl Pts',(73.5768935081044,1.07062371682216,-6.84983604599248));
#29881=CARTESIAN_POINT('Ctrl Pts',(73.6341177033895,3.04091177926917,-6.54188164906038));
#29882=CARTESIAN_POINT('Ctrl Pts',(73.6913418986746,4.85311303640158,-5.33766370386146));
#29883=CARTESIAN_POINT('Ctrl Pts',(73.7485660939597,5.90026971493948,-3.64050907030431));
#29884=CARTESIAN_POINT('Ctrl Pts',(73.8057902892448,6.94742639347738,-1.94335443674717));
#29885=CARTESIAN_POINT('Ctrl Pts',(73.8630144845299,7.21086008527498,0.216464293127474));
#29886=CARTESIAN_POINT('Ctrl Pts',(73.920238679815,6.6023393500598,2.11556236179696));
#29887=CARTESIAN_POINT('Ctrl Pts',(73.9774628751001,5.99381861484462,4.01466043046646));
#29888=CARTESIAN_POINT('Ctrl Pts',(74.0346870703852,4.52419779647035,5.61916312790649));
#29889=CARTESIAN_POINT('Ctrl Pts',(74.0919112656703,2.68569473000113,6.39167683923743));
#29890=CARTESIAN_POINT('Ctrl Pts',(74.1491354609554,0.847191663531917,7.16419055056836));
#29891=CARTESIAN_POINT('Ctrl Pts',(74.2063596562405,-1.32739978994477,7.09093574623728));
#29892=CARTESIAN_POINT('Ctrl Pts',(74.2635838515256,-3.10974706736454,6.19644754492586));
#29893=CARTESIAN_POINT('Ctrl Pts',(74.3208080468107,-4.89209434478431,5.30195934361443));
#29894=CARTESIAN_POINT('Ctrl Pts',(74.3780322420958,-6.25040525058798,3.60219296582418));
#29895=CARTESIAN_POINT('Ctrl Pts',(74.4352564373808,-6.72974280712828,1.66644854403162));
#29896=CARTESIAN_POINT('Ctrl Pts',(74.4513537370519,-6.86458158035629,1.12191912096416));
#29897=CARTESIAN_POINT('Ctrl Pts',(74.4674510367229,-6.93300000000034,0.560975745774362));
#29898=CARTESIAN_POINT('Ctrl Pts',(74.4835483363939,-6.933,-4.20066759154736E-12));
#29899=CARTESIAN_POINT('Origin',(29.75,0.,0.));
#29900=CARTESIAN_POINT('',(75.9128916636063,-6.93577247332454,-0.000335286187928552));
#29901=CARTESIAN_POINT('',(75.7335483363939,-6.94460482329128,0.000883125311795762));
#29902=CARTESIAN_POINT('',(29.75,-6.933,-8.4904762584886E-16));
#29903=CARTESIAN_POINT('Ctrl Pts',(75.9128916636063,-6.93577247332454,-0.000335286187928552));
#29904=CARTESIAN_POINT('Ctrl Pts',(75.8806965277196,-6.93514425451495,1.1180543323845));
#29905=CARTESIAN_POINT('Ctrl Pts',(75.8485013918329,-6.65226718410521,2.23682721397932));
#29906=CARTESIAN_POINT('Ctrl Pts',(75.8163062559463,-6.12942454003317,3.23224042168337));
#29907=CARTESIAN_POINT('Ctrl Pts',(75.7832209885393,-5.59212633598693,4.25517482622593));
#29908=CARTESIAN_POINT('Ctrl Pts',(75.7501357211323,-4.80140998319663,5.14783395957035));
#29909=CARTESIAN_POINT('Ctrl Pts',(75.7170504537253,-3.84154731235279,5.78177750999706));
#29910=CARTESIAN_POINT('Ctrl Pts',(75.6508799189113,-1.92182197066505,7.04966461085053));
#29911=CARTESIAN_POINT('Ctrl Pts',(75.5847093840972,0.674488643236908,7.28268938003312));
#29912=CARTESIAN_POINT('Ctrl Pts',(75.5185388492831,2.77585362956056,6.36590612130795));
#29913=CARTESIAN_POINT('Ctrl Pts',(75.4523683144691,4.87721861588421,5.44912286258278));
#29914=CARTESIAN_POINT('Ctrl Pts',(75.3861977796551,6.48363797462955,3.38253157594985));
#29915=CARTESIAN_POINT('Ctrl Pts',(75.320027244841,6.85434798412124,1.11632363563946));
#29916=CARTESIAN_POINT('Ctrl Pts',(75.253856710027,7.22505799361293,-1.14988430467093));
#29917=CARTESIAN_POINT('Ctrl Pts',(75.187686175213,6.36005865385096,-3.61570889865878));
#29918=CARTESIAN_POINT('Ctrl Pts',(75.1215156403989,4.65485526475585,-5.15369646059015));
#29919=CARTESIAN_POINT('Ctrl Pts',(75.0553451055849,2.94965187566074,-6.69168402252151));
#29920=CARTESIAN_POINT('Ctrl Pts',(74.9891745707708,0.404244437232484,-7.3018345523964));
#29921=CARTESIAN_POINT('Ctrl Pts',(74.9230040359568,-1.80934090928194,-6.70495410796962));
#29922=CARTESIAN_POINT('Ctrl Pts',(74.8568335011428,-4.02292625579636,-6.10807366354283));
#29923=CARTESIAN_POINT('Ctrl Pts',(74.7906629663288,-5.90468951039696,-4.30416224481439));
#29924=CARTESIAN_POINT('Ctrl Pts',(74.7244924315147,-6.61164537146094,-2.11484808314536));
#29925=CARTESIAN_POINT('Ctrl Pts',(74.7039588422119,-6.83102309520318,-1.43547503626127));
#29926=CARTESIAN_POINT('Ctrl Pts',(74.6834252529091,-6.93727359651782,-0.71898991290854));
#29927=CARTESIAN_POINT('Ctrl Pts',(74.6628916636062,-6.93384748847811,-0.00195291085134108));
#29928=CARTESIAN_POINT('Ctrl Pts',(74.4835483363939,-6.92866114138664,-0.00880506282216201));
#29929=CARTESIAN_POINT('Ctrl Pts',(74.5027126818701,-6.93434561264149,-0.677464884404123));
#29930=CARTESIAN_POINT('Ctrl Pts',(74.5218770273463,-6.84558152848312,-1.34433981842437));
#29931=CARTESIAN_POINT('Ctrl Pts',(74.5410413728224,-6.65631914950611,-1.98079271750886));
#29932=CARTESIAN_POINT('Ctrl Pts',(74.6072119076365,-6.00283516526842,-4.17833339369304));
#29933=CARTESIAN_POINT('Ctrl Pts',(74.6733824424504,-4.15123205783588,-6.01318909209914));
#29934=CARTESIAN_POINT('Ctrl Pts',(74.7395529772645,-1.94449844419176,-6.66373488795828));
#29935=CARTESIAN_POINT('Ctrl Pts',(74.7726382446716,-0.841131637369642,
-6.98900778588786));
#29936=CARTESIAN_POINT('Ctrl Pts',(74.8057235120786,0.351017796005385,-7.01820320818067));
#29937=CARTESIAN_POINT('Ctrl Pts',(74.8388087794856,1.47943176153331,-6.7696753978216));
#29938=CARTESIAN_POINT('Ctrl Pts',(74.8718940468926,2.60784572706124,-6.52114758746254));
#29939=CARTESIAN_POINT('Ctrl Pts',(74.9049793142996,3.67252422474206,-5.99489654445161));
#29940=CARTESIAN_POINT('Ctrl Pts',(74.9380645817066,4.54121424326715,-5.24239563710084));
#29941=CARTESIAN_POINT('Ctrl Pts',(74.9711498491136,5.40990426179223,-4.48989472975007));
#29942=CARTESIAN_POINT('Ctrl Pts',(75.0042351165207,6.08260580116156,-3.51114395805947));
#29943=CARTESIAN_POINT('Ctrl Pts',(75.0373203839277,6.4895115820401,-2.42970425104458));
#29944=CARTESIAN_POINT('Ctrl Pts',(75.0704056513348,6.89641736291859,-1.34826454402982));
#29945=CARTESIAN_POINT('Ctrl Pts',(75.1034909187418,7.03752738530635,-0.1641359016908));
#29946=CARTESIAN_POINT('Ctrl Pts',(75.1365761861488,6.87292506515188,0.974339766996876));
#29947=CARTESIAN_POINT('Ctrl Pts',(75.2027467209628,6.5437204248429,3.25129110437249));
#29948=CARTESIAN_POINT('Ctrl Pts',(75.2689172557769,4.99166641436471,5.34563054714267));
#29949=CARTESIAN_POINT('Ctrl Pts',(75.3350877905909,2.90977586653595,6.3058170384578));
#29950=CARTESIAN_POINT('Ctrl Pts',(75.4012583254049,0.827885318707192,7.26600352977293));
#29951=CARTESIAN_POINT('Ctrl Pts',(75.467428860219,-1.78384176647215,7.09203706963299));
#29952=CARTESIAN_POINT('Ctrl Pts',(75.533599395033,-3.72313617215261,5.86229663078674));
#29953=CARTESIAN_POINT('Ctrl Pts',(75.599769929847,-5.66243057783302,4.63255619194052));
#29954=CARTESIAN_POINT('Ctrl Pts',(75.6659404646611,-6.9292923040146,2.34704177438805));
#29955=CARTESIAN_POINT('Ctrl Pts',(75.7321109994751,-6.94447174479279,0.0507634976017025));
#29956=CARTESIAN_POINT('Ctrl Pts',(75.7325901117814,-6.94458165257726,0.03413713687956));
#29957=CARTESIAN_POINT('Ctrl Pts',(75.7330692240876,-6.94462593987182,0.0175102118531011));
#29958=CARTESIAN_POINT('Ctrl Pts',(75.7335483363939,-6.94460482329128,0.000883125311795762));
#29959=CARTESIAN_POINT('Origin',(29.75,0.,0.));
#29960=CARTESIAN_POINT('',(77.1628916636062,-6.933,1.77691195091256E-12));
#29961=CARTESIAN_POINT('',(76.9835483363939,-6.9297498061854,0.00533558548810259));
#29962=CARTESIAN_POINT('',(29.75,-6.933,-8.4904762584886E-16));
#29963=CARTESIAN_POINT('Ctrl Pts',(77.1628916636062,-6.93482283397445,0.00227082123790745));
#29964=CARTESIAN_POINT('Ctrl Pts',(77.1441383373442,-6.93813353830398,0.656949323559923));
#29965=CARTESIAN_POINT('Ctrl Pts',(77.1253850110821,-6.84966132346527,1.31098698841223));
#29966=CARTESIAN_POINT('Ctrl Pts',(77.10663168482,-6.6660308597263,1.93661289511069));
#29967=CARTESIAN_POINT('Ctrl Pts',(77.040461150006,-6.01809641737947,4.14411466099759));
#29968=CARTESIAN_POINT('Ctrl Pts',(76.974290615192,-4.18543272105473,5.99788733423284));
#29969=CARTESIAN_POINT('Ctrl Pts',(76.908120080378,-1.98866675453222,6.65397089400068));
#29970=CARTESIAN_POINT('Ctrl Pts',(76.8419495455639,0.208099211990228,7.31005445376851));
#29971=CARTESIAN_POINT('Ctrl Pts',(76.7757790107498,2.76896744871042,6.76844890006899));
#29972=CARTESIAN_POINT('Ctrl Pts',(76.7096084759358,4.51483985655232,5.27678745211015));
#29973=CARTESIAN_POINT('Ctrl Pts',(76.6434379411217,6.26071226439422,3.7851260041513));
#29974=CARTESIAN_POINT('Ctrl Pts',(76.5772674063078,7.19158884335782,1.34340866193312));
#29975=CARTESIAN_POINT('Ctrl Pts',(76.5110968714937,6.88184311853839,-0.931933493819985));
#29976=CARTESIAN_POINT('Ctrl Pts',(76.4449263366797,6.57209739371898,-3.20727564957302));
#29977=CARTESIAN_POINT('Ctrl Pts',(76.3787558018656,5.0217293651166,-5.31624261886099));
#29978=CARTESIAN_POINT('Ctrl Pts',(76.3125852670516,2.94573031687968,-6.28910144766352));
#29979=CARTESIAN_POINT('Ctrl Pts',(76.2464147322375,0.869731268642629,-7.2619602764661));
#29980=CARTESIAN_POINT('Ctrl Pts',(76.1802441974236,-1.73189879922904,-7.09871096478309));
#29981=CARTESIAN_POINT('Ctrl Pts',(76.1140736626095,-3.68496568754885,-5.88281096159864));
#29982=CARTESIAN_POINT('Ctrl Pts',(76.0809883952025,-4.66149913170876,-5.27486096000641));
#29983=CARTESIAN_POINT('Ctrl Pts',(76.0479031277954,-5.4758917809807,-4.40374828553883));
#29984=CARTESIAN_POINT('Ctrl Pts',(76.0148178603884,-6.04045450968852,-3.39560490218326));
#29985=CARTESIAN_POINT('Ctrl Pts',(75.9817325929814,-6.60501723839632,-2.38746151882774));
#29986=CARTESIAN_POINT('Ctrl Pts',(75.9486473255744,-6.91975004654002,-1.24228742658426));
#29987=CARTESIAN_POINT('Ctrl Pts',(75.9155620581674,-6.93517642296081,-0.0930955425921683));
#29988=CARTESIAN_POINT('Ctrl Pts',(75.914671926647,-6.93559145674997,-0.062177493591001));
#29989=CARTESIAN_POINT('Ctrl Pts',(75.9137817951266,-6.93578984232606,-0.0312565363750059));
#29990=CARTESIAN_POINT('Ctrl Pts',(75.9128916636063,-6.93577247332454,-0.000335286187928552));
#29991=CARTESIAN_POINT('Ctrl Pts',(75.7335483363939,-6.94460482329128,0.000883125311795762));
#29992=CARTESIAN_POINT('Ctrl Pts',(75.7992397589017,-6.94170951420419,-2.27886830832412));
#29993=CARTESIAN_POINT('Ctrl Pts',(75.8649311814095,-5.70926429895426,-4.56165611502022));
#29994=CARTESIAN_POINT('Ctrl Pts',(75.9306226039173,-3.8056136169074,-5.80925374870641));
#29995=CARTESIAN_POINT('Ctrl Pts',(75.9967931387313,-1.88807889286908,-7.06595058220794));
#29996=CARTESIAN_POINT('Ctrl Pts',(76.0629636735453,0.710487710582319,-7.27230211319087));
#29997=CARTESIAN_POINT('Ctrl Pts',(76.1291342083593,2.81589166875497,-6.34485547810106));
#29998=CARTESIAN_POINT('Ctrl Pts',(76.1622194757663,3.86859364784136,-5.88113216055613));
#29999=CARTESIAN_POINT('Ctrl Pts',(76.1953047431734,4.79800496560802,-5.133959301493));
#30000=CARTESIAN_POINT('Ctrl Pts',(76.2283900105804,5.49947858928678,-4.21579868844575));
#30001=CARTESIAN_POINT('Ctrl Pts',(76.2614752779874,6.20095221296551,-3.29763807539856));
#30002=CARTESIAN_POINT('Ctrl Pts',(76.2945605453944,6.67448814255641,-2.20848970836712));
#30003=CARTESIAN_POINT('Ctrl Pts',(76.3276458128014,6.85229462999235,-1.0730317336501));
#30004=CARTESIAN_POINT('Ctrl Pts',(76.3607310802085,7.03010111742829,0.0624262410669793));
#30005=CARTESIAN_POINT('Ctrl Pts',(76.3938163476155,6.91217816270932,1.2441938234698));
#30006=CARTESIAN_POINT('Ctrl Pts',(76.4269016150226,6.52495911412754,2.3328377342437));
#30007=CARTESIAN_POINT('Ctrl Pts',(76.4599868824296,6.13774006554577,3.4214816450176));
#30008=CARTESIAN_POINT('Ctrl Pts',(76.4930721498366,5.48122492310122,4.41700188416254));
#30009=CARTESIAN_POINT('Ctrl Pts',(76.5261574172436,4.62067251741759,5.18033033841466));
#30010=CARTESIAN_POINT('Ctrl Pts',(76.5923279520576,2.89956770605038,6.70698724691885));
#30011=CARTESIAN_POINT('Ctrl Pts',(76.6584984868717,0.362313841727035,7.30487701585175));
#30012=CARTESIAN_POINT('Ctrl Pts',(76.7246690216857,-1.84759209267133,6.69451473804381));
#30013=CARTESIAN_POINT('Ctrl Pts',(76.7908395564998,-4.05749802706964,6.08415246023589));
#30014=CARTESIAN_POINT('Ctrl Pts',(76.8570100913138,-5.94005603154293,4.26553813568725));
#30015=CARTESIAN_POINT('Ctrl Pts',(76.9231806261278,-6.62755912924991,2.07454205389382));
#30016=CARTESIAN_POINT('Ctrl Pts',(76.9433031962165,-6.83662996884164,1.40825648821338));
#30017=CARTESIAN_POINT('Ctrl Pts',(76.9634257663052,-6.93518472965,0.707533867475353));
#30018=CARTESIAN_POINT('Ctrl Pts',(76.9835483363939,-6.9297498061854,0.00533558548810259));
#30019=CARTESIAN_POINT('Origin',(29.75,0.,0.));
#30020=CARTESIAN_POINT('',(78.4128916636062,-6.92804963575093,0.000312599262795181));
#30021=CARTESIAN_POINT('',(78.2335483363939,-6.92245089085948,-0.0021973978771043));
#30022=CARTESIAN_POINT('',(29.75,-6.933,-8.4904762584886E-16));
#30023=CARTESIAN_POINT('Ctrl Pts',(78.4128916636062,-6.933,1.9265145034808E-12));
#30024=CARTESIAN_POINT('Ctrl Pts',(78.3556674683211,-6.93299999999945,1.99420935701807));
#30025=CARTESIAN_POINT('Ctrl Pts',(78.298443273036,-6.02307502629152,3.97063309653186));
#30026=CARTESIAN_POINT('Ctrl Pts',(78.241219077751,-4.50798484753868,5.26731066241224));
#30027=CARTESIAN_POINT('Ctrl Pts',(78.1839948824659,-2.99289466878585,6.56398822829261));
#30028=CARTESIAN_POINT('Ctrl Pts',(78.1267706871808,-0.899664345627491,
7.15779044292423));
#30029=CARTESIAN_POINT('Ctrl Pts',(78.0695464918957,1.07062371681957,6.84983604599289));
#30030=CARTESIAN_POINT('Ctrl Pts',(78.0123222966106,3.04091177926664,6.54188164906155));
#30031=CARTESIAN_POINT('Ctrl Pts',(77.9550981013255,4.85311303639945,5.33766370386337));
#30032=CARTESIAN_POINT('Ctrl Pts',(77.8978739060404,5.900269714938,3.64050907030671));
#30033=CARTESIAN_POINT('Ctrl Pts',(77.8406497107553,6.94742639347656,1.94335443675005));
#30034=CARTESIAN_POINT('Ctrl Pts',(77.7834255154702,7.21086008527505,-0.2164642931244));
#30035=CARTESIAN_POINT('Ctrl Pts',(77.7262013201851,6.60233935006072,-2.11556236179409));
#30036=CARTESIAN_POINT('Ctrl Pts',(77.6689771249,5.99381861484639,-4.01466043046379));
#30037=CARTESIAN_POINT('Ctrl Pts',(77.611752929615,4.52419779647289,-5.61916312790442));
#30038=CARTESIAN_POINT('Ctrl Pts',(77.5545287343298,2.68569473000409,-6.39167683923618));
#30039=CARTESIAN_POINT('Ctrl Pts',(77.4973045390448,0.847191663535296,-7.16419055056795));
#30040=CARTESIAN_POINT('Ctrl Pts',(77.4400803437597,-1.32739978994134,-7.0909357462379));
#30041=CARTESIAN_POINT('Ctrl Pts',(77.3828561484746,-3.10974706736149,-6.19644754492739));
#30042=CARTESIAN_POINT('Ctrl Pts',(77.3256319531895,-4.89209434478164,-5.30195934361687));
#30043=CARTESIAN_POINT('Ctrl Pts',(77.2684077579044,-6.25040525058613,-3.60219296582736));
#30044=CARTESIAN_POINT('Ctrl Pts',(77.2111835626193,-6.72974280712742,-1.66644854403513));
#30045=CARTESIAN_POINT('Ctrl Pts',(77.1950862629483,-6.8645815803558,-1.12191912096735));
#30046=CARTESIAN_POINT('Ctrl Pts',(77.1789889632773,-6.93300000000014,-0.56097574577718));
#30047=CARTESIAN_POINT('Ctrl Pts',(77.1628916636062,-6.933,1.77691195091256E-12));
#30048=CARTESIAN_POINT('Ctrl Pts',(76.9835483363939,-6.9297498061854,0.00533558548810259));
#30049=CARTESIAN_POINT('Ctrl Pts',(77.0295963011192,-6.91731266903644,-1.60155665425157));
#30050=CARTESIAN_POINT('Ctrl Pts',(77.0756442658446,-6.36031740813025,-3.21617642318602));
#30051=CARTESIAN_POINT('Ctrl Pts',(77.1216922305699,-5.33697258446145,-4.4435333213297));
#30052=CARTESIAN_POINT('Ctrl Pts',(77.1878627653839,-3.86643475102544,-6.20723477572147));
#30053=CARTESIAN_POINT('Ctrl Pts',(77.254033300198,-1.43291089321261,-7.1712598454668));
#30054=CARTESIAN_POINT('Ctrl Pts',(77.320203835012,0.842842081745409,-6.89345641489297));
#30055=CARTESIAN_POINT('Ctrl Pts',(77.3863743698261,3.11859505670343,-6.61565298431915));
#30056=CARTESIAN_POINT('Ctrl Pts',(77.4525449046401,5.23657714880673,-5.09602105342644));
#30057=CARTESIAN_POINT('Ctrl Pts',(77.5187154394541,6.24607061556865,-3.02870249342226));
#30058=CARTESIAN_POINT('Ctrl Pts',(77.5518007068611,6.75081734894962,-1.99504321342014));
#30059=CARTESIAN_POINT('Ctrl Pts',(77.5848859742681,6.97844192599519,-0.824462276140171));
#30060=CARTESIAN_POINT('Ctrl Pts',(77.6179712416751,6.92160306263817,0.329597297566678));
#30061=CARTESIAN_POINT('Ctrl Pts',(77.6510565090822,6.86476419928114,1.48365687127346));
#30062=CARTESIAN_POINT('Ctrl Pts',(77.6841417764892,6.52346189552155,2.62119508140712));
#30063=CARTESIAN_POINT('Ctrl Pts',(77.7172270438963,5.92639008272138,3.60322624674164));
#30064=CARTESIAN_POINT('Ctrl Pts',(77.7503123113033,5.32931826992122,4.58525741207615));
#30065=CARTESIAN_POINT('Ctrl Pts',(77.7833975787103,4.47647694808047,5.41178153261152));
#30066=CARTESIAN_POINT('Ctrl Pts',(77.8164828461173,3.47805314064643,5.99336046689384));
#30067=CARTESIAN_POINT('Ctrl Pts',(77.8495681135243,2.47962933321233,6.5749394011762));
#30068=CARTESIAN_POINT('Ctrl Pts',(77.8826533809313,1.33562304018492,6.91157314920548));
#30069=CARTESIAN_POINT('Ctrl Pts',(77.9157386483383,0.18564060271005,6.93916237704205));
#30070=CARTESIAN_POINT('Ctrl Pts',(77.9819091831524,-2.11432427223969,6.99434083271517));
#30071=CARTESIAN_POINT('Ctrl Pts',(78.0480797179665,-4.4381937249793,5.81334120761742));
#30072=CARTESIAN_POINT('Ctrl Pts',(78.1142502527805,-5.73216807578779,3.92076182261932));
#30073=CARTESIAN_POINT('Ctrl Pts',(78.1540162806516,-6.50979848550715,2.7833920736263));
#30074=CARTESIAN_POINT('Ctrl Pts',(78.1937823085228,-6.91547584179783,1.38903084661121));
#30075=CARTESIAN_POINT('Ctrl Pts',(78.2335483363939,-6.92245089085948,-0.0021973978771043));
#30076=CARTESIAN_POINT('Origin',(29.75,0.,0.));
#30077=CARTESIAN_POINT('',(79.6628916636062,-6.94043042295203,-0.00713010923047652));
#30078=CARTESIAN_POINT('',(79.4835483363939,-6.93525986827018,-0.000860828807844148));
#30079=CARTESIAN_POINT('',(29.75,-6.933,-8.4904762584886E-16));
#30080=CARTESIAN_POINT('Ctrl Pts',(79.6628916636062,-6.94043042295203,-0.00713010923047652));
#30081=CARTESIAN_POINT('Ctrl Pts',(79.6048514217793,-6.92467100667924,2.0081896470561));
#30082=CARTESIAN_POINT('Ctrl Pts',(79.5468111799523,-5.99531508320213,4.04002741126765));
#30083=CARTESIAN_POINT('Ctrl Pts',(79.4887709381254,-4.44984465230886,5.33171148088348));
#30084=CARTESIAN_POINT('Ctrl Pts',(79.4226004033113,-2.687884299759,6.80433500909159));
#30085=CARTESIAN_POINT('Ctrl Pts',(79.3564298684973,-0.125108764999251,
7.3149193243508));
#30086=CARTESIAN_POINT('Ctrl Pts',(79.2902593336833,2.06669920281348,6.63000898567692));
#30087=CARTESIAN_POINT('Ctrl Pts',(79.2240887988692,4.25850717062608,5.94509864700308));
#30088=CARTESIAN_POINT('Ctrl Pts',(79.1579182640551,6.07934757149164,4.0646936543963));
#30089=CARTESIAN_POINT('Ctrl Pts',(79.0917477292411,6.69232407312594,1.85551141711626));
#30090=CARTESIAN_POINT('Ctrl Pts',(79.0255771944271,7.30530057476027,-0.353670820163851));
#30091=CARTESIAN_POINT('Ctrl Pts',(78.9594066596131,6.71041317716317,-2.89163030211736));
#30092=CARTESIAN_POINT('Ctrl Pts',(78.893236124799,5.18579366300061,-4.614540173529));
#30093=CARTESIAN_POINT('Ctrl Pts',(78.860150857392,4.42348390591939,-5.47599510923475));
#30094=CARTESIAN_POINT('Ctrl Pts',(78.827065589985,3.42874111969687,-6.13368764230509));
#30095=CARTESIAN_POINT('Ctrl Pts',(78.793980322578,2.34055610925253,-6.52219444931898));
#30096=CARTESIAN_POINT('Ctrl Pts',(78.7608950551709,1.252371098808,-6.91070125633294));
#30097=CARTESIAN_POINT('Ctrl Pts',(78.7278097877639,0.0707438641416697,
-7.03002233729033));
#30098=CARTESIAN_POINT('Ctrl Pts',(78.6947245203569,-1.06492368765609,-6.85355939182368));
#30099=CARTESIAN_POINT('Ctrl Pts',(78.6616392529499,-2.20059123945372,-6.67709644635705));
#30100=CARTESIAN_POINT('Ctrl Pts',(78.6285539855429,-3.29029910838259,-6.20484947446653));
#30101=CARTESIAN_POINT('Ctrl Pts',(78.5954687181359,-4.2092890275671,-5.50446266384738));
#30102=CARTESIAN_POINT('Ctrl Pts',(78.5623834507288,-5.12827894675161,-4.80407585322824));
#30103=CARTESIAN_POINT('Ctrl Pts',(78.5292981833218,-5.87655091619167,-3.87554920388036));
#30104=CARTESIAN_POINT('Ctrl Pts',(78.4962129159148,-6.34151941390539,-2.82339661602677));
#30105=CARTESIAN_POINT('Ctrl Pts',(78.4684391651453,-6.73184175926583,-1.94015685293011));
#30106=CARTESIAN_POINT('Ctrl Pts',(78.4406654143758,-6.92252221752414,-0.969798794008508));
#30107=CARTESIAN_POINT('Ctrl Pts',(78.4128916636062,-6.91962899029542,0.00084433539633888));
#30108=CARTESIAN_POINT('Ctrl Pts',(78.2335483363939,-6.92245089085948,-0.0021973978771043));
#30109=CARTESIAN_POINT('Ctrl Pts',(78.2599528433368,-6.92708229965828,-0.925968209479977));
#30110=CARTESIAN_POINT('Ctrl Pts',(78.2863573502796,-6.75592926100566,-1.84835771580232));
#30111=CARTESIAN_POINT('Ctrl Pts',(78.3127618572225,-6.40116091921723,-2.69321436787948));
#30112=CARTESIAN_POINT('Ctrl Pts',(78.3789323920366,-5.51210016296075,-4.81045202848222));
#30113=CARTESIAN_POINT('Ctrl Pts',(78.4451029268507,-3.46989940157015,-6.44076820478922));
#30114=CARTESIAN_POINT('Ctrl Pts',(78.5112734616647,-1.20831798698859,-6.83873031983177));
#30115=CARTESIAN_POINT('Ctrl Pts',(78.5774439964787,1.05326342759283,-7.2366924348743));
#30116=CARTESIAN_POINT('Ctrl Pts',(78.6436145312927,3.53422549536492,-6.40230048865278));
#30117=CARTESIAN_POINT('Ctrl Pts',(78.7097850661068,5.09314398382109,-4.72122955159532));
#30118=CARTESIAN_POINT('Ctrl Pts',(78.7759556009208,6.65206247227726,-3.04015861453786));
#30119=CARTESIAN_POINT('Ctrl Pts',(78.8421261357349,7.28893738141711,-0.512408686644281));
#30120=CARTESIAN_POINT('Ctrl Pts',(78.9082966705489,6.72564139547028,1.71819229071338));
#30121=CARTESIAN_POINT('Ctrl Pts',(78.941381937956,6.44399340249686,2.83349277939225));
#30122=CARTESIAN_POINT('Ctrl Pts',(78.974467205363,5.86230268575175,3.87450603043722));
#30123=CARTESIAN_POINT('Ctrl Pts',(79.00755247277,5.07400169053412,4.71929339835356));
#30124=CARTESIAN_POINT('Ctrl Pts',(79.0406377401769,4.28570069531653,5.56408076626987));
#30125=CARTESIAN_POINT('Ctrl Pts',(79.073723007584,3.29078942162624,6.2126422510577));
#30126=CARTESIAN_POINT('Ctrl Pts',(79.106808274991,2.2008926306588,6.57734068040401));
#30127=CARTESIAN_POINT('Ctrl Pts',(79.139893542398,1.11099583969131,6.94203910975033));
#30128=CARTESIAN_POINT('Ctrl Pts',(79.1729788098051,-0.0738864685531249,
7.02287448365523));
#30129=CARTESIAN_POINT('Ctrl Pts',(79.2060640772121,-1.21186531751188,6.82265386689802));
#30130=CARTESIAN_POINT('Ctrl Pts',(79.2391493446191,-2.34984416647063,6.6224332501408));
#30131=CARTESIAN_POINT('Ctrl Pts',(79.2722346120261,-3.44091955614338,6.14115664272139));
#30132=CARTESIAN_POINT('Ctrl Pts',(79.3053198794331,-4.33708687488498,5.41997365012329));
#30133=CARTESIAN_POINT('Ctrl Pts',(79.3647293650867,-5.94628769563128,4.12498303918833));
#30134=CARTESIAN_POINT('Ctrl Pts',(79.4241388507403,-6.92703652059706,2.05645008161881));
#30135=CARTESIAN_POINT('Ctrl Pts',(79.4835483363939,-6.94186525225857,-0.00337695104174475));
#30136=CARTESIAN_POINT('Origin',(29.75,0.,0.));
#30137=CARTESIAN_POINT('',(80.9128916636062,-6.9365780831978,0.00570569907908797));
#30138=CARTESIAN_POINT('',(80.7335483363939,-6.933,-3.25614535334751E-12));
#30139=CARTESIAN_POINT('',(29.75,-6.933,-8.4904762584886E-16));
#30140=CARTESIAN_POINT('Ctrl Pts',(80.9128916636062,-6.9365780831978,0.00570569907908797));
#30141=CARTESIAN_POINT('Ctrl Pts',(80.9013784988108,-6.94039333737286,0.406469770832339));
#30142=CARTESIAN_POINT('Ctrl Pts',(80.8898653340155,-6.90893189083218,0.806646451518075));
#30143=CARTESIAN_POINT('Ctrl Pts',(80.8783521692201,-6.84015515512757,1.20022589492488));
#30144=CARTESIAN_POINT('Ctrl Pts',(80.8121816344061,-6.44486910952388,3.46227657559952));
#30145=CARTESIAN_POINT('Ctrl Pts',(80.7460110995921,-4.81697030490652,5.50640481680099));
#30146=CARTESIAN_POINT('Ctrl Pts',(80.6798405647781,-2.7007860187726,6.39796996131343));
#30147=CARTESIAN_POINT('Ctrl Pts',(80.613670029964,-0.584601732638681,7.28953510582587));
#30148=CARTESIAN_POINT('Ctrl Pts',(80.5474994951499,2.01986803501185,7.02853715364932));
#30149=CARTESIAN_POINT('Ctrl Pts',(80.4813289603359,3.91397706158762,5.73680291452963));
#30150=CARTESIAN_POINT('Ctrl Pts',(80.4151584255218,5.80808608816334,4.44506867540999));
#30151=CARTESIAN_POINT('Ctrl Pts',(80.3489878907078,6.99183437366439,2.12259814934748));
#30152=CARTESIAN_POINT('Ctrl Pts',(80.2828173558938,6.93937716091364,-0.177430400215159));
#30153=CARTESIAN_POINT('Ctrl Pts',(80.2497320884868,6.91314855453826,-1.32744467499651));
#30154=CARTESIAN_POINT('Ctrl Pts',(80.2166468210798,6.57786857359988,-2.47184845565289));
#30155=CARTESIAN_POINT('Ctrl Pts',(80.1835615536727,5.99747133187885,-3.47095965960107));
#30156=CARTESIAN_POINT('Ctrl Pts',(80.1504762862657,5.41707409015789,-4.47007086354912));
#30157=CARTESIAN_POINT('Ctrl Pts',(80.1173910188587,4.5915595876543,-5.32388949078905));
#30158=CARTESIAN_POINT('Ctrl Pts',(80.0843057514517,3.61023553540428,-5.92212277622558));
#30159=CARTESIAN_POINT('Ctrl Pts',(80.0512204840447,2.62891148315414,-6.52035606166219));
#30160=CARTESIAN_POINT('Ctrl Pts',(80.0181352166377,1.49177788115749,-6.86300400529537));
#30161=CARTESIAN_POINT('Ctrl Pts',(79.9850499492307,0.337786364125504,-6.92120825488567));
#30162=CARTESIAN_POINT('Ctrl Pts',(79.9519646818237,-0.816205152906479,
-6.97941250447597));
#30163=CARTESIAN_POINT('Ctrl Pts',(79.9188794144166,-1.98705458497383,-6.75317306002338));
#30164=CARTESIAN_POINT('Ctrl Pts',(79.8857941470096,-3.02131033278072,-6.24964965428966));
#30165=CARTESIAN_POINT('Ctrl Pts',(79.8196236121956,-5.08982182839451,-5.2426028428222));
#30166=CARTESIAN_POINT('Ctrl Pts',(79.7534530773815,-6.61195858696656,-3.12642018623015));
#30167=CARTESIAN_POINT('Ctrl Pts',(79.6872825425675,-6.89245438108255,-0.850997487355676));
#30168=CARTESIAN_POINT('Ctrl Pts',(79.6791522495804,-6.92691855753537,-0.571419072834691));
#30169=CARTESIAN_POINT('Ctrl Pts',(79.6710219565933,-6.94263800630402,-0.289436653199143));
#30170=CARTESIAN_POINT('Ctrl Pts',(79.6628916636062,-6.94043042295203,-0.00713010923047652));
#30171=CARTESIAN_POINT('Ctrl Pts',(79.4835483363939,-6.933,-3.60267371490863E-12));
#30172=CARTESIAN_POINT('Ctrl Pts',(79.540772531679,-6.93299999999897,-1.99420935701981));
#30173=CARTESIAN_POINT('Ctrl Pts',(79.5979967269641,-6.02307502629049,-3.97063309653345));
#30174=CARTESIAN_POINT('Ctrl Pts',(79.6552209222492,-4.50798484753726,-5.26731066241346));
#30175=CARTESIAN_POINT('Ctrl Pts',(79.7124451175342,-2.99289466878403,-6.56398822829346));
#30176=CARTESIAN_POINT('Ctrl Pts',(79.7696693128193,-0.899664345625418,
-7.15779044292451));
#30177=CARTESIAN_POINT('Ctrl Pts',(79.8268935081044,1.07062371682162,-6.84983604599257));
#30178=CARTESIAN_POINT('Ctrl Pts',(79.8841177033895,3.04091177926865,-6.54188164906062));
#30179=CARTESIAN_POINT('Ctrl Pts',(79.9413418986746,4.85311303640116,-5.33766370386184));
#30180=CARTESIAN_POINT('Ctrl Pts',(79.9985660939597,5.90026971493919,-3.64050907030478));
#30181=CARTESIAN_POINT('Ctrl Pts',(80.0557902892448,6.94742639347723,-1.94335443674772));
#30182=CARTESIAN_POINT('Ctrl Pts',(80.1130144845299,7.21086008527499,0.216464293126901));
#30183=CARTESIAN_POINT('Ctrl Pts',(80.170238679815,6.60233935005997,2.11556236179644));
#30184=CARTESIAN_POINT('Ctrl Pts',(80.2274628751001,5.99381861484494,4.01466043046598));
#30185=CARTESIAN_POINT('Ctrl Pts',(80.2846870703852,4.5241977964708,5.61916312790613));
#30186=CARTESIAN_POINT('Ctrl Pts',(80.3419112656703,2.68569473000164,6.39167683923721));
#30187=CARTESIAN_POINT('Ctrl Pts',(80.3991354609554,0.847191663532486,7.1641905505683));
#30188=CARTESIAN_POINT('Ctrl Pts',(80.4563596562405,-1.3273997899442,7.09093574623738));
#30189=CARTESIAN_POINT('Ctrl Pts',(80.5135838515256,-3.10974706736404,6.1964475449261));
#30190=CARTESIAN_POINT('Ctrl Pts',(80.5708080468107,-4.89209434478389,5.30195934361482));
#30191=CARTESIAN_POINT('Ctrl Pts',(80.6280322420957,-6.2504052505877,3.60219296582467));
#30192=CARTESIAN_POINT('Ctrl Pts',(80.6852564373808,-6.72974280712815,1.66644854403216));
#30193=CARTESIAN_POINT('Ctrl Pts',(80.7013537370518,-6.86458158035618,1.12191912096477));
#30194=CARTESIAN_POINT('Ctrl Pts',(80.7174510367228,-6.93300000000028,0.560975745775044));
#30195=CARTESIAN_POINT('Ctrl Pts',(80.7335483363939,-6.933,-3.45320994021847E-12));
#30196=CARTESIAN_POINT('Origin',(29.75,0.,0.));
#30197=CARTESIAN_POINT('',(82.1628916636062,-6.92353455550492,0.00101414875028183));
#30198=CARTESIAN_POINT('',(81.9835483363939,-6.92935402623401,0.00166396505006337));
#30199=CARTESIAN_POINT('',(29.75,-6.933,-8.4904762584886E-16));
#30200=CARTESIAN_POINT('Ctrl Pts',(82.1628916636062,-6.92353455550492,0.00101414875028183));
#30201=CARTESIAN_POINT('Ctrl Pts',(82.1317350410284,-6.92503138592253,1.0907153399273));
#30202=CARTESIAN_POINT('Ctrl Pts',(82.1005784184506,-6.68254061521535,2.17979048906057));
#30203=CARTESIAN_POINT('Ctrl Pts',(82.0694217958728,-6.19243531495591,3.14356638472189));
#30204=CARTESIAN_POINT('Ctrl Pts',(82.0032512610588,-5.15154810863604,5.19043671855075));
#30205=CARTESIAN_POINT('Ctrl Pts',(81.9370807262447,-2.9937856514116,6.67213975217042));
#30206=CARTESIAN_POINT('Ctrl Pts',(81.8709101914307,-0.713310410863843,
6.90806140509355));
#30207=CARTESIAN_POINT('Ctrl Pts',(81.8047396566167,1.56716482968418,7.14398305801671));
#30208=CARTESIAN_POINT('Ctrl Pts',(81.7385691218026,3.97035285355562,6.13412333024305));
#30209=CARTESIAN_POINT('Ctrl Pts',(81.6723985869886,5.41483843060364,4.34349648310992));
#30210=CARTESIAN_POINT('Ctrl Pts',(81.6393133195815,6.13708121912753,3.4481830595435));
#30211=CARTESIAN_POINT('Ctrl Pts',(81.6062280521745,6.61964839594568,2.35767785613726));
#30212=CARTESIAN_POINT('Ctrl Pts',(81.5731427847675,6.82121527266455,1.21993669477338));
#30213=CARTESIAN_POINT('Ctrl Pts',(81.5400575173605,7.02278214938344,0.0821955334093011));
#30214=CARTESIAN_POINT('Ctrl Pts',(81.5069722499535,6.94334872600299,-1.1027815859123));
#30215=CARTESIAN_POINT('Ctrl Pts',(81.4738869825466,6.579940063713,-2.19310910711941));
#30216=CARTESIAN_POINT('Ctrl Pts',(81.4408017151395,6.21653140142307,-3.28343662832634));
#30217=CARTESIAN_POINT('Ctrl Pts',(81.4077164477325,5.56914750022368,-4.27911455141867));
#30218=CARTESIAN_POINT('Ctrl Pts',(81.3746311803254,4.72529340221047,-5.06841450537669));
#30219=CARTESIAN_POINT('Ctrl Pts',(81.3415459129184,3.88143930419715,-5.85771445933481));
#30220=CARTESIAN_POINT('Ctrl Pts',(81.3084606455114,2.84111500936993,-6.4406364441586));
#30221=CARTESIAN_POINT('Ctrl Pts',(81.2753753781044,1.72614853324333,-6.72360380819039));
#30222=CARTESIAN_POINT('Ctrl Pts',(81.2092048432904,-0.503784419009892,
-7.28953853625396));
#30223=CARTESIAN_POINT('Ctrl Pts',(81.1430343084763,-3.03228609646078,-6.65565478114955));
#30224=CARTESIAN_POINT('Ctrl Pts',(81.0768637736623,-4.71520029189113,-5.09872634352341));
#30225=CARTESIAN_POINT('Ctrl Pts',(81.0222064036436,-6.1053003439436,-3.81269149512603));
#30226=CARTESIAN_POINT('Ctrl Pts',(80.9675490336249,-6.91846562125811,-1.89687370018916));
#30227=CARTESIAN_POINT('Ctrl Pts',(80.9128916636062,-6.9365780831978,0.00570569907908797));
#30228=CARTESIAN_POINT('Ctrl Pts',(80.7335483363939,-6.93120482123466,0.00349441528416698));
#30229=CARTESIAN_POINT('Ctrl Pts',(80.786836462586,-6.91342583053146,-1.85300233924437));
#30230=CARTESIAN_POINT('Ctrl Pts',(80.840124588778,-6.15087697410277,-3.71626439473826));
#30231=CARTESIAN_POINT('Ctrl Pts',(80.89341271497,-4.82190773278374,-4.99793256610273));
#30232=CARTESIAN_POINT('Ctrl Pts',(80.959583249784,-3.17166007474918,-6.58944411686849));
#30233=CARTESIAN_POINT('Ctrl Pts',(81.0257537845982,-0.648024325144719,
-7.28417090126887));
#30234=CARTESIAN_POINT('Ctrl Pts',(81.0919243194122,1.58784222942491,-6.76069684274643));
#30235=CARTESIAN_POINT('Ctrl Pts',(81.1580948542262,3.82370878399466,-6.23722278422395));
#30236=CARTESIAN_POINT('Ctrl Pts',(81.2242653890402,5.77180614352961,-4.49554788277849));
#30237=CARTESIAN_POINT('Ctrl Pts',(81.2904359238542,6.54140203412602,-2.33202147781674));
#30238=CARTESIAN_POINT('Ctrl Pts',(81.3566064586682,7.3109979247224,-0.168495072855053));
#30239=CARTESIAN_POINT('Ctrl Pts',(81.4227769934823,6.9020923463804,2.41688283562278));
#30240=CARTESIAN_POINT('Ctrl Pts',(81.4889475282964,5.50458035700961,4.23434991610444));
#30241=CARTESIAN_POINT('Ctrl Pts',(81.5551180631104,4.10706836763878,6.05181699658616));
#30242=CARTESIAN_POINT('Ctrl Pts',(81.6212885979244,1.72094996723906,7.10137324907152));
#30243=CARTESIAN_POINT('Ctrl Pts',(81.6874591327385,-0.572357798069008,
6.91800863538923));
#30244=CARTESIAN_POINT('Ctrl Pts',(81.7205444001455,-1.71901168072304,6.82632632854809));
#30245=CARTESIAN_POINT('Ctrl Pts',(81.7536296675526,-2.84246290460419,6.42641380516503));
#30246=CARTESIAN_POINT('Ctrl Pts',(81.7867149349595,-3.80689731953615,5.79005666067225));
#30247=CARTESIAN_POINT('Ctrl Pts',(81.8198002023665,-4.771331734468,5.15369951617955));
#30248=CARTESIAN_POINT('Ctrl Pts',(81.8528854697735,-5.57674934045072,4.28089775057717));
#30249=CARTESIAN_POINT('Ctrl Pts',(81.8859707371805,-6.11812269421474,3.26709557502076));
#30250=CARTESIAN_POINT('Ctrl Pts',(81.918496603585,-6.65034258419854,2.27043462266962));
#30251=CARTESIAN_POINT('Ctrl Pts',(81.9510224699895,-6.92737158357288,1.13750098159251));
#30252=CARTESIAN_POINT('Ctrl Pts',(81.9835483363939,-6.92935402623401,0.00166396505006337));
#30253=CARTESIAN_POINT('Origin',(29.75,0.,0.));
#30254=CARTESIAN_POINT('',(83.4128916636062,-6.93231962597778,-0.00593826529341535));
#30255=CARTESIAN_POINT('',(83.2335483363939,-6.933,-2.56308863022525E-12));
#30256=CARTESIAN_POINT('',(29.75,-6.933,-8.4904762584886E-16));
#30257=CARTESIAN_POINT('Ctrl Pts',(83.4128916636062,-6.93231962597778,-0.00593826529341535));
#30258=CARTESIAN_POINT('Ctrl Pts',(83.362091583246,-6.9151268553501,1.76512680626223));
#30259=CARTESIAN_POINT('Ctrl Pts',(83.3112915028857,-6.22396082486215,3.54762724591841));
#30260=CARTESIAN_POINT('Ctrl Pts',(83.2604914225255,-5.00363410987313,4.81599105203737));
#30261=CARTESIAN_POINT('Ctrl Pts',(83.1943208877115,-3.41407616417583,6.46812055251247));
#30262=CARTESIAN_POINT('Ctrl Pts',(83.1281503528975,-0.926700730346132,
7.24792360395334));
#30263=CARTESIAN_POINT('Ctrl Pts',(83.0619798180834,1.3323608810027,6.81258037832244));
#30264=CARTESIAN_POINT('Ctrl Pts',(83.0288945506764,2.46189168667719,6.59490876550698));
#30265=CARTESIAN_POINT('Ctrl Pts',(82.9958092832693,3.53434403673139,6.07345058342356));
#30266=CARTESIAN_POINT('Ctrl Pts',(82.9627240158623,4.42265598791498,5.33454190609151));
#30267=CARTESIAN_POINT('Ctrl Pts',(82.9296387484553,5.31096793909847,4.59563322875955));
#30268=CARTESIAN_POINT('Ctrl Pts',(82.8965534810483,6.01513949141133,3.63927405617907));
#30269=CARTESIAN_POINT('Ctrl Pts',(82.8634682136413,6.44131840033896,2.57191680721605));
#30270=CARTESIAN_POINT('Ctrl Pts',(82.8303829462343,6.86749730926663,1.5045595582529));
#30271=CARTESIAN_POINT('Ctrl Pts',(82.7972976788272,7.01568357480899,0.326204232906858));
#30272=CARTESIAN_POINT('Ctrl Pts',(82.7642124114202,6.88059876318932,-0.82133062483032));
#30273=CARTESIAN_POINT('Ctrl Pts',(82.7311271440132,6.74551395156967,-1.96886548256737));
#30274=CARTESIAN_POINT('Ctrl Pts',(82.6980418766062,6.32715806278815,-3.08557987269584));
#30275=CARTESIAN_POINT('Ctrl Pts',(82.6649566091992,5.65818466826036,-4.0213658361549));
#30276=CARTESIAN_POINT('Ctrl Pts',(82.5987860743851,4.32023787920462,-5.89293776307323));
#30277=CARTESIAN_POINT('Ctrl Pts',(82.5326155395711,1.97982106716371,-7.04079598331348));
#30278=CARTESIAN_POINT('Ctrl Pts',(82.466445004757,-0.310512453395021,-6.93784592903852));
#30279=CARTESIAN_POINT('Ctrl Pts',(82.400274469943,-2.60084597395362,-6.83489587476358));
#30280=CARTESIAN_POINT('Ctrl Pts',(82.334103935129,-4.84109620302989,-5.48113754597357));
#30281=CARTESIAN_POINT('Ctrl Pts',(82.267933400315,-5.99921533986046,-3.4982395645595));
#30282=CARTESIAN_POINT('Ctrl Pts',(82.2329194880787,-6.61203012109301,-2.4489958779279));
#30283=CARTESIAN_POINT('Ctrl Pts',(82.1979055758425,-6.9218524126878,-1.22359553981082));
#30284=CARTESIAN_POINT('Ctrl Pts',(82.1628916636062,-6.92353455550492,0.00101414875028183));
#30285=CARTESIAN_POINT('Ctrl Pts',(81.9835483363939,-6.92935402623401,0.00166396505006337));
#30286=CARTESIAN_POINT('Ctrl Pts',(81.9841077373965,-6.92938812157212,-0.0178708986160241));
#30287=CARTESIAN_POINT('Ctrl Pts',(81.9846671383991,-6.92934085990654,-0.0374066210819144));
#30288=CARTESIAN_POINT('Ctrl Pts',(81.9852265394017,-6.92921214022652,-0.056942523864537));
#30289=CARTESIAN_POINT('Ctrl Pts',(82.0183118068087,-6.92159913092891,-1.21237586168268));
#30290=CARTESIAN_POINT('Ctrl Pts',(82.0513970742157,-6.62904401078835,-2.36843995180839));
#30291=CARTESIAN_POINT('Ctrl Pts',(82.0844823416227,-6.06743435498427,-3.37234002975485));
#30292=CARTESIAN_POINT('Ctrl Pts',(82.1506528764367,-4.94421504337618,-5.38014018564764));
#30293=CARTESIAN_POINT('Ctrl Pts',(82.2168234112508,-2.74477758911402,-6.77928429282362));
#30294=CARTESIAN_POINT('Ctrl Pts',(82.2829939460648,-0.457073205771369,
-6.92973363148655));
#30295=CARTESIAN_POINT('Ctrl Pts',(82.3491644808789,1.83063117757141,-7.08018297014949));
#30296=CARTESIAN_POINT('Ctrl Pts',(82.4153350156929,4.20660248999483,-5.98193754029923));
#30297=CARTESIAN_POINT('Ctrl Pts',(82.4815055505069,5.57648760428372,-4.1389673524125));
#30298=CARTESIAN_POINT('Ctrl Pts',(82.5476760853209,6.94637271857261,-2.29599716452578));
#30299=CARTESIAN_POINT('Ctrl Pts',(82.613846620135,7.31017163472707,0.291697781397146));
#30300=CARTESIAN_POINT('Ctrl Pts',(82.680017154949,6.50154387995514,2.44094078627165));
#30301=CARTESIAN_POINT('Ctrl Pts',(82.7461876897631,5.6929161251832,4.59018379114616));
#30302=CARTESIAN_POINT('Ctrl Pts',(82.8123582245771,3.7118616994847,6.30097485497203));
#30303=CARTESIAN_POINT('Ctrl Pts',(82.8785287593911,1.47135462991242,6.78713781146553));
#30304=CARTESIAN_POINT('Ctrl Pts',(82.9446992942052,-0.769152439659738,
7.27330076795901));
#30305=CARTESIAN_POINT('Ctrl Pts',(83.0108698290192,-3.26911215310578,6.5348356171203));
#30306=CARTESIAN_POINT('Ctrl Pts',(83.0770403638333,-4.902394538607,4.91456658477292));
#30307=CARTESIAN_POINT('Ctrl Pts',(83.1101256312403,-5.71903573135766,4.10443206859918));
#30308=CARTESIAN_POINT('Ctrl Pts',(83.1432108986473,-6.31900759212212,3.07384658204822));
#30309=CARTESIAN_POINT('Ctrl Pts',(83.1762961660543,-6.64490887109431,1.96530135860606));
#30310=CARTESIAN_POINT('Ctrl Pts',(83.1953802228341,-6.83289340318271,1.32587657394482));
#30311=CARTESIAN_POINT('Ctrl Pts',(83.214464279614,-6.92969060024565,0.660513432091375));
#30312=CARTESIAN_POINT('Ctrl Pts',(83.2335483363938,-6.93172781140961,-0.00378750055469096));
#30313=CARTESIAN_POINT('Origin',(29.75,0.,0.));
#30314=CARTESIAN_POINT('',(84.6628916636062,-6.94340481590983,0.0048587949936791));
#30315=CARTESIAN_POINT('',(84.4835483363939,-6.93470434732279,0.000299062045973509));
#30316=CARTESIAN_POINT('',(29.75,-6.933,-8.4904762584886E-16));
#30317=CARTESIAN_POINT('Ctrl Pts',(84.6628916636062,-6.94340481590983,0.0048587949936791));
#30318=CARTESIAN_POINT('Ctrl Pts',(84.6586186602776,-6.94414319679649,0.153029414161253));
#30319=CARTESIAN_POINT('Ctrl Pts',(84.6543456569489,-6.93981013338403,0.301132648058085));
#30320=CARTESIAN_POINT('Ctrl Pts',(84.6500726536203,-6.93026956754333,0.44887396891849));
#30321=CARTESIAN_POINT('Ctrl Pts',(84.5839021188062,-6.78252703247977,2.73675475523645));
#30322=CARTESIAN_POINT('Ctrl Pts',(84.5177315839921,-5.38598616984263,4.93784606793614));
#30323=CARTESIAN_POINT('Ctrl Pts',(84.4515610491781,-3.37951635660294,6.06344012288267));
#30324=CARTESIAN_POINT('Ctrl Pts',(84.4184757817711,-2.3762814499831,6.62623715035594));
#30325=CARTESIAN_POINT('Ctrl Pts',(84.3853905143641,-1.22056430571257,6.92015986339094));
#30326=CARTESIAN_POINT('Ctrl Pts',(84.3523052469571,-0.0651407839431917,
6.92913991874561));
#30327=CARTESIAN_POINT('Ctrl Pts',(84.3192199795501,1.09028273782619,6.93811997410028));
#30328=CARTESIAN_POINT('Ctrl Pts',(84.2861347121431,2.2454126370945,6.66215737177462));
#30329=CARTESIAN_POINT('Ctrl Pts',(84.2530494447361,3.2598546291538,6.12198387735301));
#30330=CARTESIAN_POINT('Ctrl Pts',(84.219964177329,4.2742966212131,5.5818103829314));
#30331=CARTESIAN_POINT('Ctrl Pts',(84.186878909922,5.14805070606347,4.7774259964138));
#30332=CARTESIAN_POINT('Ctrl Pts',(84.1537936425149,5.78554847609396,3.8137451627047));
#30333=CARTESIAN_POINT('Ctrl Pts',(84.1207083751079,6.42304624612438,2.85006432899571));
#30334=CARTESIAN_POINT('Ctrl Pts',(84.0876231077009,6.82428770133504,1.72708704809516));
#30335=CARTESIAN_POINT('Ctrl Pts',(84.0545378402939,6.91732660797555,0.580542441965909));
#30336=CARTESIAN_POINT('Ctrl Pts',(83.9883673054799,7.1034044212566,-1.71254677029273));
#30337=CARTESIAN_POINT('Ctrl Pts',(83.9221967706659,6.05667204025721,-4.09990528346618));
#30338=CARTESIAN_POINT('Ctrl Pts',(83.8560262358518,4.2408596986948,-5.49956663154253));
#30339=CARTESIAN_POINT('Ctrl Pts',(83.7898557010378,2.42504735713218,-6.89922797961903));
#30340=CARTESIAN_POINT('Ctrl Pts',(83.7236851662237,-0.159844944993682,
-7.31119216259787));
#30341=CARTESIAN_POINT('Ctrl Pts',(83.6575146314097,-2.32428038332007,-6.54415658773383));
#30342=CARTESIAN_POINT('Ctrl Pts',(83.5913440965957,-4.48871582164609,-5.77712101286992));
#30343=CARTESIAN_POINT('Ctrl Pts',(83.5251735617817,-6.2326943961729,-3.8310856801635));
#30344=CARTESIAN_POINT('Ctrl Pts',(83.4590030269676,-6.75881345465409,-1.59584003905574));
#30345=CARTESIAN_POINT('Ctrl Pts',(83.4436325725138,-6.88102327279128,-1.07662493196513));
#30346=CARTESIAN_POINT('Ctrl Pts',(83.42826211806,-6.9375215999903,-0.541805036054968));
#30347=CARTESIAN_POINT('Ctrl Pts',(83.4128916636062,-6.93231962597778,-0.00593826529341535));
#30348=CARTESIAN_POINT('Ctrl Pts',(83.2335483363939,-6.933,-2.56308863022525E-12));
#30349=CARTESIAN_POINT('Ctrl Pts',(83.290772531679,-6.93299999999926,-1.99420935701877));
#30350=CARTESIAN_POINT('Ctrl Pts',(83.347996726964,-6.02307502629109,-3.97063309653254));
#30351=CARTESIAN_POINT('Ctrl Pts',(83.4052209222491,-4.50798484753805,-5.26731066241278));
#30352=CARTESIAN_POINT('Ctrl Pts',(83.4624451175342,-2.99289466878501,-6.56398822829301));
#30353=CARTESIAN_POINT('Ctrl Pts',(83.5196693128193,-0.899664345626491,
-7.15779044292437));
#30354=CARTESIAN_POINT('Ctrl Pts',(83.5768935081044,1.07062371682059,-6.84983604599273));
#30355=CARTESIAN_POINT('Ctrl Pts',(83.6341177033895,3.04091177926767,-6.54188164906108));
#30356=CARTESIAN_POINT('Ctrl Pts',(83.6913418986746,4.85311303640036,-5.33766370386257));
#30357=CARTESIAN_POINT('Ctrl Pts',(83.7485660939597,5.90026971493865,-3.64050907030567));
#30358=CARTESIAN_POINT('Ctrl Pts',(83.8057902892448,6.94742639347693,-1.94335443674876));
#30359=CARTESIAN_POINT('Ctrl Pts',(83.8630144845299,7.21086008527503,0.216464293125819));
#30360=CARTESIAN_POINT('Ctrl Pts',(83.920238679815,6.60233935006029,2.11556236179545));
#30361=CARTESIAN_POINT('Ctrl Pts',(83.9774628751001,5.99381861484554,4.01466043046508));
#30362=CARTESIAN_POINT('Ctrl Pts',(84.0346870703851,4.52419779647164,5.61916312790545));
#30363=CARTESIAN_POINT('Ctrl Pts',(84.0919112656702,2.6856947300026,6.39167683923681));
#30364=CARTESIAN_POINT('Ctrl Pts',(84.1491354609553,0.84719166353356,7.16419055056817));
#30365=CARTESIAN_POINT('Ctrl Pts',(84.2063596562404,-1.32739978994314,7.09093574623758));
#30366=CARTESIAN_POINT('Ctrl Pts',(84.2635838515255,-3.10974706736312,6.19644754492657));
#30367=CARTESIAN_POINT('Ctrl Pts',(84.3208080468106,-4.89209434478309,5.30195934361556));
#30368=CARTESIAN_POINT('Ctrl Pts',(84.3780322420957,-6.25040525058716,3.60219296582561));
#30369=CARTESIAN_POINT('Ctrl Pts',(84.4352564373808,-6.7297428071279,1.66644854403317));
#30370=CARTESIAN_POINT('Ctrl Pts',(84.4513537370518,-6.86458158035605,1.12191912096567));
#30371=CARTESIAN_POINT('Ctrl Pts',(84.4674510367228,-6.93300000000023,0.560975745775821));
#30372=CARTESIAN_POINT('Ctrl Pts',(84.4835483363939,-6.933,-2.8078928071551E-12));
#30373=CARTESIAN_POINT('Origin',(29.75,0.,0.));
#30374=CARTESIAN_POINT('',(85.9128916636062,-6.92777016594518,0.000431384726357015));
#30375=CARTESIAN_POINT('',(85.7335483363939,-6.92921246598513,0.00257278641648163));
#30376=CARTESIAN_POINT('',(29.75,-6.933,-8.4904762584886E-16));
#30377=CARTESIAN_POINT('Ctrl Pts',(85.9128916636062,-6.92137817579339,0.000958630302984043));
#30378=CARTESIAN_POINT('Ctrl Pts',(85.8889752024951,-6.92604506083378,0.836427548270157));
#30379=CARTESIAN_POINT('Ctrl Pts',(85.8650587413841,-6.78625928845202,1.67113888616492));
#30380=CARTESIAN_POINT('Ctrl Pts',(85.841142280273,-6.49492932481831,2.44996530464116));
#30381=CARTESIAN_POINT('Ctrl Pts',(85.8080570128659,-6.0919127704156,3.52736886360613));
#30382=CARTESIAN_POINT('Ctrl Pts',(85.7749717454589,-5.39888502526939,4.497825056979));
#30383=CARTESIAN_POINT('Ctrl Pts',(85.7418864780518,-4.52216542065837,5.25045171804183));
#30384=CARTESIAN_POINT('Ctrl Pts',(85.7088012106448,-3.64544581604724,6.00307837910473));
#30385=CARTESIAN_POINT('Ctrl Pts',(85.6757159432379,-2.58503435197131,6.53787550785749));
#30386=CARTESIAN_POINT('Ctrl Pts',(85.6426306758309,-1.4615458932431,6.78006064867637));
#30387=CARTESIAN_POINT('Ctrl Pts',(85.6095454084239,-0.338057434515012,
7.02224578949523));
#30388=CARTESIAN_POINT('Ctrl Pts',(85.5764601410168,0.84850801886527,6.97181894238025));
#30389=CARTESIAN_POINT('Ctrl Pts',(85.5433748736098,1.9574380566315,6.64722946720943));
#30390=CARTESIAN_POINT('Ctrl Pts',(85.5102896062027,3.06636809439786,6.32263999203856));
#30391=CARTESIAN_POINT('Ctrl Pts',(85.4772043387958,4.09766271655007,5.72388788881181));
#30392=CARTESIAN_POINT('Ctrl Pts',(85.4441190713888,4.90876287502491,4.90820577860255));
#30393=CARTESIAN_POINT('Ctrl Pts',(85.3779485365747,6.5309631919745,3.27684155818413));
#30394=CARTESIAN_POINT('Ctrl Pts',(85.3117780017607,7.27238565421453,0.777757309835552));
#30395=CARTESIAN_POINT('Ctrl Pts',(85.2456074669466,6.78887389477455,-1.46332339543877));
#30396=CARTESIAN_POINT('Ctrl Pts',(85.1794369321326,6.30536213533455,-3.70440410071322));
#30397=CARTESIAN_POINT('Ctrl Pts',(85.1132663973185,4.59691615421462,-5.68748126291356));
#30398=CARTESIAN_POINT('Ctrl Pts',(85.0470958625045,2.44863138187429,-6.49865132937342));
#30399=CARTESIAN_POINT('Ctrl Pts',(84.9809253276904,0.300346609533963,-7.30982139583328));
#30400=CARTESIAN_POINT('Ctrl Pts',(84.9147547928764,-2.28777695402661,-6.94908436655257));
#30401=CARTESIAN_POINT('Ctrl Pts',(84.8485842580624,-4.13236663206187,-5.581380721944));
#30402=CARTESIAN_POINT('Ctrl Pts',(84.786686726577,-5.8578407875103,-4.30199738851975));
#30403=CARTESIAN_POINT('Ctrl Pts',(84.7247891950916,-6.93270883683727,-2.14149936570948));
#30404=CARTESIAN_POINT('Ctrl Pts',(84.6628916636062,-6.94340481590983,0.0048587949936791));
#30405=CARTESIAN_POINT('Ctrl Pts',(84.4835483363939,-6.94155004985185,0.00150027839546349));
#30406=CARTESIAN_POINT('Ctrl Pts',(84.5109913566456,-6.93928989654419,-0.953521174230491));
#30407=CARTESIAN_POINT('Ctrl Pts',(84.5384343768973,-6.73091917705912,-1.91105609676861));
#30408=CARTESIAN_POINT('Ctrl Pts',(84.5658773971491,-6.34390333657409,-2.78785110640628));
#30409=CARTESIAN_POINT('Ctrl Pts',(84.5989626645561,-5.87731757248042,-3.84491396205739));
#30410=CARTESIAN_POINT('Ctrl Pts',(84.6320479319631,-5.15107683485604,-4.78462393491109));
#30411=CARTESIAN_POINT('Ctrl Pts',(84.6651331993701,-4.24177091760061,-5.48750565196823));
#30412=CARTESIAN_POINT('Ctrl Pts',(84.6982184667772,-3.33246500034529,-6.19038736902529));
#30413=CARTESIAN_POINT('Ctrl Pts',(84.7313037341842,-2.24009390345898,-6.65644083028586));
#30414=CARTESIAN_POINT('Ctrl Pts',(84.7643890015912,-1.09957551318182,-6.84164870671519));
#30415=CARTESIAN_POINT('Ctrl Pts',(84.7974742689982,0.0409428770954647,
-7.02685658314454));
#30416=CARTESIAN_POINT('Ctrl Pts',(84.8305595364052,1.2296085607636,-6.93121887474259));
#30417=CARTESIAN_POINT('Ctrl Pts',(84.8636448038122,2.31311716204457,-6.54491603635869));
#30418=CARTESIAN_POINT('Ctrl Pts',(84.9298153386262,4.48013436460651,-5.7723103595909));
#30419=CARTESIAN_POINT('Ctrl Pts',(84.9959858734404,6.22652323761978,-3.83704416289533));
#30420=CARTESIAN_POINT('Ctrl Pts',(85.0621564082544,6.7564304231043,-1.6064781531476));
#30421=CARTESIAN_POINT('Ctrl Pts',(85.1283269430685,7.28633760858878,0.624087856599996));
#30422=CARTESIAN_POINT('Ctrl Pts',(85.1944974778824,6.59976310654463,3.14995367939972));
#30423=CARTESIAN_POINT('Ctrl Pts',(85.2606680126964,5.01109087012319,4.80803837717989));
#30424=CARTESIAN_POINT('Ctrl Pts',(85.3268385475104,3.42241863370165,6.46612307496015));
#30425=CARTESIAN_POINT('Ctrl Pts',(85.3930090823246,0.931648662902707,7.25642664772076));
#30426=CARTESIAN_POINT('Ctrl Pts',(85.4591796171386,-1.32235953455869,6.81759708448866));
#30427=CARTESIAN_POINT('Ctrl Pts',(85.5253501519526,-3.57636773201997,6.37876752125658));
#30428=CARTESIAN_POINT('Ctrl Pts',(85.5915206867667,-5.59361415614373,4.71080482203193));
#30429=CARTESIAN_POINT('Ctrl Pts',(85.6576912215807,-6.44666043474205,2.58276854517033));
#30430=CARTESIAN_POINT('Ctrl Pts',(85.6829769265184,-6.77263447378339,1.76958337831761));
#30431=CARTESIAN_POINT('Ctrl Pts',(85.7082626314561,-6.92860868119207,0.889216953124101));
#30432=CARTESIAN_POINT('Ctrl Pts',(85.7335483363939,-6.9229639019227,0.00681729503297956));
#30433=CARTESIAN_POINT('Origin',(29.75,0.,0.));
#30434=CARTESIAN_POINT('',(87.1628916636062,-6.93297740291849,-0.000166944099082397));
#30435=CARTESIAN_POINT('',(86.9835483363939,-6.93072156200529,-0.00296430948166657));
#30436=CARTESIAN_POINT('',(29.75,-6.933,-8.4904762584886E-16));
#30437=CARTESIAN_POINT('Ctrl Pts',(87.1628916636062,-6.933,2.97289970419001E-12));
#30438=CARTESIAN_POINT('Ctrl Pts',(87.1056674683211,-6.93299999999915,1.99420935701932));
#30439=CARTESIAN_POINT('Ctrl Pts',(87.048443273036,-6.02307502629073,3.97063309653316));
#30440=CARTESIAN_POINT('Ctrl Pts',(86.9912190777509,-4.50798484753744,5.2673106624133));
#30441=CARTESIAN_POINT('Ctrl Pts',(86.9339948824658,-2.99289466878415,6.56398822829345));
#30442=CARTESIAN_POINT('Ctrl Pts',(86.8767706871807,-0.899664345625384,
7.15779044292455));
#30443=CARTESIAN_POINT('Ctrl Pts',(86.8195464918956,1.07062371682177,6.84983604599254));
#30444=CARTESIAN_POINT('Ctrl Pts',(86.7623222966105,3.04091177926893,6.54188164906054));
#30445=CARTESIAN_POINT('Ctrl Pts',(86.7050981013254,4.85311303640152,5.33766370386157));
#30446=CARTESIAN_POINT('Ctrl Pts',(86.6478739060403,5.90026971493948,3.64050907030431));
#30447=CARTESIAN_POINT('Ctrl Pts',(86.5906497107552,6.94742639347745,1.94335443674705));
#30448=CARTESIAN_POINT('Ctrl Pts',(86.5334255154701,7.210860085275,-0.21646429312776));
#30449=CARTESIAN_POINT('Ctrl Pts',(86.476201320185,6.60233935005968,-2.11556236179734));
#30450=CARTESIAN_POINT('Ctrl Pts',(86.4189771248999,5.99381861484435,-4.01466043046692));
#30451=CARTESIAN_POINT('Ctrl Pts',(86.3617529296148,4.52419779646983,-5.61916312790696));
#30452=CARTESIAN_POINT('Ctrl Pts',(86.3045287343297,2.6856947300004,-6.39167683923773));
#30453=CARTESIAN_POINT('Ctrl Pts',(86.2473045390446,0.847191663530979,-7.16419055056851));
#30454=CARTESIAN_POINT('Ctrl Pts',(86.1900803437595,-1.32739978994586,-7.09093574623711));
#30455=CARTESIAN_POINT('Ctrl Pts',(86.1328561484744,-3.10974706736559,-6.19644754492533));
#30456=CARTESIAN_POINT('Ctrl Pts',(86.0756319531893,-4.89209434478533,-5.30195934361354));
#30457=CARTESIAN_POINT('Ctrl Pts',(86.0184077579042,-6.25040525058877,-3.60219296582288));
#30458=CARTESIAN_POINT('Ctrl Pts',(85.9611835626191,-6.72974280712866,-1.66644854403009));
#30459=CARTESIAN_POINT('Ctrl Pts',(85.9450862629482,-6.86458158035627,-1.12191912096368));
#30460=CARTESIAN_POINT('Ctrl Pts',(85.9289889632772,-6.9330000000002,-0.560975745775017));
#30461=CARTESIAN_POINT('Ctrl Pts',(85.9128916636062,-6.933,2.429445533636E-12));
#30462=CARTESIAN_POINT('Ctrl Pts',(85.7335483363939,-6.933,-3.05241942832879E-12));
#30463=CARTESIAN_POINT('Ctrl Pts',(85.790772531679,-6.93299999999912,-1.99420935701939));
#30464=CARTESIAN_POINT('Ctrl Pts',(85.8479967269641,-6.02307502629068,-3.97063309653323));
#30465=CARTESIAN_POINT('Ctrl Pts',(85.9052209222492,-4.50798484753738,-5.26731066241335));
#30466=CARTESIAN_POINT('Ctrl Pts',(85.9624451175343,-2.99289466878407,-6.56398822829348));
#30467=CARTESIAN_POINT('Ctrl Pts',(86.0196693128193,-0.899664345625303,
-7.15779044292456));
#30468=CARTESIAN_POINT('Ctrl Pts',(86.0768935081044,1.07062371682185,-6.84983604599253));
#30469=CARTESIAN_POINT('Ctrl Pts',(86.1341177033895,3.04091177926901,-6.5418816490605));
#30470=CARTESIAN_POINT('Ctrl Pts',(86.1913418986746,4.85311303640158,-5.33766370386151));
#30471=CARTESIAN_POINT('Ctrl Pts',(86.2485660939597,5.90026971493953,-3.64050907030424));
#30472=CARTESIAN_POINT('Ctrl Pts',(86.3057902892448,6.94742639347747,-1.94335443674697));
#30473=CARTESIAN_POINT('Ctrl Pts',(86.3630144845299,7.210860085275,0.216464293127843));
#30474=CARTESIAN_POINT('Ctrl Pts',(86.420238679815,6.60233935005965,2.11556236179742));
#30475=CARTESIAN_POINT('Ctrl Pts',(86.4774628751001,5.99381861484431,4.01466043046699));
#30476=CARTESIAN_POINT('Ctrl Pts',(86.5346870703852,4.52419779646977,5.61916312790701));
#30477=CARTESIAN_POINT('Ctrl Pts',(86.5919112656703,2.68569473000033,6.39167683923776));
#30478=CARTESIAN_POINT('Ctrl Pts',(86.6491354609554,0.847191663530897,7.16419055056852));
#30479=CARTESIAN_POINT('Ctrl Pts',(86.7063596562405,-1.32739978994594,7.09093574623709));
#30480=CARTESIAN_POINT('Ctrl Pts',(86.7635838515256,-3.10974706736567,6.19644754492529));
#30481=CARTESIAN_POINT('Ctrl Pts',(86.8208080468107,-4.89209434478539,5.30195934361348));
#30482=CARTESIAN_POINT('Ctrl Pts',(86.8780322420958,-6.25040525058881,3.60219296582281));
#30483=CARTESIAN_POINT('Ctrl Pts',(86.9352564373809,-6.72974280712868,1.66644854403002));
#30484=CARTESIAN_POINT('Ctrl Pts',(86.9513537370519,-6.86458158035632,1.12191912096348));
#30485=CARTESIAN_POINT('Ctrl Pts',(86.9674510367229,-6.93300000000024,0.560975745774675));
#30486=CARTESIAN_POINT('Ctrl Pts',(86.9835483363939,-6.933,-2.90281687576055E-12));
#30487=CARTESIAN_POINT('Origin',(29.75,0.,0.));
#30488=CARTESIAN_POINT('',(88.4128916636062,-6.935505181738,-0.00110020350931883));
#30489=CARTESIAN_POINT('',(88.2335483363938,-6.94458427852422,-0.00039025483562369));
#30490=CARTESIAN_POINT('',(29.75,-6.933,-8.4904762584886E-16));
#30491=CARTESIAN_POINT('Ctrl Pts',(88.4128916636062,-6.935505181738,-0.00110020350931883));
#30492=CARTESIAN_POINT('Ctrl Pts',(88.3827735543372,-6.93378070856149,1.04526965719805));
#30493=CARTESIAN_POINT('Ctrl Pts',(88.3526554450683,-6.68734941614985,2.09265228946978));
#30494=CARTESIAN_POINT('Ctrl Pts',(88.3225373357993,-6.2276382020042,3.03870790965906));
#30495=CARTESIAN_POINT('Ctrl Pts',(88.2894520683923,-5.72263742940609,4.07796647985569));
#30496=CARTESIAN_POINT('Ctrl Pts',(88.2563668009853,-4.96026313710671,4.99494964068218));
#30497=CARTESIAN_POINT('Ctrl Pts',(88.2232815335783,-4.02072362537253,5.65864104328076));
#30498=CARTESIAN_POINT('Ctrl Pts',(88.1571109987643,-2.14164460190385,6.98602384847814));
#30499=CARTESIAN_POINT('Ctrl Pts',(88.0909404639502,0.446095299304411,7.30023962076365));
#30500=CARTESIAN_POINT('Ctrl Pts',(88.0247699291362,2.57513936872885,6.44971172614812));
#30501=CARTESIAN_POINT('Ctrl Pts',(87.9585993943221,4.70418343815292,5.59918383153274));
#30502=CARTESIAN_POINT('Ctrl Pts',(87.8924288595081,6.37453167579348,3.5839122700167));
#30503=CARTESIAN_POINT('Ctrl Pts',(87.8262583246941,6.81602776252033,1.33042485154879));
#30504=CARTESIAN_POINT('Ctrl Pts',(87.76008778988,7.25752384924726,-0.923062566919503));
#30505=CARTESIAN_POINT('Ctrl Pts',(87.6939172550659,6.47016778506027,-3.41476584233957));
#30506=CARTESIAN_POINT('Ctrl Pts',(87.6277467202519,4.81396388596147,-5.00539873034359));
#30507=CARTESIAN_POINT('Ctrl Pts',(87.5615761854379,3.15775998686276,-6.59603161834753));
#30508=CARTESIAN_POINT('Ctrl Pts',(87.4954056506239,0.632708252852293,-7.28559411893525));
#30509=CARTESIAN_POINT('Ctrl Pts',(87.4292351158099,-1.59848315555634,-6.75832639935306));
#30510=CARTESIAN_POINT('Ctrl Pts',(87.3630645809958,-3.82967456396472,-6.23105867977093));
#30511=CARTESIAN_POINT('Ctrl Pts',(87.2968940461817,-5.76700564677146,-4.48696074001916));
#30512=CARTESIAN_POINT('Ctrl Pts',(87.2307235113677,-6.54217468998849,-2.32085916289729));
#30513=CARTESIAN_POINT('Ctrl Pts',(87.2081128954472,-6.80705164101982,-1.58069753442065));
#30514=CARTESIAN_POINT('Ctrl Pts',(87.1855022795267,-6.93623411182673,-0.79126260129709));
#30515=CARTESIAN_POINT('Ctrl Pts',(87.1628916636062,-6.93279839181025,-0.00148945332221512));
#30516=CARTESIAN_POINT('Ctrl Pts',(86.9835483363939,-6.92663006290457,-0.00828746050336714));
#30517=CARTESIAN_POINT('Ctrl Pts',(87.0047897084878,-6.93231836757728,-0.750014360114233));
#30518=CARTESIAN_POINT('Ctrl Pts',(87.0260310805816,-6.82278736112151,-1.48975226235973));
#30519=CARTESIAN_POINT('Ctrl Pts',(87.0472724526755,-6.59102457491306,-2.18826853280899));
#30520=CARTESIAN_POINT('Ctrl Pts',(87.1134429874895,-5.86904355383633,-4.36426709766948));
#30521=CARTESIAN_POINT('Ctrl Pts',(87.1796135223035,-3.96088883031357,-6.1402386343094));
#30522=CARTESIAN_POINT('Ctrl Pts',(87.2457840571176,-1.73486522229777,-6.72135995084269));
#30523=CARTESIAN_POINT('Ctrl Pts',(87.2788693245246,-0.62185341828987,-7.01192060910934));
#30524=CARTESIAN_POINT('Ctrl Pts',(87.3119545919317,0.570625606841345,-7.00376871234934));
#30525=CARTESIAN_POINT('Ctrl Pts',(87.3450398593387,1.69070331343781,-6.72002571730325));
#30526=CARTESIAN_POINT('Ctrl Pts',(87.3781251267457,2.81078102003415,-6.43628272225719));
#30527=CARTESIAN_POINT('Ctrl Pts',(87.4112103941527,3.85845740809585,-5.87694862892509));
#30528=CARTESIAN_POINT('Ctrl Pts',(87.4442956615597,4.70315627451569,-5.0976131527676));
#30529=CARTESIAN_POINT('Ctrl Pts',(87.4773809289667,5.54785514093573,-4.31827767660994));
#30530=CARTESIAN_POINT('Ctrl Pts',(87.5104661963738,6.18957648571371,-3.3189408176271));
#30531=CARTESIAN_POINT('Ctrl Pts',(87.5435514637808,6.5624166537896,-2.22528896940409));
#30532=CARTESIAN_POINT('Ctrl Pts',(87.5766367311878,6.93525682186541,-1.13163712118134));
#30533=CARTESIAN_POINT('Ctrl Pts',(87.6097219985948,7.03921581323902,0.0563297162812662));
#30534=CARTESIAN_POINT('Ctrl Pts',(87.6428072660018,6.83904205674447,1.18909237421267));
#30535=CARTESIAN_POINT('Ctrl Pts',(87.7089778008158,6.43869454375532,3.45461769007573));
#30536=CARTESIAN_POINT('Ctrl Pts',(87.7751483356299,4.8218160392931,5.49932628781417));
#30537=CARTESIAN_POINT('Ctrl Pts',(87.8413188704439,2.71087765477093,6.39384598341667));
#30538=CARTESIAN_POINT('Ctrl Pts',(87.907489405258,0.599939270248752,7.28836567901917));
#30539=CARTESIAN_POINT('Ctrl Pts',(87.9736599400721,-2.00505899433351,7.0326964724858));
#30540=CARTESIAN_POINT('Ctrl Pts',(88.0398304748861,-3.90489207377941,5.74282880096571));
#30541=CARTESIAN_POINT('Ctrl Pts',(88.1044030953886,-5.75884717331272,4.48410940439889));
#30542=CARTESIAN_POINT('Ctrl Pts',(88.1689757158912,-6.94128313269814,2.24053698532216));
#30543=CARTESIAN_POINT('Ctrl Pts',(88.2335483363938,-6.94458427852422,-0.00039025483562369));
#30544=CARTESIAN_POINT('Origin',(29.75,0.,0.));
#30545=CARTESIAN_POINT('',(89.6628916636062,-6.93366901110661,0.000560428832954156));
#30546=CARTESIAN_POINT('',(89.4835483363938,-6.93167766374453,0.00562466873832855));
#30547=CARTESIAN_POINT('',(29.75,-6.933,-8.4904762584886E-16));
#30548=CARTESIAN_POINT('Ctrl Pts',(89.6628916636062,-6.93602175126458,0.00253131295903153));
#30549=CARTESIAN_POINT('Ctrl Pts',(89.6462153639618,-6.93907490126647,0.584461471238139));
#30550=CARTESIAN_POINT('Ctrl Pts',(89.6295390643174,-6.86919820701986,1.1657362249708));
#30551=CARTESIAN_POINT('Ctrl Pts',(89.612862764673,-6.72340785284693,1.72691162848786));
#30552=CARTESIAN_POINT('Ctrl Pts',(89.5466922298589,-6.14492066371759,3.95362123236213));
#30553=CARTESIAN_POINT('Ctrl Pts',(89.480521695045,-4.37120800409507,5.86387586171152));
#30554=CARTESIAN_POINT('Ctrl Pts',(89.4143511602309,-2.19606517438035,6.58843091097293));
#30555=CARTESIAN_POINT('Ctrl Pts',(89.3481806254169,-0.020922344665516,
7.31298596023438));
#30556=CARTESIAN_POINT('Ctrl Pts',(89.2820100906029,2.55565065514142,6.85184142940768));
#30557=CARTESIAN_POINT('Ctrl Pts',(89.2158395557888,4.34737921445182,5.41558479859921));
#30558=CARTESIAN_POINT('Ctrl Pts',(89.1496690209748,6.13910777376212,3.97932816779082));
#30559=CARTESIAN_POINT('Ctrl Pts',(89.0834984861608,7.14599189257585,1.56795943700085));
#30560=CARTESIAN_POINT('Ctrl Pts',(89.0173279513468,6.90765202347533,-0.715966666573044));
#30561=CARTESIAN_POINT('Ctrl Pts',(88.9511574165327,6.66931215437481,-2.99989277014694));
#30562=CARTESIAN_POINT('Ctrl Pts',(88.8849868817187,5.18574829735977,-5.15637624650502));
#30563=CARTESIAN_POINT('Ctrl Pts',(88.8188163469046,3.14123319515043,-6.19376929926154));
#30564=CARTESIAN_POINT('Ctrl Pts',(88.7526458120905,1.0967180929411,-7.23116235201807));
#30565=CARTESIAN_POINT('Ctrl Pts',(88.6864752772765,-1.50874825446258,-7.14946498117337));
#30566=CARTESIAN_POINT('Ctrl Pts',(88.6203047424625,-3.49893401082527,-5.99532298681402));
#30567=CARTESIAN_POINT('Ctrl Pts',(88.5872194750555,-4.49402688900667,-5.41825198963431));
#30568=CARTESIAN_POINT('Ctrl Pts',(88.5541342076485,-5.33529961942776,-4.57306983657593));
#30569=CARTESIAN_POINT('Ctrl Pts',(88.5210489402415,-5.93115617306285,-3.58310058273908));
#30570=CARTESIAN_POINT('Ctrl Pts',(88.4879636728344,-6.52701272669794,-2.59313132890222));
#30571=CARTESIAN_POINT('Ctrl Pts',(88.4548784054274,-6.87745310354699,-1.45837497428694));
#30572=CARTESIAN_POINT('Ctrl Pts',(88.4217931380204,-6.9288596655231,-0.3102298071958));
#30573=CARTESIAN_POINT('Ctrl Pts',(88.4188259798823,-6.93346991687278,-0.207261672336488));
#30574=CARTESIAN_POINT('Ctrl Pts',(88.4158588217443,-6.93567507237004,-0.104185852741362));
#30575=CARTESIAN_POINT('Ctrl Pts',(88.4128916636062,-6.935505181738,-0.00110020350931883));
#30576=CARTESIAN_POINT('Ctrl Pts',(88.2335483363938,-6.94458427852422,-0.00039025483562369));
#30577=CARTESIAN_POINT('Ctrl Pts',(88.2351462507052,-6.94466596869133,-0.0558442488051521));
#30578=CARTESIAN_POINT('Ctrl Pts',(88.2367441650167,-6.94402559831809,-0.111296622960476));
#30579=CARTESIAN_POINT('Ctrl Pts',(88.2383420793281,-6.94265547521014,-0.166732413169323));
#30580=CARTESIAN_POINT('Ctrl Pts',(88.3045126141421,-6.88591790288544,-2.46235981927781));
#30581=CARTESIAN_POINT('Ctrl Pts',(88.3706831489563,-5.57777486392631,-4.72954849498799));
#30582=CARTESIAN_POINT('Ctrl Pts',(88.4368536837703,-3.62182626347297,-5.92558002528084));
#30583=CARTESIAN_POINT('Ctrl Pts',(88.5030242185843,-1.66587766301974,-7.12161155557361));
#30584=CARTESIAN_POINT('Ctrl Pts',(88.5691947533982,0.937876498927613,-7.24648594044916));
#30585=CARTESIAN_POINT('Ctrl Pts',(88.6353652882123,3.01320420398057,-6.25356197326325));
#30586=CARTESIAN_POINT('Ctrl Pts',(88.6684505556194,4.05086805650711,-5.75709998967027));
#30587=CARTESIAN_POINT('Ctrl Pts',(88.7015358230265,4.95642529481004,-4.98118841806188));
#30588=CARTESIAN_POINT('Ctrl Pts',(88.7346210904335,5.62880203099263,-4.04151098367676));
#30589=CARTESIAN_POINT('Ctrl Pts',(88.7677063578405,6.30117876717522,-3.10183354929164));
#30590=CARTESIAN_POINT('Ctrl Pts',(88.8007916252474,6.74037500123749,-1.99839025212978));
#30591=CARTESIAN_POINT('Ctrl Pts',(88.8338768926544,6.88253661774944,-0.857921035482686));
#30592=CARTESIAN_POINT('Ctrl Pts',(88.8669621600615,7.02469823426139,0.282548181164276));
#30593=CARTESIAN_POINT('Ctrl Pts',(88.9000474274686,6.86982523322309,1.46004331729646));
#30594=CARTESIAN_POINT('Ctrl Pts',(88.9331326948756,6.44870444968859,2.53602725849965));
#30595=CARTESIAN_POINT('Ctrl Pts',(88.9662179622827,6.02758366615408,3.61201119970284));
#30596=CARTESIAN_POINT('Ctrl Pts',(88.9993032296895,5.34021510012337,4.58648394597703));
#30597=CARTESIAN_POINT('Ctrl Pts',(89.0323884970965,4.45618059126846,5.32248921711756));
#30598=CARTESIAN_POINT('Ctrl Pts',(89.0985590319105,2.68811157355832,6.79449975939887));
#30599=CARTESIAN_POINT('Ctrl Pts',(89.1647295667247,0.133378784551066,7.31264040114517));
#30600=CARTESIAN_POINT('Ctrl Pts',(89.2309001015388,-2.05632936253286,6.63337272219608));
#30601=CARTESIAN_POINT('Ctrl Pts',(89.2970706363528,-4.24603750961654,5.95410504324707));
#30602=CARTESIAN_POINT('Ctrl Pts',(89.3632411711668,-6.07072101477698,4.07742904360294));
#30603=CARTESIAN_POINT('Ctrl Pts',(89.4294117059808,-6.68927433964374,1.86597790824286));
#30604=CARTESIAN_POINT('Ctrl Pts',(89.4474572494518,-6.85796167071017,1.26288715630475));
#30605=CARTESIAN_POINT('Ctrl Pts',(89.4655027929228,-6.93694644387414,0.634898440211108));
#30606=CARTESIAN_POINT('Ctrl Pts',(89.4835483363938,-6.93167766374453,0.00562466873832855));
#30607=CARTESIAN_POINT('Origin',(29.75,0.,0.));
#30608=CARTESIAN_POINT('',(90.9128916636062,-6.92718184132294,0.00080019213586006));
#30609=CARTESIAN_POINT('',(90.7335483363939,-6.92146317547543,-0.000963293967941629));
#30610=CARTESIAN_POINT('',(29.75,-6.933,-8.4904762584886E-16));
#30611=CARTESIAN_POINT('Ctrl Pts',(90.9128916636062,-6.933,3.81528142412435E-12));
#30612=CARTESIAN_POINT('Ctrl Pts',(90.8556674683211,-6.9329999999989,1.99420935702016));
#30613=CARTESIAN_POINT('Ctrl Pts',(90.798443273036,-6.02307502629025,3.97063309653389));
#30614=CARTESIAN_POINT('Ctrl Pts',(90.7412190777509,-4.5079848475368,5.26731066241385));
#30615=CARTESIAN_POINT('Ctrl Pts',(90.6839948824658,-2.99289466878335,6.56398822829381));
#30616=CARTESIAN_POINT('Ctrl Pts',(90.6267706871807,-0.899664345624515,
7.15779044292466));
#30617=CARTESIAN_POINT('Ctrl Pts',(90.5695464918956,1.07062371682261,6.84983604599241));
#30618=CARTESIAN_POINT('Ctrl Pts',(90.5123222966105,3.04091177926973,6.54188164906017));
#30619=CARTESIAN_POINT('Ctrl Pts',(90.4550981013254,4.85311303640217,5.33766370386098));
#30620=CARTESIAN_POINT('Ctrl Pts',(90.3978739060403,5.90026971493993,3.64050907030359));
#30621=CARTESIAN_POINT('Ctrl Pts',(90.3406497107552,6.94742639347769,1.94335443674621));
#30622=CARTESIAN_POINT('Ctrl Pts',(90.2834255154701,7.21086008527498,-0.216464293128636));
#30623=CARTESIAN_POINT('Ctrl Pts',(90.226201320185,6.60233935005942,-2.11556236179814));
#30624=CARTESIAN_POINT('Ctrl Pts',(90.1689771248999,5.99381861484387,-4.01466043046765));
#30625=CARTESIAN_POINT('Ctrl Pts',(90.1117529296148,4.52419779646915,-5.61916312790751));
#30626=CARTESIAN_POINT('Ctrl Pts',(90.0545287343297,2.68569472999963,-6.39167683923806));
#30627=CARTESIAN_POINT('Ctrl Pts',(89.9973045390446,0.847191663530109,-7.16419055056861));
#30628=CARTESIAN_POINT('Ctrl Pts',(89.9400803437595,-1.32739978994672,-7.09093574623695));
#30629=CARTESIAN_POINT('Ctrl Pts',(89.8828561484744,-3.10974706736635,-6.19644754492495));
#30630=CARTESIAN_POINT('Ctrl Pts',(89.8256319531893,-4.89209434478598,-5.30195934361295));
#30631=CARTESIAN_POINT('Ctrl Pts',(89.7684077579042,-6.25040525058921,-3.60219296582212));
#30632=CARTESIAN_POINT('Ctrl Pts',(89.7111835626191,-6.72974280712887,-1.66644854402927));
#30633=CARTESIAN_POINT('Ctrl Pts',(89.6950862629482,-6.86458158035644,-1.12191912096272));
#30634=CARTESIAN_POINT('Ctrl Pts',(89.6789889632772,-6.9330000000003,-0.560975745773912));
#30635=CARTESIAN_POINT('Ctrl Pts',(89.6628916636062,-6.933,3.66595642731227E-12));
#30636=CARTESIAN_POINT('Ctrl Pts',(89.4835483363938,-6.93167766374453,0.00562466873832855));
#30637=CARTESIAN_POINT('Ctrl Pts',(89.5316733277368,-6.91762654921127,-1.67256223946896));
#30638=CARTESIAN_POINT('Ctrl Pts',(89.5797983190799,-6.30435085090587,-3.35988866458186));
#30639=CARTESIAN_POINT('Ctrl Pts',(89.6279233104229,-5.19520266043836,-4.60848500724921));
#30640=CARTESIAN_POINT('Ctrl Pts',(89.694093845237,-3.6701545117932,-6.3252705163049));
#30641=CARTESIAN_POINT('Ctrl Pts',(89.7602643800511,-1.20763506992989,-7.21261526334011));
#30642=CARTESIAN_POINT('Ctrl Pts',(89.8264349148651,1.05830213661075,-6.86368127949098));
#30643=CARTESIAN_POINT('Ctrl Pts',(89.8926054496791,3.32423934315126,-6.51474729564187));
#30644=CARTESIAN_POINT('Ctrl Pts',(89.9587759844931,5.39359431436911,-4.92953458090855));
#30645=CARTESIAN_POINT('Ctrl Pts',(90.0249465193072,6.33785313441409,-2.83161695413198));
#30646=CARTESIAN_POINT('Ctrl Pts',(90.0580317867142,6.80998254443662,-1.78265814074363));
#30647=CARTESIAN_POINT('Ctrl Pts',(90.0911170541212,7.00083791666589,-0.605523099344461));
#30648=CARTESIAN_POINT('Ctrl Pts',(90.1242023215282,6.90788674366042,0.546190508931948));
#30649=CARTESIAN_POINT('Ctrl Pts',(90.1572875889352,6.81493557065494,1.69790411720836));
#30650=CARTESIAN_POINT('Ctrl Pts',(90.1903728563423,6.43817785241471,2.824196292362));
#30651=CARTESIAN_POINT('Ctrl Pts',(90.2234581237493,5.81064588145672,3.7870480902803));
#30652=CARTESIAN_POINT('Ctrl Pts',(90.2565433911563,5.18311391049873,4.7498998881986));
#30653=CARTESIAN_POINT('Ctrl Pts',(90.2896286585634,4.30480768682298,5.54931130888157));
#30654=CARTESIAN_POINT('Ctrl Pts',(90.3227139259704,3.28866101015077,6.09933866051073));
#30655=CARTESIAN_POINT('Ctrl Pts',(90.3557991933774,2.27251433347868,6.64936601213983));
#30656=CARTESIAN_POINT('Ctrl Pts',(90.3888844607844,1.11852720381016,6.95000929471518));
#30657=CARTESIAN_POINT('Ctrl Pts',(90.4219697281914,-0.0317551929082471,
6.94157248295037));
#30658=CARTESIAN_POINT('Ctrl Pts',(90.4881402630053,-2.33231998634532,6.92469885942073));
#30659=CARTESIAN_POINT('Ctrl Pts',(90.5543107978194,-4.61806584798195,5.67150485853014));
#30660=CARTESIAN_POINT('Ctrl Pts',(90.6204813326335,-5.8521381065398,3.73933198589997));
#30661=CARTESIAN_POINT('Ctrl Pts',(90.658170333887,-6.55503330045561,2.63881699047063));
#30662=CARTESIAN_POINT('Ctrl Pts',(90.6958593351404,-6.91675055518297,1.31803155035726));
#30663=CARTESIAN_POINT('Ctrl Pts',(90.7335483363939,-6.92146317547543,-0.000963293967941629));
#30664=CARTESIAN_POINT('Origin',(29.75,0.,0.));
#30665=CARTESIAN_POINT('',(92.1628916636062,-6.93839386646797,-0.00802539788412049));
#30666=CARTESIAN_POINT('',(91.9835483363938,-6.93565096779518,-0.0017588741014353));
#30667=CARTESIAN_POINT('',(29.75,-6.933,-8.4904762584886E-16));
#30668=CARTESIAN_POINT('Ctrl Pts',(92.1628916636062,-6.93839386646797,-0.00802539788412049));
#30669=CARTESIAN_POINT('Ctrl Pts',(92.1069284483969,-6.92141512853983,1.93686533832047));
#30670=CARTESIAN_POINT('Ctrl Pts',(92.0509652331876,-6.06505943965661,3.89823190017224));
#30671=CARTESIAN_POINT('Ctrl Pts',(91.9950020179784,-4.61462848763626,5.18974649343901));
#30672=CARTESIAN_POINT('Ctrl Pts',(91.9288314831643,-2.89964854148488,6.71682479008534));
#30673=CARTESIAN_POINT('Ctrl Pts',(91.8626609483504,-0.354119244346323,
7.30741380281861));
#30674=CARTESIAN_POINT('Ctrl Pts',(91.7964904135363,1.85806218476672,6.69147739012891));
#30675=CARTESIAN_POINT('Ctrl Pts',(91.7303198787223,4.07024361387963,6.07554097743925));
#30676=CARTESIAN_POINT('Ctrl Pts',(91.6641493439082,5.94907717496707,4.25307913932677));
#30677=CARTESIAN_POINT('Ctrl Pts',(91.5979788090942,6.63093513249416,2.06417620067773));
#30678=CARTESIAN_POINT('Ctrl Pts',(91.5318082742801,7.3127930900213,-0.124726737971427));
#30679=CARTESIAN_POINT('Ctrl Pts',(91.4656377394661,6.79767544398795,-2.68007077715719));
#30680=CARTESIAN_POINT('Ctrl Pts',(91.3994672046521,5.3277578235197,-4.44988016717922));
#30681=CARTESIAN_POINT('Ctrl Pts',(91.366381937245,4.59279901328558,-5.33478486219024));
#30682=CARTESIAN_POINT('Ctrl Pts',(91.333296669838,3.61914020944273,-6.02330589491032));
#30683=CARTESIAN_POINT('Ctrl Pts',(91.300211402431,2.54365527055743,-6.44569943449522));
#30684=CARTESIAN_POINT('Ctrl Pts',(91.267126135024,1.46817033167227,-6.86809297408008));
#30685=CARTESIAN_POINT('Ctrl Pts',(91.2340408676171,0.290859257744679,-7.02435902052981));
#30686=CARTESIAN_POINT('Ctrl Pts',(91.20095560021,-0.849777359231778,-6.88354685010008));
#30687=CARTESIAN_POINT('Ctrl Pts',(91.167870332803,-1.99041397620836,-6.74273467967033));
#30688=CARTESIAN_POINT('Ctrl Pts',(91.1347850653959,-3.09437613623381,-6.30484429236105));
#30689=CARTESIAN_POINT('Ctrl Pts',(91.1016997979888,-4.03484843570422,-5.63357980649799));
#30690=CARTESIAN_POINT('Ctrl Pts',(91.0686145305818,-4.97532073517462,-4.96231532063492));
#30691=CARTESIAN_POINT('Ctrl Pts',(91.0355292631749,-5.75230317408999,-4.05767673621806));
#30692=CARTESIAN_POINT('Ctrl Pts',(91.0024439957679,-6.24999252257306,-3.02060099915746));
#30693=CARTESIAN_POINT('Ctrl Pts',(90.9725932183807,-6.6990266430109,-2.08491211443893));
#30694=CARTESIAN_POINT('Ctrl Pts',(90.9427424409935,-6.9207069805332,-1.04141502148469));
#30695=CARTESIAN_POINT('Ctrl Pts',(90.9128916636062,-6.91918773061192,0.00189965071867138));
#30696=CARTESIAN_POINT('Ctrl Pts',(90.7335483363939,-6.92146317547543,-0.000963293967941629));
#30697=CARTESIAN_POINT('Ctrl Pts',(90.7620298699545,-6.92502449704284,-0.997726133934744));
#30698=CARTESIAN_POINT('Ctrl Pts',(90.7905114035151,-6.72470736279399,-1.99346639920903));
#30699=CARTESIAN_POINT('Ctrl Pts',(90.8189929370756,-6.31368152489429,-2.8923503154485));
#30700=CARTESIAN_POINT('Ctrl Pts',(90.8851634718897,-5.35875402921189,-4.98070799979733));
#30701=CARTESIAN_POINT('Ctrl Pts',(90.9513340067037,-3.26650038236796,-6.54627162412541));
#30702=CARTESIAN_POINT('Ctrl Pts',(91.0175045415177,-0.993565712653891,
-6.87321554439442));
#30703=CARTESIAN_POINT('Ctrl Pts',(91.0836750763317,1.27936895706031,-7.20015946466345));
#30704=CARTESIAN_POINT('Ctrl Pts',(91.1498456111458,3.73298464964467,-6.2884836808732));
#30705=CARTESIAN_POINT('Ctrl Pts',(91.2160161459598,5.23849463787312,-4.55941860852503));
#30706=CARTESIAN_POINT('Ctrl Pts',(91.2821866807739,6.74400462610157,-2.83035353617686));
#30707=CARTESIAN_POINT('Ctrl Pts',(91.348357215588,7.30140890997411,-0.283899175270764));
#30708=CARTESIAN_POINT('Ctrl Pts',(91.414527750402,6.66853635908363,1.92796777875305));
#30709=CARTESIAN_POINT('Ctrl Pts',(91.447613017809,6.35210008363843,3.03390125576483));
#30710=CARTESIAN_POINT('Ctrl Pts',(91.480698285216,5.73809459950255,4.05618788105605));
#30711=CARTESIAN_POINT('Ctrl Pts',(91.513783552623,4.92372512177406,4.87587471747353));
#30712=CARTESIAN_POINT('Ctrl Pts',(91.54686882003,4.10935564404549,5.69556155389111));
#30713=CARTESIAN_POINT('Ctrl Pts',(91.579954087437,3.09462217272427,6.31264860143489));
#30714=CARTESIAN_POINT('Ctrl Pts',(91.613039354844,1.99383914151695,6.64303727789786));
#30715=CARTESIAN_POINT('Ctrl Pts',(91.6461246222511,0.893056110309632,6.97342595436083));
#30716=CARTESIAN_POINT('Ctrl Pts',(91.6792098896581,-0.293776480783792,
7.01711625974298));
#30717=CARTESIAN_POINT('Ctrl Pts',(91.7122951570651,-1.4249271508334,6.78135723510452));
#30718=CARTESIAN_POINT('Ctrl Pts',(91.7453804244721,-2.55607782088288,6.54559821046609));
#30719=CARTESIAN_POINT('Ctrl Pts',(91.7784656918791,-3.63154656988856,6.03038985580711));
#30720=CARTESIAN_POINT('Ctrl Pts',(91.8115509592862,-4.50469000490483,5.28149646293935));
#30721=CARTESIAN_POINT('Ctrl Pts',(91.868883418322,-6.0177338502121,3.98376175701588));
#30722=CARTESIAN_POINT('Ctrl Pts',(91.9262158773579,-6.92322764173258,1.98430883930039));
#30723=CARTESIAN_POINT('Ctrl Pts',(91.9835483363938,-6.94004001014585,-0.0046709324541017));
#30724=CARTESIAN_POINT('Origin',(29.75,0.,0.));
#30725=CARTESIAN_POINT('',(93.4128916636062,-6.93875336632197,0.00522259790129709));
#30726=CARTESIAN_POINT('',(93.2335483363939,-6.93307491442268,0.000658892883751194));
#30727=CARTESIAN_POINT('',(29.75,-6.933,-8.4904762584886E-16));
#30728=CARTESIAN_POINT('Ctrl Pts',(93.4128916636062,-6.93875336632197,0.00522259790129709));
#30729=CARTESIAN_POINT('Ctrl Pts',(93.4034555254285,-6.94167326281239,0.333422550527998));
#30730=CARTESIAN_POINT('Ctrl Pts',(93.3940193872508,-6.92062603608355,0.661249996353714));
#30731=CARTESIAN_POINT('Ctrl Pts',(93.3845832490732,-6.8743862713196,0.985432969693625));
#30732=CARTESIAN_POINT('Ctrl Pts',(93.3184127142592,-6.55013180339034,3.25875287235075));
#30733=CARTESIAN_POINT('Ctrl Pts',(93.2522421794451,-4.98704472552019,5.35285735196643));
#30734=CARTESIAN_POINT('Ctrl Pts',(93.1860716446311,-2.89981832568375,6.31025502044848));
#30735=CARTESIAN_POINT('Ctrl Pts',(93.1199011098171,-0.812591925847067,
7.26765268893064));
#30736=CARTESIAN_POINT('Ctrl Pts',(93.053730575003,1.79877379595603,7.08834354627892));
#30737=CARTESIAN_POINT('Ctrl Pts',(92.9875600401889,3.73240540926872,5.85655820253256));
#30738=CARTESIAN_POINT('Ctrl Pts',(92.9213895053749,5.66603702258108,4.6247728587864));
#30739=CARTESIAN_POINT('Ctrl Pts',(92.8552189705608,6.92193452740331,2.34051131394602));
#30740=CARTESIAN_POINT('Ctrl Pts',(92.7890484357468,6.9415300532182,0.0399680947605974));
#30741=CARTESIAN_POINT('Ctrl Pts',(92.7559631683398,6.95132781612565,-1.11030351483225));
#30742=CARTESIAN_POINT('Ctrl Pts',(92.7228779009328,6.6520500842812,-2.26464554301135));
#30743=CARTESIAN_POINT('Ctrl Pts',(92.6897926335258,6.103225371949,-3.28144227352618));
#30744=CARTESIAN_POINT('Ctrl Pts',(92.6567073661188,5.55440065961681,-4.29823900404101));
#30745=CARTESIAN_POINT('Ctrl Pts',(92.6236220987117,4.75602896679687,-5.17749043689156));
#30746=CARTESIAN_POINT('Ctrl Pts',(92.5905368313047,3.79392030748638,-5.80616116709036));
#30747=CARTESIAN_POINT('Ctrl Pts',(92.5574515638977,2.83181164817599,-6.43483189728908));
#30748=CARTESIAN_POINT('Ctrl Pts',(92.5243662964907,1.70596602237508,-6.81292192483611));
#30749=CARTESIAN_POINT('Ctrl Pts',(92.4912810290837,0.554363195424337,-6.90723568316918));
#30750=CARTESIAN_POINT('Ctrl Pts',(92.4581957616767,-0.597239631526407,
-7.00154944150225));
#30751=CARTESIAN_POINT('Ctrl Pts',(92.4251104942697,-1.77459965962699,-6.81208693062137));
#30752=CARTESIAN_POINT('Ctrl Pts',(92.3920252268626,-2.8241163389132,-6.34119892706528));
#30753=CARTESIAN_POINT('Ctrl Pts',(92.3258546920486,-4.92314969748599,-5.39942291995293));
#30754=CARTESIAN_POINT('Ctrl Pts',(92.2596841572346,-6.51080966080111,-3.33194494213933));
#30755=CARTESIAN_POINT('Ctrl Pts',(92.1935136224205,-6.86242434487645,-1.06642216295277));
#30756=CARTESIAN_POINT('Ctrl Pts',(92.1833063028158,-6.91666364441026,-0.716947655242347));
#30757=CARTESIAN_POINT('Ctrl Pts',(92.173098983211,-6.94149067575369,-0.362760580031751));
#30758=CARTESIAN_POINT('Ctrl Pts',(92.1628916636062,-6.93839386646797,-0.00802539788412049));
#30759=CARTESIAN_POINT('Ctrl Pts',(91.9835483363938,-6.933,-2.3049617769999E-12));
#30760=CARTESIAN_POINT('Ctrl Pts',(92.0407725316789,-6.93299999999934,-1.99420935701865));
#30761=CARTESIAN_POINT('Ctrl Pts',(92.097996726964,-6.02307502629111,-3.97063309653258));
#30762=CARTESIAN_POINT('Ctrl Pts',(92.1552209222491,-4.50798484753795,-5.26731066241287));
#30763=CARTESIAN_POINT('Ctrl Pts',(92.2124451175342,-2.99289466878478,-6.56398822829316));
#30764=CARTESIAN_POINT('Ctrl Pts',(92.2696693128193,-0.899664345626074,
-7.15779044292446));
#30765=CARTESIAN_POINT('Ctrl Pts',(92.3268935081044,1.07062371682111,-6.84983604599264));
#30766=CARTESIAN_POINT('Ctrl Pts',(92.3841177033895,3.0409117792683,-6.54188164906083));
#30767=CARTESIAN_POINT('Ctrl Pts',(92.4413418986746,4.853113036401,-5.33766370386204));
#30768=CARTESIAN_POINT('Ctrl Pts',(92.4985660939597,5.90026971493913,-3.64050907030488));
#30769=CARTESIAN_POINT('Ctrl Pts',(92.5557902892448,6.94742639347726,-1.94335443674772));
#30770=CARTESIAN_POINT('Ctrl Pts',(92.6130144845299,7.21086008527502,0.216464293127065));
#30771=CARTESIAN_POINT('Ctrl Pts',(92.670238679815,6.60233935005988,2.11556236179671));
#30772=CARTESIAN_POINT('Ctrl Pts',(92.7274628751001,5.99381861484474,4.01466043046635));
#30773=CARTESIAN_POINT('Ctrl Pts',(92.7846870703852,4.52419779647037,5.61916312790652));
#30774=CARTESIAN_POINT('Ctrl Pts',(92.8419112656703,2.68569473000102,6.39167683923747));
#30775=CARTESIAN_POINT('Ctrl Pts',(92.8991354609554,0.847191663531669,7.16419055056843));
#30776=CARTESIAN_POINT('Ctrl Pts',(92.9563596562405,-1.32739978994518,7.09093574623724));
#30777=CARTESIAN_POINT('Ctrl Pts',(93.0135838515256,-3.109747067365,6.19644754492562));
#30778=CARTESIAN_POINT('Ctrl Pts',(93.0708080468107,-4.89209434478482,5.30195934361401));
#30779=CARTESIAN_POINT('Ctrl Pts',(93.1280322420958,-6.25040525058842,3.60219296582348));
#30780=CARTESIAN_POINT('Ctrl Pts',(93.1852564373809,-6.7297428071285,1.66644854403074));
#30781=CARTESIAN_POINT('Ctrl Pts',(93.2013537370519,-6.86458158035613,1.12191912096447));
#30782=CARTESIAN_POINT('Ctrl Pts',(93.2174510367228,-6.93300000000011,0.560975745775948));
#30783=CARTESIAN_POINT('Ctrl Pts',(93.2335483363938,-6.933,-1.36723965482588E-12));
#30784=CARTESIAN_POINT('Origin',(29.75,0.,0.));
#30785=CARTESIAN_POINT('',(94.6628916636061,-6.92404070110412,0.00207036192589771));
#30786=CARTESIAN_POINT('',(94.4835483363939,-6.92908201353558,0.00220150041010815));
#30787=CARTESIAN_POINT('',(29.75,-6.933,-8.4904762584886E-16));
#30788=CARTESIAN_POINT('Ctrl Pts',(94.6628916636061,-6.92404070110412,0.00207036192589771));
#30789=CARTESIAN_POINT('Ctrl Pts',(94.6338120676461,-6.92690635206978,1.01894162261975));
#30790=CARTESIAN_POINT('Ctrl Pts',(94.604732471686,-6.71688041784802,2.03469379117756));
#30791=CARTESIAN_POINT('Ctrl Pts',(94.5756528757259,-6.28784118309068,2.94810413677931));
#30792=CARTESIAN_POINT('Ctrl Pts',(94.5094823409118,-5.31156367018941,5.02656668337304));
#30793=CARTESIAN_POINT('Ctrl Pts',(94.4433118060977,-3.20126007432825,6.57511485341535));
#30794=CARTESIAN_POINT('Ctrl Pts',(94.3771412712837,-0.929291360962711,
6.88233548188621));
#30795=CARTESIAN_POINT('Ctrl Pts',(94.3109707364697,1.3426773524027,7.18955611035705));
#30796=CARTESIAN_POINT('Ctrl Pts',(94.2448002016557,3.77631118327259,6.2554491972566));
#30797=CARTESIAN_POINT('Ctrl Pts',(94.1786296668417,5.27616304063658,4.51093565648535));
#30798=CARTESIAN_POINT('Ctrl Pts',(94.1455443994346,6.02608896931861,3.63867888609968));
#30799=CARTESIAN_POINT('Ctrl Pts',(94.1124591320276,6.54256940462418,2.56382045879623));
#30800=CARTESIAN_POINT('Ctrl Pts',(94.0793738646205,6.77966658558774,1.43294951884275));
#30801=CARTESIAN_POINT('Ctrl Pts',(94.0462885972135,7.0167637665513,0.302078578889283));
#30802=CARTESIAN_POINT('Ctrl Pts',(94.0132033298066,6.97447769317291,-0.884804873713921));
#30803=CARTESIAN_POINT('Ctrl Pts',(93.9801180623996,6.64539163981147,-1.98597803394435));
#30804=CARTESIAN_POINT('Ctrl Pts',(93.9470327949925,6.31630558644999,-3.0871511941749));
#30805=CARTESIAN_POINT('Ctrl Pts',(93.9139475275855,5.70041955310533,-4.10261406203237));
#30806=CARTESIAN_POINT('Ctrl Pts',(93.8808622601784,4.88169681195711,-4.91795278255235));
#30807=CARTESIAN_POINT('Ctrl Pts',(93.8477769927714,4.06297407080907,-5.73329150307215));
#30808=CARTESIAN_POINT('Ctrl Pts',(93.8146917253644,3.0414146218575,-6.34850607625464));
#30809=CARTESIAN_POINT('Ctrl Pts',(93.7816064579574,1.93585631061123,-6.66625061582574));
#30810=CARTESIAN_POINT('Ctrl Pts',(93.7154359231434,-0.275260311881576,
-7.30173969496801));
#30811=CARTESIAN_POINT('Ctrl Pts',(93.6492653883293,-2.82237238355351,-6.74734863966452));
#30812=CARTESIAN_POINT('Ctrl Pts',(93.5830948535153,-4.55321749039531,-5.24388544916344));
#30813=CARTESIAN_POINT('Ctrl Pts',(93.5263604568789,-6.03723833265783,-3.95482110628342));
#30814=CARTESIAN_POINT('Ctrl Pts',(93.4696260602425,-6.9211976075459,-1.96806625584167));
#30815=CARTESIAN_POINT('Ctrl Pts',(93.4128916636062,-6.93875336632197,0.00522259790129709));
#30816=CARTESIAN_POINT('Ctrl Pts',(93.2335483363938,-6.93338545573979,0.00339018893299717));
#30817=CARTESIAN_POINT('Ctrl Pts',(93.2889134892035,-6.91513820903545,-1.92436519451582));
#30818=CARTESIAN_POINT('Ctrl Pts',(93.3442786420133,-6.08482141908014,-3.85875145648536));
#30819=CARTESIAN_POINT('Ctrl Pts',(93.3996437948231,-4.66302902386902,-5.14648272525469));
#30820=CARTESIAN_POINT('Ctrl Pts',(93.4658143296372,-2.96375143840046,-6.68553504294682));
#30821=CARTESIAN_POINT('Ctrl Pts',(93.5319848644511,-0.419597565822329,
-7.30089166661355));
#30822=CARTESIAN_POINT('Ctrl Pts',(93.5981553992651,1.79877943452019,-6.7076566169575));
#30823=CARTESIAN_POINT('Ctrl Pts',(93.6643259340792,4.01715643486283,-6.11442156730142));
#30824=CARTESIAN_POINT('Ctrl Pts',(93.7304964688933,5.9097565629698,-4.31259484432236));
#30825=CARTESIAN_POINT('Ctrl Pts',(93.7966670037073,6.6112226499871,-2.12602911959458));
#30826=CARTESIAN_POINT('Ctrl Pts',(93.8628375385213,7.3126887370044,0.0605366051331999));
#30827=CARTESIAN_POINT('Ctrl Pts',(93.9290080733354,6.82302078293202,2.63184133160969));
#30828=CARTESIAN_POINT('Ctrl Pts',(93.9951786081494,5.36927895395365,4.40465295266497));
#30829=CARTESIAN_POINT('Ctrl Pts',(94.0613491429634,3.91553712497536,6.17746457372014));
#30830=CARTESIAN_POINT('Ctrl Pts',(94.1275196777775,1.4977214210912,7.1517830893542));
#30831=CARTESIAN_POINT('Ctrl Pts',(94.1936902125915,-0.788719383856762,
6.89669186362991));
#30832=CARTESIAN_POINT('Ctrl Pts',(94.2267754799985,-1.93193978633081,6.76914625076775));
#30833=CARTESIAN_POINT('Ctrl Pts',(94.2598607474055,-3.0423164640708,6.33424820256598));
#30834=CARTESIAN_POINT('Ctrl Pts',(94.2929460148126,-3.98634989426118,5.66800122228379));
#30835=CARTESIAN_POINT('Ctrl Pts',(94.3260312822196,-4.93038332445145,5.00175424200167));
#30836=CARTESIAN_POINT('Ctrl Pts',(94.3591165496266,-5.70807350709216,4.1041583296392));
#30837=CARTESIAN_POINT('Ctrl Pts',(94.3922018170336,-6.21743341290116,3.07389989328311));
#30838=CARTESIAN_POINT('Ctrl Pts',(94.4226506568204,-6.68620454220678,2.12573847504145));
#30839=CARTESIAN_POINT('Ctrl Pts',(94.4530994966071,-6.92770579363022,1.06521479942219));
#30840=CARTESIAN_POINT('Ctrl Pts',(94.4835483363939,-6.92908201353558,0.00220150041010815));
#30841=CARTESIAN_POINT('Origin',(29.75,0.,0.));
#30842=CARTESIAN_POINT('',(95.9128916636062,-6.93006097531607,-0.0057025460704313));
#30843=CARTESIAN_POINT('',(95.7335483363938,-6.93097598691781,-0.00393591295944164));
#30844=CARTESIAN_POINT('',(29.75,-6.933,-8.4904762584886E-16));
#30845=CARTESIAN_POINT('Ctrl Pts',(95.9128916636062,-6.93006097531607,-0.0057025460704313));
#30846=CARTESIAN_POINT('Ctrl Pts',(95.8641686098637,-6.91417425872587,1.69433574802711));
#30847=CARTESIAN_POINT('Ctrl Pts',(95.8154455561211,-6.2837585161334,3.40437531631781));
#30848=CARTESIAN_POINT('Ctrl Pts',(95.7667225023785,-5.15199618764788,4.65693669714884));
#30849=CARTESIAN_POINT('Ctrl Pts',(95.7005519675645,-3.61495544808387,6.35803402357966));
#30850=CARTESIAN_POINT('Ctrl Pts',(95.6343814327504,-1.1532200453151,7.21534852515465));
#30851=CARTESIAN_POINT('Ctrl Pts',(95.5682108979364,1.11836667277205,6.85096291871172));
#30852=CARTESIAN_POINT('Ctrl Pts',(95.5351256305294,2.25416003181581,6.66877011549023));
#30853=CARTESIAN_POINT('Ctrl Pts',(95.5020403631224,3.3424162196891,6.18115228526414));
#30854=CARTESIAN_POINT('Ctrl Pts',(95.4689550957154,4.25343193671011,5.47042412387387));
#30855=CARTESIAN_POINT('Ctrl Pts',(95.4358698283084,5.16444765373091,4.75969596248375));
#30856=CARTESIAN_POINT('Ctrl Pts',(95.4027845609013,5.89822289989943,3.82585746992961));
#30857=CARTESIAN_POINT('Ctrl Pts',(95.3696992934943,6.35761782886665,2.77236980575509));
#30858=CARTESIAN_POINT('Ctrl Pts',(95.3366140260872,6.81701275783391,1.71888214158046));
#30859=CARTESIAN_POINT('Ctrl Pts',(95.3035287586802,7.00202736959979,0.545745305785123));
#30860=CARTESIAN_POINT('Ctrl Pts',(95.2704434912732,6.90294467185206,-0.605457011385599));
#30861=CARTESIAN_POINT('Ctrl Pts',(95.2373582238662,6.80386197410433,-1.75665932855619));
#30862=CARTESIAN_POINT('Ctrl Pts',(95.2042729564592,6.42068196684316,-2.88592712710245));
#30863=CARTESIAN_POINT('Ctrl Pts',(95.1711876890522,5.78134147007617,-3.84220349990833));
#30864=CARTESIAN_POINT('Ctrl Pts',(95.1050171542381,4.50266047654211,-5.75475624552021));
#30865=CARTESIAN_POINT('Ctrl Pts',(95.0388466194241,2.19933752498479,-6.97534328817024));
#30866=CARTESIAN_POINT('Ctrl Pts',(94.9726760846101,-0.0930966390109256,
-6.94416713037601));
#30867=CARTESIAN_POINT('Ctrl Pts',(94.9065055497961,-2.38553080300677,-6.91299097258179));
#30868=CARTESIAN_POINT('Ctrl Pts',(94.840335014982,-4.66707617944086,-5.63005161434315));
#30869=CARTESIAN_POINT('Ctrl Pts',(94.7741644801679,-5.88672315268717,-3.68439347365119));
#30870=CARTESIAN_POINT('Ctrl Pts',(94.737073541314,-6.57037867149475,-2.59378286683231));
#30871=CARTESIAN_POINT('Ctrl Pts',(94.6999826024601,-6.92038557175193,-1.2949459310265));
#30872=CARTESIAN_POINT('Ctrl Pts',(94.6628916636061,-6.92404070110412,0.00207036192589771));
#30873=CARTESIAN_POINT('Ctrl Pts',(94.4835483363939,-6.92908201353558,0.00220150041010815));
#30874=CARTESIAN_POINT('Ctrl Pts',(94.4861847640141,-6.92920117420624,-0.0898400237292746));
#30875=CARTESIAN_POINT('Ctrl Pts',(94.4888211916344,-6.92752010633732,-0.18190021269113));
#30876=CARTESIAN_POINT('Ctrl Pts',(94.4914576192547,-6.92403046519316,-0.273907744256341));
#30877=CARTESIAN_POINT('Ctrl Pts',(94.5245428866617,-6.88023798269881,-1.42853598508922));
#30878=CARTESIAN_POINT('Ctrl Pts',(94.5576281540687,-6.55162338873298,-2.57487150640527));
#30879=CARTESIAN_POINT('Ctrl Pts',(94.5907134214757,-5.95885134174323,-3.5606920135467));
#30880=CARTESIAN_POINT('Ctrl Pts',(94.6568839562896,-4.7733072477636,-5.53233302782977));
#30881=CARTESIAN_POINT('Ctrl Pts',(94.7230544911038,-2.53113334168807,-6.86191398541422));
#30882=CARTESIAN_POINT('Ctrl Pts',(94.7892250259179,-0.239839551955025,
-6.94064846452462));
#30883=CARTESIAN_POINT('Ctrl Pts',(94.8553955607319,2.05145423777802,-7.01938294363501));
#30884=CARTESIAN_POINT('Ctrl Pts',(94.9215660955459,4.39186791116858,-5.84727094427134));
#30885=CARTESIAN_POINT('Ctrl Pts',(94.9877366303599,5.70336724912391,-3.96230573866875));
#30886=CARTESIAN_POINT('Ctrl Pts',(95.053907165174,7.01486658707917,-2.07734053306627));
#30887=CARTESIAN_POINT('Ctrl Pts',(95.120077699988,7.29745158959932,0.520477878775046));
#30888=CARTESIAN_POINT('Ctrl Pts',(95.186248234802,6.42191537663093,2.64334402612632));
#30889=CARTESIAN_POINT('Ctrl Pts',(95.2524187696161,5.5463791636625,4.76621017347772));
#30890=CARTESIAN_POINT('Ctrl Pts',(95.3185893044301,3.5127217352054,6.41412405633902));
#30891=CARTESIAN_POINT('Ctrl Pts',(95.3847598392442,1.2580890031021,6.82988551727358));
#30892=CARTESIAN_POINT('Ctrl Pts',(95.4509303740582,-0.996543729001065,
7.24564697820812));
#30893=CARTESIAN_POINT('Ctrl Pts',(95.5171009088724,-3.4721517647504,6.42925601721605));
#30894=CARTESIAN_POINT('Ctrl Pts',(95.5832714436863,-5.05389323211731,4.75863427116323));
#30895=CARTESIAN_POINT('Ctrl Pts',(95.6163567110933,-5.84476396580081,3.92332339813677));
#30896=CARTESIAN_POINT('Ctrl Pts',(95.6494419785002,-6.41216805738867,2.8744548288451));
#30897=CARTESIAN_POINT('Ctrl Pts',(95.6825272459073,-6.70319462303771,1.75624747144725));
#30898=CARTESIAN_POINT('Ctrl Pts',(95.6995342760694,-6.85279285717295,1.1814482406943));
#30899=CARTESIAN_POINT('Ctrl Pts',(95.7165413062316,-6.92936292591762,0.588327388208185));
#30900=CARTESIAN_POINT('Ctrl Pts',(95.7335483363938,-6.93097598691781,-0.00393591295944164));
#30901=CARTESIAN_POINT('Origin',(29.75,0.,0.));
#30902=CARTESIAN_POINT('',(97.1628916636062,-6.94438291503296,0.0033794907004818));
#30903=CARTESIAN_POINT('',(96.9835483363938,-6.94194141381233,0.000872210908587178));
#30904=CARTESIAN_POINT('',(29.75,-6.933,-8.4904762584886E-16));
#30905=CARTESIAN_POINT('Ctrl Pts',(97.1628916636062,-6.94438291503296,0.0033794907004818));
#30906=CARTESIAN_POINT('Ctrl Pts',(97.1606956868953,-6.94459561280772,0.0794883938480412));
#30907=CARTESIAN_POINT('Ctrl Pts',(97.1584997101843,-6.94345033553247,0.155584207710589));
#30908=CARTESIAN_POINT('Ctrl Pts',(97.1563037334734,-6.94092737286312,0.231627553260109));
#30909=CARTESIAN_POINT('Ctrl Pts',(97.0901331986593,-6.86490389396477,2.52301289399314));
#30910=CARTESIAN_POINT('Ctrl Pts',(97.0239626638451,-5.53797669587943,4.76675832492743));
#30911=CARTESIAN_POINT('Ctrl Pts',(96.9577921290311,-3.5677397385306,5.95463433692111));
#30912=CARTESIAN_POINT('Ctrl Pts',(96.9247068616242,-2.5826212598563,6.54857234291788));
#30913=CARTESIAN_POINT('Ctrl Pts',(96.8916215942172,-1.43667534136616,6.87854299417956));
#30914=CARTESIAN_POINT('Ctrl Pts',(96.8585363268102,-0.282099721775767,
6.92370154485739));
#30915=CARTESIAN_POINT('Ctrl Pts',(96.8254510594032,0.872475897814623,6.96886009553523));
#30916=CARTESIAN_POINT('Ctrl Pts',(96.7923657919961,2.03568121850526,6.72920654562922));
#30917=CARTESIAN_POINT('Ctrl Pts',(96.7592805245891,3.06654158312319,6.22106594698705));
#30918=CARTESIAN_POINT('Ctrl Pts',(96.726195257182,4.09740194774136,5.71292534834477));
#30919=CARTESIAN_POINT('Ctrl Pts',(96.6931099897751,4.99591735628674,4.9362977009662));
#30920=CARTESIAN_POINT('Ctrl Pts',(96.660024722368,5.66328080375355,3.99305320188991));
#30921=CARTESIAN_POINT('Ctrl Pts',(96.626939454961,6.33064425122035,3.04980870281361));
#30922=CARTESIAN_POINT('Ctrl Pts',(96.593854187554,6.76685573760857,1.93994735203959));
#30923=CARTESIAN_POINT('Ctrl Pts',(96.560768920147,6.89575386284522,0.796878655370808));
#30924=CARTESIAN_POINT('Ctrl Pts',(96.4945983853329,7.15355011331848,-1.4892587379665));
#30925=CARTESIAN_POINT('Ctrl Pts',(96.4284278505189,6.18209291918581,-3.90822551488283));
#30926=CARTESIAN_POINT('Ctrl Pts',(96.3622573157048,4.41100253414985,-5.36406382908644));
#30927=CARTESIAN_POINT('Ctrl Pts',(96.2960867808908,2.63991214911409,-6.81990214328987));
#30928=CARTESIAN_POINT('Ctrl Pts',(96.2299162460767,0.0691885731752734,
-7.31261199478086));
#30929=CARTESIAN_POINT('Ctrl Pts',(96.1637457112627,-2.1182055609885,-6.61373343479036));
#30930=CARTESIAN_POINT('Ctrl Pts',(96.0975751764487,-4.30559969515253,-5.91485487479979));
#30931=CARTESIAN_POINT('Ctrl Pts',(96.0314046416347,-6.10966438754142,-4.02438790332748));
#30932=CARTESIAN_POINT('Ctrl Pts',(95.9652341068207,-6.70552369555624,-1.80671434194794));
#30933=CARTESIAN_POINT('Ctrl Pts',(95.9477866257492,-6.86263658616644,-1.22197042845769));
#30934=CARTESIAN_POINT('Ctrl Pts',(95.9303391446777,-6.93574992881354,-0.614477729042277));
#30935=CARTESIAN_POINT('Ctrl Pts',(95.9128916636062,-6.93006097531607,-0.0057025460704313));
#30936=CARTESIAN_POINT('Ctrl Pts',(95.7335483363938,-6.93097598691781,-0.00393591295944164));
#30937=CARTESIAN_POINT('Ctrl Pts',(95.7496265736387,-6.93250095495774,-0.56385435708546));
#30938=CARTESIAN_POINT('Ctrl Pts',(95.7657048108836,-6.86703250395054,-1.12300635793202));
#30939=CARTESIAN_POINT('Ctrl Pts',(95.7817830481285,-6.73294086289519,-1.66518651644247));
#30940=CARTESIAN_POINT('Ctrl Pts',(95.8148683155355,-6.45701149739346,-2.78086700143006));
#30941=CARTESIAN_POINT('Ctrl Pts',(95.8479535829424,-5.89050372667986,-3.82468182590149));
#30942=CARTESIAN_POINT('Ctrl Pts',(95.8810388503494,-5.11180054835783,-4.67832432491541));
#30943=CARTESIAN_POINT('Ctrl Pts',(95.9141241177564,-4.33309737003554,-5.53196682392962));
#30944=CARTESIAN_POINT('Ctrl Pts',(95.9472093851635,-3.34219878410467,-6.19543699748618));
#30945=CARTESIAN_POINT('Ctrl Pts',(95.9802946525705,-2.25314033729704,-6.56580501909516));
#30946=CARTESIAN_POINT('Ctrl Pts',(96.0464651873846,-0.0750234436820296,
-7.30654106231305));
#30947=CARTESIAN_POINT('Ctrl Pts',(96.1126357221986,2.49573289343994,-6.8748684977409));
#30948=CARTESIAN_POINT('Ctrl Pts',(96.1788062570126,4.2966487576269,-5.4560914189897));
#30949=CARTESIAN_POINT('Ctrl Pts',(96.2449767918266,6.09756462181375,-4.03731434023859));
#30950=CARTESIAN_POINT('Ctrl Pts',(96.3111473266407,7.12864001306566,-1.63143274730855));
#30951=CARTESIAN_POINT('Ctrl Pts',(96.3773178614547,6.913716874689,0.654815792194409));
#30952=CARTESIAN_POINT('Ctrl Pts',(96.4434883962688,6.69879373631232,2.9410643316975));
#30953=CARTESIAN_POINT('Ctrl Pts',(96.5096589310827,5.23787206830692,5.10767981777348));
#30954=CARTESIAN_POINT('Ctrl Pts',(96.5758294658968,3.19893187329868,6.16401651644934));
#30955=CARTESIAN_POINT('Ctrl Pts',(96.6420000007108,1.15999167829055,7.22035321512515));
#30956=CARTESIAN_POINT('Ctrl Pts',(96.708170535525,-1.45696704372035,7.16641112640097));
#30957=CARTESIAN_POINT('Ctrl Pts',(96.774341070339,-3.44741502385695,6.0287190821994));
#30958=CARTESIAN_POINT('Ctrl Pts',(96.840511605153,-5.43786300399367,4.89102703799777));
#30959=CARTESIAN_POINT('Ctrl Pts',(96.9066821399668,-6.80180024225602,2.66958503831864));
#30960=CARTESIAN_POINT('Ctrl Pts',(96.972852674781,-6.93163671608136,0.372624965083196));
#30961=CARTESIAN_POINT('Ctrl Pts',(96.9764178953186,-6.93863221134688,0.248866418320443));
#30962=CARTESIAN_POINT('Ctrl Pts',(96.9799831158562,-6.94204514118107,0.124888644370122));
#30963=CARTESIAN_POINT('Ctrl Pts',(96.9835483363938,-6.94194141381233,0.000872210908587178));
#30964=CARTESIAN_POINT('Origin',(29.75,0.,0.));
#30965=CARTESIAN_POINT('',(98.4128916636062,-6.92920931711453,0.000661134518076692));
#30966=CARTESIAN_POINT('',(98.2335483363938,-6.92927911623139,0.00329186758170552));
#30967=CARTESIAN_POINT('',(29.75,-6.933,-8.4904762584886E-16));
#30968=CARTESIAN_POINT('Ctrl Pts',(98.4128916636061,-6.92277218803937,0.001783836750055));
#30969=CARTESIAN_POINT('Ctrl Pts',(98.3910522291127,-6.92795854075618,0.764408199582078));
#30970=CARTESIAN_POINT('Ctrl Pts',(98.3692127946193,-6.81209375619514,1.52619914819609));
#30971=CARTESIAN_POINT('Ctrl Pts',(98.3473733601259,-6.56846622737201,2.24537042560992));
#30972=CARTESIAN_POINT('Ctrl Pts',(98.314288092719,-6.19938698490055,3.33486631122398));
#30973=CARTESIAN_POINT('Ctrl Pts',(98.281202825312,-5.53708965775431,4.3265491885863));
#30974=CARTESIAN_POINT('Ctrl Pts',(98.248117557905,-4.68436907918055,5.10626180931842));
#30975=CARTESIAN_POINT('Ctrl Pts',(98.215032290498,-3.83164850060668,5.88597443005063));
#30976=CARTESIAN_POINT('Ctrl Pts',(98.1819470230908,-2.7885046706052,6.45371679415264));
#30977=CARTESIAN_POINT('Ctrl Pts',(98.1488617556838,-1.67315143243921,6.73096598430807));
#30978=CARTESIAN_POINT('Ctrl Pts',(98.1157764882768,-0.557798194273473,
7.00821517446343));
#30979=CARTESIAN_POINT('Ctrl Pts',(98.0826912208698,0.629764452056806,6.99497119067236));
#30980=CARTESIAN_POINT('Ctrl Pts',(98.0496059534628,1.7483153549858,6.70526783617236));
#30981=CARTESIAN_POINT('Ctrl Pts',(98.0165206860558,2.8668662579148,6.41556448167235));
#30982=CARTESIAN_POINT('Ctrl Pts',(97.9834354186488,3.91640541744259,5.8494017564634));
#30983=CARTESIAN_POINT('Ctrl Pts',(97.9503501512418,4.75265142482019,5.05951987470007));
#30984=CARTESIAN_POINT('Ctrl Pts',(97.8841796164277,6.42514343957568,3.47975611117313));
#30985=CARTESIAN_POINT('Ctrl Pts',(97.8180090816137,7.24446284573023,1.00511572142863));
#30986=CARTESIAN_POINT('Ctrl Pts',(97.7518385467997,6.83136924535634,-1.25000734093417));
#30987=CARTESIAN_POINT('Ctrl Pts',(97.6856680119856,6.41827564498251,-3.50513040329671));
#30988=CARTESIAN_POINT('Ctrl Pts',(97.6194974771716,4.7727690380803,-5.54073613827742));
#30989=CARTESIAN_POINT('Ctrl Pts',(97.5533269423575,2.65094026756886,-6.4187834083141));
#30990=CARTESIAN_POINT('Ctrl Pts',(97.4871564075435,0.529111497057312,-7.29683067835084));
#30991=CARTESIAN_POINT('Ctrl Pts',(97.4209858727295,-2.06903943706366,-7.01731948344348));
#30992=CARTESIAN_POINT('Ctrl Pts',(97.3548153379154,-3.95555502426836,-5.70805126072392));
#30993=CARTESIAN_POINT('Ctrl Pts',(97.2908407798123,-5.77946352652212,-4.44223323125975));
#30994=CARTESIAN_POINT('Ctrl Pts',(97.2268662217093,-6.93818647129019,-2.21387236916584));
#30995=CARTESIAN_POINT('Ctrl Pts',(97.1628916636062,-6.94438291503296,0.0033794907004818));
#30996=CARTESIAN_POINT('Ctrl Pts',(96.9835483363938,-6.94194141381233,0.000872210908587178));
#30997=CARTESIAN_POINT('Ctrl Pts',(97.0130683832633,-6.94108255059348,-1.02598458231818));
#30998=CARTESIAN_POINT('Ctrl Pts',(97.0425884301328,-6.69912695613847,-2.05549181351691));
#30999=CARTESIAN_POINT('Ctrl Pts',(97.0721084770023,-6.25348840864668,-2.98514757729132));
#31000=CARTESIAN_POINT('Ctrl Pts',(97.1051937444093,-5.75402881849591,-4.02708052804132));
#31001=CARTESIAN_POINT('Ctrl Pts',(97.1382790118161,-4.99871659239096,-4.94358687453451));
#31002=CARTESIAN_POINT('Ctrl Pts',(97.1713642792231,-4.06784541551554,-5.61764830451808));
#31003=CARTESIAN_POINT('Ctrl Pts',(97.2044495466301,-3.13697423864023,-6.29170973450157));
#31004=CARTESIAN_POINT('Ctrl Pts',(97.2375348140372,-2.03054411099448,-6.7233262479755));
#31005=CARTESIAN_POINT('Ctrl Pts',(97.2706200814443,-0.884785181006302,
-6.87272715293996));
#31006=CARTESIAN_POINT('Ctrl Pts',(97.3037053488513,0.260973748982006,-7.02212805790444));
#31007=CARTESIAN_POINT('Ctrl Pts',(97.3367906162583,1.44606148131276,-6.88931335435939));
#31008=CARTESIAN_POINT('Ctrl Pts',(97.3698758836653,2.51694132343833,-6.46926914749254));
#31009=CARTESIAN_POINT('Ctrl Pts',(97.4360464184792,4.65870100768948,-5.62918073375883));
#31010=CARTESIAN_POINT('Ctrl Pts',(97.5022169532934,6.34362913111992,-3.64017430673796));
#31011=CARTESIAN_POINT('Ctrl Pts',(97.5683874881074,6.80342467766202,-1.39410787752219));
#31012=CARTESIAN_POINT('Ctrl Pts',(97.6345580229215,7.26322022420409,0.851958551693452));
#31013=CARTESIAN_POINT('Ctrl Pts',(97.7007285577355,6.49788319385797,3.35508498310395));
#31014=CARTESIAN_POINT('Ctrl Pts',(97.7668990925495,4.85806604502377,4.96260607415636));
#31015=CARTESIAN_POINT('Ctrl Pts',(97.8330696273635,3.21824889618947,6.57012716520887));
#31016=CARTESIAN_POINT('Ctrl Pts',(97.8992401621775,0.703951628866997,7.28204291590319));
#31017=CARTESIAN_POINT('Ctrl Pts',(97.9654106969916,-1.53520881853428,6.77284272876324));
#31018=CARTESIAN_POINT('Ctrl Pts',(98.0315812318057,-3.77436926593531,6.26364254162335));
#31019=CARTESIAN_POINT('Ctrl Pts',(98.0977517666198,-5.73839289341521,4.53332641664947));
#31020=CARTESIAN_POINT('Ctrl Pts',(98.1639223014338,-6.52437983792119,2.37962010609202));
#31021=CARTESIAN_POINT('Ctrl Pts',(98.1871309797538,-6.80005719507182,1.62422834300578));
#31022=CARTESIAN_POINT('Ctrl Pts',(98.2103396580738,-6.93081387900884,0.81675162228316));
#31023=CARTESIAN_POINT('Ctrl Pts',(98.2335483363938,-6.92470486363958,0.00733871095478924));
#31024=CARTESIAN_POINT('Origin',(29.75,0.,0.));
#31025=CARTESIAN_POINT('',(99.6628916636061,-6.933,4.46781500684779E-12));
#31026=CARTESIAN_POINT('',(99.4835483363938,-6.92933028435402,-0.00338549438887613));
#31027=CARTESIAN_POINT('',(29.75,-6.933,-8.4904762584886E-16));
#31028=CARTESIAN_POINT('Ctrl Pts',(99.6628916636061,-6.933,5.25579579857549E-12));
#31029=CARTESIAN_POINT('Ctrl Pts',(99.605667468321,-6.93299999999849,1.99420935702147));
#31030=CARTESIAN_POINT('Ctrl Pts',(99.548443273036,-6.02307502628955,3.97063309653488));
#31031=CARTESIAN_POINT('Ctrl Pts',(99.4912190777509,-4.507984847536,5.26731066241453));
#31032=CARTESIAN_POINT('Ctrl Pts',(99.4339948824658,-2.99289466878246,6.56398822829418));
#31033=CARTESIAN_POINT('Ctrl Pts',(99.3767706871807,-0.899664345623711,
7.15779044292472));
#31034=CARTESIAN_POINT('Ctrl Pts',(99.3195464918956,1.07062371682325,6.84983604599231));
#31035=CARTESIAN_POINT('Ctrl Pts',(99.2623222966105,3.04091177927021,6.5418816490599));
#31036=CARTESIAN_POINT('Ctrl Pts',(99.2050981013254,4.85311303640243,5.33766370386068));
#31037=CARTESIAN_POINT('Ctrl Pts',(99.1478739060403,5.90026971494006,3.64050907030337));
#31038=CARTESIAN_POINT('Ctrl Pts',(99.0906497107552,6.94742639347769,1.94335443674606));
#31039=CARTESIAN_POINT('Ctrl Pts',(99.0334255154701,7.21086008527494,-0.216464293128621));
#31040=CARTESIAN_POINT('Ctrl Pts',(98.976201320185,6.60233935005946,-2.11556236179801));
#31041=CARTESIAN_POINT('Ctrl Pts',(98.9189771248999,5.99381861484398,-4.01466043046741));
#31042=CARTESIAN_POINT('Ctrl Pts',(98.8617529296148,4.52419779646946,-5.61916312790721));
#31043=CARTESIAN_POINT('Ctrl Pts',(98.8045287343297,2.68569473000012,-6.39167683923785));
#31044=CARTESIAN_POINT('Ctrl Pts',(98.7473045390446,0.847191663530777,-7.1641905505685));
#31045=CARTESIAN_POINT('Ctrl Pts',(98.6900803437595,-1.32739978994589,-7.09093574623707));
#31046=CARTESIAN_POINT('Ctrl Pts',(98.6328561484744,-3.10974706736552,-6.19644754492536));
#31047=CARTESIAN_POINT('Ctrl Pts',(98.5756319531893,-4.89209434478515,-5.30195934361366));
#31048=CARTESIAN_POINT('Ctrl Pts',(98.5184077579043,-6.25040525058856,-3.60219296582318));
#31049=CARTESIAN_POINT('Ctrl Pts',(98.4611835626192,-6.72974280712855,-1.66644854403055));
#31050=CARTESIAN_POINT('Ctrl Pts',(98.4450862629482,-6.86458158035639,-1.12191912096339));
#31051=CARTESIAN_POINT('Ctrl Pts',(98.4289889632772,-6.93300000000035,-0.560975745773916));
#31052=CARTESIAN_POINT('Ctrl Pts',(98.4128916636062,-6.933,4.31821245427955E-12));
#31053=CARTESIAN_POINT('Ctrl Pts',(98.2335483363938,-6.933,-7.69384556065233E-13));
#31054=CARTESIAN_POINT('Ctrl Pts',(98.2907725316789,-6.93299999999978,-1.99420935701711));
#31055=CARTESIAN_POINT('Ctrl Pts',(98.347996726964,-6.02307502629199,-3.97063309653124));
#31056=CARTESIAN_POINT('Ctrl Pts',(98.4052209222491,-4.50798484753911,-5.26731066241187));
#31057=CARTESIAN_POINT('Ctrl Pts',(98.4624451175342,-2.99289466878623,-6.5639882282925));
#31058=CARTESIAN_POINT('Ctrl Pts',(98.5196693128193,-0.89966434562766,-7.15779044292426));
#31059=CARTESIAN_POINT('Ctrl Pts',(98.5768935081044,1.0706237168196,-6.84983604599288));
#31060=CARTESIAN_POINT('Ctrl Pts',(98.6341177033895,3.04091177926685,-6.5418816490615));
#31061=CARTESIAN_POINT('Ctrl Pts',(98.6913418986746,4.85311303639982,-5.33766370386311));
#31062=CARTESIAN_POINT('Ctrl Pts',(98.7485660939597,5.90026971493833,-3.64050907030619));
#31063=CARTESIAN_POINT('Ctrl Pts',(98.8057902892448,6.94742639347683,-1.94335443674926));
#31064=CARTESIAN_POINT('Ctrl Pts',(98.8630144845299,7.21086008527507,0.216464293125468));
#31065=CARTESIAN_POINT('Ctrl Pts',(98.920238679815,6.60233935006035,2.11556236179524));
#31066=CARTESIAN_POINT('Ctrl Pts',(98.9774628751001,5.99381861484563,4.01466043046502));
#31067=CARTESIAN_POINT('Ctrl Pts',(99.0346870703851,4.52419779647162,5.61916312790552));
#31068=CARTESIAN_POINT('Ctrl Pts',(99.0919112656702,2.68569473000244,6.39167683923688));
#31069=CARTESIAN_POINT('Ctrl Pts',(99.1491354609553,0.847191663533256,7.16419055056824));
#31070=CARTESIAN_POINT('Ctrl Pts',(99.2063596562404,-1.32739978994361,7.09093574623753));
#31071=CARTESIAN_POINT('Ctrl Pts',(99.2635838515255,-3.10974706736363,6.19644754492631));
#31072=CARTESIAN_POINT('Ctrl Pts',(99.3208080468106,-4.89209434478364,5.30195934361509));
#31073=CARTESIAN_POINT('Ctrl Pts',(99.3780322420957,-6.25040525058763,3.60219296582487));
#31074=CARTESIAN_POINT('Ctrl Pts',(99.4352564373808,-6.72974280712813,1.66644854403223));
#31075=CARTESIAN_POINT('Ctrl Pts',(99.4513537370518,-6.86458158035598,1.12191912096561));
#31076=CARTESIAN_POINT('Ctrl Pts',(99.4674510367228,-6.93300000000008,0.560975745776695));
#31077=CARTESIAN_POINT('Ctrl Pts',(99.4835483363938,-6.933,-1.01391117723892E-12));
#31078=CARTESIAN_POINT('Origin',(29.75,0.,0.));
#31079=CARTESIAN_POINT('',(100.912891663606,-6.933,5.40539835114373E-12));
#31080=CARTESIAN_POINT('',(100.733548336394,-6.94397743835492,-0.00162794009456958));
#31081=CARTESIAN_POINT('',(29.75,-6.933,-8.4904762584886E-16));
#31082=CARTESIAN_POINT('Ctrl Pts',(100.912891663606,-6.93501187936537,-0.00181345658265553));
#31083=CARTESIAN_POINT('Ctrl Pts',(100.884850580955,-6.93263583601006,0.972625129661142));
#31084=CARTESIAN_POINT('Ctrl Pts',(100.856809498304,-6.71995816851569,1.94841025277312));
#31085=CARTESIAN_POINT('Ctrl Pts',(100.828768415652,-6.31974308779576,2.84219468712902));
#31086=CARTESIAN_POINT('Ctrl Pts',(100.795683148245,-5.84753510885921,3.89675799991803));
#31087=CARTESIAN_POINT('Ctrl Pts',(100.762597880838,-5.11425070045544,4.83716570681445));
#31088=CARTESIAN_POINT('Ctrl Pts',(100.729512613431,-4.1959559550899,5.52995393753654));
#31089=CARTESIAN_POINT('Ctrl Pts',(100.663342078617,-2.35936646435863,6.91553039898088));
#31090=CARTESIAN_POINT('Ctrl Pts',(100.597171543803,0.217264374219888,7.31062895572762));
#31091=CARTESIAN_POINT('Ctrl Pts',(100.531001008989,2.37189911809706,6.52719071977832));
#31092=CARTESIAN_POINT('Ctrl Pts',(100.464830474175,4.52653386197423,5.74375248382901));
#31093=CARTESIAN_POINT('Ctrl Pts',(100.398659939361,6.25917251115006,3.78177745518367));
#31094=CARTESIAN_POINT('Ctrl Pts',(100.332489404547,6.77102160540967,1.54322103541326));
#31095=CARTESIAN_POINT('Ctrl Pts',(100.266318869733,7.28287069966925,-0.695335384357018));
#31096=CARTESIAN_POINT('Ctrl Pts',(100.200148334919,6.57393023901274,-3.21047319525232));
#31097=CARTESIAN_POINT('Ctrl Pts',(100.133977800105,4.96835042337348,-4.85219113552126));
#31098=CARTESIAN_POINT('Ctrl Pts',(100.067807265291,3.36277060773414,-6.49390907579028));
#31099=CARTESIAN_POINT('Ctrl Pts',(100.001636730477,0.860551437111937,-7.26220714543285));
#31100=CARTESIAN_POINT('Ctrl Pts',(99.9354661956629,-1.38605742730384,-6.80506935504743));
#31101=CARTESIAN_POINT('Ctrl Pts',(99.8692956608489,-3.63266629171949,-6.34793156466204));
#31102=CARTESIAN_POINT('Ctrl Pts',(99.8031251260347,-5.62366484992875,-4.66535791424881));
#31103=CARTESIAN_POINT('Ctrl Pts',(99.7369545912207,-6.46628669943668,-2.52459367998469));
#31104=CARTESIAN_POINT('Ctrl Pts',(99.7122669486825,-6.78066147476532,-1.72589343791122));
#31105=CARTESIAN_POINT('Ctrl Pts',(99.6875793061444,-6.93518562941577,-0.863414429982868));
#31106=CARTESIAN_POINT('Ctrl Pts',(99.6628916636062,-6.93186678979006,-0.000948267261432489));
#31107=CARTESIAN_POINT('Ctrl Pts',(99.4835483363938,-6.92482311535644,-0.00754358095680571));
#31108=CARTESIAN_POINT('Ctrl Pts',(99.5068667351054,-6.93021552428664,-0.822381842477515));
#31109=CARTESIAN_POINT('Ctrl Pts',(99.5301851338169,-6.79757852095591,-1.63512275943323));
#31110=CARTESIAN_POINT('Ctrl Pts',(99.5535035325285,-6.51926479436836,-2.39359784836531));
#31111=CARTESIAN_POINT('Ctrl Pts',(99.6196740673425,-5.72949494944151,-4.54591983661744));
#31112=CARTESIAN_POINT('Ctrl Pts',(99.6858446021565,-3.76666029668156,-6.26126512949026));
#31113=CARTESIAN_POINT('Ctrl Pts',(99.7520151369706,-1.52353023483686,-6.7723919372603));
#31114=CARTESIAN_POINT('Ctrl Pts',(99.7851004043776,-0.401965203914322,
-7.02795534114536));
#31115=CARTESIAN_POINT('Ctrl Pts',(99.8181856717847,0.789673679279438,-6.98246412375461));
#31116=CARTESIAN_POINT('Ctrl Pts',(99.8512709391917,1.90031642472727,-6.66378427180821));
#31117=CARTESIAN_POINT('Ctrl Pts',(99.8843562065988,3.01095917017484,-6.34510441986188));
#31118=CARTESIAN_POINT('Ctrl Pts',(99.9174414740057,4.04060577787652,-5.75323593336004));
#31119=CARTESIAN_POINT('Ctrl Pts',(99.9505267414127,4.86048491773434,-4.94783034897748));
#31120=CARTESIAN_POINT('Ctrl Pts',(99.9836120088197,5.68036405759236,-4.14242476459473));
#31121=CARTESIAN_POINT('Ctrl Pts',(100.016697276227,6.29047572960643,-3.12348208233117));
#31122=CARTESIAN_POINT('Ctrl Pts',(100.049782543634,6.6288845593698,-2.01869087129143));
#31123=CARTESIAN_POINT('Ctrl Pts',(100.082867811041,6.9672933891331,-0.913899660251946));
#31124=CARTESIAN_POINT('Ctrl Pts',(100.115953078448,7.03399937664582,0.276740079563676));
#31125=CARTESIAN_POINT('Ctrl Pts',(100.149038345855,6.79845053797514,1.40267858436484));
#31126=CARTESIAN_POINT('Ctrl Pts',(100.215208880669,6.32735286063373,3.65455559396744));
#31127=CARTESIAN_POINT('Ctrl Pts',(100.281379415483,4.64723587855842,5.64762766351217));
#31128=CARTESIAN_POINT('Ctrl Pts',(100.347549950297,2.5093203053586,6.4756031166143));
#31129=CARTESIAN_POINT('Ctrl Pts',(100.413720485111,0.371404732158899,7.30357856971639));
#31130=CARTESIAN_POINT('Ctrl Pts',(100.479891019925,-2.22430943216523,6.96645740637609));
#31131=CARTESIAN_POINT('Ctrl Pts',(100.546061554739,-4.08281761268181,5.61772775120349));
#31132=CARTESIAN_POINT('Ctrl Pts',(100.608557148624,-5.83810903971579,4.34390306432321));
#31133=CARTESIAN_POINT('Ctrl Pts',(100.671052742509,-6.93580568086616,2.16771393087575));
#31134=CARTESIAN_POINT('Ctrl Pts',(100.733548336394,-6.94397743835492,-0.00162794009456958));
#31135=CARTESIAN_POINT('Origin',(29.75,0.,0.));
#31136=CARTESIAN_POINT('',(102.162891663606,-6.933,4.76702011198427E-12));
#31137=CARTESIAN_POINT('',(101.983548336394,-6.93371908702931,0.00569271503419462));
#31138=CARTESIAN_POINT('',(29.75,-6.933,-8.4904762584886E-16));
#31139=CARTESIAN_POINT('Ctrl Pts',(102.162891663606,-6.933,4.76702011198427E-12));
#31140=CARTESIAN_POINT('Ctrl Pts',(102.105667468321,-6.93299999999863,1.99420935702098));
#31141=CARTESIAN_POINT('Ctrl Pts',(102.048443273036,-6.02307502628983,3.97063309653446));
#31142=CARTESIAN_POINT('Ctrl Pts',(101.991219077751,-4.50798484753637,5.26731066241421));
#31143=CARTESIAN_POINT('Ctrl Pts',(101.933994882466,-2.99289466878292,6.56398822829397));
#31144=CARTESIAN_POINT('Ctrl Pts',(101.876770687181,-0.899664345624216,
7.15779044292466));
#31145=CARTESIAN_POINT('Ctrl Pts',(101.819546491896,1.07062371682277,6.84983604599239));
#31146=CARTESIAN_POINT('Ctrl Pts',(101.76232229661,3.04091177926975,6.54188164906011));
#31147=CARTESIAN_POINT('Ctrl Pts',(101.705098101325,4.85311303640206,5.33766370386103));
#31148=CARTESIAN_POINT('Ctrl Pts',(101.64787390604,5.9002697149398,3.64050907030379));
#31149=CARTESIAN_POINT('Ctrl Pts',(101.590649710755,6.94742639347755,1.94335443674655));
#31150=CARTESIAN_POINT('Ctrl Pts',(101.53342551547,7.21086008527496,-0.216464293128111));
#31151=CARTESIAN_POINT('Ctrl Pts',(101.476201320185,6.60233935005961,-2.11556236179755));
#31152=CARTESIAN_POINT('Ctrl Pts',(101.4189771249,5.99381861484427,-4.01466043046699));
#31153=CARTESIAN_POINT('Ctrl Pts',(101.361752929615,4.52419779646985,-5.61916312790689));
#31154=CARTESIAN_POINT('Ctrl Pts',(101.30452873433,2.68569473000057,-6.39167683923766));
#31155=CARTESIAN_POINT('Ctrl Pts',(101.247304539045,0.847191663531283,-7.16419055056844));
#31156=CARTESIAN_POINT('Ctrl Pts',(101.19008034376,-1.32739978994539,-7.09093574623716));
#31157=CARTESIAN_POINT('Ctrl Pts',(101.132856148474,-3.10974706736508,-6.19644754492558));
#31158=CARTESIAN_POINT('Ctrl Pts',(101.075631953189,-4.89209434478478,-5.301959343614));
#31159=CARTESIAN_POINT('Ctrl Pts',(101.018407757904,-6.2504052505883,-3.60219296582362));
#31160=CARTESIAN_POINT('Ctrl Pts',(100.961183562619,-6.72974280712843,-1.66644854403103));
#31161=CARTESIAN_POINT('Ctrl Pts',(100.945086262948,-6.86458158035643,-1.12191912096336));
#31162=CARTESIAN_POINT('Ctrl Pts',(100.928988963277,-6.93300000000044,-0.560975745773355));
#31163=CARTESIAN_POINT('Ctrl Pts',(100.912891663606,-6.933,5.40539835114373E-12));
#31164=CARTESIAN_POINT('Ctrl Pts',(100.733548336394,-6.94397743835492,-0.00162794009456958));
#31165=CARTESIAN_POINT('Ctrl Pts',(100.737223277323,-6.94445796384787,-0.129192184793122));
#31166=CARTESIAN_POINT('Ctrl Pts',(100.740898218252,-6.94117111235913,-0.256732752915367));
#31167=CARTESIAN_POINT('Ctrl Pts',(100.744573159181,-6.93402905925297,-0.384064773836234));
#31168=CARTESIAN_POINT('Ctrl Pts',(100.810743693995,-6.8054301285985,-2.6767894966986));
#31169=CARTESIAN_POINT('Ctrl Pts',(100.876914228809,-5.42693007058041,-4.9019007954182));
#31170=CARTESIAN_POINT('Ctrl Pts',(100.943084763623,-3.4344862106255,-6.03609381867223));
#31171=CARTESIAN_POINT('Ctrl Pts',(101.009255298437,-1.44204235067071,-7.1702868419262));
#31172=CARTESIAN_POINT('Ctrl Pts',(101.075425833251,1.16434531122071,-7.21356158971465));
#31173=CARTESIAN_POINT('Ctrl Pts',(101.141596368065,3.20756104559799,-6.15613426324448));
#31174=CARTESIAN_POINT('Ctrl Pts',(101.174681635472,4.22916891278669,-5.62742060000936));
#31175=CARTESIAN_POINT('Ctrl Pts',(101.207766902879,5.10998379809678,-4.82353141820959));
#31176=CARTESIAN_POINT('Ctrl Pts',(101.240852170286,5.75260410317904,-3.86325890504045));
#31177=CARTESIAN_POINT('Ctrl Pts',(101.273937437693,6.39522440826123,-2.90298639187141));
#31178=CARTESIAN_POINT('Ctrl Pts',(101.3070227051,6.79965013311558,-1.78633054733313));
#31179=CARTESIAN_POINT('Ctrl Pts',(101.340107972508,6.90602743040454,-0.641968790741197));
#31180=CARTESIAN_POINT('Ctrl Pts',(101.373193239915,7.01240472769351,0.502392965850864));
#31181=CARTESIAN_POINT('Ctrl Pts',(101.406278507322,6.82073359741688,1.67446063449685));
#31182=CARTESIAN_POINT('Ctrl Pts',(101.439363774729,6.36612416211952,2.73672915864262));
#31183=CARTESIAN_POINT('Ctrl Pts',(101.472449042136,5.9115147268222,3.79899768278826));
#31184=CARTESIAN_POINT('Ctrl Pts',(101.505534309543,5.19396698650421,4.75146706243399));
#31185=CARTESIAN_POINT('Ctrl Pts',(101.53861957695,4.2873175361163,5.45942719274101));
#31186=CARTESIAN_POINT('Ctrl Pts',(101.604790111764,2.47401863534027,6.8753474533552));
#31187=CARTESIAN_POINT('Ctrl Pts',(101.670960646578,-0.0956871057154265,
7.31323071661412));
#31188=CARTESIAN_POINT('Ctrl Pts',(101.737131181392,-2.2630495505609,6.56572393955883));
#31189=CARTESIAN_POINT('Ctrl Pts',(101.803301716206,-4.43041199540625,5.81821716250359));
#31190=CARTESIAN_POINT('Ctrl Pts',(101.86947225102,-6.19543114404131,3.88532034513432));
#31191=CARTESIAN_POINT('Ctrl Pts',(101.935642785834,-6.7444279485813,1.6555833991261));
#31192=CARTESIAN_POINT('Ctrl Pts',(101.951611302687,-6.87691387680221,1.1174950777781));
#31193=CARTESIAN_POINT('Ctrl Pts',(101.967579819541,-6.9385821686616,0.562119642924724));
#31194=CARTESIAN_POINT('Ctrl Pts',(101.983548336394,-6.93371908702931,0.00569271503419462));
#31195=CARTESIAN_POINT('Origin',(29.75,0.,0.));
#31196=CARTESIAN_POINT('',(103.412891663606,-6.933,4.91634510879635E-12));
#31197=CARTESIAN_POINT('',(103.233548336394,-6.92083937541073,0.000353000077293465));
#31198=CARTESIAN_POINT('',(29.75,-6.933,-8.4904762584886E-16));
#31199=CARTESIAN_POINT('Ctrl Pts',(103.412891663606,-6.933,4.91634510879635E-12));
#31200=CARTESIAN_POINT('Ctrl Pts',(103.355667468321,-6.93299999999859,1.99420935702113));
#31201=CARTESIAN_POINT('Ctrl Pts',(103.298443273036,-6.02307502628974,3.97063309653459));
#31202=CARTESIAN_POINT('Ctrl Pts',(103.241219077751,-4.50798484753626,5.26731066241431));
#31203=CARTESIAN_POINT('Ctrl Pts',(103.183994882466,-2.99289466878278,6.56398822829403));
#31204=CARTESIAN_POINT('Ctrl Pts',(103.126770687181,-0.899664345624063,
7.15779044292468));
#31205=CARTESIAN_POINT('Ctrl Pts',(103.069546491896,1.07062371682291,6.84983604599236));
#31206=CARTESIAN_POINT('Ctrl Pts',(103.01232229661,3.04091177926989,6.54188164906005));
#31207=CARTESIAN_POINT('Ctrl Pts',(102.955098101325,4.85311303640217,5.33766370386092));
#31208=CARTESIAN_POINT('Ctrl Pts',(102.89787390604,5.90026971493988,3.64050907030366));
#31209=CARTESIAN_POINT('Ctrl Pts',(102.840649710755,6.94742639347759,1.9433544367464));
#31210=CARTESIAN_POINT('Ctrl Pts',(102.78342551547,7.21086008527495,-0.216464293128266));
#31211=CARTESIAN_POINT('Ctrl Pts',(102.726201320185,6.60233935005957,-2.11556236179769));
#31212=CARTESIAN_POINT('Ctrl Pts',(102.6689771249,5.99381861484418,-4.01466043046711));
#31213=CARTESIAN_POINT('Ctrl Pts',(102.611752929615,4.52419779646973,-5.61916312790699));
#31214=CARTESIAN_POINT('Ctrl Pts',(102.55452873433,2.68569473000043,-6.39167683923772));
#31215=CARTESIAN_POINT('Ctrl Pts',(102.497304539045,0.847191663531128,-7.16419055056846));
#31216=CARTESIAN_POINT('Ctrl Pts',(102.44008034376,-1.32739978994555,-7.09093574623713));
#31217=CARTESIAN_POINT('Ctrl Pts',(102.382856148474,-3.10974706736522,-6.19644754492551));
#31218=CARTESIAN_POINT('Ctrl Pts',(102.325631953189,-4.89209434478489,-5.3019593436139));
#31219=CARTESIAN_POINT('Ctrl Pts',(102.268407757904,-6.25040525058838,-3.60219296582349));
#31220=CARTESIAN_POINT('Ctrl Pts',(102.211183562619,-6.72974280712847,-1.66644854403088));
#31221=CARTESIAN_POINT('Ctrl Pts',(102.195086262948,-6.8645815803564,-1.12191912096347));
#31222=CARTESIAN_POINT('Ctrl Pts',(102.178988963277,-6.93300000000039,-0.560975745773731));
#31223=CARTESIAN_POINT('Ctrl Pts',(102.162891663606,-6.933,4.76702011198427E-12));
#31224=CARTESIAN_POINT('Ctrl Pts',(101.983548336394,-6.93371908702931,0.00569271503419462));
#31225=CARTESIAN_POINT('Ctrl Pts',(102.033750354355,-6.91843047170635,-1.74360904444629));
#31226=CARTESIAN_POINT('Ctrl Pts',(102.083952372315,-6.24557536097976,-3.5033032932907));
#31227=CARTESIAN_POINT('Ctrl Pts',(102.134154390276,-5.0483366904737,-4.7689161666655));
#31228=CARTESIAN_POINT('Ctrl Pts',(102.20032492509,-3.47027416738121,-6.4371017118016));
#31229=CARTESIAN_POINT('Ctrl Pts',(102.266495459904,-0.981174660751704,
-7.24689572742639));
#31230=CARTESIAN_POINT('Ctrl Pts',(102.332665994718,1.27272408831404,-6.82717346445915));
#31231=CARTESIAN_POINT('Ctrl Pts',(102.398836529532,3.52662283737954,-6.40745120149195));
#31232=CARTESIAN_POINT('Ctrl Pts',(102.465007064346,5.54532082888111,-4.75821265993281));
#31233=CARTESIAN_POINT('Ctrl Pts',(102.53117759916,6.42341876570948,-2.63175384271813));
#31234=CARTESIAN_POINT('Ctrl Pts',(102.564262866567,6.86246773412369,-1.56852443411073));
#31235=CARTESIAN_POINT('Ctrl Pts',(102.597348133974,7.01636668886959,-0.385989956589359));
#31236=CARTESIAN_POINT('Ctrl Pts',(102.630433401381,6.8873943833032,0.762247954493993));
#31237=CARTESIAN_POINT('Ctrl Pts',(102.663518668788,6.75842207773681,1.91048586557734));
#31238=CARTESIAN_POINT('Ctrl Pts',(102.696603936195,6.34657851185811,3.02442721022279));
#31239=CARTESIAN_POINT('Ctrl Pts',(102.729689203602,5.68920193750754,3.96715516611671));
#31240=CARTESIAN_POINT('Ctrl Pts',(102.762774471009,5.03182536315704,4.90988312201052));
#31241=CARTESIAN_POINT('Ctrl Pts',(102.795859738416,4.12891578033466,5.68139768915293));
#31242=CARTESIAN_POINT('Ctrl Pts',(102.828945005823,3.09604298671421,6.19933392871387));
#31243=CARTESIAN_POINT('Ctrl Pts',(102.86203027323,2.06317019309352,6.71727016827494));
#31244=CARTESIAN_POINT('Ctrl Pts',(102.895115540637,0.900334188675,6.98162808025441));
#31245=CARTESIAN_POINT('Ctrl Pts',(102.928200808044,-0.249119839419829,
6.93717350467326));
#31246=CARTESIAN_POINT('Ctrl Pts',(102.994371342858,-2.54802789560923,6.84826435351098));
#31247=CARTESIAN_POINT('Ctrl Pts',(103.060541877673,-4.79340804650275,5.52410525210601));
#31248=CARTESIAN_POINT('Ctrl Pts',(103.126712412487,-5.96636769431135,3.55423418686299));
#31249=CARTESIAN_POINT('Ctrl Pts',(103.162324387122,-6.59763672279808,2.49407956353618));
#31250=CARTESIAN_POINT('Ctrl Pts',(103.197936361758,-6.91828681390554,1.24689908283008));
#31251=CARTESIAN_POINT('Ctrl Pts',(103.233548336394,-6.92083937541073,0.000353000077293465));
#31252=CARTESIAN_POINT('Origin',(29.75,0.,0.));
#31253=CARTESIAN_POINT('',(104.662891663606,-6.93409162044397,-0.00297428074398909));
#31254=CARTESIAN_POINT('',(104.483548336394,-6.93479064018689,-0.00208547980832093));
#31255=CARTESIAN_POINT('',(29.75,-6.933,-8.4904762584886E-16));
#31256=CARTESIAN_POINT('Ctrl Pts',(104.662891663606,-6.933,5.06567010560843E-12));
#31257=CARTESIAN_POINT('Ctrl Pts',(104.605667468321,-6.93299999999854,1.99420935702154));
#31258=CARTESIAN_POINT('Ctrl Pts',(104.548443273036,-6.0230750262894,3.97063309653523));
#31259=CARTESIAN_POINT('Ctrl Pts',(104.491219077751,-4.50798484753555,5.26731066241492));
#31260=CARTESIAN_POINT('Ctrl Pts',(104.433994882466,-2.99289466878169,6.56398822829461));
#31261=CARTESIAN_POINT('Ctrl Pts',(104.376770687181,-0.89966434562254,7.15779044292494));
#31262=CARTESIAN_POINT('Ctrl Pts',(104.319546491896,1.07062371682462,6.8498360459921));
#31263=CARTESIAN_POINT('Ctrl Pts',(104.26232229661,3.04091177927178,6.54188164905925));
#31264=CARTESIAN_POINT('Ctrl Pts',(104.205098101325,4.85311303640397,5.33766370385939));
#31265=CARTESIAN_POINT('Ctrl Pts',(104.14787390604,5.9002697149412,3.64050907030152));
#31266=CARTESIAN_POINT('Ctrl Pts',(104.090649710755,6.94742639347844,1.94335443674366));
#31267=CARTESIAN_POINT('Ctrl Pts',(104.03342551547,7.21086008527493,-0.216464293131451));
#31268=CARTESIAN_POINT('Ctrl Pts',(103.976201320185,6.60233935005856,-2.11556236180084));
#31269=CARTESIAN_POINT('Ctrl Pts',(103.9189771249,5.99381861484219,-4.01466043047022));
#31270=CARTESIAN_POINT('Ctrl Pts',(103.861752929615,4.52419779646666,-5.61916312790956));
#31271=CARTESIAN_POINT('Ctrl Pts',(103.80452873433,2.68569472999666,-6.39167683923931));
#31272=CARTESIAN_POINT('Ctrl Pts',(103.747304539045,0.847191663526659,-7.16419055056906));
#31273=CARTESIAN_POINT('Ctrl Pts',(103.690080343759,-1.3273997899503,-7.09093574623631));
#31274=CARTESIAN_POINT('Ctrl Pts',(103.632856148474,-3.10974706736958,-6.19644754492333));
#31275=CARTESIAN_POINT('Ctrl Pts',(103.575631953189,-4.89209434478886,-5.30195934361034));
#31276=CARTESIAN_POINT('Ctrl Pts',(103.518407757904,-6.25040525059126,-3.60219296581864));
#31277=CARTESIAN_POINT('Ctrl Pts',(103.461183562619,-6.72974280712983,-1.66644854402538));
#31278=CARTESIAN_POINT('Ctrl Pts',(103.445086262948,-6.86458158035687,-1.12191912095965));
#31279=CARTESIAN_POINT('Ctrl Pts',(103.428988963277,-6.9330000000004,-0.560975745771742));
#31280=CARTESIAN_POINT('Ctrl Pts',(103.412891663606,-6.933,4.91634510879635E-12));
#31281=CARTESIAN_POINT('Ctrl Pts',(103.233548336394,-6.92083937541073,0.000353000077293465));
#31282=CARTESIAN_POINT('Ctrl Pts',(103.264106896572,-6.92302972304416,-1.06930555928247));
#31283=CARTESIAN_POINT('Ctrl Pts',(103.29466545675,-6.69099468583458,-2.13849699113908));
#31284=CARTESIAN_POINT('Ctrl Pts',(103.325224016929,-6.22000895328616,-3.08864911670163));
#31285=CARTESIAN_POINT('Ctrl Pts',(103.391394551743,-5.20015141972855,-5.14607832594236));
#31286=CARTESIAN_POINT('Ctrl Pts',(103.457565086557,-3.05989720788957,-6.64535371534269));
#31287=CARTESIAN_POINT('Ctrl Pts',(103.523735621371,-0.777838836008096,
-6.9009587370364));
#31288=CARTESIAN_POINT('Ctrl Pts',(103.589906156185,1.50421953587338,-7.15656375873012));
#31289=CARTESIAN_POINT('Ctrl Pts',(103.656076690999,3.92808206779747,-6.16849841271689));
#31290=CARTESIAN_POINT('Ctrl Pts',(103.722247225813,5.37870678028656,-4.39313526885716));
#31291=CARTESIAN_POINT('Ctrl Pts',(103.788417760627,6.82933149277582,-2.61777212499723));
#31292=CARTESIAN_POINT('Ctrl Pts',(103.854588295441,7.30671838583013,-0.0551111832906592));
#31293=CARTESIAN_POINT('Ctrl Pts',(103.920758830255,6.60489006341062,2.13585209660723));
#31294=CARTESIAN_POINT('Ctrl Pts',(103.953844097662,6.25397590220092,3.23133373655599));
#31295=CARTESIAN_POINT('Ctrl Pts',(103.986929365069,5.60825793712291,4.23389096105253));
#31296=CARTESIAN_POINT('Ctrl Pts',(104.020014632476,4.76861880313492,5.0276732238417));
#31297=CARTESIAN_POINT('Ctrl Pts',(104.053099899883,3.92897966914701,5.82145548663078));
#31298=CARTESIAN_POINT('Ctrl Pts',(104.08618516729,2.89541936624924,6.40646278771246));
#31299=CARTESIAN_POINT('Ctrl Pts',(104.119270434697,1.78482986806082,6.70221762849317));
#31300=CARTESIAN_POINT('Ctrl Pts',(104.152355702104,0.674240369872153,6.99797246927394));
#31301=CARTESIAN_POINT('Ctrl Pts',(104.185440969511,-0.513378323607498,
7.00447484975354));
#31302=CARTESIAN_POINT('Ctrl Pts',(104.218526236918,-1.63659125345655,6.73340867650101));
#31303=CARTESIAN_POINT('Ctrl Pts',(104.251611504325,-2.75980418330561,6.46234250324848));
#31304=CARTESIAN_POINT('Ctrl Pts',(104.284696771732,-3.81861134952433,5.91370777626388));
#31305=CARTESIAN_POINT('Ctrl Pts',(104.317782039139,-4.66787442237867,5.13783858297635));
#31306=CARTESIAN_POINT('Ctrl Pts',(104.373037471557,-6.08622168099608,3.84206583773441));
#31307=CARTESIAN_POINT('Ctrl Pts',(104.428292903976,-6.92010719630414,1.91248924632851));
#31308=CARTESIAN_POINT('Ctrl Pts',(104.483548336394,-6.93794935432642,-0.0057642951309926));
#31309=CARTESIAN_POINT('Origin',(29.75,0.,0.));
#31310=CARTESIAN_POINT('',(105.912891663606,-6.94073003849348,0.00450623896247018));
#31311=CARTESIAN_POINT('',(105.733548336394,-6.93358984723115,0.000731892616234763));
#31312=CARTESIAN_POINT('',(29.75,-6.933,-8.4904762584886E-16));
#31313=CARTESIAN_POINT('Ctrl Pts',(105.912891663606,-6.94073003849348,0.00450623896247018));
#31314=CARTESIAN_POINT('Ctrl Pts',(105.905532552046,-6.94274293080495,0.260275666085527));
#31315=CARTESIAN_POINT('Ctrl Pts',(105.898173440486,-6.9300008501143,0.515842442486986));
#31316=CARTESIAN_POINT('Ctrl Pts',(105.890814328926,-6.90187421034804,0.769673494383096));
#31317=CARTESIAN_POINT('Ctrl Pts',(105.824643794112,-6.64896938879624,3.05203276010309));
#31318=CARTESIAN_POINT('Ctrl Pts',(105.758473259298,-5.15222728481638,5.19405918682688));
#31319=CARTESIAN_POINT('Ctrl Pts',(105.692302724484,-3.09600615901486,6.21635022080577));
#31320=CARTESIAN_POINT('Ctrl Pts',(105.62613218967,-1.03978503321322,7.23864125478473));
#31321=CARTESIAN_POINT('Ctrl Pts',(105.559961654856,1.57591511441003,7.14119689601862));
#31322=CARTESIAN_POINT('Ctrl Pts',(105.493791120042,3.54717258793725,5.97056873725912));
#31323=CARTESIAN_POINT('Ctrl Pts',(105.427620585228,5.51843006146448,4.79994057849962));
#31324=CARTESIAN_POINT('Ctrl Pts',(105.361450050414,6.84524486089555,2.55612861974682));
#31325=CARTESIAN_POINT('Ctrl Pts',(105.2952795156,6.93687390358686,0.257327369497228));
#31326=CARTESIAN_POINT('Ctrl Pts',(105.262194248193,6.98268842493251,-0.892073255627436));
#31327=CARTESIAN_POINT('Ctrl Pts',(105.229108980786,6.71970650709327,-2.05522120362623));
#31328=CARTESIAN_POINT('Ctrl Pts',(105.196023713379,6.20299267374967,-3.08870606767955));
#31329=CARTESIAN_POINT('Ctrl Pts',(105.162938445972,5.686278840406,-4.122190931733));
#31330=CARTESIAN_POINT('Ctrl Pts',(105.129853178565,4.91583309155763,-5.0260127118412));
#31331=CARTESIAN_POINT('Ctrl Pts',(105.096767911158,3.97388357095785,-5.68450421781766));
#31332=CARTESIAN_POINT('Ctrl Pts',(105.063682643751,3.03193405035818,-6.34299572379403));
#31333=CARTESIAN_POINT('Ctrl Pts',(105.030597376344,1.91848075800698,-6.75615695563902));
#31334=CARTESIAN_POINT('Ctrl Pts',(104.997512108937,0.770396244159204,-6.88648770729243));
#31335=CARTESIAN_POINT('Ctrl Pts',(104.96442684153,-0.377688269688576,-7.01681845894584));
#31336=CARTESIAN_POINT('Ctrl Pts',(104.931341574123,-1.56040400503286,-6.86431873040768));
#31337=CARTESIAN_POINT('Ctrl Pts',(104.898256306716,-2.62415213036371,-6.4265280307381));
#31338=CARTESIAN_POINT('Ctrl Pts',(104.832085771902,-4.75164838102565,-5.55094663139886));
#31339=CARTESIAN_POINT('Ctrl Pts',(104.765915237088,-6.40327419163353,-3.53420134753374));
#31340=CARTESIAN_POINT('Ctrl Pts',(104.699744702274,-6.82566286200369,-1.28080076989636));
#31341=CARTESIAN_POINT('Ctrl Pts',(104.687460356051,-6.90407795539624,-0.862464225520248));
#31342=CARTESIAN_POINT('Ctrl Pts',(104.675176009829,-6.94012772985068,-0.435971421728557));
#31343=CARTESIAN_POINT('Ctrl Pts',(104.662891663606,-6.93617806097948,-0.00865909541846954));
#31344=CARTESIAN_POINT('Ctrl Pts',(104.483548336394,-6.933,-4.16056078478277E-13));
#31345=CARTESIAN_POINT('Ctrl Pts',(104.540772531679,-6.93299999999988,-1.9942093570165));
#31346=CARTESIAN_POINT('Ctrl Pts',(104.597996726964,-6.02307502629244,-3.97063309653042));
#31347=CARTESIAN_POINT('Ctrl Pts',(104.655220922249,-4.50798484753998,-5.26731066241113));
#31348=CARTESIAN_POINT('Ctrl Pts',(104.712445117534,-2.99289466878752,-6.56398822829183));
#31349=CARTESIAN_POINT('Ctrl Pts',(104.769669312819,-0.899664345629392,
-7.15779044292397));
#31350=CARTESIAN_POINT('Ctrl Pts',(104.826893508104,1.07062371681769,-6.84983604599318));
#31351=CARTESIAN_POINT('Ctrl Pts',(104.884117703389,3.04091177926477,-6.54188164906239));
#31352=CARTESIAN_POINT('Ctrl Pts',(104.941341898675,4.85311303639787,-5.33766370386479));
#31353=CARTESIAN_POINT('Ctrl Pts',(104.99856609396,5.9002697149369,-3.6405090703085));
#31354=CARTESIAN_POINT('Ctrl Pts',(105.055790289245,6.94742639347593,-1.94335443675221));
#31355=CARTESIAN_POINT('Ctrl Pts',(105.11301448453,7.2108600852751,0.216464293122072));
#31356=CARTESIAN_POINT('Ctrl Pts',(105.170238679815,6.60233935006142,2.1155623617919));
#31357=CARTESIAN_POINT('Ctrl Pts',(105.2274628751,5.99381861484774,4.01466043046174));
#31358=CARTESIAN_POINT('Ctrl Pts',(105.284687070385,4.52419779647485,5.61916312790282));
#31359=CARTESIAN_POINT('Ctrl Pts',(105.34191126567,2.68569473000639,6.39167683923522));
#31360=CARTESIAN_POINT('Ctrl Pts',(105.399135460955,0.847191663537936,7.16419055056762));
#31361=CARTESIAN_POINT('Ctrl Pts',(105.45635965624,-1.32739978993864,7.09093574623839));
#31362=CARTESIAN_POINT('Ctrl Pts',(105.513583851525,-3.10974706735908,6.19644754492859));
#31363=CARTESIAN_POINT('Ctrl Pts',(105.57080804681,-4.89209434477952,5.3019593436188));
#31364=CARTESIAN_POINT('Ctrl Pts',(105.628032242096,-6.25040525058464,3.60219296582991));
#31365=CARTESIAN_POINT('Ctrl Pts',(105.685256437381,-6.72974280712672,1.66644854403793));
#31366=CARTESIAN_POINT('Ctrl Pts',(105.701353737052,-6.86458158035544,1.12191912096977));
#31367=CARTESIAN_POINT('Ctrl Pts',(105.717451036723,-6.93300000000002,0.560975745779151));
#31368=CARTESIAN_POINT('Ctrl Pts',(105.733548336394,-6.933,-2.66453525910038E-13));
#31369=CARTESIAN_POINT('Origin',(29.75,0.,0.));
#31370=CARTESIAN_POINT('',(107.162891663606,-6.92488577809423,0.00304253374609986));
#31371=CARTESIAN_POINT('',(106.983548336394,-6.9289346271905,0.00268695564041597));
#31372=CARTESIAN_POINT('',(29.75,-6.933,-8.4904762584886E-16));
#31373=CARTESIAN_POINT('Ctrl Pts',(107.162891663606,-6.92488577809423,0.00304253374609986));
#31374=CARTESIAN_POINT('Ctrl Pts',(107.135889094264,-6.92884091747773,0.947002408294073));
#31375=CARTESIAN_POINT('Ctrl Pts',(107.108886524921,-6.74871798472496,1.88952811505199));
#31376=CARTESIAN_POINT('Ctrl Pts',(107.081883955579,-6.377079692959,2.74976127902586));
#31377=CARTESIAN_POINT('Ctrl Pts',(107.015713420765,-5.46636989302528,4.85778617854933));
#31378=CARTESIAN_POINT('Ctrl Pts',(106.949542885951,-3.40559421461705,6.4716374201663));
#31379=CARTESIAN_POINT('Ctrl Pts',(106.883372351137,-1.1443604745777,6.84985187732506));
#31380=CARTESIAN_POINT('Ctrl Pts',(106.817201816323,1.11687326546152,7.2280663344838));
#31381=CARTESIAN_POINT('Ctrl Pts',(106.751031281509,3.57856506713182,6.37064400718454));
#31382=CARTESIAN_POINT('Ctrl Pts',(106.684860746695,5.1323120236005,4.67395393953337));
#31383=CARTESIAN_POINT('Ctrl Pts',(106.651775479288,5.90918550183488,3.82560890570773));
#31384=CARTESIAN_POINT('Ctrl Pts',(106.618690211881,6.45907276876884,2.76744693679409));
#31385=CARTESIAN_POINT('Ctrl Pts',(106.585604944474,6.7314677163284,1.64455469040912));
#31386=CARTESIAN_POINT('Ctrl Pts',(106.552519677067,7.00386266388793,0.521662444024272));
#31387=CARTESIAN_POINT('Ctrl Pts',(106.51943440966,6.99876529207313,-0.665960079831897));
#31388=CARTESIAN_POINT('Ctrl Pts',(106.486349142253,6.70432462161403,-1.77689798385835));
#31389=CARTESIAN_POINT('Ctrl Pts',(106.453263874846,6.4098839511549,-2.88783588788493));
#31390=CARTESIAN_POINT('Ctrl Pts',(106.420178607439,5.8260999820514,-3.92208917208177));
#31391=CARTESIAN_POINT('Ctrl Pts',(106.387093340031,5.03331171364945,-4.76266734495707));
#31392=CARTESIAN_POINT('Ctrl Pts',(106.354008072624,4.2405234452475,-5.60324551783236));
#31393=CARTESIAN_POINT('Ctrl Pts',(106.320922805217,3.2387308775471,-6.25014857938612));
#31394=CARTESIAN_POINT('Ctrl Pts',(106.28783753781,2.14366517559393,-6.60235830564033));
#31395=CARTESIAN_POINT('Ctrl Pts',(106.221667002996,-0.0464662283121736,
-7.30677775814868));
#31396=CARTESIAN_POINT('Ctrl Pts',(106.155496468182,-2.60969016922931,-6.83242386945914));
#31397=CARTESIAN_POINT('Ctrl Pts',(106.089325933368,-4.38676837012615,-5.38390087275648));
#31398=CARTESIAN_POINT('Ctrl Pts',(106.030514510114,-5.96621001318147,-4.09647438766379));
#31399=CARTESIAN_POINT('Ctrl Pts',(105.97170308686,-6.92464371329922,-2.03951278580644));
#31400=CARTESIAN_POINT('Ctrl Pts',(105.912891663606,-6.94073003849348,0.00450623896247018));
#31401=CARTESIAN_POINT('Ctrl Pts',(105.733548336394,-6.93549738005571,0.00309879224510982));
#31402=CARTESIAN_POINT('Ctrl Pts',(105.790990515821,-6.91749353528686,-1.99592298257485));
#31403=CARTESIAN_POINT('Ctrl Pts',(105.848432695249,-6.01582286335993,-4.00079412588348));
#31404=CARTESIAN_POINT('Ctrl Pts',(105.905874874676,-4.499576288691,-5.28998465377729));
#31405=CARTESIAN_POINT('Ctrl Pts',(105.97204540949,-2.75293561878853,-6.77506804647284));
#31406=CARTESIAN_POINT('Ctrl Pts',(106.038215944304,-0.190759207781901,
-7.31045081068274));
#31407=CARTESIAN_POINT('Ctrl Pts',(106.104386479118,2.00795219744992,-6.64803671598811));
#31408=CARTESIAN_POINT('Ctrl Pts',(106.170557013932,4.20666360268163,-5.98562262129351));
#31409=CARTESIAN_POINT('Ctrl Pts',(106.236727548746,6.04191000213856,-4.12541166769451));
#31410=CARTESIAN_POINT('Ctrl Pts',(106.30289808356,6.6745582169174,-1.91795138426491));
#31411=CARTESIAN_POINT('Ctrl Pts',(106.369068618374,7.30720643169628,0.289508899164824));
#31412=CARTESIAN_POINT('Ctrl Pts',(106.435239153188,6.73725646179693,2.8442185124252));
#31413=CARTESIAN_POINT('Ctrl Pts',(106.501409688002,5.22871076598718,4.57063552106892));
#31414=CARTESIAN_POINT('Ctrl Pts',(106.567580222817,3.72016507017752,6.29705252971253));
#31415=CARTESIAN_POINT('Ctrl Pts',(106.63375075763,1.27302364845756,7.19517693373959));
#31416=CARTESIAN_POINT('Ctrl Pts',(106.699921292445,-1.00430731665786,6.86860993177073));
#31417=CARTESIAN_POINT('Ctrl Pts',(106.733006559852,-2.14297279921577,6.70532643078627));
#31418=CARTESIAN_POINT('Ctrl Pts',(106.766091827259,-3.23918566762253,6.23587007830273));
#31419=CARTESIAN_POINT('Ctrl Pts',(106.799177094666,-4.16189215621188,5.54038633360014));
#31420=CARTESIAN_POINT('Ctrl Pts',(106.832262362073,-5.08459864480092,4.84490258889778));
#31421=CARTESIAN_POINT('Ctrl Pts',(106.86534762948,-5.83379875357268,3.92339145197653));
#31422=CARTESIAN_POINT('Ctrl Pts',(106.898432896887,-6.31064547973526,2.87768808353459));
#31423=CARTESIAN_POINT('Ctrl Pts',(106.926804710056,-6.7195587902587,1.98095963232713));
#31424=CARTESIAN_POINT('Ctrl Pts',(106.955176523225,-6.92819206609309,0.992904155184515));
#31425=CARTESIAN_POINT('Ctrl Pts',(106.983548336394,-6.9289346271905,0.00268695564041597));
#31426=CARTESIAN_POINT('Origin',(29.75,0.,0.));
#31427=CARTESIAN_POINT('',(108.412891663606,-6.92776634541837,-0.00844704756396031));
#31428=CARTESIAN_POINT('',(108.233548336394,-6.93028901950621,-0.00380765172104063));
#31429=CARTESIAN_POINT('',(29.75,-6.933,-8.4904762584886E-16));
#31430=CARTESIAN_POINT('Ctrl Pts',(108.412891663606,-6.92776634541837,-0.00844704756396031));
#31431=CARTESIAN_POINT('Ctrl Pts',(108.366245636481,-6.91355352143459,1.621272426568));
#31432=CARTESIAN_POINT('Ctrl Pts',(108.319599609356,-6.3407349699669,3.26180305496299));
#31433=CARTESIAN_POINT('Ctrl Pts',(108.272953582232,-5.29536157004919,4.49505663430979));
#31434=CARTESIAN_POINT('Ctrl Pts',(108.206783047418,-3.81242891283097,6.24450999479188));
#31435=CARTESIAN_POINT('Ctrl Pts',(108.140612512604,-1.37855827834812,7.17438608402479));
#31436=CARTESIAN_POINT('Ctrl Pts',(108.074441977789,0.903318468414054,6.88158564177937));
#31437=CARTESIAN_POINT('Ctrl Pts',(108.041356710382,2.04425684179514,6.73518542065666));
#31438=CARTESIAN_POINT('Ctrl Pts',(108.008271442975,3.14719674324603,6.28311606666432));
#31439=CARTESIAN_POINT('Ctrl Pts',(107.975186175568,4.08001313168627,5.60148092342676));
#31440=CARTESIAN_POINT('Ctrl Pts',(107.942100908161,5.0128295201265,4.9198457801892));
#31441=CARTESIAN_POINT('Ctrl Pts',(107.909015640754,5.77552239555616,4.00864484770638));
#31442=CARTESIAN_POINT('Ctrl Pts',(107.875930373347,6.26769096176187,2.96986524175247));
#31443=CARTESIAN_POINT('Ctrl Pts',(107.84284510594,6.75985952796753,1.93108563579867));
#31444=CARTESIAN_POINT('Ctrl Pts',(107.809759838533,6.98150378494936,0.764727356373722));
#31445=CARTESIAN_POINT('Ctrl Pts',(107.776674571126,6.9185152599161,-0.388891218753205));
#31446=CARTESIAN_POINT('Ctrl Pts',(107.743589303719,6.85552673488282,-1.5425097938804));
#31447=CARTESIAN_POINT('Ctrl Pts',(107.710504036312,6.50790542783433,-2.68338866470967));
#31448=CARTESIAN_POINT('Ctrl Pts',(107.677418768905,5.89882838853818,-3.65929881778214));
#31449=CARTESIAN_POINT('Ctrl Pts',(107.611248234091,4.68067430994609,-5.61111912392676));
#31450=CARTESIAN_POINT('Ctrl Pts',(107.545077699277,2.41669730236367,-6.90306455904472));
#31451=CARTESIAN_POINT('Ctrl Pts',(107.478907164463,0.124409193473775,-6.94364573346948));
#31452=CARTESIAN_POINT('Ctrl Pts',(107.412736629649,-2.16787891541625,-6.98422690789425));
#31453=CARTESIAN_POINT('Ctrl Pts',(107.346566094835,-4.48847812561356,-5.77344382162591));
#31454=CARTESIAN_POINT('Ctrl Pts',(107.280395560021,-5.76845576998274,-3.86695299977675));
#31455=CARTESIAN_POINT('Ctrl Pts',(107.241227594549,-6.5261059887696,-2.73845423681513));
#31456=CARTESIAN_POINT('Ctrl Pts',(107.202059629078,-6.91914874022781,-1.36619708578935));
#31457=CARTESIAN_POINT('Ctrl Pts',(107.162891663606,-6.92488577809423,0.00304253374609986));
#31458=CARTESIAN_POINT('Ctrl Pts',(106.983548336394,-6.9289346271905,0.00268695564041597));
#31459=CARTESIAN_POINT('Ctrl Pts',(106.988261790632,-6.92905799004118,-0.161819395360096));
#31460=CARTESIAN_POINT('Ctrl Pts',(106.99297524487,-6.92344363092686,-0.326385409256667));
#31461=CARTESIAN_POINT('Ctrl Pts',(106.997688699108,-6.91205665349178,-0.490602246874311));
#31462=CARTESIAN_POINT('Ctrl Pts',(107.030773966515,-6.83212775753224,-1.64329360887824));
#31463=CARTESIAN_POINT('Ctrl Pts',(107.063859233922,-6.46777662205971,-2.77878073292303));
#31464=CARTESIAN_POINT('Ctrl Pts',(107.096944501329,-5.8444237086234,-3.74555518589093));
#31465=CARTESIAN_POINT('Ctrl Pts',(107.163115036143,-4.59771788175101,-5.6791040918264));
#31466=CARTESIAN_POINT('Ctrl Pts',(107.229285570957,-2.31500494302391,-6.93780231345459));
#31467=CARTESIAN_POINT('Ctrl Pts',(107.295456105771,-0.0223697880795398,
-6.94474846410226));
#31468=CARTESIAN_POINT('Ctrl Pts',(107.361626640585,2.27026536686496,-6.95169461474993));
#31469=CARTESIAN_POINT('Ctrl Pts',(107.427797175399,4.57282273802673,-5.70688869441693));
#31470=CARTESIAN_POINT('Ctrl Pts',(107.493967710213,5.82465096202989,-3.78176859055449));
#31471=CARTESIAN_POINT('Ctrl Pts',(107.560138245027,7.07647918603296,-1.85664848669215));
#31472=CARTESIAN_POINT('Ctrl Pts',(107.626308779841,7.27757826287754,0.748785800699566));
#31473=CARTESIAN_POINT('Ctrl Pts',(107.692479314655,6.3359900190534,2.84317392207816));
#31474=CARTESIAN_POINT('Ctrl Pts',(107.758649849469,5.3944017752292,4.93756204345687));
#31475=CARTESIAN_POINT('Ctrl Pts',(107.824820384283,3.31012621073615,6.5209039988224));
#31476=CARTESIAN_POINT('Ctrl Pts',(107.890990919097,1.04358538120297,6.86590294655329));
#31477=CARTESIAN_POINT('Ctrl Pts',(107.957161453911,-1.22295544833022,7.21090189428418));
#31478=CARTESIAN_POINT('Ctrl Pts',(108.023331988725,-3.67176154290354,6.31755783438044));
#31479=CARTESIAN_POINT('Ctrl Pts',(108.089502523539,-5.20043113550107,4.59806048243787));
#31480=CARTESIAN_POINT('Ctrl Pts',(108.122587790946,-5.96476593179974,3.73831180646669));
#31481=CARTESIAN_POINT('Ctrl Pts',(108.155673058353,-6.49906660260453,2.67202480748586));
#31482=CARTESIAN_POINT('Ctrl Pts',(108.18875832576,-6.75491755697916,1.54537328180927));
#31483=CARTESIAN_POINT('Ctrl Pts',(108.203688329305,-6.87037243931928,1.03696236087581));
#31484=CARTESIAN_POINT('Ctrl Pts',(108.218618332849,-6.92912546191901,0.516259163369478));
#31485=CARTESIAN_POINT('Ctrl Pts',(108.233548336394,-6.93028901950621,-0.00380765172104063));
#31486=CARTESIAN_POINT('Origin',(-87.75,0.,0.));
#31487=CARTESIAN_POINT('',(-86.1648283363937,-6.93261614350334,-0.000140194423062512));
#31488=CARTESIAN_POINT('',(-86.3441716636063,-6.93270425418277,-0.000130097846330653));
#31489=CARTESIAN_POINT('',(-87.75,-6.933,-8.4904762584886E-16));
#31490=CARTESIAN_POINT('',(-86.51072,1.15840596835136,6.8358145694558));
#31491=CARTESIAN_POINT('Ctrl Pts',(-86.1648283363937,-6.93261614350334,
-0.000140194423062512));
#31492=CARTESIAN_POINT('Ctrl Pts',(-86.1862819769683,-6.93206966311315,
0.747603057917331));
#31493=CARTESIAN_POINT('Ctrl Pts',(-86.2077356175428,-6.81152017995217,
1.49551828662709));
#31494=CARTESIAN_POINT('Ctrl Pts',(-86.2291892581174,-6.57390952823857,
2.20418517192447));
#31495=CARTESIAN_POINT('Ctrl Pts',(-86.2622185198563,-6.20809262270579,
3.2952234951791));
#31496=CARTESIAN_POINT('Ctrl Pts',(-86.2952477815952,-5.56481047477723,
4.29323309462037));
#31497=CARTESIAN_POINT('Ctrl Pts',(-86.3282770433341,-4.72221552560607,
5.07695161393405));
#31498=CARTESIAN_POINT('Ctrl Pts',(-86.361306305073,-3.87962057643491,5.86067013324773));
#31499=CARTESIAN_POINT('Ctrl Pts',(-86.3943355668118,-2.83771282602114,
6.43009757243381));
#31500=CARTESIAN_POINT('Ctrl Pts',(-86.4273648285507,-1.72308180962127,
6.71607370144116));
#31501=CARTESIAN_POINT('Ctrl Pts',(-86.4551498857004,-0.785425777936701,
6.95664411293718));
#31502=CARTESIAN_POINT('Ctrl Pts',(-86.4829349428502,0.2036936247524,6.99662727440187));
#31503=CARTESIAN_POINT('Ctrl Pts',(-86.51072,1.15840596835136,6.8358145694558));
#31504=CARTESIAN_POINT('',(-86.51072,-6.933,-8.4904762584886E-16));
#31505=CARTESIAN_POINT('Origin',(-86.51072,0.,0.));
#31506=CARTESIAN_POINT('',(-109.067,-6.933,-8.4904762584886E-16));
#31507=CARTESIAN_POINT('',(-87.75,-6.933,-8.4904762584886E-16));
#31508=CARTESIAN_POINT('Origin',(-109.067,0.,0.));
#31509=CARTESIAN_POINT('',(-86.51072,-4.64214617842358,5.1494628708388));
#31510=CARTESIAN_POINT('Origin',(-86.51072,0.,0.));
#31511=CARTESIAN_POINT('Ctrl Pts',(-86.51072,-4.64214617842358,5.14946287083879));
#31512=CARTESIAN_POINT('Ctrl Pts',(-86.4776907382611,-5.49707636744032,
4.37875901117264));
#31513=CARTESIAN_POINT('Ctrl Pts',(-86.4446614765222,-6.15592316322177,
3.39140242300292));
#31514=CARTESIAN_POINT('Ctrl Pts',(-86.4116322147833,-6.53873675821753,
2.30636006071919));
#31515=CARTESIAN_POINT('Ctrl Pts',(-86.389145364391,-6.79936238487788,1.56764584231125));
#31516=CARTESIAN_POINT('Ctrl Pts',(-86.3666585139986,-6.93204373903408,
0.783653246999931));
#31517=CARTESIAN_POINT('Ctrl Pts',(-86.3441716636063,-6.93270425418277,
-0.000130097846330653));
#31518=CARTESIAN_POINT('Origin',(-87.75,0.,0.));
#31519=CARTESIAN_POINT('',(-84.9148283363937,-6.93288145074965,0.000176808201168416));
#31520=CARTESIAN_POINT('',(-85.0941716636063,-6.9327762777167,0.000168448225849813));
#31521=CARTESIAN_POINT('',(-87.75,-6.933,-8.4904762584886E-16));
#31522=CARTESIAN_POINT('Ctrl Pts',(-84.9148283363937,-6.93288145074965,
0.000176808201168416));
#31523=CARTESIAN_POINT('Ctrl Pts',(-84.9235682410294,-6.93318021234269,
0.304763539330887));
#31524=CARTESIAN_POINT('Ctrl Pts',(-84.932308145665,-6.91347845811148,0.609311906094795));
#31525=CARTESIAN_POINT('Ctrl Pts',(-84.9410480503007,-6.87346355102493,
0.911167498725949));
#31526=CARTESIAN_POINT('Ctrl Pts',(-84.9740773120396,-6.72224189647419,
2.05191992017604));
#31527=CARTESIAN_POINT('Ctrl Pts',(-85.0071065737784,-6.28091092139654,
3.15421455619275));
#31528=CARTESIAN_POINT('Ctrl Pts',(-85.0401358355174,-5.60308949675388,
4.08412970976292));
#31529=CARTESIAN_POINT('Ctrl Pts',(-85.0731650972563,-4.92526807211124,
5.01404486333308));
#31530=CARTESIAN_POINT('Ctrl Pts',(-85.1061943589952,-4.01095619790362,
5.77158053445669));
#31531=CARTESIAN_POINT('Ctrl Pts',(-85.1392236207341,-2.97123687706053,
6.26470101639398));
#31532=CARTESIAN_POINT('Ctrl Pts',(-85.1722528824729,-1.93151755621743,
6.75782149833127));
#31533=CARTESIAN_POINT('Ctrl Pts',(-85.2052821442118,-0.766390788738866,
6.98652679108223));
#31534=CARTESIAN_POINT('Ctrl Pts',(-85.2383114059506,0.382588027107184,
6.92303067917854));
#31535=CARTESIAN_POINT('Ctrl Pts',(-85.2713406676895,1.53156684295325,6.85953456727484));
#31536=CARTESIAN_POINT('Ctrl Pts',(-85.3043699294285,2.6643977071668,6.50383705071648));
#31537=CARTESIAN_POINT('Ctrl Pts',(-85.3373991911674,3.64344896848527,5.8991530776003));
#31538=CARTESIAN_POINT('Ctrl Pts',(-85.3704284529063,4.62250022980373,5.29446910448412));
#31539=CARTESIAN_POINT('Ctrl Pts',(-85.4034577146451,5.44777188822712,4.44079867481011));
#31540=CARTESIAN_POINT('Ctrl Pts',(-85.436486976384,6.01899874927411,3.4418572653518));
#31541=CARTESIAN_POINT('Ctrl Pts',(-85.4695162381229,6.5902256103211,2.44291585589349));
#31542=CARTESIAN_POINT('Ctrl Pts',(-85.5025454998618,6.90740767399169,1.29870346665087));
#31543=CARTESIAN_POINT('Ctrl Pts',(-85.5355747616007,6.9320093702799,0.148234495631678));
#31544=CARTESIAN_POINT('Ctrl Pts',(-85.5686040233396,6.95661106656811,-1.0022344753875));
#31545=CARTESIAN_POINT('Ctrl Pts',(-85.6016332850785,6.68863239547394,-2.15896002818325));
#31546=CARTESIAN_POINT('Ctrl Pts',(-85.6346625468174,6.1606310238489,-3.18140738363518));
#31547=CARTESIAN_POINT('Ctrl Pts',(-85.6676918085563,5.63262965222386,-4.20385473908712));
#31548=CARTESIAN_POINT('Ctrl Pts',(-85.7007210702952,4.84460558006794,-5.09202389719524));
#31549=CARTESIAN_POINT('Ctrl Pts',(-85.7337503320341,3.89229868783116,-5.73800817878655));
#31550=CARTESIAN_POINT('Ctrl Pts',(-85.766779593773,2.93999179559439,-6.38399246037785));
#31551=CARTESIAN_POINT('Ctrl Pts',(-85.7998088555118,1.82340208327677,-6.78779186545236));
#31552=CARTESIAN_POINT('Ctrl Pts',(-85.8328381172507,0.678187944654679,
-6.90034705779794));
#31553=CARTESIAN_POINT('Ctrl Pts',(-85.8658673789896,-0.467026193967406,
-7.01290225014353));
#31554=CARTESIAN_POINT('Ctrl Pts',(-85.8988966407285,-1.64086475889396,
-6.83421322976019));
#31555=CARTESIAN_POINT('Ctrl Pts',(-85.9319259024674,-2.70071379568421,
-6.38599018928669));
#31556=CARTESIAN_POINT('Ctrl Pts',(-85.9649551642063,-3.76056283247446,
-5.93776714881318));
#31557=CARTESIAN_POINT('Ctrl Pts',(-85.9979844259452,-4.70642234112842,
-5.22001008824951));
#31558=CARTESIAN_POINT('Ctrl Pts',(-86.0310136876841,-5.4233767471659,-4.31992059426439));
#31559=CARTESIAN_POINT('Ctrl Pts',(-86.0640429494229,-6.14033115320338,
-3.41983110027927));
#31560=CARTESIAN_POINT('Ctrl Pts',(-86.0970722111618,-6.62838045662438,
-2.33740917287272));
#31561=CARTESIAN_POINT('Ctrl Pts',(-86.1301014729007,-6.82822927676637,
-1.20416468563544));
#31562=CARTESIAN_POINT('Ctrl Pts',(-86.141677094065,-6.89826942027279,-0.807001437648487));
#31563=CARTESIAN_POINT('Ctrl Pts',(-86.1532527152294,-6.9329110048789,-0.403595849755758));
#31564=CARTESIAN_POINT('Ctrl Pts',(-86.1648283363937,-6.93261614350334,
-0.000140194423062512));
#31565=CARTESIAN_POINT('Ctrl Pts',(-86.3441716636063,-6.93270425418277,
-0.000130097846330653));
#31566=CARTESIAN_POINT('Ctrl Pts',(-86.3336292522597,-6.93301392060011,
-0.367587802405469));
#31567=CARTESIAN_POINT('Ctrl Pts',(-86.3230868409132,-6.90430574294555,
-0.734999514245483));
#31568=CARTESIAN_POINT('Ctrl Pts',(-86.3125444295667,-6.84615964459705,
-1.09767788462958));
#31569=CARTESIAN_POINT('Ctrl Pts',(-86.2795151678278,-6.66398854177075,
-2.23394533129684));
#31570=CARTESIAN_POINT('Ctrl Pts',(-86.2464859060889,-6.19286594190809,
-3.32375208823362));
#31571=CARTESIAN_POINT('Ctrl Pts',(-86.21345664435,-5.49002272730517,-4.23488005538391));
#31572=CARTESIAN_POINT('Ctrl Pts',(-86.1804273826111,-4.78717951270224,
-5.1460080225342));
#31573=CARTESIAN_POINT('Ctrl Pts',(-86.1473981208722,-3.85261568335905,
-5.878457199898));
#31574=CARTESIAN_POINT('Ctrl Pts',(-86.1143688591333,-2.79987809561172,
-6.34314896472182));
#31575=CARTESIAN_POINT('Ctrl Pts',(-86.0813395973944,-1.7471405078644,-6.80784072954562));
#31576=CARTESIAN_POINT('Ctrl Pts',(-86.0483103356556,-0.576229161712943,
-7.00477508182944));
#31577=CARTESIAN_POINT('Ctrl Pts',(-86.0152810739167,0.570599361365794,
-6.91007040330406));
#31578=CARTESIAN_POINT('Ctrl Pts',(-85.9822518121778,1.71742788444454,-6.81536572477869));
#31579=CARTESIAN_POINT('Ctrl Pts',(-85.9492225504389,2.84017358445056,-6.42902201544412));
#31580=CARTESIAN_POINT('Ctrl Pts',(-85.9161932887,3.80242930172544,-5.7979555409898));
#31581=CARTESIAN_POINT('Ctrl Pts',(-85.8831640269611,4.76468501900033,-5.16688906653548));
#31582=CARTESIAN_POINT('Ctrl Pts',(-85.8501347652222,5.56645075354407,-4.29109982696142));
#31583=CARTESIAN_POINT('Ctrl Pts',(-85.8171055034833,6.11031752189778,-3.27700142574845));
#31584=CARTESIAN_POINT('Ctrl Pts',(-85.7840762417444,6.65418429025149,-2.26290302453548));
#31585=CARTESIAN_POINT('Ctrl Pts',(-85.7510469800056,6.94015209241517,-1.11049546168359));
#31586=CARTESIAN_POINT('Ctrl Pts',(-85.7180177182666,6.93347749064973,0.0402165186038079));
#31587=CARTESIAN_POINT('Ctrl Pts',(-85.6849884565277,6.92680288888429,1.19092849889121));
#31588=CARTESIAN_POINT('Ctrl Pts',(-85.6519591947888,6.62748588318974,2.33994489661413));
#31589=CARTESIAN_POINT('Ctrl Pts',(-85.6189299330499,6.07189165634794,3.34766498136383));
#31590=CARTESIAN_POINT('Ctrl Pts',(-85.5859006713111,5.51629742950615,4.35538506611354));
#31591=CARTESIAN_POINT('Ctrl Pts',(-85.5528714095722,4.70442598151711,5.22180883789003));
#31592=CARTESIAN_POINT('Ctrl Pts',(-85.5198421478333,3.73491441718631,5.84167269083401));
#31593=CARTESIAN_POINT('Ctrl Pts',(-85.4868128860944,2.76540285285553,6.46153654377797));
#31594=CARTESIAN_POINT('Ctrl Pts',(-85.4537836243555,1.63825117218298,6.83484047788943));
#31595=CARTESIAN_POINT('Ctrl Pts',(-85.4207543626166,0.490401067077939,
6.9162298278678));
#31596=CARTESIAN_POINT('Ctrl Pts',(-85.3877251008777,-0.65744903802711,
6.99761917784616));
#31597=CARTESIAN_POINT('Ctrl Pts',(-85.3546958391389,-1.82599756756465,
6.78709394369144));
#31598=CARTESIAN_POINT('Ctrl Pts',(-85.3216665774,-2.87327341347956,6.31023190183795));
#31599=CARTESIAN_POINT('Ctrl Pts',(-85.2886373156611,-3.92054925939447,
5.83336985998445));
#31600=CARTESIAN_POINT('Ctrl Pts',(-85.2556080539222,-4.84655242168673,
5.09017101043218));
#31601=CARTESIAN_POINT('Ctrl Pts',(-85.2225787921833,-5.53877947518409,
4.17092907015388));
#31602=CARTESIAN_POINT('Ctrl Pts',(-85.1895495304444,-6.23100652868145,
3.2516871298756));
#31603=CARTESIAN_POINT('Ctrl Pts',(-85.1565202687055,-6.68945747338392,
2.15640209887129));
#31604=CARTESIAN_POINT('Ctrl Pts',(-85.1234910069666,-6.85843347527675,
1.01814413035879));
#31605=CARTESIAN_POINT('Ctrl Pts',(-85.1137178925132,-6.90843222545892,
0.681342009507277));
#31606=CARTESIAN_POINT('Ctrl Pts',(-85.1039447780597,-6.93308673909412,
0.340777503273612));
#31607=CARTESIAN_POINT('Ctrl Pts',(-85.0941716636063,-6.9327762777167,0.000168448225849813));
#31608=CARTESIAN_POINT('Origin',(-87.75,0.,0.));
#31609=CARTESIAN_POINT('',(-83.6648283363937,-6.93338479581795,-0.000128863436223425));
#31610=CARTESIAN_POINT('',(-83.8441716636063,-6.93347143000264,-0.000100837253274565));
#31611=CARTESIAN_POINT('',(-87.75,-6.933,-8.4904762584886E-16));
#31612=CARTESIAN_POINT('Ctrl Pts',(-83.6648283363937,-6.93338479581795,
-0.000128863436223425));
#31613=CARTESIAN_POINT('Ctrl Pts',(-83.6938837668294,-6.93251907425441,
1.01224445621453));
#31614=CARTESIAN_POINT('Ctrl Pts',(-83.722939197265,-6.70811950439672,2.02498894125545));
#31615=CARTESIAN_POINT('Ctrl Pts',(-83.7519946277007,-6.27864669710701,
2.94165311522865));
#31616=CARTESIAN_POINT('Ctrl Pts',(-83.7850238894395,-5.79043607523614,
3.98368692697662));
#31617=CARTESIAN_POINT('Ctrl Pts',(-83.8180531511784,-5.03722165824491,
4.90156193873623));
#31618=CARTESIAN_POINT('Ctrl Pts',(-83.8510824129173,-4.11051414613749,
5.5837622488632));
#31619=CARTESIAN_POINT('Ctrl Pts',(-83.8841116746562,-3.18380663403007,
6.26596255899017));
#31620=CARTESIAN_POINT('Ctrl Pts',(-83.9171409363951,-2.08360602680646,
6.7124881674845));
#31621=CARTESIAN_POINT('Ctrl Pts',(-83.950170198134,-0.943579611550886,
6.86908908910737));
#31622=CARTESIAN_POINT('Ctrl Pts',(-83.9831994598728,0.196446803704693,
7.02569001073024));
#31623=CARTESIAN_POINT('Ctrl Pts',(-84.0162287216118,1.37629902699225,6.89236624548166));
#31624=CARTESIAN_POINT('Ctrl Pts',(-84.0492579833507,2.45263261293338,6.48531577206538));
#31625=CARTESIAN_POINT('Ctrl Pts',(-84.0822872450896,3.52896619887452,6.07826529864909));
#31626=CARTESIAN_POINT('Ctrl Pts',(-84.1153165068284,4.50178114746923,5.3974881170651));
#31627=CARTESIAN_POINT('Ctrl Pts',(-84.1483457685673,5.25288670863111,4.52569426980176));
#31628=CARTESIAN_POINT('Ctrl Pts',(-84.1813750303062,6.00399226979299,3.65390042253842));
#31629=CARTESIAN_POINT('Ctrl Pts',(-84.2144042920451,6.53338844352204,2.59108990959573));
#31630=CARTESIAN_POINT('Ctrl Pts',(-84.247433553784,6.7767570046951,1.46638736244647));
#31631=CARTESIAN_POINT('Ctrl Pts',(-84.2804628155229,7.02012556586816,0.34168481529722));
#31632=CARTESIAN_POINT('Ctrl Pts',(-84.3134920772618,6.97746651448524,-0.844909766058596));
#31633=CARTESIAN_POINT('Ctrl Pts',(-84.3465213390007,6.65396265051231,-1.94923278317452));
#31634=CARTESIAN_POINT('Ctrl Pts',(-84.3795506007396,6.33045878653939,-3.05355580029043));
#31635=CARTESIAN_POINT('Ctrl Pts',(-84.4125798624785,5.72611010997647,-4.07560725316645));
#31636=CARTESIAN_POINT('Ctrl Pts',(-84.4456091242173,4.91434109224742,-4.89121447357585));
#31637=CARTESIAN_POINT('Ctrl Pts',(-84.4786383859562,4.10257207451836,-5.70682169398526));
#31638=CARTESIAN_POINT('Ctrl Pts',(-84.5116676476951,3.08338271562318,-6.31598468192806));
#31639=CARTESIAN_POINT('Ctrl Pts',(-84.544696909434,1.98059795779642,-6.64469405818632));
#31640=CARTESIAN_POINT('Ctrl Pts',(-84.5777261711729,0.877813199969654,
-6.97340343444458));
#31641=CARTESIAN_POINT('Ctrl Pts',(-84.6107554329119,-0.308566956788687,
-7.02165919901831));
#31642=CARTESIAN_POINT('Ctrl Pts',(-84.6437846946507,-1.43440496524513,
-6.78359858727645));
#31643=CARTESIAN_POINT('Ctrl Pts',(-84.6768139563896,-2.56024297370157,
-6.5455379755346));
#31644=CARTESIAN_POINT('Ctrl Pts',(-84.7098432181284,-3.62553883385612,
-6.02116098747716));
#31645=CARTESIAN_POINT('Ctrl Pts',(-84.7428724798673,-4.5008659605355,-5.274176049627));
#31646=CARTESIAN_POINT('Ctrl Pts',(-84.7759017416062,-5.37619308721488,
-4.52719111177684));
#31647=CARTESIAN_POINT('Ctrl Pts',(-84.8089310033451,-6.0615514804191,-3.55759822413396));
#31648=CARTESIAN_POINT('Ctrl Pts',(-84.841960265084,-6.4736745100093,-2.48319667687079));
#31649=CARTESIAN_POINT('Ctrl Pts',(-84.8662496221873,-6.77674526936564,
-1.69309355376585));
#31650=CARTESIAN_POINT('Ctrl Pts',(-84.8905389792905,-6.93205115255709,
-0.846310217657153));
#31651=CARTESIAN_POINT('Ctrl Pts',(-84.9148283363937,-6.93288145074965,
0.000176808201168416));
#31652=CARTESIAN_POINT('Ctrl Pts',(-85.0941716636063,-6.9327762777167,0.000168448225849813));
#31653=CARTESIAN_POINT('Ctrl Pts',(-85.0709155163209,-6.93203750242105,
-0.810346397239332));
#31654=CARTESIAN_POINT('Ctrl Pts',(-85.0476593690354,-6.78993411546133,
-1.62111350115066));
#31655=CARTESIAN_POINT('Ctrl Pts',(-85.02440322175,-6.51157649632067,-2.38203667921726));
#31656=CARTESIAN_POINT('Ctrl Pts',(-84.9913739600111,-6.11624245638856,
-3.46272861426011));
#31657=CARTESIAN_POINT('Ctrl Pts',(-84.9583446982721,-5.44607331744114,
-4.44288157832512));
#31658=CARTESIAN_POINT('Ctrl Pts',(-84.9253154365332,-4.58249031378848,
-5.20341328099003));
#31659=CARTESIAN_POINT('Ctrl Pts',(-84.8922861747943,-3.71890731013583,
-5.96394498365495));
#31660=CARTESIAN_POINT('Ctrl Pts',(-84.8592569130555,-2.66191044177793,
-6.50485542491976));
#31661=CARTESIAN_POINT('Ctrl Pts',(-84.8262276513166,-1.53991801948317,
-6.76042747955588));
#31662=CARTESIAN_POINT('Ctrl Pts',(-84.7931983895778,-0.417925597188426,
-7.01599953419199));
#31663=CARTESIAN_POINT('Ctrl Pts',(-84.7601691278388,0.769062379043175,
-6.98623320219942));
#31664=CARTESIAN_POINT('Ctrl Pts',(-84.7271398660999,1.87683451565091,-6.67474489662896));
#31665=CARTESIAN_POINT('Ctrl Pts',(-84.694110604361,2.98460665225864,-6.3632565910585));
#31666=CARTESIAN_POINT('Ctrl Pts',(-84.6610813426221,4.01316294924251,-5.77004631191016));
#31667=CARTESIAN_POINT('Ctrl Pts',(-84.6280520808833,4.83754044181217,-4.96718528931603));
#31668=CARTESIAN_POINT('Ctrl Pts',(-84.5950228191444,5.66191793438184,-4.16432426672191));
#31669=CARTESIAN_POINT('Ctrl Pts',(-84.5619935574055,6.28211662253732,-3.15181250068199));
#31670=CARTESIAN_POINT('Ctrl Pts',(-84.5289642956666,6.62278636049758,-2.05266364779728));
#31671=CARTESIAN_POINT('Ctrl Pts',(-84.4959350339277,6.96345609845784,-0.953514794912575));
#31672=CARTESIAN_POINT('Ctrl Pts',(-84.4629057721888,7.0245968862229,0.232271144816923));
#31673=CARTESIAN_POINT('Ctrl Pts',(-84.4298765104499,6.79878051192343,1.36062881713992));
#31674=CARTESIAN_POINT('Ctrl Pts',(-84.396847248711,6.57296413762396,2.48898648946292));
#31675=CARTESIAN_POINT('Ctrl Pts',(-84.3638179869722,6.06019060125995,3.55991589437942));
#31676=CARTESIAN_POINT('Ctrl Pts',(-84.3307887252333,5.32275858457524,4.4433060076109));
#31677=CARTESIAN_POINT('Ctrl Pts',(-84.2977594634944,4.58532656789052,5.32669612084239));
#31678=CARTESIAN_POINT('Ctrl Pts',(-84.2647302017554,3.62323607088509,6.02254694238886));
#31679=CARTESIAN_POINT('Ctrl Pts',(-84.2317009400166,2.55337489186155,6.44631707946529));
#31680=CARTESIAN_POINT('Ctrl Pts',(-84.1986716782776,1.48351371283801,6.87008721654171));
#31681=CARTESIAN_POINT('Ctrl Pts',(-84.1656424165388,0.305881851796347,
7.02177666914809));
#31682=CARTESIAN_POINT('Ctrl Pts',(-84.1326131547999,-0.836446005598494,
6.88295614593155));
#31683=CARTESIAN_POINT('Ctrl Pts',(-84.099583893061,-1.97877386299333,6.74413562271501));
#31684=CARTESIAN_POINT('Ctrl Pts',(-84.0665546313221,-3.08579771674133,
6.31480512367556));
#31685=CARTESIAN_POINT('Ctrl Pts',(-84.0335253695832,-4.02302129925474,
5.64712553897888));
#31686=CARTESIAN_POINT('Ctrl Pts',(-84.0004961078443,-4.96024488176816,
4.97944595428219));
#31687=CARTESIAN_POINT('Ctrl Pts',(-83.9674668461054,-5.72766819304699,
4.07341728392825));
#31688=CARTESIAN_POINT('Ctrl Pts',(-83.9344375843665,-6.23205424395508,
3.03911617540227));
#31689=CARTESIAN_POINT('Ctrl Pts',(-83.9043489441131,-6.69153440293035,
2.09689971854705));
#31690=CARTESIAN_POINT('Ctrl Pts',(-83.8742603038597,-6.93272917490753,
1.04823446896903));
#31691=CARTESIAN_POINT('Ctrl Pts',(-83.8441716636063,-6.93347143000264,
-0.000100837253274565));
#31692=CARTESIAN_POINT('Origin',(-87.75,0.,0.));
#31693=CARTESIAN_POINT('',(-82.4148283363938,-6.93241284950548,5.58784473136953E-6));
#31694=CARTESIAN_POINT('',(-82.5941716636063,-6.93241904285695,-2.76930968138527E-5));
#31695=CARTESIAN_POINT('',(-87.75,-6.933,-8.4904762584886E-16));
#31696=CARTESIAN_POINT('Ctrl Pts',(-82.4148283363938,-6.93241284950548,
5.58784473136953E-6));
#31697=CARTESIAN_POINT('Ctrl Pts',(-82.4311700308905,-6.93242887600529,
0.569625986647833));
#31698=CARTESIAN_POINT('Ctrl Pts',(-82.4475117253872,-6.86301704074712,
1.1392425477305));
#31699=CARTESIAN_POINT('Ctrl Pts',(-82.4638534198839,-6.72413178121344,
1.69138380809983));
#31700=CARTESIAN_POINT('Ctrl Pts',(-82.4968826816228,-6.44342174898704,
2.80735242501566));
#31701=CARTESIAN_POINT('Ctrl Pts',(-82.5299119433617,-5.87890526500855,
3.85193254855472));
#31702=CARTESIAN_POINT('Ctrl Pts',(-82.5629412051006,-5.09916744587612,
4.6982144221336));
#31703=CARTESIAN_POINT('Ctrl Pts',(-82.5959704668395,-4.31942962674368,
5.54449629571249));
#31704=CARTESIAN_POINT('Ctrl Pts',(-82.6289997285784,-3.32447047245728,
6.1924799193312));
#31705=CARTESIAN_POINT('Ctrl Pts',(-82.6620289903173,-2.23517111145839,
6.56343945656001));
#31706=CARTESIAN_POINT('Ctrl Pts',(-82.6950582520562,-1.14587175045949,
6.93439899378882));
#31707=CARTESIAN_POINT('Ctrl Pts',(-82.728087513795,0.0377678172519116,
7.02833444462773));
#31708=CARTESIAN_POINT('Ctrl Pts',(-82.7611167755339,1.17194300834543,6.83383325686376));
#31709=CARTESIAN_POINT('Ctrl Pts',(-82.7941460372728,2.30611819943894,6.6393320690998));
#31710=CARTESIAN_POINT('Ctrl Pts',(-82.8271752990117,3.39082901391457,6.15639424273297));
#31711=CARTESIAN_POINT('Ctrl Pts',(-82.8602045607506,4.2942900747329,5.44369361293207));
#31712=CARTESIAN_POINT('Ctrl Pts',(-82.8932338224895,5.19775113555124,4.73099298313117));
#31713=CARTESIAN_POINT('Ctrl Pts',(-82.9262630842284,5.91996244271229,3.78852954989618));
#31714=CARTESIAN_POINT('Ctrl Pts',(-82.9592923459673,6.37317997435674,2.73080654970013));
#31715=CARTESIAN_POINT('Ctrl Pts',(-82.9923216077062,6.82639750600119,1.6730835495041));
#31716=CARTESIAN_POINT('Ctrl Pts',(-83.0253508694451,7.01062126212906,0.50010098234701));
#31717=CARTESIAN_POINT('Ctrl Pts',(-83.058380131184,6.90346924300647,-0.645631325363448));
#31718=CARTESIAN_POINT('Ctrl Pts',(-83.0914093929228,6.79631722388389,-1.79136363307392));
#31719=CARTESIAN_POINT('Ctrl Pts',(-83.1244386546617,6.39778942951084,-2.90984568133773));
#31720=CARTESIAN_POINT('Ctrl Pts',(-83.1574679164006,5.75630441987701,-3.86518910574001));
#31721=CARTESIAN_POINT('Ctrl Pts',(-83.1904971781395,5.11481941024318,-4.82053253014231));
#31722=CARTESIAN_POINT('Ctrl Pts',(-83.2235264398784,4.23037718534855,-5.61273733068305));
#31723=CARTESIAN_POINT('Ctrl Pts',(-83.2565557016173,3.2104317785833,-6.14555572690456));
#31724=CARTESIAN_POINT('Ctrl Pts',(-83.2895849633562,2.19048637181805,-6.67837412312607));
#31725=CARTESIAN_POINT('Ctrl Pts',(-83.3226142250951,1.03503778318217,-6.95180611502837));
#31726=CARTESIAN_POINT('Ctrl Pts',(-83.3556434868339,-0.115534426365817,
-6.93263147684566));
#31727=CARTESIAN_POINT('Ctrl Pts',(-83.3886727485728,-1.26610663591381,
-6.91345683866295));
#31728=CARTESIAN_POINT('Ctrl Pts',(-83.4217020103117,-2.4118024663739,-6.60167557039524));
#31729=CARTESIAN_POINT('Ctrl Pts',(-83.4547312720506,-3.41342725408578,
-6.03516708786852));
#31730=CARTESIAN_POINT('Ctrl Pts',(-83.4877605337895,-4.41505204179766,
-5.46865860534179));
#31731=CARTESIAN_POINT('Ctrl Pts',(-83.5207897955284,-5.27260578676133,
-4.64742290855603));
#31732=CARTESIAN_POINT('Ctrl Pts',(-83.5538190572673,-5.88190123270214,
-3.67123484486677));
#31733=CARTESIAN_POINT('Ctrl Pts',(-83.5868483190062,-6.49119667864295,
-2.69504678117752));
#31734=CARTESIAN_POINT('Ctrl Pts',(-83.6198775807451,-6.85223382556092,
-1.56390635058475));
#31735=CARTESIAN_POINT('Ctrl Pts',(-83.652906842484,-6.92114898564465,-0.415239829420204));
#31736=CARTESIAN_POINT('Ctrl Pts',(-83.6568806737872,-6.92944033719148,
-0.277040949442562));
#31737=CARTESIAN_POINT('Ctrl Pts',(-83.6608545050905,-6.93350319817502,
-0.138588377815766));
#31738=CARTESIAN_POINT('Ctrl Pts',(-83.6648283363937,-6.93338479581795,
-0.000128863436223425));
#31739=CARTESIAN_POINT('Ctrl Pts',(-83.8441716636063,-6.93347143000264,
-0.000100837253274565));
#31740=CARTESIAN_POINT('Ctrl Pts',(-83.8412310421208,-6.9335439720405,-0.102556691006701));
#31741=CARTESIAN_POINT('Ctrl Pts',(-83.8382904206354,-6.93131982367475,
-0.205009393294928));
#31742=CARTESIAN_POINT('Ctrl Pts',(-83.8353497991499,-6.92677829211024,
-0.307359267230395));
#31743=CARTESIAN_POINT('Ctrl Pts',(-83.802320537411,-6.87576749881995,-1.45696005463907));
#31744=CARTESIAN_POINT('Ctrl Pts',(-83.7692912756721,-6.53239712170201,
-2.59358808275837));
#31745=CARTESIAN_POINT('Ctrl Pts',(-83.7362620139332,-5.93838444983376,
-3.57915036750032));
#31746=CARTESIAN_POINT('Ctrl Pts',(-83.7032327521943,-5.34437177796551,
-4.56471265224226));
#31747=CARTESIAN_POINT('Ctrl Pts',(-83.6702034904554,-4.49971681134696,
-5.39920919360684));
#31748=CARTESIAN_POINT('Ctrl Pts',(-83.6371742287166,-3.50703968776827,
-5.98125403704088));
#31749=CARTESIAN_POINT('Ctrl Pts',(-83.6041449669777,-2.51436256418959,
-6.5632988804749));
#31750=CARTESIAN_POINT('Ctrl Pts',(-83.5711157052388,-1.37366328365078,
-6.8928920259784));
#31751=CARTESIAN_POINT('Ctrl Pts',(-83.5380864434999,-0.223529461180919,
-6.92999002937145));
#31752=CARTESIAN_POINT('Ctrl Pts',(-83.505057181761,0.92660436128894,-6.9670880327645));
#31753=CARTESIAN_POINT('Ctrl Pts',(-83.4720279200221,2.08617272568984,-6.7116908940471));
#31754=CARTESIAN_POINT('Ctrl Pts',(-83.4389986582832,3.11429554484444,-6.19482772049098));
#31755=CARTESIAN_POINT('Ctrl Pts',(-83.4059693965443,4.14241836399906,-5.67796454693485));
#31756=CARTESIAN_POINT('Ctrl Pts',(-83.3729401348054,5.03909563790738,-4.89963533853999));
#31757=CARTESIAN_POINT('Ctrl Pts',(-83.3399108730665,5.69538685353336,-3.95440208069459));
#31758=CARTESIAN_POINT('Ctrl Pts',(-83.3068816113276,6.35167806915934,-3.0091688228492));
#31759=CARTESIAN_POINT('Ctrl Pts',(-83.2738523495888,6.76758322650299,-1.89703151555327));
#31760=CARTESIAN_POINT('Ctrl Pts',(-83.2408230878499,6.89257252790607,-0.753107678062462));
#31761=CARTESIAN_POINT('Ctrl Pts',(-83.207793826111,7.01756182930914,0.390816159428331));
#31762=CARTESIAN_POINT('Ctrl Pts',(-83.1747645643721,6.85163527477164,1.566526527114));
#31763=CARTESIAN_POINT('Ctrl Pts',(-83.1417353026332,6.41495187189151,2.63118218839321));
#31764=CARTESIAN_POINT('Ctrl Pts',(-83.1087060408942,5.97826846901137,3.69583784967243));
#31765=CARTESIAN_POINT('Ctrl Pts',(-83.0756767791554,5.27082821778859,4.64943880454518));
#31766=CARTESIAN_POINT('Ctrl Pts',(-83.0426475174165,4.37858055193037,5.37612867939927));
#31767=CARTESIAN_POINT('Ctrl Pts',(-83.0096182556777,3.48633288607215,6.10281855425335));
#31768=CARTESIAN_POINT('Ctrl Pts',(-82.9765889939388,2.40927780557849,6.60259734908875));
#31769=CARTESIAN_POINT('Ctrl Pts',(-82.9435597321999,1.27827056512267,6.81474515954507));
#31770=CARTESIAN_POINT('Ctrl Pts',(-82.910530470461,0.14726332466687,7.02689297000139));
#31771=CARTESIAN_POINT('Ctrl Pts',(-82.8775012087221,-1.0376960757511,6.95140979607861));
#31772=CARTESIAN_POINT('Ctrl Pts',(-82.8444719469832,-2.13264270162839,
6.59746635720057));
#31773=CARTESIAN_POINT('Ctrl Pts',(-82.8114426852443,-3.22758932750568,
6.24352291832251));
#31774=CARTESIAN_POINT('Ctrl Pts',(-82.7784134235054,-4.23252317884229,
5.61111921448919));
#31775=CARTESIAN_POINT('Ctrl Pts',(-82.7453841617665,-5.02535126575494,
4.77708822223092));
#31776=CARTESIAN_POINT('Ctrl Pts',(-82.7123549000276,-5.81817935266758,
3.94305722997265));
#31777=CARTESIAN_POINT('Ctrl Pts',(-82.6793256382887,-6.39890167515627,
2.90739894928944));
#31778=CARTESIAN_POINT('Ctrl Pts',(-82.6462963765498,-6.69696421163009,
1.79593919032573));
#31779=CARTESIAN_POINT('Ctrl Pts',(-82.6289214722353,-6.8537587561742,1.21126045562967));
#31780=CARTESIAN_POINT('Ctrl Pts',(-82.6115465679208,-6.93233450307243,
0.605605618975589));
#31781=CARTESIAN_POINT('Ctrl Pts',(-82.5941716636063,-6.93241904285695,
-2.76930968138527E-5));
#31782=CARTESIAN_POINT('Origin',(-87.75,0.,0.));
#31783=CARTESIAN_POINT('',(-81.1648283363937,-6.93341558550125,0.000120073986537225));
#31784=CARTESIAN_POINT('',(-81.3441716636063,-6.93331923438577,0.000144398752376666));
#31785=CARTESIAN_POINT('',(-87.75,-6.933,-8.4904762584886E-16));
#31786=CARTESIAN_POINT('Ctrl Pts',(-81.1648283363937,-6.93341558550125,
0.000120073986537225));
#31787=CARTESIAN_POINT('Ctrl Pts',(-81.1684562949515,-6.93351814222822,
0.126526778809456));
#31788=CARTESIAN_POINT('Ctrl Pts',(-81.1720842535094,-6.93013211229906,
0.252927991280468));
#31789=CARTESIAN_POINT('Ctrl Pts',(-81.1757122120672,-6.92322057912816,
0.379136136715153));
#31790=CARTESIAN_POINT('Ctrl Pts',(-81.2087414738061,-6.86029735812661,
1.52814646930247));
#31791=CARTESIAN_POINT('Ctrl Pts',(-81.241770735545,-6.5051647142299,2.66115454536162));
#31792=CARTESIAN_POINT('Ctrl Pts',(-81.2747999972839,-5.90096897616487,
3.64050718166668));
#31793=CARTESIAN_POINT('Ctrl Pts',(-81.3078292590228,-5.29677323809984,
4.61985981797174));
#31794=CARTESIAN_POINT('Ctrl Pts',(-81.3408585207617,-4.44351440586649,
5.44555701452271));
#31795=CARTESIAN_POINT('Ctrl Pts',(-81.3738877825006,-3.44485793150741,
6.01728188048037));
#31796=CARTESIAN_POINT('Ctrl Pts',(-81.4069170442394,-2.44620145714835,
6.58900674643802));
#31797=CARTESIAN_POINT('Ctrl Pts',(-81.4399463059783,-1.30214734066357,
6.90675928180237));
#31798=CARTESIAN_POINT('Ctrl Pts',(-81.4729755677172,-0.15169078804013,
6.93193460025776));
#31799=CARTESIAN_POINT('Ctrl Pts',(-81.5060048294561,0.998765764583344,
6.95710991871314));
#31800=CARTESIAN_POINT('Ctrl Pts',(-81.539034091195,2.15562475334548,6.68970802025954));
#31801=CARTESIAN_POINT('Ctrl Pts',(-81.5720633529339,3.17833526275718,6.16221651315021));
#31802=CARTESIAN_POINT('Ctrl Pts',(-81.6050926146728,4.20104577216889,5.63472500604088));
#31803=CARTESIAN_POINT('Ctrl Pts',(-81.6381218764117,5.08960780223017,4.84714389027584));
#31804=CARTESIAN_POINT('Ctrl Pts',(-81.6711511381506,5.73606678975991,3.8951591983949));
#31805=CARTESIAN_POINT('Ctrl Pts',(-81.7041803998895,6.38252577728964,2.94317450651398));
#31806=CARTESIAN_POINT('Ctrl Pts',(-81.7372096616284,6.78688172228784,1.82678623851717));
#31807=CARTESIAN_POINT('Ctrl Pts',(-81.7702389233673,6.9000079820046,0.681628378003572));
#31808=CARTESIAN_POINT('Ctrl Pts',(-81.8032681851061,7.01313424172135,-0.463529482510025));
#31809=CARTESIAN_POINT('Ctrl Pts',(-81.836297446845,6.83503081615665,-1.63745693554042));
#31810=CARTESIAN_POINT('Ctrl Pts',(-81.8693267085839,6.38733612430369,-2.69752935713257));
#31811=CARTESIAN_POINT('Ctrl Pts',(-81.9023559703228,5.93964143245071,-3.75760177872474));
#31812=CARTESIAN_POINT('Ctrl Pts',(-81.9353852320616,5.22235547430947,-4.70381916887868));
#31813=CARTESIAN_POINT('Ctrl Pts',(-81.9684144938006,4.32262387355884,-5.42122220953598));
#31814=CARTESIAN_POINT('Ctrl Pts',(-82.0014437555395,3.42289227280822,-6.13862525019326));
#31815=CARTESIAN_POINT('Ctrl Pts',(-82.0344730172784,2.34071502944824,-6.62721394135391));
#31816=CARTESIAN_POINT('Ctrl Pts',(-82.0675022790173,1.20756970794717,-6.82762790417546));
#31817=CARTESIAN_POINT('Ctrl Pts',(-82.1005315407562,0.0744243864461097,
-7.028041866997));
#31818=CARTESIAN_POINT('Ctrl Pts',(-82.133560802495,-1.10968901319603,-6.94028110147943));
#31819=CARTESIAN_POINT('Ctrl Pts',(-82.1665900642339,-2.20090834012137,
-6.57500797534202));
#31820=CARTESIAN_POINT('Ctrl Pts',(-82.1996193259728,-3.29212766704672,
-6.2097348492046));
#31821=CARTESIAN_POINT('Ctrl Pts',(-82.2326485877117,-4.29045292125526,
-5.56694936244733));
#31822=CARTESIAN_POINT('Ctrl Pts',(-82.2656778494506,-5.07459401484698,
-4.72474581135389));
#31823=CARTESIAN_POINT('Ctrl Pts',(-82.2987071111895,-5.8587351084387,-3.88254226026045));
#31824=CARTESIAN_POINT('Ctrl Pts',(-82.3317363729284,-6.4286920414136,-2.84092064483084));
#31825=CARTESIAN_POINT('Ctrl Pts',(-82.3647656346673,-6.71521871766388,
-1.72643128196972));
#31826=CARTESIAN_POINT('Ctrl Pts',(-82.3814532019094,-6.85998226746399,
-1.16335129760796));
#31827=CARTESIAN_POINT('Ctrl Pts',(-82.3981407691516,-6.93239648380404,
-0.581670853936292));
#31828=CARTESIAN_POINT('Ctrl Pts',(-82.4148283363938,-6.93241284950548,
5.58784473136953E-6));
#31829=CARTESIAN_POINT('Ctrl Pts',(-82.5941716636063,-6.93241904285695,
-2.76930968138527E-5));
#31830=CARTESIAN_POINT('Ctrl Pts',(-82.5785173061819,-6.93249521110396,
-0.545688271345749));
#31831=CARTESIAN_POINT('Ctrl Pts',(-82.5628629487576,-6.86885565040568,
-1.0913313768807));
#31832=CARTESIAN_POINT('Ctrl Pts',(-82.5472085913332,-6.74130112803958,
-1.62159992855644));
#31833=CARTESIAN_POINT('Ctrl Pts',(-82.5141793295943,-6.47217275751627,
-2.74041805123071));
#31834=CARTESIAN_POINT('Ctrl Pts',(-82.4811500678554,-5.91851326601068,
-3.79079305933502));
#31835=CARTESIAN_POINT('Ctrl Pts',(-82.4481208061165,-5.14758871546834,
-4.64511115513774));
#31836=CARTESIAN_POINT('Ctrl Pts',(-82.4150915443776,-4.37666416492601,
-5.49942925094045));
#31837=CARTESIAN_POINT('Ctrl Pts',(-82.3820622826387,-3.38847455534694,
-6.15769043444157));
#31838=CARTESIAN_POINT('Ctrl Pts',(-82.3490330208998,-2.30307855909514,
-6.53992021188625));
#31839=CARTESIAN_POINT('Ctrl Pts',(-82.3160037591609,-1.21768256284332,
-6.92214998933094));
#31840=CARTESIAN_POINT('Ctrl Pts',(-82.2829744974221,-0.0350801799187911,
-7.02834836071917));
#31841=CARTESIAN_POINT('Ctrl Pts',(-82.2499452356832,1.10105001761894,-6.84561290798008));
#31842=CARTESIAN_POINT('Ctrl Pts',(-82.2169159739443,2.23718021515667,-6.66287745524098));
#31843=CARTESIAN_POINT('Ctrl Pts',(-82.1838867122054,3.32683822730758,-6.19120817837455));
#31844=CARTESIAN_POINT('Ctrl Pts',(-82.1508574504665,4.23763762438095,-5.48790985636909));
#31845=CARTESIAN_POINT('Ctrl Pts',(-82.1178281887276,5.14843702145431,-4.78461153436364));
#31846=CARTESIAN_POINT('Ctrl Pts',(-82.0847989269887,5.88037780345013,-3.84968416721917));
#31847=CARTESIAN_POINT('Ctrl Pts',(-82.0517696652499,6.34453387998692,-2.79671540792056));
#31848=CARTESIAN_POINT('Ctrl Pts',(-82.018740403511,6.8086899565237,-1.74374664862195));
#31849=CARTESIAN_POINT('Ctrl Pts',(-81.9857111417721,7.00506132760144,-0.572736497169197));
#31850=CARTESIAN_POINT('Ctrl Pts',(-81.9526818800332,6.90979013651598,0.574044855833212));
#31851=CARTESIAN_POINT('Ctrl Pts',(-81.9196526182943,6.81451894543051,1.72082620883562));
#31852=CARTESIAN_POINT('Ctrl Pts',(-81.8866233565553,6.42760519218184,2.84337876338767));
#31853=CARTESIAN_POINT('Ctrl Pts',(-81.8535940948165,5.79605640557224,3.80531961477969));
#31854=CARTESIAN_POINT('Ctrl Pts',(-81.8205648330776,5.16450761896264,4.76726046617172));
#31855=CARTESIAN_POINT('Ctrl Pts',(-81.7875355713387,4.28832379899209,5.56858961440372));
#31856=CARTESIAN_POINT('Ctrl Pts',(-81.7545063095998,3.27395563604716,6.11195072954594));
#31857=CARTESIAN_POINT('Ctrl Pts',(-81.721477047861,2.25958747310221,6.65531184468816));
#31858=CARTESIAN_POINT('Ctrl Pts',(-81.688447786122,1.10703496718287,6.94070492674061));
#31859=CARTESIAN_POINT('Ctrl Pts',(-81.6554185243831,-0.0436741761479686,
6.93345655452891));
#31860=CARTESIAN_POINT('Ctrl Pts',(-81.6223892626442,-1.19438331947877,
6.9262081823172));
#31861=CARTESIAN_POINT('Ctrl Pts',(-81.5893600009054,-2.34324910022105,
6.62631835584136));
#31862=CARTESIAN_POINT('Ctrl Pts',(-81.5563307391665,-3.35069172617371,
6.0702217573457));
#31863=CARTESIAN_POINT('Ctrl Pts',(-81.5233014774276,-4.35813435212639,
5.51412515885003));
#31864=CARTESIAN_POINT('Ctrl Pts',(-81.4902722156887,-5.22415382328944,
4.70182178833453));
#31865=CARTESIAN_POINT('Ctrl Pts',(-81.4572429539498,-5.84353435218509,
3.7320012730484));
#31866=CARTESIAN_POINT('Ctrl Pts',(-81.4242136922109,-6.46291488108073,
2.76218075776228));
#31867=CARTESIAN_POINT('Ctrl Pts',(-81.391184430472,-6.83565646770898,1.63484309770552));
#31868=CARTESIAN_POINT('Ctrl Pts',(-81.3581551687331,-6.91647341022511,
0.486952557084495));
#31869=CARTESIAN_POINT('Ctrl Pts',(-81.3534940003575,-6.92787849035219,
0.324959499870164));
#31870=CARTESIAN_POINT('Ctrl Pts',(-81.3488328319819,-6.9334697367279,0.162557121164403));
#31871=CARTESIAN_POINT('Ctrl Pts',(-81.3441716636063,-6.93331923438577,
0.000144398752376666));
#31872=CARTESIAN_POINT('Origin',(-87.75,0.,0.));
#31873=CARTESIAN_POINT('',(-79.9148283363937,-6.93284541734693,-0.000174722887704981));
#31874=CARTESIAN_POINT('',(-80.0941716636063,-6.93295492521967,-0.000178757583534305));
#31875=CARTESIAN_POINT('',(-87.75,-6.933,-8.4904762584886E-16));
#31876=CARTESIAN_POINT('Ctrl Pts',(-79.9148283363937,-6.93284541734693,
-0.000174722887704981));
#31877=CARTESIAN_POINT('Ctrl Pts',(-79.9387718207516,-6.9320436991393,0.834271057150727));
#31878=CARTESIAN_POINT('Ctrl Pts',(-79.9627153051094,-6.78122672642066,
1.66899880820083));
#31879=CARTESIAN_POINT('Ctrl Pts',(-79.9866587894672,-6.48653785546341,
2.44939871133041));
#31880=CARTESIAN_POINT('Ctrl Pts',(-80.0196880512061,-6.08002409560584,
3.52593511999483));
#31881=CARTESIAN_POINT('Ctrl Pts',(-80.052717312945,-5.39973204692025,4.49908938508927));
#31882=CARTESIAN_POINT('Ctrl Pts',(-80.0857465746839,-4.52831281137459,
5.25062953175785));
#31883=CARTESIAN_POINT('Ctrl Pts',(-80.1187758364227,-3.65689357582891,
6.00216967842645));
#31884=CARTESIAN_POINT('Ctrl Pts',(-80.1518050981616,-2.59434715342316,
6.53209570666917));
#31885=CARTESIAN_POINT('Ctrl Pts',(-80.1848343599005,-1.46976609032717,
6.77602501745318));
#31886=CARTESIAN_POINT('Ctrl Pts',(-80.2178636216394,-0.345185027231233,
7.01995432823717));
#31887=CARTESIAN_POINT('Ctrl Pts',(-80.2508928833782,0.841430676554926,
6.97788692156249));
#31888=CARTESIAN_POINT('Ctrl Pts',(-80.2839221451171,1.94591485633796,6.6549337163724));
#31889=CARTESIAN_POINT('Ctrl Pts',(-80.3169514068561,3.050399036121,6.33198051118231));
#31890=CARTESIAN_POINT('Ctrl Pts',(-80.349980668595,4.07275169190092,5.72814150747681));
#31891=CARTESIAN_POINT('Ctrl Pts',(-80.3830099303339,4.88876356125384,4.91677925471376));
#31892=CARTESIAN_POINT('Ctrl Pts',(-80.4160391920728,5.70477543060677,4.1054170019507));
#31893=CARTESIAN_POINT('Ctrl Pts',(-80.4490684538116,6.31444651353271,3.08653150013008));
#31894=CARTESIAN_POINT('Ctrl Pts',(-80.4820977155505,6.64370570051452,1.9839107748026));
#31895=CARTESIAN_POINT('Ctrl Pts',(-80.5151269772894,6.97296488749633,0.881290049475117));
#31896=CARTESIAN_POINT('Ctrl Pts',(-80.5481562390284,7.02181217853402,-0.305065899359219));
#31897=CARTESIAN_POINT('Ctrl Pts',(-80.5811855007673,6.78431294240529,-1.43102246556055));
#31898=CARTESIAN_POINT('Ctrl Pts',(-80.6142147625062,6.54681370627656,-2.55697903176186));
#31899=CARTESIAN_POINT('Ctrl Pts',(-80.647244024245,6.02296794298142,-3.62253621533017));
#31900=CARTESIAN_POINT('Ctrl Pts',(-80.6802732859838,5.27641953852623,-4.49823568200751));
#31901=CARTESIAN_POINT('Ctrl Pts',(-80.7133025477227,4.52987113407103,-5.37393514868486));
#31902=CARTESIAN_POINT('Ctrl Pts',(-80.7463318094616,3.56062008845578,-6.05977689847124));
#31903=CARTESIAN_POINT('Ctrl Pts',(-80.7793610712005,2.48642416051135,-6.47243557646211));
#31904=CARTESIAN_POINT('Ctrl Pts',(-80.8123903329394,1.41222823256689,-6.88509425445299));
#31905=CARTESIAN_POINT('Ctrl Pts',(-80.8454195946783,0.233087422293255,
-7.02456986064836));
#31906=CARTESIAN_POINT('Ctrl Pts',(-80.8784488564172,-0.90774025703015,
-6.87391700729604));
#31907=CARTESIAN_POINT('Ctrl Pts',(-80.9114781181561,-2.04856793635356,
-6.72326415394373));
#31908=CARTESIAN_POINT('Ctrl Pts',(-80.944507379895,-3.15108248472673,-6.28248284104374));
#31909=CARTESIAN_POINT('Ctrl Pts',(-80.9775366416339,-4.08133548612042,
-5.60512515892028));
#31910=CARTESIAN_POINT('Ctrl Pts',(-81.0105659033728,-5.01158848751409,
-4.92776747679684));
#31911=CARTESIAN_POINT('Ctrl Pts',(-81.0435951651117,-5.76957994192829,
-4.01383342544995));
#31912=CARTESIAN_POINT('Ctrl Pts',(-81.0766244268506,-6.26321877008219,
-2.97436010521878));
#31913=CARTESIAN_POINT('Ctrl Pts',(-81.1060257300316,-6.7026359439577,-2.04906330390524));
#31914=CARTESIAN_POINT('Ctrl Pts',(-81.1354270332127,-6.93258445654129,
-1.02429125634669));
#31915=CARTESIAN_POINT('Ctrl Pts',(-81.1648283363937,-6.93341558550125,
0.000120073986537225));
#31916=CARTESIAN_POINT('Ctrl Pts',(-81.3441716636063,-6.93331923438577,
0.000144398752376666));
#31917=CARTESIAN_POINT('Ctrl Pts',(-81.315803570243,-6.93240326994323,-0.988307187091753));
#31918=CARTESIAN_POINT('Ctrl Pts',(-81.2874354768797,-6.71881306293981,
-1.97714190358189));
#31919=CARTESIAN_POINT('Ctrl Pts',(-81.2590673835164,-6.30879853137859,
-2.87641935706139));
#31920=CARTESIAN_POINT('Ctrl Pts',(-81.2260381217775,-5.83141441161191,
-3.92345730940097));
#31921=CARTESIAN_POINT('Ctrl Pts',(-81.1930088600387,-5.08775387367453,
-4.84908979289483));
#31922=CARTESIAN_POINT('Ctrl Pts',(-81.1599795982998,-4.16816688280468,
-5.54085842305075));
#31923=CARTESIAN_POINT('Ctrl Pts',(-81.1269503365609,-3.24857989193482,
-6.23262705320668));
#31924=CARTESIAN_POINT('Ctrl Pts',(-81.093921074822,-2.15306644813249,-6.69053183002466));
#31925=CARTESIAN_POINT('Ctrl Pts',(-81.0608918130831,-1.01472437831761,
-6.85894027261136));
#31926=CARTESIAN_POINT('Ctrl Pts',(-81.0278625513442,0.123617691497245,
-7.02734871519806));
#31927=CARTESIAN_POINT('Ctrl Pts',(-80.9948332896053,1.30478838732467,-6.90626082355348));
#31928=CARTESIAN_POINT('Ctrl Pts',(-80.9618040278665,2.38528307786546,-6.51038799655218));
#31929=CARTESIAN_POINT('Ctrl Pts',(-80.9287747661276,3.46577776840626,-6.11451516955088));
#31930=CARTESIAN_POINT('Ctrl Pts',(-80.8957455043887,4.44559645366045,-5.44385740719286));
#31931=CARTESIAN_POINT('Ctrl Pts',(-80.8627162426498,5.2056974746501,-4.57989530771432));
#31932=CARTESIAN_POINT('Ctrl Pts',(-80.8296869809109,5.96579849563975,-3.71593320823578));
#31933=CARTESIAN_POINT('Ctrl Pts',(-80.796657719172,6.50618185236486,-2.65866677163672));
#31934=CARTESIAN_POINT('Ctrl Pts',(-80.7636284574331,6.76119444774047,-1.53654705982131));
#31935=CARTESIAN_POINT('Ctrl Pts',(-80.7305991956942,7.01620704311609,-0.414427348005899));
#31936=CARTESIAN_POINT('Ctrl Pts',(-80.6975699339554,6.98584887714221,0.772545639025848));
#31937=CARTESIAN_POINT('Ctrl Pts',(-80.6645406722164,6.67380827143942,1.8801623289676));
#31938=CARTESIAN_POINT('Ctrl Pts',(-80.6315114104775,6.36176766573663,2.98777901890934));
#31939=CARTESIAN_POINT('Ctrl Pts',(-80.5984821487386,5.76804462030492,4.01603941176109));
#31940=CARTESIAN_POINT('Ctrl Pts',(-80.5654528869998,4.96477266083155,4.8400164930981));
#31941=CARTESIAN_POINT('Ctrl Pts',(-80.5324236252609,4.16150070135818,5.66399357443512));
#31942=CARTESIAN_POINT('Ctrl Pts',(-80.499394363522,3.14867982784313,6.28368734425741));
#31943=CARTESIAN_POINT('Ctrl Pts',(-80.4663651017831,2.04936125256192,6.6238090011488));
#31944=CARTESIAN_POINT('Ctrl Pts',(-80.4333358400442,0.950042677280704,
6.9639306580402));
#31945=CARTESIAN_POINT('Ctrl Pts',(-80.4003065783053,-0.235773599766704,
7.02448020200071));
#31946=CARTESIAN_POINT('Ctrl Pts',(-80.3672773165664,-1.36401853908634,
6.79810125345532));
#31947=CARTESIAN_POINT('Ctrl Pts',(-80.3342480548275,-2.49226347840598,
6.57172230490993));
#31948=CARTESIAN_POINT('Ctrl Pts',(-80.3012187930887,-3.56293707999787,
6.05841486385864));
#31949=CARTESIAN_POINT('Ctrl Pts',(-80.2681895313498,-4.44595939777042,
5.32054247803539));
#31950=CARTESIAN_POINT('Ctrl Pts',(-80.2351602696109,-5.32898171554296,
4.58267009221216));
#31951=CARTESIAN_POINT('Ctrl Pts',(-80.2021310078719,-6.02435274949617,
3.62023276161698));
#31952=CARTESIAN_POINT('Ctrl Pts',(-80.169101746133,-6.44758939807997,2.55016042259479));
#31953=CARTESIAN_POINT('Ctrl Pts',(-80.1441250519574,-6.76764052181244,
1.74097280681279));
#31954=CARTESIAN_POINT('Ctrl Pts',(-80.1191483577819,-6.93207516122631,
0.870235521082701));
#31955=CARTESIAN_POINT('Ctrl Pts',(-80.0941716636063,-6.93295492521967,
-0.000178757583534305));
#31956=CARTESIAN_POINT('Origin',(-87.75,0.,0.));
#31957=CARTESIAN_POINT('',(-78.6648283363938,-6.93264414159005,0.000146499032823016));
#31958=CARTESIAN_POINT('',(-78.8441716636063,-6.93256537376933,0.000124608584710398));
#31959=CARTESIAN_POINT('',(-87.75,-6.933,-8.4904762584886E-16));
#31960=CARTESIAN_POINT('Ctrl Pts',(-78.6648283363938,-6.93264414159005,
0.000146499032823016));
#31961=CARTESIAN_POINT('Ctrl Pts',(-78.6760580848127,-6.93294570416691,
0.391543037810179));
#31962=CARTESIAN_POINT('Ctrl Pts',(-78.6872878332316,-6.90035368842132,
0.782889892230009));
#31963=CARTESIAN_POINT('Ctrl Pts',(-78.6985175816505,-6.83441674149118,
1.16853549413445));
#31964=CARTESIAN_POINT('Ctrl Pts',(-78.7315468433894,-6.64048108085322,
2.30280752308806));
#31965=CARTESIAN_POINT('Ctrl Pts',(-78.7645761051282,-6.15808415438807,
3.38775899689383));
#31966=CARTESIAN_POINT('Ctrl Pts',(-78.7976053668671,-5.44583408141055,
4.29157529995388));
#31967=CARTESIAN_POINT('Ctrl Pts',(-78.830634628606,-4.73358400843304,5.19539160301392));
#31968=CARTESIAN_POINT('Ctrl Pts',(-78.8636638903449,-3.79148078894316,
5.91807273532824));
#31969=CARTESIAN_POINT('Ctrl Pts',(-78.8966931520838,-2.73398389576414,
6.37181759430771));
#31970=CARTESIAN_POINT('Ctrl Pts',(-78.9297224138227,-1.67648700258512,
6.82556245328718));
#31971=CARTESIAN_POINT('Ctrl Pts',(-78.9627516755616,-0.50359643571695,
7.0103710389318));
#31972=CARTESIAN_POINT('Ctrl Pts',(-78.9957809373005,0.642189155875181,
6.90379029848845));
#31973=CARTESIAN_POINT('Ctrl Pts',(-79.0288101990394,1.78797474746733,6.7972095580451));
#31974=CARTESIAN_POINT('Ctrl Pts',(-79.0618394607782,2.90665536378344,6.39923949151378));
#31975=CARTESIAN_POINT('Ctrl Pts',(-79.0948687225171,3.86231851566927,5.75823089854386));
#31976=CARTESIAN_POINT('Ctrl Pts',(-79.127897984256,4.81798166755509,5.11722230557395));
#31977=CARTESIAN_POINT('Ctrl Pts',(-79.1609272459949,5.61062735501063,4.23317518616545));
#31978=CARTESIAN_POINT('Ctrl Pts',(-79.1939565077338,6.14395423265796,3.21349557093693));
#31979=CARTESIAN_POINT('Ctrl Pts',(-79.2269857694727,6.67728111030527,2.19381595570843));
#31980=CARTESIAN_POINT('Ctrl Pts',(-79.2600150312116,6.95128917814437,1.03850384465991));
#31981=CARTESIAN_POINT('Ctrl Pts',(-79.2930442929505,6.93268822089381,-0.112077782397874));
#31982=CARTESIAN_POINT('Ctrl Pts',(-79.3260735546894,6.91408726364324,-1.26265940945566));
#31983=CARTESIAN_POINT('Ctrl Pts',(-79.3591028164283,6.60287728130299,-2.40851055252272));
#31984=CARTESIAN_POINT('Ctrl Pts',(-79.3921320781672,6.03686828213871,-3.41041767845737));
#31985=CARTESIAN_POINT('Ctrl Pts',(-79.425161339906,5.47085928297442,-4.41232480439202));
#31986=CARTESIAN_POINT('Ctrl Pts',(-79.4581906016449,4.6500512669861,-5.27028791319426));
#31987=CARTESIAN_POINT('Ctrl Pts',(-79.4912198633838,3.67416712106713,-5.88007001351993));
#31988=CARTESIAN_POINT('Ctrl Pts',(-79.5242491251227,2.69828297514816,-6.48985211384559));
#31989=CARTESIAN_POINT('Ctrl Pts',(-79.5572783868616,1.56732269929855,-6.85145320569469));
#31990=CARTESIAN_POINT('Ctrl Pts',(-79.5903076486005,0.4186906822092,-6.92094108557919));
#31991=CARTESIAN_POINT('Ctrl Pts',(-79.6233369103394,-0.729941334880146,
-6.9904289654637));
#31992=CARTESIAN_POINT('Ctrl Pts',(-79.6563661720783,-1.89624509320922,
-6.76780363338362));
#31993=CARTESIAN_POINT('Ctrl Pts',(-79.6893954338172,-2.93852219862291,
-6.28011263319595));
#31994=CARTESIAN_POINT('Ctrl Pts',(-79.7224246955561,-3.98079930403662,
-5.79242163300826));
#31995=CARTESIAN_POINT('Ctrl Pts',(-79.755453957295,-4.89904975653494,-5.03966496471298));
#31996=CARTESIAN_POINT('Ctrl Pts',(-79.7884832190338,-5.58171204084191,
-4.11329771479616));
#31997=CARTESIAN_POINT('Ctrl Pts',(-79.8215124807727,-6.26437432514887,
-3.18693046487936));
#31998=CARTESIAN_POINT('Ctrl Pts',(-79.8545417425116,-6.71144844126449,
-2.08695263334102));
#31999=CARTESIAN_POINT('Ctrl Pts',(-79.8875710042505,-6.86861776380751,
-0.947004441454659));
#32000=CARTESIAN_POINT('Ctrl Pts',(-79.8966567816316,-6.91185232009428,
-0.63342445352396));
#32001=CARTESIAN_POINT('Ctrl Pts',(-79.9057425590127,-6.93314964345906,
-0.316819889510455));
#32002=CARTESIAN_POINT('Ctrl Pts',(-79.9148283363937,-6.93284541734693,
-0.000174722887704981));
#32003=CARTESIAN_POINT('Ctrl Pts',(-80.0941716636063,-6.93295492521967,
-0.000178757583534305));
#32004=CARTESIAN_POINT('Ctrl Pts',(-80.086119096043,-6.93323856399694,-0.280803156382215));
#32005=CARTESIAN_POINT('Ctrl Pts',(-80.0780665284797,-6.9165216776303,-0.561393980579732));
#32006=CARTESIAN_POINT('Ctrl Pts',(-80.0700139609165,-6.88253823603364,
-0.839877762973264));
#32007=CARTESIAN_POINT('Ctrl Pts',(-80.0369846991776,-6.74314816218912,
-1.98213626206991));
#32008=CARTESIAN_POINT('Ctrl Pts',(-80.0039554374386,-6.31326575128568,
-3.08894591281398));
#32009=CARTESIAN_POINT('Ctrl Pts',(-79.9709261756997,-5.64511894725778,
-4.0258364719041));
#32010=CARTESIAN_POINT('Ctrl Pts',(-79.9378969139608,-4.97697214322988,
-4.96272703099423));
#32011=CARTESIAN_POINT('Ctrl Pts',(-79.904867652222,-4.07056094607752,-5.72969849843039));
#32012=CARTESIAN_POINT('Ctrl Pts',(-79.8718383904831,-3.03600847781199,
-6.23356878119234));
#32013=CARTESIAN_POINT('Ctrl Pts',(-79.8388091287442,-2.00145600954648,
-6.73743906395428));
#32014=CARTESIAN_POINT('Ctrl Pts',(-79.8057798670053,-0.838762270167813,
-6.97820816204202));
#32015=CARTESIAN_POINT('Ctrl Pts',(-79.7727506052664,0.310812940218244,
-6.92662418089757));
#32016=CARTESIAN_POINT('Ctrl Pts',(-79.7397213435275,1.46038815060428,-6.87504019975313));
#32017=CARTESIAN_POINT('Ctrl Pts',(-79.7066920817886,2.59684483199772,-6.5311031393765));
#32018=CARTESIAN_POINT('Ctrl Pts',(-79.6736628200497,3.58211081783791,-5.93659913721069));
#32019=CARTESIAN_POINT('Ctrl Pts',(-79.6406335583108,4.56737680367813,-5.34209513504485));
#32020=CARTESIAN_POINT('Ctrl Pts',(-79.6076042965719,5.40145209396511,-4.49702419108981));
#32021=CARTESIAN_POINT('Ctrl Pts',(-79.574575034833,5.98300191343629,-3.50405698170275));
#32022=CARTESIAN_POINT('Ctrl Pts',(-79.5415457730942,6.56455173290748,-2.51108977231567));
#32023=CARTESIAN_POINT('Ctrl Pts',(-79.5085165113553,6.89357608156287,-1.37022629749662));
#32024=CARTESIAN_POINT('Ctrl Pts',(-79.4754872496164,6.93010062037677,-0.220074120822001));
#32025=CARTESIAN_POINT('Ctrl Pts',(-79.4424579878775,6.96662515919067,0.93007805585257));
#32026=CARTESIAN_POINT('Ctrl Pts',(-79.4094287261386,6.71064988816308,2.08951893438267));
#32027=CARTESIAN_POINT('Ctrl Pts',(-79.3763994643997,6.19327415391706,3.11738391630306));
#32028=CARTESIAN_POINT('Ctrl Pts',(-79.3433702026608,5.67589841967103,4.14524889822346));
#32029=CARTESIAN_POINT('Ctrl Pts',(-79.310340940922,4.89712222220651,5.0415379835342));
#32030=CARTESIAN_POINT('Ctrl Pts',(-79.2773116791831,3.95156185320478,5.69735782161336));
#32031=CARTESIAN_POINT('Ctrl Pts',(-79.2442824174442,3.00600148420302,6.35317765969253));
#32032=CARTESIAN_POINT('Ctrl Pts',(-79.2112531557053,1.89365694366406,6.76852825054014));
#32033=CARTESIAN_POINT('Ctrl Pts',(-79.1782238939664,0.749670928347523,
6.89294717275511));
#32034=CARTESIAN_POINT('Ctrl Pts',(-79.1451946322275,-0.394315086968993,
7.01736609497008));
#32035=CARTESIAN_POINT('Ctrl Pts',(-79.1121653704886,-1.56994257706304,
6.8508533485524));
#32036=CARTESIAN_POINT('Ctrl Pts',(-79.0791361087497,-2.63438037442674,
6.41363915963763));
#32037=CARTESIAN_POINT('Ctrl Pts',(-79.0461068470108,-3.69881817179041,
5.97642497072288));
#32038=CARTESIAN_POINT('Ctrl Pts',(-79.0130775852719,-4.65206627642376,
5.26850933931104));
#32039=CARTESIAN_POINT('Ctrl Pts',(-78.980048323533,-5.37831118374589,4.37589945474024));
#32040=CARTESIAN_POINT('Ctrl Pts',(-78.9470190617941,-6.10455609106804,
3.48328957016942));
#32041=CARTESIAN_POINT('Ctrl Pts',(-78.9139898000553,-6.60379780107896,
2.40598543243962));
#32042=CARTESIAN_POINT('Ctrl Pts',(-78.8809605383164,-6.81538166176488,
1.27487255507408));
#32043=CARTESIAN_POINT('Ctrl Pts',(-78.8686975800797,-6.89393758189603,
0.854917967963368));
#32044=CARTESIAN_POINT('Ctrl Pts',(-78.856434621843,-6.93284114622974,0.427546085291084));
#32045=CARTESIAN_POINT('Ctrl Pts',(-78.8441716636063,-6.93256537376933,
0.000124608584710398));
#32046=CARTESIAN_POINT('Origin',(-87.75,0.,0.));
#32047=CARTESIAN_POINT('',(-77.4148283363937,-6.93355988365441,-5.3614765520571E-5));
#32048=CARTESIAN_POINT('',(-77.5941716636063,-6.93359074487482,-1.65665743479807E-5));
#32049=CARTESIAN_POINT('',(-87.75,-6.933,-8.4904762584886E-16));
#32050=CARTESIAN_POINT('Ctrl Pts',(-77.4148283363937,-6.93355988365441,
-5.3614765520571E-5));
#32051=CARTESIAN_POINT('Ctrl Pts',(-77.4463736106126,-6.9331052532896,1.09899237861107));
#32052=CARTESIAN_POINT('Ctrl Pts',(-77.4779188848315,-6.66710498440094,
2.198250639548));
#32053=CARTESIAN_POINT('Ctrl Pts',(-77.5094641590504,-6.16380047409797,
3.17526236914945));
#32054=CARTESIAN_POINT('Ctrl Pts',(-77.5424934207893,-5.63681895890149,
4.19823576018895));
#32055=CARTESIAN_POINT('Ctrl Pts',(-77.5755226825282,-4.8496809805689,5.08719036996541));
#32056=CARTESIAN_POINT('Ctrl Pts',(-77.6085519442671,-3.89801873329636,
5.73412393939105));
#32057=CARTESIAN_POINT('Ctrl Pts',(-77.641581206006,-2.94635648602384,6.38105750881668));
#32058=CARTESIAN_POINT('Ctrl Pts',(-77.6746104677449,-1.83016996981136,
6.7859700378915));
#32059=CARTESIAN_POINT('Ctrl Pts',(-77.7076397294838,-0.685068656715781,
6.89966726248539));
#32060=CARTESIAN_POINT('Ctrl Pts',(-77.7406689912226,0.460032656379802,
7.01336448707927));
#32061=CARTESIAN_POINT('Ctrl Pts',(-77.7736982529615,1.6340487663585,6.83584640719222));
#32062=CARTESIAN_POINT('Ctrl Pts',(-77.8067275147004,2.69434427801713,6.38868032608795));
#32063=CARTESIAN_POINT('Ctrl Pts',(-77.8397567764393,3.75463978967577,5.94151424498368));
#32064=CARTESIAN_POINT('Ctrl Pts',(-77.8727860381782,4.70121470301435,5.22470016266219));
#32065=CARTESIAN_POINT('Ctrl Pts',(-77.9058152999171,5.41906626321042,4.32532637292975));
#32066=CARTESIAN_POINT('Ctrl Pts',(-77.938844561656,6.13691782340649,3.42595258319731));
#32067=CARTESIAN_POINT('Ctrl Pts',(-77.9718738233948,6.62604603046005,2.34401908605393));
#32068=CARTESIAN_POINT('Ctrl Pts',(-78.0049030851337,6.82702495782282,1.21097383237262));
#32069=CARTESIAN_POINT('Ctrl Pts',(-78.0379323468726,7.02800388518558,0.0779285786913365));
#32070=CARTESIAN_POINT('Ctrl Pts',(-78.0709616086116,6.94083353285755,-1.10622843152787));
#32071=CARTESIAN_POINT('Ctrl Pts',(-78.1039908703505,6.57610453715848,-2.19762974902292));
#32072=CARTESIAN_POINT('Ctrl Pts',(-78.1370201320894,6.21137554145941,-3.28903106651797));
#32073=CARTESIAN_POINT('Ctrl Pts',(-78.1700493938282,5.56908790238929,-4.28767669128886));
#32074=CARTESIAN_POINT('Ctrl Pts',(-78.2030786555671,4.7272754309446,-5.07223761247583));
#32075=CARTESIAN_POINT('Ctrl Pts',(-78.236107917306,3.88546295949989,-5.85679853366282));
#32076=CARTESIAN_POINT('Ctrl Pts',(-78.2691371790449,2.8441256556806,-6.42727475126589));
#32077=CARTESIAN_POINT('Ctrl Pts',(-78.3021664407838,1.72977929436205,-6.71435707943979));
#32078=CARTESIAN_POINT('Ctrl Pts',(-78.3351957025227,0.615432933043514,
-7.00143940761369));
#32079=CARTESIAN_POINT('Ctrl Pts',(-78.3682249642616,-0.571922485774274,
-7.00512784635843));
#32080=CARTESIAN_POINT('Ctrl Pts',(-78.4012542260005,-1.68803092678632,
-6.72497427412476));
#32081=CARTESIAN_POINT('Ctrl Pts',(-78.4342834877393,-2.80413936779834,
-6.44482070189109));
#32082=CARTESIAN_POINT('Ctrl Pts',(-78.4673127494782,-3.84900083100463,
-5.88082511867903));
#32083=CARTESIAN_POINT('Ctrl Pts',(-78.5003420112171,-4.69567137886439,
-5.10150935499884));
#32084=CARTESIAN_POINT('Ctrl Pts',(-78.533371272956,-5.54234192672416,-4.32219359131866));
#32085=CARTESIAN_POINT('Ctrl Pts',(-78.5664005346949,-6.1908215592374,-3.32755764717036));
#32086=CARTESIAN_POINT('Ctrl Pts',(-78.5994297964338,-6.56232417808864,
-2.23844338304549));
#32087=CARTESIAN_POINT('Ctrl Pts',(-78.6212293097538,-6.80751816250399,
-1.51962135500671));
#32088=CARTESIAN_POINT('Ctrl Pts',(-78.6430288230738,-6.93205873956981,
-0.759643813464775));
#32089=CARTESIAN_POINT('Ctrl Pts',(-78.6648283363938,-6.93264414159005,
0.000146499032823016));
#32090=CARTESIAN_POINT('Ctrl Pts',(-78.8441716636063,-6.93256537376933,
0.000124608584710398));
#32091=CARTESIAN_POINT('Ctrl Pts',(-78.8234053601041,-6.9320983759618,-0.723678240394669));
#32092=CARTESIAN_POINT('Ctrl Pts',(-78.8026390566018,-6.81927829988588,
-1.44762330827946));
#32093=CARTESIAN_POINT('Ctrl Pts',(-78.7818727530997,-6.59640219545387,
-2.13593195186867));
#32094=CARTESIAN_POINT('Ctrl Pts',(-78.7488434913608,-6.24191285709603,
-3.23070196444461));
#32095=CARTESIAN_POINT('Ctrl Pts',(-78.715814229622,-5.60900816901946,-4.23532037259521));
#32096=CARTESIAN_POINT('Ctrl Pts',(-78.6827849678831,-4.77458197411304,
-5.02773251075243));
#32097=CARTESIAN_POINT('Ctrl Pts',(-78.6497557061442,-3.94015577920663,
-5.82014464890964));
#32098=CARTESIAN_POINT('Ctrl Pts',(-78.6167264444052,-2.9042080774704,-6.40035051707347));
#32099=CARTESIAN_POINT('Ctrl Pts',(-78.5836971826663,-1.79259984184248,
-6.69785883952688));
#32100=CARTESIAN_POINT('Ctrl Pts',(-78.5506679209274,-0.680991606214557,
-6.9953671619803));
#32101=CARTESIAN_POINT('Ctrl Pts',(-78.5176386591886,0.506277163305044,
-7.01017793872329));
#32102=CARTESIAN_POINT('Ctrl Pts',(-78.4846093974497,1.62496095874294,-6.74049175578187));
#32103=CARTESIAN_POINT('Ctrl Pts',(-78.4515801357108,2.74364475418086,-6.47080557284044));
#32104=CARTESIAN_POINT('Ctrl Pts',(-78.4185508739719,3.79374357553707,-5.91662243021457));
#32105=CARTESIAN_POINT('Ctrl Pts',(-78.385521612233,4.64767717999083,-5.14527201008796));
#32106=CARTESIAN_POINT('Ctrl Pts',(-78.3524923504941,5.50161078444459,-4.37392158996134));
#32107=CARTESIAN_POINT('Ctrl Pts',(-78.3194630887553,6.15937917199591,-3.38540389233398));
#32108=CARTESIAN_POINT('Ctrl Pts',(-78.2864338270164,6.54106772042358,-2.29981745015442));
#32109=CARTESIAN_POINT('Ctrl Pts',(-78.2534045652775,6.92275626885124,-1.21423100797489));
#32110=CARTESIAN_POINT('Ctrl Pts',(-78.2203753035385,7.02836497815528,-0.0315758212431301));
#32111=CARTESIAN_POINT('Ctrl Pts',(-78.1873460417997,6.84506307040986,1.10446312265876));
#32112=CARTESIAN_POINT('Ctrl Pts',(-78.1543167800608,6.66176116266444,2.24050206656066));
#32113=CARTESIAN_POINT('Ctrl Pts',(-78.1212875183219,6.18954863786957,3.32992476763274));
#32114=CARTESIAN_POINT('Ctrl Pts',(-78.088258256583,5.48579627613764,4.24037338496465));
#32115=CARTESIAN_POINT('Ctrl Pts',(-78.0552289948441,4.78204391440569,5.15082200229657));
#32116=CARTESIAN_POINT('Ctrl Pts',(-78.0221997331052,3.84675171573669,5.88229653588832));
#32117=CARTESIAN_POINT('Ctrl Pts',(-77.9891704713663,2.79355165779576,6.34592754153627));
#32118=CARTESIAN_POINT('Ctrl Pts',(-77.9561412096274,1.74035159985484,6.80955854718422));
#32119=CARTESIAN_POINT('Ctrl Pts',(-77.9231119478886,0.56924368264199,7.00534602488837));
#32120=CARTESIAN_POINT('Ctrl Pts',(-77.8900826861497,-0.577490025328187,
6.9095030572284));
#32121=CARTESIAN_POINT('Ctrl Pts',(-77.8570534244108,-1.72422373329835,
6.81366008956843));
#32122=CARTESIAN_POINT('Ctrl Pts',(-77.8240241626719,-2.84658323202583,
6.42618667654436));
#32123=CARTESIAN_POINT('Ctrl Pts',(-77.790994900933,-3.80820907184011,5.79415834201627));
#32124=CARTESIAN_POINT('Ctrl Pts',(-77.7579656391941,-4.76983491165438,
5.16213000748818));
#32125=CARTESIAN_POINT('Ctrl Pts',(-77.7249363774552,-5.57072709255544,
4.28554675145607));
#32126=CARTESIAN_POINT('Ctrl Pts',(-77.6919071157163,-6.11358237332966,
3.27090779321506));
#32127=CARTESIAN_POINT('Ctrl Pts',(-77.6593286316797,-6.64902885829029,
2.27011645354264));
#32128=CARTESIAN_POINT('Ctrl Pts',(-77.626750147643,-6.93343366709735,1.13501201807639));
#32129=CARTESIAN_POINT('Ctrl Pts',(-77.5941716636063,-6.93359074487482,
-1.65665743479807E-5));
#32130=CARTESIAN_POINT('Origin',(-87.75,0.,0.));
#32131=CARTESIAN_POINT('',(-76.1648283363937,-6.93245908794419,-7.27747633805231E-5));
#32132=CARTESIAN_POINT('',(-76.3441716636063,-6.93250871142555,-0.000101958036885148));
#32133=CARTESIAN_POINT('',(-87.75,-6.933,-8.4904762584886E-16));
#32134=CARTESIAN_POINT('Ctrl Pts',(-76.1648283363937,-6.93245908794419,
-7.27747633805231E-5));
#32135=CARTESIAN_POINT('Ctrl Pts',(-76.1836598746737,-6.93221658934376,
0.656323270318536));
#32136=CARTESIAN_POINT('Ctrl Pts',(-76.2024914129537,-6.83971996360292,
1.31278624755817));
#32137=CARTESIAN_POINT('Ctrl Pts',(-76.2213229512337,-6.65590312778372,
1.94259644573592));
#32138=CARTESIAN_POINT('Ctrl Pts',(-76.2543522129726,-6.33350066166455,
3.04724151360787));
#32139=CARTESIAN_POINT('Ctrl Pts',(-76.2873814747115,-5.73017148093525,
4.06989511813717));
#32140=CARTESIAN_POINT('Ctrl Pts',(-76.3204107364504,-4.91921619484598,
4.8863114335654));
#32141=CARTESIAN_POINT('Ctrl Pts',(-76.3534399981892,-4.10826090875669,
5.70272774899365));
#32142=CARTESIAN_POINT('Ctrl Pts',(-76.3864692599281,-3.0896795173074,6.31290677532083));
#32143=CARTESIAN_POINT('Ctrl Pts',(-76.4194985216671,-1.98722309859757,
6.64271569117836));
#32144=CARTESIAN_POINT('Ctrl Pts',(-76.4525277834059,-0.884766679887746,
6.97252460703589));
#32145=CARTESIAN_POINT('Ctrl Pts',(-76.4855570451448,0.301564766082627,
7.02196341242377));
#32146=CARTESIAN_POINT('Ctrl Pts',(-76.5185863068837,1.42763961011382,6.78502561093626));
#32147=CARTESIAN_POINT('Ctrl Pts',(-76.5516155686226,2.55371445414502,6.54808780944875));
#32148=CARTESIAN_POINT('Ctrl Pts',(-76.5846448303615,3.61953269623705,6.02477340108585));
#32149=CARTESIAN_POINT('Ctrl Pts',(-76.6176740921004,4.49560428520284,5.27866171565225));
#32150=CARTESIAN_POINT('Ctrl Pts',(-76.6507033538393,5.37167587416864,4.53255003021866));
#32151=CARTESIAN_POINT('Ctrl Pts',(-76.6837326155782,6.05800081000821,3.56364106771436));
#32152=CARTESIAN_POINT('Ctrl Pts',(-76.7167618773171,6.47119503382389,2.48965102607572));
#32153=CARTESIAN_POINT('Ctrl Pts',(-76.7497911390559,6.88438925763956,1.41566098443711));
#32154=CARTESIAN_POINT('Ctrl Pts',(-76.7828204007948,7.02445276943136,0.236589863664146));
#32155=CARTESIAN_POINT('Ctrl Pts',(-76.8158496625337,6.874368754704,-0.904312789789189));
#32156=CARTESIAN_POINT('Ctrl Pts',(-76.8488789242726,6.72428473997664,-2.04521544324256));
#32157=CARTESIAN_POINT('Ctrl Pts',(-76.8819081860115,6.28405319873012,-3.1479496293763));
#32158=CARTESIAN_POINT('Ctrl Pts',(-76.9149374477504,5.60715942757398,-4.078540247588));
#32159=CARTESIAN_POINT('Ctrl Pts',(-76.9479667094893,4.93026565641784,-5.00913086579971));
#32160=CARTESIAN_POINT('Ctrl Pts',(-76.9809959712282,4.01670965535209,-5.76757791608937));
#32161=CARTESIAN_POINT('Ctrl Pts',(-77.014025232967,2.97748259404187,-6.26173496721194));
#32162=CARTESIAN_POINT('Ctrl Pts',(-77.0470544947059,1.93825553273165,-6.7558920183345));
#32163=CARTESIAN_POINT('Ctrl Pts',(-77.0800837564448,0.773357411176957,
-6.98575907028995));
#32164=CARTESIAN_POINT('Ctrl Pts',(-77.1131130181837,-0.375684152281078,
-6.92340875690233));
#32165=CARTESIAN_POINT('Ctrl Pts',(-77.1461422799226,-1.5247257157391,-6.8610584435147));
#32166=CARTESIAN_POINT('Ctrl Pts',(-77.1791715416615,-2.65791072110042,
-6.50649076478404));
#32167=CARTESIAN_POINT('Ctrl Pts',(-77.2122008034004,-3.63756448936863,
-5.90278340980857));
#32168=CARTESIAN_POINT('Ctrl Pts',(-77.2452300651393,-4.61721825763681,
-5.29907605483312));
#32169=CARTESIAN_POINT('Ctrl Pts',(-77.2782593268782,-5.44334078881188,
-4.44622902361285));
#32170=CARTESIAN_POINT('Ctrl Pts',(-77.3112885886171,-6.01556351663744,
-3.44785773701984));
#32171=CARTESIAN_POINT('Ctrl Pts',(-77.344317850356,-6.58778624446302,-2.44948645042679));
#32172=CARTESIAN_POINT('Ctrl Pts',(-77.3773471120949,-6.9061091689391,-1.30559090846094));
#32173=CARTESIAN_POINT('Ctrl Pts',(-77.4103763738337,-6.93185810514696,
-0.155147051326755));
#32174=CARTESIAN_POINT('Ctrl Pts',(-77.4118603613537,-6.93301499143427,
-0.103458208265699));
#32175=CARTESIAN_POINT('Ctrl Pts',(-77.4133443488737,-6.93358127087656,
-0.0517561463953276));
#32176=CARTESIAN_POINT('Ctrl Pts',(-77.4148283363937,-6.93355988365441,
-5.3614765520571E-5));
#32177=CARTESIAN_POINT('Ctrl Pts',(-77.5941716636063,-6.93359074487482,
-1.65665743479807E-5));
#32178=CARTESIAN_POINT('Ctrl Pts',(-77.5937208859041,-6.93359291830805,
-0.0157215814777106));
#32179=CARTESIAN_POINT('Ctrl Pts',(-77.5932701082019,-6.93354067154366,
-0.0314265818591758));
#32180=CARTESIAN_POINT('Ctrl Pts',(-77.5928193304997,-6.93343391661625,
-0.047131211712011));
#32181=CARTESIAN_POINT('Ctrl Pts',(-77.5597900687608,-6.92561179848128,
-1.19783659794813));
#32182=CARTESIAN_POINT('Ctrl Pts',(-77.5267608070219,-6.62514918156395,
-2.34655270997042));
#32183=CARTESIAN_POINT('Ctrl Pts',(-77.493731545283,-6.06855033845775,-3.35371793936318));
#32184=CARTESIAN_POINT('Ctrl Pts',(-77.4607022835441,-5.51195149535157,
-4.3608831687559));
#32185=CARTESIAN_POINT('Ctrl Pts',(-77.4276730218052,-4.69921642605653,
-5.2264975155191));
#32186=CARTESIAN_POINT('Ctrl Pts',(-77.3946437600663,-3.72908720644287,
-5.84539441218008));
#32187=CARTESIAN_POINT('Ctrl Pts',(-77.3616144983274,-2.75895798682919,
-6.46429130884108));
#32188=CARTESIAN_POINT('Ctrl Pts',(-77.3285852365886,-1.63143461689687,
-6.83647075539986));
#32189=CARTESIAN_POINT('Ctrl Pts',(-77.2955559748497,-0.483503923405929,
-6.91671534640924));
#32190=CARTESIAN_POINT('Ctrl Pts',(-77.2625267131108,0.664426770085027,
-6.99695993741863));
#32191=CARTESIAN_POINT('Ctrl Pts',(-77.2294974513719,1.83276478713461,-6.78526967287862));
#32192=CARTESIAN_POINT('Ctrl Pts',(-77.196468189633,2.87956458425637,-6.30736355637587));
#32193=CARTESIAN_POINT('Ctrl Pts',(-77.1634389278941,3.92636438137815,-5.82945743987311));
#32194=CARTESIAN_POINT('Ctrl Pts',(-77.1304096661552,4.85162595857206,-5.08533547140764));
#32195=CARTESIAN_POINT('Ctrl Pts',(-77.0973804044163,5.54293599407229,-4.1654036770546));
#32196=CARTESIAN_POINT('Ctrl Pts',(-77.0643511426775,6.23424602957248,-3.24547188270159));
#32197=CARTESIAN_POINT('Ctrl Pts',(-77.0313218809385,6.69160452337899,-2.14973026246101));
#32198=CARTESIAN_POINT('Ctrl Pts',(-76.9982926191996,6.85944536446558,-1.01130436522037));
#32199=CARTESIAN_POINT('Ctrl Pts',(-76.9652633574607,7.02728620555217,0.127121532020305));
#32200=CARTESIAN_POINT('Ctrl Pts',(-76.9322340957219,6.90560939391885,1.30823170626106));
#32201=CARTESIAN_POINT('Ctrl Pts',(-76.899204833983,6.5091978784254,2.38852887918575));
#32202=CARTESIAN_POINT('Ctrl Pts',(-76.8661755722441,6.11278636293196,3.46882605211044));
#32203=CARTESIAN_POINT('Ctrl Pts',(-76.8331463105052,5.44164014357837,4.44831022371903));
#32204=CARTESIAN_POINT('Ctrl Pts',(-76.8001170487663,4.57729916297956,5.20798037628682));
#32205=CARTESIAN_POINT('Ctrl Pts',(-76.7670877870274,3.71295818238075,5.96765052885462));
#32206=CARTESIAN_POINT('Ctrl Pts',(-76.7340585252885,2.65542244053669,6.50750666238162));
#32207=CARTESIAN_POINT('Ctrl Pts',(-76.7010292635496,1.53317571820417,6.76195973400546));
#32208=CARTESIAN_POINT('Ctrl Pts',(-76.6680000018108,0.410928995871668,
7.0164128056293));
#32209=CARTESIAN_POINT('Ctrl Pts',(-76.6349707400718,-0.77602870694931,
6.98546281535));
#32210=CARTESIAN_POINT('Ctrl Pts',(-76.601941478333,-1.88348967488557,6.67286998762912));
#32211=CARTESIAN_POINT('Ctrl Pts',(-76.5689122165941,-2.99095064282184,
6.36027715990825));
#32212=CARTESIAN_POINT('Ctrl Pts',(-76.5358829548552,-4.0189148758734,5.76604149474581));
#32213=CARTESIAN_POINT('Ctrl Pts',(-76.5028536931163,-4.84249134112358,
4.9623587978244));
#32214=CARTESIAN_POINT('Ctrl Pts',(-76.4698244313774,-5.66606780637378,
4.15867610090298));
#32215=CARTESIAN_POINT('Ctrl Pts',(-76.4367951696385,-6.2852565038226,3.14554637222259));
#32216=CARTESIAN_POINT('Ctrl Pts',(-76.4037659078996,-6.62482999509395,
2.0460583479719));
#32217=CARTESIAN_POINT('Ctrl Pts',(-76.3839011598018,-6.82905926058937,
1.3847946233713));
#32218=CARTESIAN_POINT('Ctrl Pts',(-76.364036411704,-6.93214707574568,0.692293673219922));
#32219=CARTESIAN_POINT('Ctrl Pts',(-76.3441716636063,-6.93250871142555,
-0.000101958036885148));
#32220=CARTESIAN_POINT('Origin',(-87.75,0.,0.));
#32221=CARTESIAN_POINT('',(-74.9148283363937,-6.93316696520231,0.00016807782604461));
#32222=CARTESIAN_POINT('',(-75.0941716636063,-6.93305363032429,0.000176774812155918));
#32223=CARTESIAN_POINT('',(-87.75,-6.933,-8.4904762584886E-16));
#32224=CARTESIAN_POINT('Ctrl Pts',(-74.9148283363937,-6.93316696520231,
0.00016807782604461));
#32225=CARTESIAN_POINT('Ctrl Pts',(-74.9209461387348,-6.93338316350285,
0.213348952983918));
#32226=CARTESIAN_POINT('Ctrl Pts',(-74.9270639410759,-6.92374509836824,
0.426510353887417));
#32227=CARTESIAN_POINT('Ctrl Pts',(-74.933181743417,-6.90410963765511,0.63874682673552));
#32228=CARTESIAN_POINT('Ctrl Pts',(-74.9662110051559,-6.7981002023875,1.78458541736159));
#32229=CARTESIAN_POINT('Ctrl Pts',(-74.9992402668948,-6.40068796263517,
2.90346432362064));
#32230=CARTESIAN_POINT('Ctrl Pts',(-75.0322695286337,-5.76015594568697,
3.8594469654076));
#32231=CARTESIAN_POINT('Ctrl Pts',(-75.0652987903726,-5.11962392873879,
4.81542960719453));
#32232=CARTESIAN_POINT('Ctrl Pts',(-75.0983280521114,-4.23597213459477,
5.60851598450938));
#32233=CARTESIAN_POINT('Ctrl Pts',(-75.1313573138503,-3.21655856440023,
6.1423512109949));
#32234=CARTESIAN_POINT('Ctrl Pts',(-75.1643865755892,-2.19714499420567,
6.67618643748043));
#32235=CARTESIAN_POINT('Ctrl Pts',(-75.1974158373281,-1.04196964796058,
6.95077051313662));
#32236=CARTESIAN_POINT('Ctrl Pts',(-75.230445099067,0.108621110566956,6.93274324144246));
#32237=CARTESIAN_POINT('Ctrl Pts',(-75.2634743608059,1.25921186909442,6.9147159697483));
#32238=CARTESIAN_POINT('Ctrl Pts',(-75.2965036225447,2.40521803990433,6.60407735070382));
#32239=CARTESIAN_POINT('Ctrl Pts',(-75.3295328842836,3.40740725498283,6.03856797561452));
#32240=CARTESIAN_POINT('Ctrl Pts',(-75.3625621460225,4.40959647006133,5.47305860052522));
#32241=CARTESIAN_POINT('Ctrl Pts',(-75.3955914077615,5.26796872940841,4.65267846939111));
#32242=CARTESIAN_POINT('Ctrl Pts',(-75.4286206695004,5.87823733252418,3.6770984838519));
#32243=CARTESIAN_POINT('Ctrl Pts',(-75.4616499312393,6.48850593563994,2.7015184983127));
#32244=CARTESIAN_POINT('Ctrl Pts',(-75.4946791929781,6.85067088252439,1.57073865836841));
#32245=CARTESIAN_POINT('Ctrl Pts',(-75.527708454717,6.92073146493465,0.422141430909675));
#32246=CARTESIAN_POINT('Ctrl Pts',(-75.5607377164559,6.9907920473449,-0.726455796549087));
#32247=CARTESIAN_POINT('Ctrl Pts',(-75.5937669781948,6.76874826528096,-1.89287041152229));
#32248=CARTESIAN_POINT('Ctrl Pts',(-75.6267962399337,6.28157700801878,-2.9353905514866));
#32249=CARTESIAN_POINT('Ctrl Pts',(-75.6598255016726,5.7944057507566,-3.97791069145091));
#32250=CARTESIAN_POINT('Ctrl Pts',(-75.6928547634115,5.04210701829618,-4.89653635640633));
#32251=CARTESIAN_POINT('Ctrl Pts',(-75.7258840251504,4.11608026086934,-5.57966044518022));
#32252=CARTESIAN_POINT('Ctrl Pts',(-75.7589132868893,3.1900535034425,-6.2627845339541));
#32253=CARTESIAN_POINT('Ctrl Pts',(-75.7919425486281,2.09029872104924,-6.71040704654646));
#32254=CARTESIAN_POINT('Ctrl Pts',(-75.824971810367,0.950429035928664,-6.86814473093649));
#32255=CARTESIAN_POINT('Ctrl Pts',(-75.8580010721059,-0.189440649191916,
-7.02588241532651));
#32256=CARTESIAN_POINT('Ctrl Pts',(-75.8910303338448,-1.36942523703982,
-6.8937352715142));
#32257=CARTESIAN_POINT('Ctrl Pts',(-75.9240595955837,-2.44616420079535,
-6.48775832627682));
#32258=CARTESIAN_POINT('Ctrl Pts',(-75.9570888573226,-3.52290316455086,
-6.08178138103944));
#32259=CARTESIAN_POINT('Ctrl Pts',(-75.9901181190614,-4.496396504214,-5.40197463437701));
#32260=CARTESIAN_POINT('Ctrl Pts',(-76.0231473808003,-5.24837104955287,
-4.5309302271876));
#32261=CARTESIAN_POINT('Ctrl Pts',(-76.0561766425392,-6.00034559489176,
-3.65988581999817));
#32262=CARTESIAN_POINT('Ctrl Pts',(-76.0892059042781,-6.53080134590636,
-2.59760375228175));
#32263=CARTESIAN_POINT('Ctrl Pts',(-76.122235166017,-6.77529134565915,-1.47314445281622));
#32264=CARTESIAN_POINT('Ctrl Pts',(-76.1364328894759,-6.88038607748807,
-0.989792378500842));
#32265=CARTESIAN_POINT('Ctrl Pts',(-76.1506306129348,-6.93264191570988,
-0.494951599266496));
#32266=CARTESIAN_POINT('Ctrl Pts',(-76.1648283363937,-6.93245908794419,
-7.27747633805231E-5));
#32267=CARTESIAN_POINT('Ctrl Pts',(-76.3441716636063,-6.93250871142555,
-0.000101958036885148));
#32268=CARTESIAN_POINT('Ctrl Pts',(-76.3310071499652,-6.93274837003171,
-0.458957599591355));
#32269=CARTESIAN_POINT('Ctrl Pts',(-76.3178426363241,-6.88787264551702,
-0.917766987091575));
#32270=CARTESIAN_POINT('Ctrl Pts',(-76.304678122683,-6.79742030494444,-1.3674079219937));
#32271=CARTESIAN_POINT('Ctrl Pts',(-76.2716488609441,-6.57047883842969,
-2.49553984788754));
#32272=CARTESIAN_POINT('Ctrl Pts',(-76.2386195992052,-6.05663762030631,
-3.56595737985428));
#32273=CARTESIAN_POINT('Ctrl Pts',(-76.2055903374663,-5.31832504878431,
-4.44861168261239));
#32274=CARTESIAN_POINT('Ctrl Pts',(-76.1725610757274,-4.58001247726231,
-5.33126598537049));
#32275=CARTESIAN_POINT('Ctrl Pts',(-76.1395318139885,-3.61722855234165,
-6.02615705891999));
#32276=CARTESIAN_POINT('Ctrl Pts',(-76.1065025522496,-2.54694531934537,
-6.44886011380824));
#32277=CARTESIAN_POINT('Ctrl Pts',(-76.0734732905107,-1.47666208634905,
-6.8715631686965));
#32278=CARTESIAN_POINT('Ctrl Pts',(-76.0404440287718,-0.298879545277113,
-7.02207820492352));
#32279=CARTESIAN_POINT('Ctrl Pts',(-76.0074147670329,0.843309311550133,
-6.88211861509629));
#32280=CARTESIAN_POINT('Ctrl Pts',(-75.974385505294,1.98549816837733,-6.74215902526907));
#32281=CARTESIAN_POINT('Ctrl Pts',(-75.9413562435551,3.09209334095979,-6.31172480938761));
#32282=CARTESIAN_POINT('Ctrl Pts',(-75.9083269818163,4.02865064371125,-5.64311095213686));
#32283=CARTESIAN_POINT('Ctrl Pts',(-75.8752977200774,4.96520794646275,-4.97449709488609));
#32284=CARTESIAN_POINT('Ctrl Pts',(-75.8422684583385,5.73172737938323,-4.06770359626603));
#32285=CARTESIAN_POINT('Ctrl Pts',(-75.8092391965996,6.23508176873444,-3.03290002545378));
#32286=CARTESIAN_POINT('Ctrl Pts',(-75.7762099348607,6.73843615808564,-1.99809645464153));
#32287=CARTESIAN_POINT('Ctrl Pts',(-75.7431806731218,6.97862550386755,-0.835282811637106));
#32288=CARTESIAN_POINT('Ctrl Pts',(-75.7101514113829,6.92646834769301,0.314266535935534));
#32289=CARTESIAN_POINT('Ctrl Pts',(-75.677122149644,6.87431119151848,1.46381588350816));
#32290=CARTESIAN_POINT('Ctrl Pts',(-75.6440928879051,6.52980753338749,2.60010093564904));
#32291=CARTESIAN_POINT('Ctrl Pts',(-75.6110636261663,5.93481234872058,3.58507037764613));
#32292=CARTESIAN_POINT('Ctrl Pts',(-75.5780343644274,5.33981716405367,4.57003981964324));
#32293=CARTESIAN_POINT('Ctrl Pts',(-75.5450051026885,4.49433045285084,5.40369365149659));
#32294=CARTESIAN_POINT('Ctrl Pts',(-75.5119758409496,3.5010734045118,5.98474830242862));
#32295=CARTESIAN_POINT('Ctrl Pts',(-75.4789465792107,2.5078163561728,6.56580295336062));
#32296=CARTESIAN_POINT('Ctrl Pts',(-75.4459173174718,1.36678897069762,6.89425842337131));
#32297=CARTESIAN_POINT('Ctrl Pts',(-75.4128880557329,0.216618725751648,
6.930209488526));
#32298=CARTESIAN_POINT('Ctrl Pts',(-75.379858793994,-0.93355151919432,6.96616055368069));
#32299=CARTESIAN_POINT('Ctrl Pts',(-75.3468295322551,-2.09286462361106,
6.70960721397939));
#32300=CARTESIAN_POINT('Ctrl Pts',(-75.3138002705162,-3.1204715127651,6.19171904766548));
#32301=CARTESIAN_POINT('Ctrl Pts',(-75.2807710087774,-4.14807840191918,
5.67383088135156));
#32302=CARTESIAN_POINT('Ctrl Pts',(-75.2477417470385,-5.04397907581053,
4.89460788842503));
#32303=CARTESIAN_POINT('Ctrl Pts',(-75.2147124852996,-5.69932737330293,
3.94872064333779));
#32304=CARTESIAN_POINT('Ctrl Pts',(-75.1816832235607,-6.35467567079534,
3.00283339825053));
#32305=CARTESIAN_POINT('Ctrl Pts',(-75.1486539618218,-6.76947159188878,
1.89028190100257));
#32306=CARTESIAN_POINT('Ctrl Pts',(-75.1156247000829,-6.89332010398449,
0.746233992260691));
#32307=CARTESIAN_POINT('Ctrl Pts',(-75.108473687924,-6.92013397051462,0.498541489460373));
#32308=CARTESIAN_POINT('Ctrl Pts',(-75.1013226757651,-6.93330980226047,
0.249372605904462));
#32309=CARTESIAN_POINT('Ctrl Pts',(-75.0941716636063,-6.93305363032429,
0.000176774812155918));
#32310=CARTESIAN_POINT('Origin',(-87.75,0.,0.));
#32311=CARTESIAN_POINT('',(-73.6648283363937,-6.9331147324061,-0.00017295491683611));
#32312=CARTESIAN_POINT('',(-73.8441716636062,-6.9332265516286,-0.000160595751058418));
#32313=CARTESIAN_POINT('',(-87.75,-6.933,-8.4904762584886E-16));
#32314=CARTESIAN_POINT('Ctrl Pts',(-73.6648283363937,-6.9331147324061,-0.00017295491683611));
#32315=CARTESIAN_POINT('Ctrl Pts',(-73.6912616645348,-6.93217036533797,
0.920942522637482));
#32316=CARTESIAN_POINT('Ctrl Pts',(-73.7176949926758,-6.74746695301234,
1.84242538290147));
#32317=CARTESIAN_POINT('Ctrl Pts',(-73.7441283208169,-6.3900229396157,2.6911585290748));
#32318=CARTESIAN_POINT('Ctrl Pts',(-73.7771575825558,-5.94338558042776,
3.75167686720537));
#32319=CARTESIAN_POINT('Ctrl Pts',(-73.8101868442948,-5.22704355212943,
4.69860906840553));
#32320=CARTESIAN_POINT('Ctrl Pts',(-73.8432161060336,-4.32802779700381,
5.41690896967904));
#32321=CARTESIAN_POINT('Ctrl Pts',(-73.8762453677725,-3.42901204187819,
6.13520887095255));
#32322=CARTESIAN_POINT('Ctrl Pts',(-73.9092746295114,-2.34732255992529,
6.62487647229942));
#32323=CARTESIAN_POINT('Ctrl Pts',(-73.9423038912502,-1.21437765574423,
6.82642031423909));
#32324=CARTESIAN_POINT('Ctrl Pts',(-73.9753331529891,-0.0814327515631799,
7.02796415617876));
#32325=CARTESIAN_POINT('Ctrl Pts',(-74.0083624147281,1.10276757484602,6.94138423871124));
#32326=CARTESIAN_POINT('Ctrl Pts',(-74.041391676467,2.1943506115832,6.57719946412387));
#32327=CARTESIAN_POINT('Ctrl Pts',(-74.0744209382059,3.28593364832035,6.21301468953652));
#32328=CARTESIAN_POINT('Ctrl Pts',(-74.1074501999447,4.28489939538549,5.57122505782934));
#32329=CARTESIAN_POINT('Ctrl Pts',(-74.1404794616836,5.06987994912212,4.729803875312));
#32330=CARTESIAN_POINT('Ctrl Pts',(-74.1735087234225,5.85486050285878,3.88838269279463));
#32331=CARTESIAN_POINT('Ctrl Pts',(-74.2065379851614,6.42585586326691,2.8473299594671));
#32332=CARTESIAN_POINT('Ctrl Pts',(-74.2395672469003,6.71349377199439,1.73312687672298));
#32333=CARTESIAN_POINT('Ctrl Pts',(-74.2725965086392,7.00113168072186,0.61892379397887));
#32334=CARTESIAN_POINT('Ctrl Pts',(-74.3056257703781,7.00541213776869,-0.568429638181864));
#32335=CARTESIAN_POINT('Ctrl Pts',(-74.3386550321169,6.72581509517529,-1.68467762582019));
#32336=CARTESIAN_POINT('Ctrl Pts',(-74.3716842938559,6.44621805258187,-2.80092561345853));
#32337=CARTESIAN_POINT('Ctrl Pts',(-74.4047135555948,5.88274351034823,-3.84606815657449));
#32338=CARTESIAN_POINT('Ctrl Pts',(-74.4377428173337,5.10384999586191,-4.6931271682288));
#32339=CARTESIAN_POINT('Ctrl Pts',(-74.4707720790725,4.32495648137559,-5.54018617988311));
#32340=CARTESIAN_POINT('Ctrl Pts',(-74.5038013408114,3.33064399463661,-6.18916166007575));
#32341=CARTESIAN_POINT('Ctrl Pts',(-74.5368306025503,2.24171509814475,-6.56120726819209));
#32342=CARTESIAN_POINT('Ctrl Pts',(-74.5698598642892,1.15278620165293,-6.93325287630843));
#32343=CARTESIAN_POINT('Ctrl Pts',(-74.6028891260281,-0.0307591045917431,
-7.02836861234847));
#32344=CARTESIAN_POINT('Ctrl Pts',(-74.635918387767,-1.16512768941995,-6.83499852704987));
#32345=CARTESIAN_POINT('Ctrl Pts',(-74.6689476495059,-2.2994962742482,-6.64162844175125));
#32346=CARTESIAN_POINT('Ctrl Pts',(-74.7019769112448,-3.38468813765996,
-6.15977253511398));
#32347=CARTESIAN_POINT('Ctrl Pts',(-74.7350061729836,-4.28885945826866,
-5.44797319602862));
#32348=CARTESIAN_POINT('Ctrl Pts',(-74.7680354347225,-5.19303077887736,
-4.73617385694327));
#32349=CARTESIAN_POINT('Ctrl Pts',(-74.8010646964614,-5.91618155668299,
-3.79443108540985));
#32350=CARTESIAN_POINT('Ctrl Pts',(-74.8340939582003,-6.37045363019433,
-2.73716056214661));
#32351=CARTESIAN_POINT('Ctrl Pts',(-74.8610054175981,-6.74058374568103,
-1.87572160585925));
#32352=CARTESIAN_POINT('Ctrl Pts',(-74.8879168769959,-6.93221593549224,
-0.937588349456712));
#32353=CARTESIAN_POINT('Ctrl Pts',(-74.9148283363937,-6.93316696520231,
0.00016807782604461));
#32354=CARTESIAN_POINT('Ctrl Pts',(-75.0941716636063,-6.93305363032429,
0.000176774812155918));
#32355=CARTESIAN_POINT('Ctrl Pts',(-75.0682934140262,-6.93212658934707,
-0.90161891061375));
#32356=CARTESIAN_POINT('Ctrl Pts',(-75.0424151644463,-6.75529560991023,
-1.80376749780292));
#32357=CARTESIAN_POINT('Ctrl Pts',(-75.0165369148662,-6.41232485292237,
-2.63757790554064));
#32358=CARTESIAN_POINT('Ctrl Pts',(-74.9835076531273,-5.97457998666652,
-3.70179757436449));
#32359=CARTESIAN_POINT('Ctrl Pts',(-74.9504783913884,-5.2661891510568,-4.65469259177645));
#32360=CARTESIAN_POINT('Ctrl Pts',(-74.9174491296495,-4.37321726968046,
-5.38049235101869));
#32361=CARTESIAN_POINT('Ctrl Pts',(-74.8844198679106,-3.48024538830414,
-6.1062921102609));
#32362=CARTESIAN_POINT('Ctrl Pts',(-74.8513906061717,-2.40269246116121,
-6.60499661133342));
#32363=CARTESIAN_POINT('Ctrl Pts',(-74.8183613444329,-1.27147422808607,
-6.81601646964816));
#32364=CARTESIAN_POINT('Ctrl Pts',(-74.785332082694,-0.140255995010866,
-7.02703632796292));
#32365=CARTESIAN_POINT('Ctrl Pts',(-74.7523028209551,1.04462754399656,-6.95037154351987));
#32366=CARTESIAN_POINT('Ctrl Pts',(-74.7192735592162,2.13922067110611,-6.59533639380998));
#32367=CARTESIAN_POINT('Ctrl Pts',(-74.6862442974773,3.23381379821559,-6.24030124410011));
#32368=CARTESIAN_POINT('Ctrl Pts',(-74.6532150357384,4.2381165134272,-5.60689572912343));
#32369=CARTESIAN_POINT('Ctrl Pts',(-74.6201857739995,5.03011250583151,-4.77207453901125));
#32370=CARTESIAN_POINT('Ctrl Pts',(-74.5871565122606,5.82210849823583,-3.93725334889907));
#32371=CARTESIAN_POINT('Ctrl Pts',(-74.5541272505218,6.40179776783287,-2.90101648365138));
#32372=CARTESIAN_POINT('Ctrl Pts',(-74.5210979887829,6.69875180230388,-1.7892600477104));
#32373=CARTESIAN_POINT('Ctrl Pts',(-74.488068727044,6.9957058367749,-0.677503611769395));
#32374=CARTESIAN_POINT('Ctrl Pts',(-74.4550394653051,7.0099246361199,0.509772394864872));
#32375=CARTESIAN_POINT('Ctrl Pts',(-74.4220102035662,6.73968070780564,1.62832158495628));
#32376=CARTESIAN_POINT('Ctrl Pts',(-74.3889809418273,6.46943677949138,2.74687077504773));
#32377=CARTESIAN_POINT('Ctrl Pts',(-74.3559516800884,5.91473012351782,3.79669314859627));
#32378=CARTESIAN_POINT('Ctrl Pts',(-74.3229224183495,5.14295402556832,4.65024204940911));
#32379=CARTESIAN_POINT('Ctrl Pts',(-74.2898931566106,4.37117792761887,5.50379095022191));
#32380=CARTESIAN_POINT('Ctrl Pts',(-74.2568638948718,3.38233238769347,6.16106637829903));
#32381=CARTESIAN_POINT('Ctrl Pts',(-74.2238346331329,2.29655576946821,6.54221360282011));
#32382=CARTESIAN_POINT('Ctrl Pts',(-74.190805371394,1.21077915124288,6.92336082734121));
#32383=CARTESIAN_POINT('Ctrl Pts',(-74.1577761096551,0.0280714547176494,
7.02837984830623));
#32384=CARTESIAN_POINT('Ctrl Pts',(-74.1247468479162,-1.10787595312376,
6.8445115311242));
#32385=CARTESIAN_POINT('Ctrl Pts',(-74.0917175861773,-2.24382336096507,
6.66064321394219));
#32386=CARTESIAN_POINT('Ctrl Pts',(-74.0586883244384,-3.33301048012259,
6.18788755861318));
#32387=CARTESIAN_POINT('Ctrl Pts',(-74.0256590626995,-4.24310809137114,
5.48368133211101));
#32388=CARTESIAN_POINT('Ctrl Pts',(-73.9926298009606,-5.15320570261977,
4.77947510560879));
#32389=CARTESIAN_POINT('Ctrl Pts',(-73.9596005392217,-5.88421380595942,
3.84381830793336));
#32390=CARTESIAN_POINT('Ctrl Pts',(-73.9265712774829,-6.34731962545765,
2.79038721318067));
#32391=CARTESIAN_POINT('Ctrl Pts',(-73.899104739524,-6.7324300669436,1.91437292682431));
#32392=CARTESIAN_POINT('Ctrl Pts',(-73.8716382015651,-6.93227843232692,
0.956914352367065));
#32393=CARTESIAN_POINT('Ctrl Pts',(-73.8441716636062,-6.9332265516286,-0.000160595751058418));
#32394=CARTESIAN_POINT('Origin',(-87.75,0.,0.));
#32395=CARTESIAN_POINT('',(-72.4148283363937,-6.93247994518944,8.66496906495873E-5));
#32396=CARTESIAN_POINT('',(-72.5941716636063,-6.93243957992525,5.60106990600447E-5));
#32397=CARTESIAN_POINT('',(-87.75,-6.933,-8.4904762584886E-16));
#32398=CARTESIAN_POINT('Ctrl Pts',(-72.4148283363937,-6.93247994518944,
8.66496906495873E-5));
#32399=CARTESIAN_POINT('Ctrl Pts',(-72.4285479285959,-6.93269109193388,
0.478295513083371));
#32400=CARTESIAN_POINT('Ctrl Pts',(-72.442267520798,-6.88392184964319,0.956461913326707));
#32401=CARTESIAN_POINT('Ctrl Pts',(-72.4559871130002,-6.78573659267738,
1.42425639974906));
#32402=CARTESIAN_POINT('Ctrl Pts',(-72.4890163747391,-6.54936028473497,
2.55044924166249));
#32403=CARTESIAN_POINT('Ctrl Pts',(-72.522045636478,-6.02657736140281,3.61652827731066));
#32404=CARTESIAN_POINT('Ctrl Pts',(-72.5550748982169,-5.2809025804778,4.4929717707693));
#32405=CARTESIAN_POINT('Ctrl Pts',(-72.5881041599558,-4.53522779955277,
5.36941526422797));
#32406=CARTESIAN_POINT('Ctrl Pts',(-72.6211334216947,-3.56666116103487,
6.05622321549709));
#32407=CARTESIAN_POINT('Ctrl Pts',(-72.6541626834336,-2.49287727270111,
6.46995288241554));
#32408=CARTESIAN_POINT('Ctrl Pts',(-72.6871919451724,-1.41909338436735,
6.88368254933399));
#32409=CARTESIAN_POINT('Ctrl Pts',(-72.7202212069113,-0.240092246217731,
7.02433393190177));
#32410=CARTESIAN_POINT('Ctrl Pts',(-72.7532504686502,0.900885097731738,
6.87481879311097));
#32411=CARTESIAN_POINT('Ctrl Pts',(-72.7862797303891,2.04186244168121,6.72530365432016));
#32412=CARTESIAN_POINT('Ctrl Pts',(-72.819308992128,3.14481599143052,6.28562199417078));
#32413=CARTESIAN_POINT('Ctrl Pts',(-72.8523382538669,4.07574399511096,5.60919230226098));
#32414=CARTESIAN_POINT('Ctrl Pts',(-72.8853675156058,5.0066719987914,4.93276261035119));
#32415=CARTESIAN_POINT('Ctrl Pts',(-72.9183967773447,5.76557445640296,4.019584886681));
#32416=CARTESIAN_POINT('Ctrl Pts',(-72.9514260390835,6.26024960764436,2.98060434264857));
#32417=CARTESIAN_POINT('Ctrl Pts',(-72.9844553008224,6.75492475888575,1.94162379861618));
#32418=CARTESIAN_POINT('Ctrl Pts',(-73.0174845625613,6.98537260375701,0.77684043422156));
#32419=CARTESIAN_POINT('Ctrl Pts',(-73.0505138243002,6.92359521348393,-0.37223207444993));
#32420=CARTESIAN_POINT('Ctrl Pts',(-73.0835430860391,6.86181782321086,-1.52130458312149));
#32421=CARTESIAN_POINT('Ctrl Pts',(-73.116572347778,6.50781519779342,-2.65466623606991));
#32422=CARTESIAN_POINT('Ctrl Pts',(-73.1496016095169,5.90459637599201,-3.6346208927547));
#32423=CARTESIAN_POINT('Ctrl Pts',(-73.1826308712558,5.30137755419063,-4.61457554943943));
#32424=CARTESIAN_POINT('Ctrl Pts',(-73.2156601329947,4.44894253600529,-5.44112320986056));
#32425=CARTESIAN_POINT('Ctrl Pts',(-73.2486893947336,3.45085668537816,-6.0138436572967));
#32426=CARTESIAN_POINT('Ctrl Pts',(-73.2817186564725,2.45277083475103,-6.58656410473285));
#32427=CARTESIAN_POINT('Ctrl Pts',(-73.3147479182114,1.3090341516821,-6.90545733918401));
#32428=CARTESIAN_POINT('Ctrl Pts',(-73.3477771799502,0.158603276043082,
-6.93177988674304));
#32429=CARTESIAN_POINT('Ctrl Pts',(-73.3808064416891,-0.991827599595997,
-6.95810243430206));
#32430=CARTESIAN_POINT('Ctrl Pts',(-73.413835703428,-2.14895266780516,-6.6918542949689));
#32431=CARTESIAN_POINT('Ctrl Pts',(-73.446864965167,-3.17218868615638,-6.16538290269537));
#32432=CARTESIAN_POINT('Ctrl Pts',(-73.4798942269059,-4.19542470450755,
-5.63891151042187));
#32433=CARTESIAN_POINT('Ctrl Pts',(-73.5129234886447,-5.08477167300079,
-4.85221686520803));
#32434=CARTESIAN_POINT('Ctrl Pts',(-73.5459527503836,-5.73217966349153,
-3.9008772991317));
#32435=CARTESIAN_POINT('Ctrl Pts',(-73.5789820121225,-6.37958765398229,
-2.94953773305535));
#32436=CARTESIAN_POINT('Ctrl Pts',(-73.6120112738614,-6.78505666647053,
-1.83355324611651));
#32437=CARTESIAN_POINT('Ctrl Pts',(-73.6450405356003,-6.89932482767586,
-0.688508765116595));
#32438=CARTESIAN_POINT('Ctrl Pts',(-73.6516364691981,-6.92214414497133,
-0.459843727946572));
#32439=CARTESIAN_POINT('Ctrl Pts',(-73.6582324027959,-6.93335038122188,
-0.230019779101979));
#32440=CARTESIAN_POINT('Ctrl Pts',(-73.6648283363937,-6.9331147324061,-0.00017295491683611));
#32441=CARTESIAN_POINT('Ctrl Pts',(-73.8441716636062,-6.9332265516286,-0.000160595751058418));
#32442=CARTESIAN_POINT('Ctrl Pts',(-73.8386089398262,-6.93341857167108,
-0.19399440113044));
#32443=CARTESIAN_POINT('Ctrl Pts',(-73.8330462160462,-6.92545223918872,
-0.387812471190364));
#32444=CARTESIAN_POINT('Ctrl Pts',(-73.8274834922662,-6.90921426020527,
-0.580935051256329));
#32445=CARTESIAN_POINT('Ctrl Pts',(-73.7944542305273,-6.81279953979783,
-1.72762082911074));
#32446=CARTESIAN_POINT('Ctrl Pts',(-73.7614249687884,-6.42476656332614,
-2.84978699298969));
#32447=CARTESIAN_POINT('Ctrl Pts',(-73.7283957070495,-5.79225883800486,
-3.81109758216143));
#32448=CARTESIAN_POINT('Ctrl Pts',(-73.6953664453106,-5.15975111268355,
-4.77240817133319));
#32449=CARTESIAN_POINT('Ctrl Pts',(-73.6623371835717,-4.28276863851263,
-5.57286318579773));
#32450=CARTESIAN_POINT('Ctrl Pts',(-73.6293079218328,-3.26785913721962,
-6.11521249724753));
#32451=CARTESIAN_POINT('Ctrl Pts',(-73.5962786600939,-2.25294963592661,
-6.65756180869732));
#32452=CARTESIAN_POINT('Ctrl Pts',(-73.5632493983551,-1.1001131075115,-6.94180541713237));
#32453=CARTESIAN_POINT('Ctrl Pts',(-73.5302201366162,0.050588235559008,
-6.93340955501874));
#32454=CARTESIAN_POINT('Ctrl Pts',(-73.4971908748773,1.20128957862948,-6.9250136929051));
#32455=CARTESIAN_POINT('Ctrl Pts',(-73.4641616131384,2.34985573635535,-6.62397836024279));
#32456=CARTESIAN_POINT('Ctrl Pts',(-73.4311323513995,3.35674331880206,-6.06687741089926));
#32457=CARTESIAN_POINT('Ctrl Pts',(-73.3981030896606,4.36363090124879,-5.50977646155573));
#32458=CARTESIAN_POINT('Ctrl Pts',(-73.3650738279217,5.22883990841635,-4.69660989553097));
#32459=CARTESIAN_POINT('Ctrl Pts',(-73.3320445661828,5.847253018982,-3.72617221276849));
#32460=CARTESIAN_POINT('Ctrl Pts',(-73.299015304444,6.46566612954764,-2.755734530006));
#32461=CARTESIAN_POINT('Ctrl Pts',(-73.265986042705,6.83728334351137,-1.62802573050579));
#32462=CARTESIAN_POINT('Ctrl Pts',(-73.2329567809661,6.91695556306483,-0.480055169525972));
#32463=CARTESIAN_POINT('Ctrl Pts',(-73.1999275192272,6.99662778261828,0.667915391453817));
#32464=CARTESIAN_POINT('Ctrl Pts',(-73.1668982574884,6.78435500776147,1.83614771391322));
#32465=CARTESIAN_POINT('Ctrl Pts',(-73.1338689957495,6.30592701333244,2.88270909557768));
#32466=CARTESIAN_POINT('Ctrl Pts',(-73.1008397340106,5.8274990189034,3.92927047724217));
#32467=CARTESIAN_POINT('Ctrl Pts',(-73.0678104722717,5.08291580490211,4.85416091811173));
#32468=CARTESIAN_POINT('Ctrl Pts',(-73.0347812105328,4.16263943576538,5.54501218709328));
#32469=CARTESIAN_POINT('Ctrl Pts',(-73.0017519487939,3.24236306662865,6.23586345607482));
#32470=CARTESIAN_POINT('Ctrl Pts',(-72.968722687055,2.14639354235647,6.69267555316836));
#32471=CARTESIAN_POINT('Ctrl Pts',(-72.9356934253161,1.00788410070812,6.85994875102882));
#32472=CARTESIAN_POINT('Ctrl Pts',(-72.9026641635773,-0.130625340940225,
7.02722194888928));
#32473=CARTESIAN_POINT('Ctrl Pts',(-72.8696349018384,-1.31167469996475,
6.90495624751666));
#32474=CARTESIAN_POINT('Ctrl Pts',(-72.8366056400995,-2.39177408670627,
6.50800614208088));
#32475=CARTESIAN_POINT('Ctrl Pts',(-72.8035763783606,-3.4718734734478,6.1110560366451));
#32476=CARTESIAN_POINT('Ctrl Pts',(-72.7705471166217,-4.45102288790632,
5.43942152714615));
#32477=CARTESIAN_POINT('Ctrl Pts',(-72.7375178548828,-5.21026198319463,
4.57470188030638));
#32478=CARTESIAN_POINT('Ctrl Pts',(-72.7044885931439,-5.96950107848292,
3.70998223346664));
#32479=CARTESIAN_POINT('Ctrl Pts',(-72.671459331405,-6.508829854601,2.65217744928609));
#32480=CARTESIAN_POINT('Ctrl Pts',(-72.6384300696661,-6.76272333921484,
1.5298039954324));
#32481=CARTESIAN_POINT('Ctrl Pts',(-72.6236772676462,-6.87612703386224,
1.02848630059374));
#32482=CARTESIAN_POINT('Ctrl Pts',(-72.6089244656262,-6.93258528704124,
0.514286907138951));
#32483=CARTESIAN_POINT('Ctrl Pts',(-72.5941716636063,-6.93243957992525,
5.60106990600447E-5));
#32484=CARTESIAN_POINT('Origin',(-87.75,0.,0.));
#32485=CARTESIAN_POINT('',(-71.1648283363937,-6.93357792730774,3.67079550465076E-5));
#32486=CARTESIAN_POINT('',(-71.3441716636063,-6.93353164992697,7.2489118278869E-5));
#32487=CARTESIAN_POINT('',(-87.75,-6.933,-8.4904762584886E-16));
#32488=CARTESIAN_POINT('Ctrl Pts',(-71.1648283363937,-6.93357792730774,
3.67079550465076E-5));
#32489=CARTESIAN_POINT('Ctrl Pts',(-71.165834192657,-6.93358820915741,0.0350807501651851));
#32490=CARTESIAN_POINT('Ctrl Pts',(-71.1668400489202,-6.93332806093716,
0.0701246392026087));
#32491=CARTESIAN_POINT('Ctrl Pts',(-71.1678459051835,-6.93279653847796,
0.105164411732063));
#32492=CARTESIAN_POINT('Ctrl Pts',(-71.2008751669224,-6.91534295682192,
1.25576401568685));
#32493=CARTESIAN_POINT('Ctrl Pts',(-71.2339044286613,-6.60527577829948,
2.40192492933702));
#32494=CARTESIAN_POINT('Ctrl Pts',(-71.2669336904002,-6.04026616787353,
3.40439598441036));
#32495=CARTESIAN_POINT('Ctrl Pts',(-71.2999629521391,-5.47525655744756,
4.40686703948373));
#32496=CARTESIAN_POINT('Ctrl Pts',(-71.332992213878,-4.65530451511805,5.26564823598026));
#32497=CARTESIAN_POINT('Ctrl Pts',(-71.3660214756168,-3.68002893249243,
5.87640319017046));
#32498=CARTESIAN_POINT('Ctrl Pts',(-71.3990507373557,-2.70475334986681,
6.48715814436066));
#32499=CARTESIAN_POINT('Ctrl Pts',(-71.4320799990946,-1.57415422694506,
6.84988685624452));
#32500=CARTESIAN_POINT('Ctrl Pts',(-71.4651092608335,-0.425592074663672,
6.92052012376312));
#32501=CARTESIAN_POINT('Ctrl Pts',(-71.4981385225724,0.722970077617721,
6.99115339128172));
#32502=CARTESIAN_POINT('Ctrl Pts',(-71.5311677843113,1.88949525925877,6.76969121443506));
#32503=CARTESIAN_POINT('Ctrl Pts',(-71.5641970460502,2.93225817459818,6.28303982121147));
#32504=CARTESIAN_POINT('Ctrl Pts',(-71.5972263077891,3.97502108993757,5.7963884279879));
#32505=CARTESIAN_POINT('Ctrl Pts',(-71.630255569528,4.89402173897534,5.04454781838742));
#32506=CARTESIAN_POINT('Ctrl Pts',(-71.6632848312669,5.57760746238822,4.11886178366526));
#32507=CARTESIAN_POINT('Ctrl Pts',(-71.6963140930058,6.26119318580114,3.19317574894305));
#32508=CARTESIAN_POINT('Ctrl Pts',(-71.7293433547446,6.70936398358914,2.09364428909914));
#32509=CARTESIAN_POINT('Ctrl Pts',(-71.7623726164835,6.86766999061181,0.953853394121363));
#32510=CARTESIAN_POINT('Ctrl Pts',(-71.7954018782224,7.02597599763448,-0.185937500856344));
#32511=CARTESIAN_POINT('Ctrl Pts',(-71.8284311399613,6.89441721389184,-1.36598783096791));
#32512=CARTESIAN_POINT('Ctrl Pts',(-71.8614604017002,6.48897718420248,-2.44292908213207));
#32513=CARTESIAN_POINT('Ctrl Pts',(-71.8944896634391,6.08353715451311,-3.51987033329624));
#32514=CARTESIAN_POINT('Ctrl Pts',(-71.9275189251779,5.40421587887703,-4.493702505513));
#32515=CARTESIAN_POINT('Ctrl Pts',(-71.9605481869168,4.53354651658966,-5.2461112625777));
#32516=CARTESIAN_POINT('Ctrl Pts',(-71.9935774486557,3.66287715430227,-5.99852001964243));
#32517=CARTESIAN_POINT('Ctrl Pts',(-72.0266067103947,2.60085970536358,-6.52950536155508));
#32518=CARTESIAN_POINT('Ctrl Pts',(-72.0596359721336,1.47652244907446,-6.77455598949526));
#32519=CARTESIAN_POINT('Ctrl Pts',(-72.0926652338725,0.352185192785344,
-7.01960661743543));
#32520=CARTESIAN_POINT('Ctrl Pts',(-72.1256944956113,-0.834471870854206,
-6.97872253140312));
#32521=CARTESIAN_POINT('Ctrl Pts',(-72.1587237573502,-1.93927755219505,
-6.65687088450567));
#32522=CARTESIAN_POINT('Ctrl Pts',(-72.1917530190891,-3.04408323353587,
-6.33501923760822));
#32523=CARTESIAN_POINT('Ctrl Pts',(-72.224782280828,-4.06703753257799,-5.73220002984564));
#32524=CARTESIAN_POINT('Ctrl Pts',(-72.2578115425669,-4.88385809111654,
-4.9216519120375));
#32525=CARTESIAN_POINT('Ctrl Pts',(-72.2908408043058,-5.70067864965511,
-4.11110379422934));
#32526=CARTESIAN_POINT('Ctrl Pts',(-72.3238700660447,-6.31136546769011,
-3.09282676637561));
#32527=CARTESIAN_POINT('Ctrl Pts',(-72.3568993277835,-6.64172403043128,
-1.99053492835938));
#32528=CARTESIAN_POINT('Ctrl Pts',(-72.3762089973202,-6.83485927897507,
-1.34610965196703));
#32529=CARTESIAN_POINT('Ctrl Pts',(-72.395518666857,-6.93218276625011,-0.672969443054267));
#32530=CARTESIAN_POINT('Ctrl Pts',(-72.4148283363937,-6.93247994518944,
8.66496906495873E-5));
#32531=CARTESIAN_POINT('Ctrl Pts',(-72.5941716636063,-6.93243957992525,
5.60106990600447E-5));
#32532=CARTESIAN_POINT('Ctrl Pts',(-72.5758952038873,-6.93225907114917,
-0.636997225174157));
#32533=CARTESIAN_POINT('Ctrl Pts',(-72.5576187441684,-6.84520613908146,
-1.27409880997282));
#32534=CARTESIAN_POINT('Ctrl Pts',(-72.5393422844495,-6.67193004491143,
-1.8868165525589));
#32535=CARTESIAN_POINT('Ctrl Pts',(-72.5063130227106,-6.35878507288456,
-2.99412152316961));
#32536=CARTESIAN_POINT('Ctrl Pts',(-72.4732837609717,-5.76403693572121,
-4.02178934086416));
#32537=CARTESIAN_POINT('Ctrl Pts',(-72.4402544992328,-4.95994370115113,
-4.84496498528249));
#32538=CARTESIAN_POINT('Ctrl Pts',(-72.4072252374939,-4.15585046658107,
-5.66814062970079));
#32539=CARTESIAN_POINT('Ctrl Pts',(-72.374195975755,-3.14241213460429,-6.28682410084286));
#32540=CARTESIAN_POINT('Ctrl Pts',(-72.3411667140161,-2.04275493472216,
-6.62584934207459));
#32541=CARTESIAN_POINT('Ctrl Pts',(-72.3081374522772,-0.94309773484001,
-6.96487458330633));
#32542=CARTESIAN_POINT('Ctrl Pts',(-72.2751081905383,0.24277833294748,-7.02424159462772));
#32543=CARTESIAN_POINT('Ctrl Pts',(-72.2420789287995,1.37079696495661,-6.79673766656238));
#32544=CARTESIAN_POINT('Ctrl Pts',(-72.2090496670606,2.49881559696574,-6.56923373849704));
#32545=CARTESIAN_POINT('Ctrl Pts',(-72.1760204053217,3.56897679319648,-6.05485887104497));
#32546=CARTESIAN_POINT('Ctrl Pts',(-72.1429911435828,4.45126286150812,-5.31610629737223));
#32547=CARTESIAN_POINT('Ctrl Pts',(-72.1099618818439,5.33354892981976,-4.57735372369949));
#32548=CARTESIAN_POINT('Ctrl Pts',(-72.076932620105,6.02795987021227,-3.61422344380608));
#32549=CARTESIAN_POINT('Ctrl Pts',(-72.0439033583661,6.45012922631898,-2.5437295829132));
#32550=CARTESIAN_POINT('Ctrl Pts',(-72.0108740966272,6.87229858242569,-1.47323572202035));
#32551=CARTESIAN_POINT('Ctrl Pts',(-71.9778448348883,7.02222635424661,-0.295378280127947));
#32552=CARTESIAN_POINT('Ctrl Pts',(-71.9448155731494,6.88169728323131,0.846740650476222));
#32553=CARTESIAN_POINT('Ctrl Pts',(-71.9117863114105,6.74116821221601,1.98885958108042));
#32554=CARTESIAN_POINT('Ctrl Pts',(-71.8787570496716,6.31018229836454,3.09524000039637));
#32555=CARTESIAN_POINT('Ctrl Pts',(-71.8457277879328,5.64110155411151,4.0314638139766));
#32556=CARTESIAN_POINT('Ctrl Pts',(-71.8126985261939,4.9720208098585,4.96768762755681));
#32557=CARTESIAN_POINT('Ctrl Pts',(-71.779669264455,4.06484523520388,5.73375483540125));
#32558=CARTESIAN_POINT('Ctrl Pts',(-71.7466400027161,3.02979081910206,6.23659320620537));
#32559=CARTESIAN_POINT('Ctrl Pts',(-71.7136107409772,1.9947364030002,6.7394315770095));
#32560=CARTESIAN_POINT('Ctrl Pts',(-71.6805814792383,0.831803145451077,
6.97904111077336));
#32561=CARTESIAN_POINT('Ctrl Pts',(-71.6475522174994,-0.31772005352466,
6.92631079253525));
#32562=CARTESIAN_POINT('Ctrl Pts',(-71.6145229557605,-1.46724325250037,
6.87358047429715));
#32563=CARTESIAN_POINT('Ctrl Pts',(-71.5814936940217,-2.60335639290266,
6.5285103040571));
#32564=CARTESIAN_POINT('Ctrl Pts',(-71.5484644322828,-3.58802904618852,
5.93302408480781));
#32565=CARTESIAN_POINT('Ctrl Pts',(-71.5154351705439,-4.57270169947441,
5.3375378655585));
#32566=CARTESIAN_POINT('Ctrl Pts',(-71.482405908805,-5.40593386564384,4.49163559729995));
#32567=CARTESIAN_POINT('Ctrl Pts',(-71.4493766470661,-5.98649320358376,
3.49808895693742));
#32568=CARTESIAN_POINT('Ctrl Pts',(-71.4163473853272,-6.56705254152368,
2.5045423165749));
#32569=CARTESIAN_POINT('Ctrl Pts',(-71.3833181235883,-6.89493905123409,
1.36335130410841));
#32570=CARTESIAN_POINT('Ctrl Pts',(-71.3502888618495,-6.93031663379197,
0.213163276828843));
#32571=CARTESIAN_POINT('Ctrl Pts',(-71.3482497957684,-6.93250067378638,
0.142156258512689));
#32572=CARTESIAN_POINT('Ctrl Pts',(-71.3462107296874,-6.9335698957285,0.0711149505267199));
#32573=CARTESIAN_POINT('Ctrl Pts',(-71.3441716636063,-6.93353164992697,
7.2489118278869E-5));
#32574=CARTESIAN_POINT('Origin',(-87.75,0.,0.));
#32575=CARTESIAN_POINT('',(-69.9148283363937,-6.93260597399068,-0.000136960269141728));
#32576=CARTESIAN_POINT('',(-70.0941716636062,-6.93269186048085,-0.000156184372951973));
#32577=CARTESIAN_POINT('',(-87.75,-6.933,-8.4904762584886E-16));
#32578=CARTESIAN_POINT('Ctrl Pts',(-69.9148283363937,-6.93260597399068,
-0.000136960269141728));
#32579=CARTESIAN_POINT('Ctrl Pts',(-69.9361497184569,-6.93207477653448,
0.74300050956666));
#32580=CARTESIAN_POINT('Ctrl Pts',(-69.9574711005202,-6.81303361409483,
1.48630411053334));
#32581=CARTESIAN_POINT('Ctrl Pts',(-69.9787924825834,-6.57829275596597,
2.19107092861746));
#32582=CARTESIAN_POINT('Ctrl Pts',(-70.0118217443223,-6.21465229302841,
3.28283541322393));
#32583=CARTESIAN_POINT('Ctrl Pts',(-70.0448510060613,-5.57336082823614,
4.28212103423564));
#32584=CARTESIAN_POINT('Ctrl Pts',(-70.0778802678001,-4.73233114382751,
5.06752102537199));
#32585=CARTESIAN_POINT('Ctrl Pts',(-70.110909529539,-3.89130145941882,5.85292101650838));
#32586=CARTESIAN_POINT('Ctrl Pts',(-70.1439387912779,-2.85053355539373,
6.42443537776939));
#32587=CARTESIAN_POINT('Ctrl Pts',(-70.1769680530168,-1.73647402822026,
6.71262879554228));
#32588=CARTESIAN_POINT('Ctrl Pts',(-70.2099973147557,-0.622414501046784,
7.00082221331518));
#32589=CARTESIAN_POINT('Ctrl Pts',(-70.2430265764946,0.564936649275099,
7.00569468759997));
#32590=CARTESIAN_POINT('Ctrl Pts',(-70.2760558382335,1.68132390603513,6.72665424415598));
#32591=CARTESIAN_POINT('Ctrl Pts',(-70.3090850999724,2.79771116279514,6.44761380071201));
#32592=CARTESIAN_POINT('Ctrl Pts',(-70.3421143617113,3.84313452599332,5.88466043953927));
#32593=CARTESIAN_POINT('Ctrl Pts',(-70.3751436234501,4.69058179085922,5.10618936788353));
#32594=CARTESIAN_POINT('Ctrl Pts',(-70.408172885189,5.53802905572517,4.32771829622775));
#32595=CARTESIAN_POINT('Ctrl Pts',(-70.4412021469279,6.18750022225883,3.33372951408891));
#32596=CARTESIAN_POINT('Ctrl Pts',(-70.4742314086668,6.56008872714797,2.24498625594301));
#32597=CARTESIAN_POINT('Ctrl Pts',(-70.5072606704057,6.9326772320371,1.15624299779714));
#32598=CARTESIAN_POINT('Ctrl Pts',(-70.5402899321446,7.02838307528173,-0.0272547363557275));
#32599=CARTESIAN_POINT('Ctrl Pts',(-70.5733191938835,6.8355786133952,-1.16171959504913));
#32600=CARTESIAN_POINT('Ctrl Pts',(-70.6063484556224,6.64277415150867,-2.29618445374251));
#32601=CARTESIAN_POINT('Ctrl Pts',(-70.6393777173613,6.16145938449097,-3.38161643697636));
#32602=CARTESIAN_POINT('Ctrl Pts',(-70.6724069791002,5.45011095625454,-4.28614255035237));
#32603=CARTESIAN_POINT('Ctrl Pts',(-70.7054362408391,4.7387625280181,-5.1906686637284));
#32604=CARTESIAN_POINT('Ctrl Pts',(-70.7384655025779,3.79738043856291,-5.91428890724661));
#32605=CARTESIAN_POINT('Ctrl Pts',(-70.7714947643168,2.740336548058,-6.36908808235563));
#32606=CARTESIAN_POINT('Ctrl Pts',(-70.8045240260557,1.68329265755312,-6.82388725746464));
#32607=CARTESIAN_POINT('Ctrl Pts',(-70.8375532877946,0.510586965998494,
-7.00986536416448));
#32608=CARTESIAN_POINT('Ctrl Pts',(-70.8705825495335,-0.635304338800435,
-6.90442726042705));
#32609=CARTESIAN_POINT('Ctrl Pts',(-70.9036118112724,-1.78119564359943,
-6.79898915668962));
#32610=CARTESIAN_POINT('Ctrl Pts',(-70.9366410730113,-2.90027256164274,
-6.40213484251487));
#32611=CARTESIAN_POINT('Ctrl Pts',(-70.9696703347502,-3.85657445566894,
-5.76207956082774));
#32612=CARTESIAN_POINT('Ctrl Pts',(-71.0026995964891,-4.81287634969511,
-5.12202427914062));
#32613=CARTESIAN_POINT('Ctrl Pts',(-71.0357288582279,-5.60640321970419,
-4.23876802994113));
#32614=CARTESIAN_POINT('Ctrl Pts',(-71.0687581199668,-6.14074666231391,
-3.21962075821167));
#32615=CARTESIAN_POINT('Ctrl Pts',(-71.1007815254425,-6.65881748270362,
-2.23151007684142));
#32616=CARTESIAN_POINT('Ctrl Pts',(-71.1328049309181,-6.93325058447245,
-1.11565905712287));
#32617=CARTESIAN_POINT('Ctrl Pts',(-71.1648283363937,-6.93357792730774,
3.67079550465076E-5));
#32618=CARTESIAN_POINT('Ctrl Pts',(-71.3441716636063,-6.93353164992697,
7.2489118278869E-5));
#32619=CARTESIAN_POINT('Ctrl Pts',(-71.3131814679485,-6.93295038143177,
-1.0796471921201));
#32620=CARTESIAN_POINT('Ctrl Pts',(-71.2821912722906,-6.67655934644521,
-2.1596332980329));
#32621=CARTESIAN_POINT('Ctrl Pts',(-71.2512010766328,-6.19016240212286,
-3.12355833346308));
#32622=CARTESIAN_POINT('Ctrl Pts',(-71.2181718148939,-5.67176193249052,
-4.1509068743828));
#32623=CARTESIAN_POINT('Ctrl Pts',(-71.185142553155,-4.8920923378205,-5.04641891412959));
#32624=CARTESIAN_POINT('Ctrl Pts',(-71.1521132914161,-3.94587845179987,
-5.70129550811248));
#32625=CARTESIAN_POINT('Ctrl Pts',(-71.1190840296772,-2.99966456577927,
-6.35617210209535));
#32626=CARTESIAN_POINT('Ctrl Pts',(-71.0860547679383,-1.88690638840805,
-6.77041325031432));
#32627=CARTESIAN_POINT('Ctrl Pts',(-71.0530255061994,-0.742796870656711,
-6.89369132150147));
#32628=CARTESIAN_POINT('Ctrl Pts',(-71.0199962444605,0.401312647094657,
-7.01696939268861));
#32629=CARTESIAN_POINT('Ctrl Pts',(-70.9869669827217,1.57677350522616,-6.84928438684391));
#32630=CARTESIAN_POINT('Ctrl Pts',(-70.9539377209828,2.64077478094005,-6.41100895207245));
#32631=CARTESIAN_POINT('Ctrl Pts',(-70.9209084592439,3.70477605665393,-5.97273351730099));
#32632=CARTESIAN_POINT('Ctrl Pts',(-70.8878791975049,4.65731774995022,-5.26386765360277));
#32633=CARTESIAN_POINT('Ctrl Pts',(-70.8548499357661,5.38267218067527,-4.37053399741801));
#32634=CARTESIAN_POINT('Ctrl Pts',(-70.8218206740272,6.10802661140029,-3.47720034123327));
#32635=CARTESIAN_POINT('Ctrl Pts',(-70.7887914122883,6.60619377955409,-2.39939889256199));
#32636=CARTESIAN_POINT('Ctrl Pts',(-70.7557621505494,6.81664958303712,-1.26807558500348));
#32637=CARTESIAN_POINT('Ctrl Pts',(-70.7227328888105,7.02710538652015,-0.136752277444937));
#32638=CARTESIAN_POINT('Ctrl Pts',(-70.6897036270716,6.94984982533242,1.04809288900076));
#32639=CARTESIAN_POINT('Ctrl Pts',(-70.6566743653327,6.59426895253398,2.14250885852276));
#32640=CARTESIAN_POINT('Ctrl Pts',(-70.6236451035938,6.23868807973553,3.2369248280448));
#32641=CARTESIAN_POINT('Ctrl Pts',(-70.590615841855,5.60478189532636,4.24091160064306));
#32642=CARTESIAN_POINT('Ctrl Pts',(-70.5575865801161,4.76956591754889,5.03249125040055));
#32643=CARTESIAN_POINT('Ctrl Pts',(-70.5245573183772,3.93434993977144,5.82407090015802));
#32644=CARTESIAN_POINT('Ctrl Pts',(-70.4915280566383,2.89782416862569,6.40324342707473));
#32645=CARTESIAN_POINT('Ctrl Pts',(-70.4584987948994,1.78591980875956,6.69964309973914));
#32646=CARTESIAN_POINT('Ctrl Pts',(-70.4254695331605,0.674015448893421,
6.99604277240355));
#32647=CARTESIAN_POINT('Ctrl Pts',(-70.3924402714216,-0.513267499693122,
7.00966959081566));
#32648=CARTESIAN_POINT('Ctrl Pts',(-70.3594110096827,-1.63168180636135,
6.73886798431246));
#32649=CARTESIAN_POINT('Ctrl Pts',(-70.3263817479438,-2.75009611302958,
6.46806637780926));
#32650=CARTESIAN_POINT('Ctrl Pts',(-70.293352486205,-3.79964177777951,5.91283634639075));
#32651=CARTESIAN_POINT('Ctrl Pts',(-70.2603232244661,-4.65280576275503,
5.14063476248562));
#32652=CARTESIAN_POINT('Ctrl Pts',(-70.2272939627272,-5.50596974773053,
4.36843317858052));
#32653=CARTESIAN_POINT('Ctrl Pts',(-70.1942647009883,-6.16275205293163,
3.3792600421888));
#32654=CARTESIAN_POINT('Ctrl Pts',(-70.1612354392494,-6.54335785879107,
2.29329351784705));
#32655=CARTESIAN_POINT('Ctrl Pts',(-70.1388808473683,-6.80095633388884,
1.55829863240126));
#32656=CARTESIAN_POINT('Ctrl Pts',(-70.1165262554873,-6.93204550151055,
0.778965200746742));
#32657=CARTESIAN_POINT('Ctrl Pts',(-70.0941716636062,-6.93269186048085,
-0.000156184372951973));
#32658=CARTESIAN_POINT('Origin',(-87.75,0.,0.));
#32659=CARTESIAN_POINT('',(-68.6648283363937,-6.93289541479494,0.00017741184833428));
#32660=CARTESIAN_POINT('',(-68.8441716636063,-6.93278929229388,0.000169878797845651));
#32661=CARTESIAN_POINT('',(-87.75,-6.933,-8.4904762584886E-16));
#32662=CARTESIAN_POINT('Ctrl Pts',(-68.6648283363937,-6.93289541479494,
0.00017741184833428));
#32663=CARTESIAN_POINT('Ctrl Pts',(-68.673435982518,-6.9331916959442,0.300153181373251));
#32664=CARTESIAN_POINT('Ctrl Pts',(-68.6820436286424,-6.91408350322542,
0.600091477363466));
#32665=CARTESIAN_POINT('Ctrl Pts',(-68.6906512747667,-6.87526712238957,
0.897457181683508));
#32666=CARTESIAN_POINT('Ctrl Pts',(-68.7236805365056,-6.7263208966894,2.03850893244921));
#32667=CARTESIAN_POINT('Ctrl Pts',(-68.7567097982446,-6.28718922697543,
3.14168157166794));
#32668=CARTESIAN_POINT('Ctrl Pts',(-68.7897390599834,-5.61122378248358,
4.07294672939748));
#32669=CARTESIAN_POINT('Ctrl Pts',(-68.8227683217223,-4.93525833799173,
5.00421188712702));
#32670=CARTESIAN_POINT('Ctrl Pts',(-68.8557975834612,-4.02245911872201,
5.76356956336737));
#32671=CARTESIAN_POINT('Ctrl Pts',(-68.8888268452001,-2.983725350259,6.25876269174234));
#32672=CARTESIAN_POINT('Ctrl Pts',(-68.9218561069389,-1.94499158179603,
6.75395582011729));
#32673=CARTESIAN_POINT('Ctrl Pts',(-68.9548853686779,-0.780323264139777,
6.98498440062688));
#32674=CARTESIAN_POINT('Ctrl Pts',(-68.9879146304168,0.368779904078343,
6.92377994882979));
#32675=CARTESIAN_POINT('Ctrl Pts',(-69.0209438921557,1.51788307229653,6.86257549703268));
#32676=CARTESIAN_POINT('Ctrl Pts',(-69.0539731538946,2.65142109107649,6.5091380129289));
#32677=CARTESIAN_POINT('Ctrl Pts',(-69.0870024156334,3.63167639255737,5.90640787426305));
#32678=CARTESIAN_POINT('Ctrl Pts',(-69.1200316773723,4.6119316940382,5.30367773559724));
#32679=CARTESIAN_POINT('Ctrl Pts',(-69.1530609391112,5.43890427821992,4.45165494236935));
#32680=CARTESIAN_POINT('Ctrl Pts',(-69.1860902008501,6.01212230288514,3.45385477583784));
#32681=CARTESIAN_POINT('Ctrl Pts',(-69.219119462589,6.58534032755038,2.4560546093063));
#32682=CARTESIAN_POINT('Ctrl Pts',(-69.2521487243279,6.90480379269919,1.31247706947107));
#32683=CARTESIAN_POINT('Ctrl Pts',(-69.2851779860668,6.93169994506568,0.162059461329396));
#32684=CARTESIAN_POINT('Ctrl Pts',(-69.3182072478057,6.95859609743217,-0.988358146812281));
#32685=CARTESIAN_POINT('Ctrl Pts',(-69.3512365095445,6.69292493701634,-2.14561582326041));
#32686=CARTESIAN_POINT('Ctrl Pts',(-69.3842657712834,6.16696379854899,-3.16911421454174));
#32687=CARTESIAN_POINT('Ctrl Pts',(-69.4172950330223,5.64100266008167,-4.19261260582304));
#32688=CARTESIAN_POINT('Ctrl Pts',(-69.4503242947612,4.85475154356283,-5.08235171193756));
#32689=CARTESIAN_POINT('Ctrl Pts',(-69.4833535565001,3.90373489519033,-5.73023396254479));
#32690=CARTESIAN_POINT('Ctrl Pts',(-69.516382818239,2.95271824681782,-6.37811621315202));
#32691=CARTESIAN_POINT('Ctrl Pts',(-69.5494120799779,1.83693606659164,-6.78414160825195));
#32692=CARTESIAN_POINT('Ctrl Pts',(-69.5824413417168,0.691948702350952,
-6.89898067766109));
#32693=CARTESIAN_POINT('Ctrl Pts',(-69.6154706034557,-0.453038661889801,
-7.01381974707024));
#32694=CARTESIAN_POINT('Ctrl Pts',(-69.6484998651946,-1.62723121014506,
-6.83747249078857));
#32695=CARTESIAN_POINT('Ctrl Pts',(-69.6815291269334,-2.68797211109765,
-6.39136396455314));
#32696=CARTESIAN_POINT('Ctrl Pts',(-69.7145583886723,-3.74871301205017,
-5.94525543831773));
#32697=CARTESIAN_POINT('Ctrl Pts',(-69.7475876504112,-4.69600226570003,
-5.2293856421286));
#32698=CARTESIAN_POINT('Ctrl Pts',(-69.7806169121501,-5.41475032947817,
-4.33072814510943));
#32699=CARTESIAN_POINT('Ctrl Pts',(-69.813646173889,-6.13349839325633,-3.43207064809025));
#32700=CARTESIAN_POINT('Ctrl Pts',(-69.8466754356279,-6.62370526716277,
-2.35062545024102));
#32701=CARTESIAN_POINT('Ctrl Pts',(-69.8797046973668,-6.82581397357457,
-1.21778117721575));
#32702=CARTESIAN_POINT('Ctrl Pts',(-69.8914125770424,-6.89745543001326,
-0.816221961491587));
#32703=CARTESIAN_POINT('Ctrl Pts',(-69.9031204567181,-6.9328976622069,-0.408204507367422));
#32704=CARTESIAN_POINT('Ctrl Pts',(-69.9148283363937,-6.93260597399068,
-0.000136960269141728));
#32705=CARTESIAN_POINT('Ctrl Pts',(-70.0941716636062,-6.93269186048085,
-0.000156184372951973));
#32706=CARTESIAN_POINT('Ctrl Pts',(-70.0834969937484,-6.93300050707366,
-0.372198922151348));
#32707=CARTESIAN_POINT('Ctrl Pts',(-70.0728223238906,-6.90356541513618,
-0.744193308803663));
#32708=CARTESIAN_POINT('Ctrl Pts',(-70.0621476540327,-6.84395829026021,
-1.11128850816545));
#32709=CARTESIAN_POINT('Ctrl Pts',(-70.0291183922938,-6.65952360935215,
-2.24714409754429));
#32710=CARTESIAN_POINT('Ctrl Pts',(-69.9960891305549,-6.18622494101828,
-3.33609536401019));
#32711=CARTESIAN_POINT('Ctrl Pts',(-69.963059868816,-5.48156502481484,-4.2458417429208));
#32712=CARTESIAN_POINT('Ctrl Pts',(-69.9300306070771,-4.77690510861136,
-5.15558812183147));
#32713=CARTESIAN_POINT('Ctrl Pts',(-69.8970013453382,-3.84088394453828,
-5.88612961318685));
#32714=CARTESIAN_POINT('Ctrl Pts',(-69.8639720835994,-2.78722207486187,
-6.34871013140502));
#32715=CARTESIAN_POINT('Ctrl Pts',(-69.8309428218605,-1.73356020518553,
-6.81129064962317));
#32716=CARTESIAN_POINT('Ctrl Pts',(-69.7979135601216,-0.562257629905866,
-7.00591019470415));
#32717=CARTESIAN_POINT('Ctrl Pts',(-69.7648842983827,0.584379932761237,
-6.90892374551841));
#32718=CARTESIAN_POINT('Ctrl Pts',(-69.7318550366438,1.73101749542841,-6.81193729633265));
#32719=CARTESIAN_POINT('Ctrl Pts',(-69.6988257749049,2.85299004548303,-6.42334485288014));
#32720=CARTESIAN_POINT('Ctrl Pts',(-69.665796513166,3.81398514502586,-5.79035789401002));
#32721=CARTESIAN_POINT('Ctrl Pts',(-69.6327672514271,4.77498024456863,-5.15737093513994));
#32722=CARTESIAN_POINT('Ctrl Pts',(-69.5997379896882,5.57499789359964,-4.27998946085228));
#32723=CARTESIAN_POINT('Ctrl Pts',(-69.5667087279493,6.11684110089434,-3.26480966881867));
#32724=CARTESIAN_POINT('Ctrl Pts',(-69.5336794662104,6.65868430818905,-2.24962987678502));
#32725=CARTESIAN_POINT('Ctrl Pts',(-69.5006502044716,6.94235307374744,-1.0966517670055));
#32726=CARTESIAN_POINT('Ctrl Pts',(-69.4676209427327,6.9333834697424,0.0540452468295327));
#32727=CARTESIAN_POINT('Ctrl Pts',(-69.4345916809938,6.92441386573736,1.2047422606645));
#32728=CARTESIAN_POINT('Ctrl Pts',(-69.4015624192549,6.62280589216886,2.353158178555));
#32729=CARTESIAN_POINT('Ctrl Pts',(-69.368533157516,6.06520297508595,3.35976786373859));
#32730=CARTESIAN_POINT('Ctrl Pts',(-69.3355038957771,5.50760005800299,4.36637754892227));
#32731=CARTESIAN_POINT('Ctrl Pts',(-69.3024746340382,4.69400219740564,5.23118100139905));
#32732=CARTESIAN_POINT('Ctrl Pts',(-69.2694453722993,3.7232562927498,5.84911017212886));
#32733=CARTESIAN_POINT('Ctrl Pts',(-69.2364161105604,2.75251038809402,6.46703934285863));
#32734=CARTESIAN_POINT('Ctrl Pts',(-69.2033868488216,1.6246164393798,6.83809423184139));
#32735=CARTESIAN_POINT('Ctrl Pts',(-69.1703575870827,0.476606296302118,
6.91719406013208));
#32736=CARTESIAN_POINT('Ctrl Pts',(-69.1373283253438,-0.671403846775601,
6.99629388842278));
#32737=CARTESIAN_POINT('Ctrl Pts',(-69.1042990636049,-1.83953018421682,
6.78343865602139));
#32738=CARTESIAN_POINT('Ctrl Pts',(-69.0712698018661,-2.88585289024383,
6.30448890260542));
#32739=CARTESIAN_POINT('Ctrl Pts',(-69.0382405401271,-3.93217559627087,
5.82553914918944));
#32740=CARTESIAN_POINT('Ctrl Pts',(-69.0052112783882,-4.85669467088372,
5.08049487475885));
#32741=CARTESIAN_POINT('Ctrl Pts',(-68.9721820166493,-5.54708700159773,
4.1598741596237));
#32742=CARTESIAN_POINT('Ctrl Pts',(-68.9391527549104,-6.23747933231171,
3.2392534444886));
#32743=CARTESIAN_POINT('Ctrl Pts',(-68.9061234931715,-6.69374491912688,
2.14305628864894));
#32744=CARTESIAN_POINT('Ctrl Pts',(-68.8730942314327,-6.86045043217612,
1.00446358563143));
#32745=CARTESIAN_POINT('Ctrl Pts',(-68.8634533754906,-6.90910982543695,
0.672121666719093));
#32746=CARTESIAN_POINT('Ctrl Pts',(-68.8538125195484,-6.93309904925115,
0.33616769826188));
#32747=CARTESIAN_POINT('Ctrl Pts',(-68.8441716636063,-6.93278929229388,
0.000169878797845651));
#32748=CARTESIAN_POINT('Origin',(-87.75,0.,0.));
#32749=CARTESIAN_POINT('',(-67.4148283363937,-6.93337279743796,-0.000131731084783704));
#32750=CARTESIAN_POINT('',(-67.5941716636062,-6.9334612849287,-0.000104716709421631));
#32751=CARTESIAN_POINT('',(-87.75,-6.933,-8.4904762584886E-16));
#32752=CARTESIAN_POINT('Ctrl Pts',(-67.4148283363937,-6.93337279743796,
-0.000131731084783704));
#32753=CARTESIAN_POINT('Ctrl Pts',(-67.4437515083181,-6.93249558801675,
1.00763853557119));
#32754=CARTESIAN_POINT('Ctrl Pts',(-67.4726746802424,-6.71019820674341,
2.01578265024431));
#32755=CARTESIAN_POINT('Ctrl Pts',(-67.5015978521667,-6.28450099732112,
2.92912494075186));
#32756=CARTESIAN_POINT('Ctrl Pts',(-67.5346271139056,-5.79836951117891,
3.97213023938542));
#32757=CARTESIAN_POINT('Ctrl Pts',(-67.5676563756445,-5.04698736297379,
4.89150590247039));
#32758=CARTESIAN_POINT('Ctrl Pts',(-67.6006856373834,-4.1216423195172,5.57555315608241));
#32759=CARTESIAN_POINT('Ctrl Pts',(-67.6337148991223,-3.1962972760606,6.25960040969444));
#32760=CARTESIAN_POINT('Ctrl Pts',(-67.6667441608612,-2.09698933735247,
6.70831925383352));
#32761=CARTESIAN_POINT('Ctrl Pts',(-67.6997734226,-0.957277496925685,6.86719351183532));
#32762=CARTESIAN_POINT('Ctrl Pts',(-67.7328026843389,0.182434343501171,
7.02606776983713));
#32763=CARTESIAN_POINT('Ctrl Pts',(-67.7658319460778,1.36255008564665,6.89509744170168));
#32764=CARTESIAN_POINT('Ctrl Pts',(-67.7988612078167,2.43969334714329,6.49019444427998));
#32765=CARTESIAN_POINT('Ctrl Pts',(-67.8318904695556,3.51683660863984,6.08529144685832));
#32766=CARTESIAN_POINT('Ctrl Pts',(-67.8649197312945,4.49100738948749,5.40645578015041));
#32767=CARTESIAN_POINT('Ctrl Pts',(-67.8979489930334,5.24385017583266,4.53616167136526));
#32768=CARTESIAN_POINT('Ctrl Pts',(-67.9309782547723,5.99669296217787,3.66586756258006));
#32769=CARTESIAN_POINT('Ctrl Pts',(-67.9640075165112,6.52820775402063,2.60411501171758));
#32770=CARTESIAN_POINT('Ctrl Pts',(-67.9970367782501,6.7738189469558,1.47990008199233));
#32771=CARTESIAN_POINT('Ctrl Pts',(-68.0300660399889,7.01943013989096,0.355685152267077));
#32772=CARTESIAN_POINT('Ctrl Pts',(-68.0630953017278,6.97913773391853,-0.830992156320916));
#32773=CARTESIAN_POINT('Ctrl Pts',(-68.0961245634667,6.65783698737675,-1.93595817837977));
#32774=CARTESIAN_POINT('Ctrl Pts',(-68.1291538252056,6.33653624083498,-3.04092420043856));
#32775=CARTESIAN_POINT('Ctrl Pts',(-68.1621830869445,5.73422715372385,-4.06417893596827));
#32776=CARTESIAN_POINT('Ctrl Pts',(-68.1952123486834,4.92408640515072,-4.88140353361028));
#32777=CARTESIAN_POINT('Ctrl Pts',(-68.2282416104223,4.11394565657754,-5.69862813125233));
#32778=CARTESIAN_POINT('Ctrl Pts',(-68.2612708721612,3.0959732465424,-6.30982259100668));
#32779=CARTESIAN_POINT('Ctrl Pts',(-68.2943001339001,1.99384626352711,-6.64073071896694));
#32780=CARTESIAN_POINT('Ctrl Pts',(-68.327329395639,0.891719280511826,-6.9716388469272));
#32781=CARTESIAN_POINT('Ctrl Pts',(-68.3603586573778,-0.294562275483611,
-7.0222606430933));
#32782=CARTESIAN_POINT('Ctrl Pts',(-68.3933879191167,-1.4208728354367,-6.7864458872314));
#32783=CARTESIAN_POINT('Ctrl Pts',(-68.4264171808556,-2.54718339538978,
-6.55063113136949));
#32784=CARTESIAN_POINT('Ctrl Pts',(-68.4594464425945,-3.61352295930058,
-6.02837982347959));
#32785=CARTESIAN_POINT('Ctrl Pts',(-68.4924757043334,-4.49033813929784,
-5.28314213255427));
#32786=CARTESIAN_POINT('Ctrl Pts',(-68.5255049660723,-5.3671533192951,-4.53790444162894));
#32787=CARTESIAN_POINT('Ctrl Pts',(-68.5585342278112,-6.05444411537879,
-3.56968036766821));
#32788=CARTESIAN_POINT('Ctrl Pts',(-68.5915634895501,-6.46870912257745,
-2.49610289953149));
#32789=CARTESIAN_POINT('Ctrl Pts',(-68.6159851051646,-6.77501390311845,
-1.70230688717924));
#32790=CARTESIAN_POINT('Ctrl Pts',(-68.6404067207792,-6.93205480584839,
-0.850913912212287));
#32791=CARTESIAN_POINT('Ctrl Pts',(-68.6648283363937,-6.93289541479494,
0.00017741184833428));
#32792=CARTESIAN_POINT('Ctrl Pts',(-68.8441716636063,-6.93278929229388,
0.000169878797845651));
#32793=CARTESIAN_POINT('Ctrl Pts',(-68.8207832578095,-6.9320378318988,-0.814950002218331));
#32794=CARTESIAN_POINT('Ctrl Pts',(-68.7973948520128,-6.78827910312482,
-1.63032796042549));
#32795=CARTESIAN_POINT('Ctrl Pts',(-68.774006446216,-6.50681278781459,-2.39501869962106));
#32796=CARTESIAN_POINT('Ctrl Pts',(-68.7409771844771,-6.1093241911205,-3.4749200316607));
#32797=CARTESIAN_POINT('Ctrl Pts',(-68.7079479227382,-5.43720155844903,
-4.45373444554453));
#32798=CARTESIAN_POINT('Ctrl Pts',(-68.6749186609993,-4.57210346034106,
-5.21254229480466));
#32799=CARTESIAN_POINT('Ctrl Pts',(-68.6418893992604,-3.70700536223314,
-5.97135014406476));
#32800=CARTESIAN_POINT('Ctrl Pts',(-68.6088601375215,-2.64893179868877,
-6.51015142870117));
#32801=CARTESIAN_POINT('Ctrl Pts',(-68.5758308757826,-1.52643189234264,
-6.76348526318229));
#32802=CARTESIAN_POINT('Ctrl Pts',(-68.5428016140437,-0.403931985996506,
-7.01681909766341));
#32803=CARTESIAN_POINT('Ctrl Pts',(-68.5097723523049,0.782994263151457,
-6.98468548198923));
#32804=CARTESIAN_POINT('Ctrl Pts',(-68.476743090566,1.89014296115799,-6.67098844351297));
#32805=CARTESIAN_POINT('Ctrl Pts',(-68.4437138288271,2.99729165916456,-6.3572914050367));
#32806=CARTESIAN_POINT('Ctrl Pts',(-68.4106845670882,4.0246628060297,-5.7620309437584));
#32807=CARTESIAN_POINT('Ctrl Pts',(-68.3776553053493,4.84743742496519,-4.95752737142637));
#32808=CARTESIAN_POINT('Ctrl Pts',(-68.3446260436104,5.67021204390068,-4.15302379909433));
#32809=CARTESIAN_POINT('Ctrl Pts',(-68.3115967818716,6.28839013490641,-3.13927711570861));
#32810=CARTESIAN_POINT('Ctrl Pts',(-68.2785675201327,6.62686704182652,-2.03945101360489));
#32811=CARTESIAN_POINT('Ctrl Pts',(-68.2455382583938,6.96534394874662,-0.939624911501181));
#32812=CARTESIAN_POINT('Ctrl Pts',(-68.2125089966549,7.02411967158108,0.246280609320601));
#32813=CARTESIAN_POINT('Ctrl Pts',(-68.179479734916,6.7960533385008,1.3741856670747));
#32814=CARTESIAN_POINT('Ctrl Pts',(-68.1464504731771,6.56798700542051,2.5020907248288));
#32815=CARTESIAN_POINT('Ctrl Pts',(-68.1134212114382,6.05307861642555,3.57199531951521));
#32816=CARTESIAN_POINT('Ctrl Pts',(-68.0803919496993,5.31388622430591,4.45391293391699));
#32817=CARTESIAN_POINT('Ctrl Pts',(-68.0473626879604,4.57469383218627,5.33583054831877));
#32818=CARTESIAN_POINT('Ctrl Pts',(-68.0143334262215,3.61121743694198,6.02976118243583));
#32819=CARTESIAN_POINT('Ctrl Pts',(-67.9813041644826,2.54051321418835,6.4513967350567));
#32820=CARTESIAN_POINT('Ctrl Pts',(-67.9482749027437,1.46980899143475,6.87303228767757));
#32821=CARTESIAN_POINT('Ctrl Pts',(-67.9152456410048,0.291876941171729,
7.02237275880227));
#32822=CARTESIAN_POINT('Ctrl Pts',(-67.882216379266,-0.8501717790824,6.88127424103013));
#32823=CARTESIAN_POINT('Ctrl Pts',(-67.8491871175271,-1.99222049933653,
6.74017572325799));
#32824=CARTESIAN_POINT('Ctrl Pts',(-67.8161578557882,-3.09838588958184,
6.30863821658903));
#32825=CARTESIAN_POINT('Ctrl Pts',(-67.7831285940493,-4.0342759816279,5.63909075269439));
#32826=CARTESIAN_POINT('Ctrl Pts',(-67.7500993323104,-4.97016607367399,
4.96954328879973));
#32827=CARTESIAN_POINT('Ctrl Pts',(-67.7170700705715,-5.73578086752079,
4.06198586767938));
#32828=CARTESIAN_POINT('Ctrl Pts',(-67.6840408088326,-6.23810309398541,
3.02668086153105));
#32829=CARTESIAN_POINT('Ctrl Pts',(-67.6540844270905,-6.69369173209929,
2.08769553909514));
#32830=CARTESIAN_POINT('Ctrl Pts',(-67.6241280453483,-6.93269975711327,
1.04362692257891));
#32831=CARTESIAN_POINT('Ctrl Pts',(-67.5941716636062,-6.9334612849287,-0.000104716709421631));
#32832=CARTESIAN_POINT('Origin',(-88.8777445817596,0.,0.));
#32833=CARTESIAN_POINT('',(-67.0027445817596,-6.21958441806809,-0.000118169414145055));
#32834=CARTESIAN_POINT('',(-66.7562554182403,-6.21873914925953,1.11460959661969E-5));
#32835=CARTESIAN_POINT('',(-88.8777445817596,-6.21925,-6.18233832090354E-13));
#32836=CARTESIAN_POINT('',(-66.51072,4.88120307569155,-3.85434375923658));
#32837=CARTESIAN_POINT('Ctrl Pts',(-67.0027445817596,-6.21958441806809,
-0.000118169414144789));
#32838=CARTESIAN_POINT('Ctrl Pts',(-66.9986384919451,-6.21969613078843,
-0.128457828390552));
#32839=CARTESIAN_POINT('Ctrl Pts',(-66.9615031403916,-6.18450232485475,
-1.28909667822277));
#32840=CARTESIAN_POINT('Ctrl Pts',(-66.8913385270993,-5.49220424623203,
-3.44324500874027));
#32841=CARTESIAN_POINT('Ctrl Pts',(-66.7922507418826,-3.17999782273006,
-5.64870137951734));
#32842=CARTESIAN_POINT('Ctrl Pts',(-66.693162956666,-0.0950831417423778,
-6.481612708114));
#32843=CARTESIAN_POINT('Ctrl Pts',(-66.5993193760384,2.84842541282538,-5.77881590697225));
#32844=CARTESIAN_POINT('Ctrl Pts',(-66.5385050571497,4.34230708651471,-4.53542015418599));
#32845=CARTESIAN_POINT('Ctrl Pts',(-66.51072,4.88120307569155,-3.85434375923658));
#32846=CARTESIAN_POINT('',(-66.51072,-2.0540967914958,-5.87024334535347));
#32847=CARTESIAN_POINT('Origin',(-66.51072,0.,0.));
#32848=CARTESIAN_POINT('Ctrl Pts',(-66.7562554182403,-6.21873914925953,
1.11460959660928E-5));
#32849=CARTESIAN_POINT('Ctrl Pts',(-66.7404688023046,-6.2188028846916,-0.493595494752219));
#32850=CARTESIAN_POINT('Ctrl Pts',(-66.6916529246301,-6.0392566751686,-2.01992285710156));
#32851=CARTESIAN_POINT('Ctrl Pts',(-66.6098077852167,-4.80376045256683,
-4.35266662668044));
#32852=CARTESIAN_POINT('Ctrl Pts',(-66.5437492617389,-3.02869324528072,
-5.529215668825));
#32853=CARTESIAN_POINT('Ctrl Pts',(-66.51072,-2.05409679149563,-5.87024334535353));
#32854=CARTESIAN_POINT('Origin',(-88.8777445817596,0.,0.));
#32855=CARTESIAN_POINT('',(-68.2527445817596,-6.21915618180635,0.000159147358266852));
#32856=CARTESIAN_POINT('',(-68.0062554182403,-6.21966379580164,-9.39361602741995E-5));
#32857=CARTESIAN_POINT('',(-88.8777445817596,-6.21925,-6.18233832090354E-13));
#32858=CARTESIAN_POINT('Ctrl Pts',(-68.2527445817596,-6.21915618180635,
0.000159147358266866));
#32859=CARTESIAN_POINT('Ctrl Pts',(-68.2283229661451,-6.21840211326586,
-0.763312613374919));
#32860=CARTESIAN_POINT('Ctrl Pts',(-68.1708720887917,-5.88700259581307,
-2.55998606699028));
#32861=CARTESIAN_POINT('Ctrl Pts',(-68.0803919496993,-4.1980722627264,-4.9392744512594));
#32862=CARTESIAN_POINT('Ctrl Pts',(-67.9813041644827,-1.3283914609729,-6.34473158955201));
#32863=CARTESIAN_POINT('Ctrl Pts',(-67.882216379266,1.864071354745,-6.20850069132352));
#32864=CARTESIAN_POINT('Ctrl Pts',(-67.7831285940493,4.60358884116279,-4.5636840994466));
#32865=CARTESIAN_POINT('Ctrl Pts',(-67.6840408088326,6.22449355341539,-1.80995107740288));
#32866=CARTESIAN_POINT('Ctrl Pts',(-67.584953023616,6.33292650272045,1.38357676830714));
#32867=CARTESIAN_POINT('Ctrl Pts',(-67.4858652383993,4.90253993016824,4.24091322523118));
#32868=CARTESIAN_POINT('Ctrl Pts',(-67.3867774531826,2.2808992426794,6.06776251998367));
#32869=CARTESIAN_POINT('Ctrl Pts',(-67.287689667966,-0.894970436826739,
6.42022345172595));
#32870=CARTESIAN_POINT('Ctrl Pts',(-67.1886018827492,-3.8533741139406,5.21265327802973));
#32871=CARTESIAN_POINT('Ctrl Pts',(-67.0936201873472,-5.79166403763128,
2.84100179801934));
#32872=CARTESIAN_POINT('Ctrl Pts',(-67.031667753684,-6.21879751705943,0.903902489881935));
#32873=CARTESIAN_POINT('Ctrl Pts',(-67.0027445817596,-6.21958441806809,
-0.000118169414144789));
#32874=CARTESIAN_POINT('Ctrl Pts',(-68.0062554182403,-6.21966379580164,
-9.39361602741995E-5));
#32875=CARTESIAN_POINT('Ctrl Pts',(-68.0031825382435,-6.21973387011156,
-0.0961360936374352));
#32876=CARTESIAN_POINT('Ctrl Pts',(-67.9670803965079,-6.19413651603434,
-1.22446285990289));
#32877=CARTESIAN_POINT('Ctrl Pts',(-67.8979489930334,-5.54518383041795,
-3.35725764403967));
#32878=CARTESIAN_POINT('Ctrl Pts',(-67.7988612078167,-3.26761528590833,
-5.59847600248888));
#32879=CARTESIAN_POINT('Ctrl Pts',(-67.6997734226,-0.196058420264034,-6.47933655521552));
#32880=CARTESIAN_POINT('Ctrl Pts',(-67.6006856373834,2.92313831475997,-5.78580232210167));
#32881=CARTESIAN_POINT('Ctrl Pts',(-67.5015978521667,5.33204969326613,-3.6863915925369));
#32882=CARTESIAN_POINT('Ctrl Pts',(-67.4025100669501,6.44534250489529,-0.691237361863573));
#32883=CARTESIAN_POINT('Ctrl Pts',(-67.3034222817333,5.99249846114462,2.47188303450135));
#32884=CARTESIAN_POINT('Ctrl Pts',(-67.2043344965166,4.08355785429189,5.03435879238504));
#32885=CARTESIAN_POINT('Ctrl Pts',(-67.1052467113001,1.18235847344737,6.37356827685746));
#32886=CARTESIAN_POINT('Ctrl Pts',(-67.0061589260833,-2.0061249511844,6.16404616060605));
#32887=CARTESIAN_POINT('Ctrl Pts',(-66.9070711408667,-4.70717390764343,
4.4568144926439));
#32888=CARTESIAN_POINT('Ctrl Pts',(-66.8237699715857,-6.01628953715405,
2.11103777105964));
#32889=CARTESIAN_POINT('Ctrl Pts',(-66.7734980640435,-6.21866953538632,
0.539144074200984));
#32890=CARTESIAN_POINT('Ctrl Pts',(-66.7562554182403,-6.21873914925953,
1.11460959660928E-5));
#32891=CARTESIAN_POINT('Origin',(-88.8777445817596,0.,0.));
#32892=CARTESIAN_POINT('',(-69.5027445817596,-6.21889653883479,-0.000122860255921536));
#32893=CARTESIAN_POINT('',(-69.2562554182403,-6.2190609845808,0.000152389832417943));
#32894=CARTESIAN_POINT('',(-88.8777445817596,-6.21925,-6.18233832090354E-13));
#32895=CARTESIAN_POINT('Ctrl Pts',(-69.5027445817596,-6.21889653883479,
-0.000122860255920947));
#32896=CARTESIAN_POINT('Ctrl Pts',(-69.491036702084,-6.21915819784801,-0.366179991698439));
#32897=CARTESIAN_POINT('Ctrl Pts',(-69.4462995606695,-6.09767174240742,
-1.76475426852759));
#32898=CARTESIAN_POINT('Ctrl Pts',(-69.368533157516,-5.062316570275,-4.04885091949506));
#32899=CARTESIAN_POINT('Ctrl Pts',(-69.2694453722994,-2.5130181320396,-5.97536464946014));
#32900=CARTESIAN_POINT('Ctrl Pts',(-69.1703575870826,0.646911338205425,
-6.44994174752579));
#32901=CARTESIAN_POINT('Ctrl Pts',(-69.0712698018661,3.64964968713308,-5.35726609262518));
#32902=CARTESIAN_POINT('Ctrl Pts',(-68.9721820166493,5.76557017887249,-2.96284379245084));
#32903=CARTESIAN_POINT('Ctrl Pts',(-68.8730942314327,6.48053139238009,0.151511380309847));
#32904=CARTESIAN_POINT('Ctrl Pts',(-68.774006446216,5.62080696329017,3.22905123951376));
#32905=CARTESIAN_POINT('Ctrl Pts',(-68.6749186609993,3.39529885244121,5.52197324591022));
#32906=CARTESIAN_POINT('Ctrl Pts',(-68.5758308757827,0.344776860533978,
6.47312689065817));
#32907=CARTESIAN_POINT('Ctrl Pts',(-68.476743090566,-2.78952146684973,5.85139409129237));
#32908=CARTESIAN_POINT('Ctrl Pts',(-68.3776553053494,-5.24600201399085,
3.80784790870568));
#32909=CARTESIAN_POINT('Ctrl Pts',(-68.3029891357472,-6.13650745964284,
1.5707483996713));
#32910=CARTESIAN_POINT('Ctrl Pts',(-68.2613522278839,-6.21942196091174,
0.269252513090079));
#32911=CARTESIAN_POINT('Ctrl Pts',(-68.2527445817596,-6.21915618180635,
0.000159147358266866));
#32912=CARTESIAN_POINT('Ctrl Pts',(-69.2562554182403,-6.2190609845808,0.00015238983241829));
#32913=CARTESIAN_POINT('Ctrl Pts',(-69.2328670124436,-6.21838688677859,
-0.731051175724831));
#32914=CARTESIAN_POINT('Ctrl Pts',(-69.176449344908,-5.90731157488004,-2.49542371037046));
#32915=CARTESIAN_POINT('Ctrl Pts',(-69.0870024156334,-4.27451566553321,
-4.87326979575939));
#32916=CARTESIAN_POINT('Ctrl Pts',(-68.9879146304167,-1.42707991907126,
-6.32326542080269));
#32917=CARTESIAN_POINT('Ctrl Pts',(-68.8888268452001,1.76711786327968,-6.23678900830517));
#32918=CARTESIAN_POINT('Ctrl Pts',(-68.7897390599834,4.5319287698749,-4.63485321262994));
#32919=CARTESIAN_POINT('Ctrl Pts',(-68.6906512747668,6.19553936809527,-1.90670779478191));
#32920=CARTESIAN_POINT('Ctrl Pts',(-68.5915634895501,6.35371371436876,1.28474305349599));
#32921=CARTESIAN_POINT('Ctrl Pts',(-68.4924757043333,4.96801747972696,4.16401789144663));
#32922=CARTESIAN_POINT('Ctrl Pts',(-68.3933879191168,2.37515699892946,6.03149002309199));
#32923=CARTESIAN_POINT('Ctrl Pts',(-68.2943001338999,-0.794836035946308,
6.43338778381987));
#32924=CARTESIAN_POINT('Ctrl Pts',(-68.1952123486834,-3.77169415073787,
5.27205518392761));
#32925=CARTESIAN_POINT('Ctrl Pts',(-68.0991974434635,-5.76818315324227,
2.9054232627965));
#32926=CARTESIAN_POINT('Ctrl Pts',(-68.0362117999824,-6.21898066701678,
0.936185884645314));
#32927=CARTESIAN_POINT('Ctrl Pts',(-68.0062554182403,-6.21966379580164,
-9.39361602741995E-5));
#32928=CARTESIAN_POINT('Origin',(-88.8777445817596,0.,0.));
#32929=CARTESIAN_POINT('',(-70.7527445817596,-6.2197684298873,3.29288831883953E-5));
#32930=CARTESIAN_POINT('',(-70.5062554182403,-6.2189735833399,-0.000140105245378663));
#32931=CARTESIAN_POINT('',(-88.8777445817596,-6.21925,-6.18233832090354E-13));
#32932=CARTESIAN_POINT('Ctrl Pts',(-70.7527445817596,-6.2197684298873,3.29288831883321E-5));
#32933=CARTESIAN_POINT('Ctrl Pts',(-70.720721176284,-6.2194747868859,-1.00080233535455));
#32934=CARTESIAN_POINT('Ctrl Pts',(-70.6556685090695,-5.71938164108245,
-3.03419205074321));
#32935=CARTESIAN_POINT('Ctrl Pts',(-70.5575865801161,-3.6055588131454,-5.38703893348903));
#32936=CARTESIAN_POINT('Ctrl Pts',(-70.4584987948994,-0.593953827191011,
-6.45503382463191));
#32937=CARTESIAN_POINT('Ctrl Pts',(-70.3594110096827,2.56197428713231,-5.95453865366998));
#32938=CARTESIAN_POINT('Ctrl Pts',(-70.2603232244661,5.09537565443828,-4.00716729949408));
#32939=CARTESIAN_POINT('Ctrl Pts',(-70.1612354392494,6.39066637913534,-1.08610591406471));
#32940=CARTESIAN_POINT('Ctrl Pts',(-70.0621476540327,6.13310750176651,2.09886521667122));
#32941=CARTESIAN_POINT('Ctrl Pts',(-69.9630598688161,4.38528251151797,4.77383913848715));
#32942=CARTESIAN_POINT('Ctrl Pts',(-69.8639720835993,1.57189036458139,6.28883164886079));
#32943=CARTESIAN_POINT('Ctrl Pts',(-69.7648842983828,-1.62345089099596,
6.27571908473456));
#32944=CARTESIAN_POINT('Ctrl Pts',(-69.665796513166,-4.42431449424472,4.73768763026785));
#32945=CARTESIAN_POINT('Ctrl Pts',(-69.578416607625,-5.94621050523724,2.36620931821423));
#32946=CARTESIAN_POINT('Ctrl Pts',(-69.5240659638229,-6.21842002797665,
0.666508858953097));
#32947=CARTESIAN_POINT('Ctrl Pts',(-69.5027445817596,-6.21889653883479,
-0.000122860255920947));
#32948=CARTESIAN_POINT('Ctrl Pts',(-70.5062554182403,-6.2189735833399,-0.000140105245378629));
#32949=CARTESIAN_POINT('Ctrl Pts',(-70.4955807483825,-6.21925045487056,
-0.33388116927637));
#32950=CARTESIAN_POINT('Ctrl Pts',(-70.4518768167858,-6.11114483612411,
-1.70009682182616));
#32951=CARTESIAN_POINT('Ctrl Pts',(-70.3751436234501,-5.12478244935701,
-3.96948957977628));
#32952=CARTESIAN_POINT('Ctrl Pts',(-70.2760558382335,-2.60580814184455,
-5.93548705710717));
#32953=CARTESIAN_POINT('Ctrl Pts',(-70.1769680530168,0.546343974688648,
-6.45923764375577));
#32954=CARTESIAN_POINT('Ctrl Pts',(-70.0778802678002,3.56574154367478,-5.4134766944083));
#32955=CARTESIAN_POINT('Ctrl Pts',(-69.9787924825834,5.71870985338321,-3.05231064769102));
#32956=CARTESIAN_POINT('Ctrl Pts',(-69.8797046973668,6.48210534027158,0.0505275648778713));
#32957=CARTESIAN_POINT('Ctrl Pts',(-69.7806169121501,5.67043273550486,3.14108823010512));
#32958=CARTESIAN_POINT('Ctrl Pts',(-69.6815291269334,3.4809180256302,5.46840492063578));
#32959=CARTESIAN_POINT('Ctrl Pts',(-69.5824413417167,0.445585078619785,
6.46696966243845));
#32960=CARTESIAN_POINT('Ctrl Pts',(-69.4833535565002,-2.69801930222453,
5.89414408731404));
#32961=CARTESIAN_POINT('Ctrl Pts',(-69.3842657712834,-5.18603974998983,
3.88911743056271));
#32962=CARTESIAN_POINT('Ctrl Pts',(-69.3085663918635,-6.12409405569377,
1.63540272655992));
#32963=CARTESIAN_POINT('Ctrl Pts',(-69.2658962741825,-6.21933885216436,
0.301559347672218));
#32964=CARTESIAN_POINT('Ctrl Pts',(-69.2562554182403,-6.2190609845808,0.00015238983241829));
#32965=CARTESIAN_POINT('Origin',(-88.8777445817596,0.,0.));
#32966=CARTESIAN_POINT('',(-72.0027445817596,-6.21878348465591,7.77291339505116E-5));
#32967=CARTESIAN_POINT('',(-71.7562554182403,-6.21972691674719,6.50263875292059E-5));
#32968=CARTESIAN_POINT('',(-88.8777445817596,-6.21925,-6.18233832090354E-13));
#32969=CARTESIAN_POINT('Ctrl Pts',(-72.0027445817596,-6.21878348465591,
7.77291339506408E-5));
#32970=CARTESIAN_POINT('Ctrl Pts',(-71.9834349122229,-6.21851690018761,
-0.603687467000913));
#32971=CARTESIAN_POINT('Ctrl Pts',(-71.9310959809473,-5.98187890039571,
-2.24039980722369));
#32972=CARTESIAN_POINT('Ctrl Pts',(-71.8457277879328,-4.56597889785132,
-4.60131280509741));
#32973=CARTESIAN_POINT('Ctrl Pts',(-71.7466400027161,-1.81305439576657,
-6.22359032905994));
#32974=CARTESIAN_POINT('Ctrl Pts',(-71.6475522174995,1.38041896772984,-6.33361557875979));
#32975=CARTESIAN_POINT('Ctrl Pts',(-71.5484644322828,4.238468305381,-4.90465383592539));
#32976=CARTESIAN_POINT('Ctrl Pts',(-71.4493766470661,6.06662444709443,-2.28392439539779));
#32977=CARTESIAN_POINT('Ctrl Pts',(-71.3502888618495,6.42066900174233,0.89176925044665));
#32978=CARTESIAN_POINT('Ctrl Pts',(-71.2512010766327,5.2145737035411,3.8507744566924));
#32979=CARTESIAN_POINT('Ctrl Pts',(-71.1521132914161,2.7414041723735,5.87409107774727));
#32980=CARTESIAN_POINT('Ctrl Pts',(-71.0530255061994,-0.397891256411005,
6.47007924016768));
#32981=CARTESIAN_POINT('Ctrl Pts',(-70.9539377209828,-3.44050423574074,
5.49392149833132));
#32982=CARTESIAN_POINT('Ctrl Pts',(-70.854849935766,-5.64711900824516,3.18281160810583));
#32983=CARTESIAN_POINT('Ctrl Pts',(-70.787785556025,-6.21188125558683,1.09517235362907));
#32984=CARTESIAN_POINT('Ctrl Pts',(-70.7537504380229,-6.21977765322404,
0.0314691988263317));
#32985=CARTESIAN_POINT('Ctrl Pts',(-70.7527445817596,-6.2197684298873,3.29288831883321E-5));
#32986=CARTESIAN_POINT('Ctrl Pts',(-71.7562554182403,-6.21972691674719,
6.50263875293274E-5));
#32987=CARTESIAN_POINT('Ctrl Pts',(-71.7252652225825,-6.21920548964646,
-0.968497879647463));
#32988=CARTESIAN_POINT('Ctrl Pts',(-71.6612457651859,-5.74408110420307,
-2.96984607376813));
#32989=CARTESIAN_POINT('Ctrl Pts',(-71.5641970460501,-3.68905021568418,
-5.33021117624344));
#32990=CARTESIAN_POINT('Ctrl Pts',(-71.4651092608335,-0.694449915114697,
-6.44499666350474));
#32991=CARTESIAN_POINT('Ctrl Pts',(-71.3660214756168,2.46889276854356,-5.99373098951091));
#32992=CARTESIAN_POINT('Ctrl Pts',(-71.2669336904001,5.03232631507441,-4.0860658995909));
#32993=CARTESIAN_POINT('Ctrl Pts',(-71.1678459051835,6.37296939622566,-1.1855394350089));
#32994=CARTESIAN_POINT('Ctrl Pts',(-71.0687581199668,6.16506301417589,2.00305783951203));
#32995=CARTESIAN_POINT('Ctrl Pts',(-70.9696703347502,4.4591257413993,4.70493786351959));
#32996=CARTESIAN_POINT('Ctrl Pts',(-70.8705825495335,1.66967835836243,6.26357859827801));
#32997=CARTESIAN_POINT('Ctrl Pts',(-70.7714947643168,-1.5254793560455,6.30025042450449));
#32998=CARTESIAN_POINT('Ctrl Pts',(-70.6724069791001,-4.34996523899484,
4.8060425608526));
#32999=CARTESIAN_POINT('Ctrl Pts',(-70.5839938637413,-5.92705381389802,
2.43080553078847));
#33000=CARTESIAN_POINT('Ctrl Pts',(-70.5286100101214,-6.21839376680658,
0.698770997366347));
#33001=CARTESIAN_POINT('Ctrl Pts',(-70.5062554182403,-6.2189735833399,-0.000140105245378629));
#33002=CARTESIAN_POINT('Origin',(-88.8777445817596,0.,0.));
#33003=CARTESIAN_POINT('',(-73.2527445817597,-6.21935292074379,-0.000155149267013152));
#33004=CARTESIAN_POINT('',(-73.0062554182403,-6.21874727498198,5.02444159825033E-5));
#33005=CARTESIAN_POINT('',(-88.8777445817596,-6.21925,-6.18233832090354E-13));
#33006=CARTESIAN_POINT('Ctrl Pts',(-73.2527445817597,-6.21935292074379,
-0.000155149267012482));
#33007=CARTESIAN_POINT('Ctrl Pts',(-73.2461486481618,-6.21956430959384,
-0.206339320810795));
#33008=CARTESIAN_POINT('Ctrl Pts',(-73.2065234528251,-6.15917337788624,
-1.44487133897756));
#33009=CARTESIAN_POINT('Ctrl Pts',(-73.1338689957495,-5.3590851523311,-3.64697808548958));
#33010=CARTESIAN_POINT('Ctrl Pts',(-73.0347812105328,-2.96571815371499,
-5.7640921799276));
#33011=CARTESIAN_POINT('Ctrl Pts',(-72.9356934253162,0.148280150248475,
-6.48060613083523));
#33012=CARTESIAN_POINT('Ctrl Pts',(-72.8366056400995,3.22624828792765,-5.62241627866711));
#33013=CARTESIAN_POINT('Ctrl Pts',(-72.7375178548829,5.52027965393766,-3.3980517018284));
#33014=CARTESIAN_POINT('Ctrl Pts',(-72.6384300696661,6.47295417930641,-0.348004337008301));
#33015=CARTESIAN_POINT('Ctrl Pts',(-72.5393422844495,5.85278422724426,2.78660359852236));
#33016=CARTESIAN_POINT('Ctrl Pts',(-72.4402544992328,3.81046310673336,5.24410275816569));
#33017=CARTESIAN_POINT('Ctrl Pts',(-72.3411667140162,0.842248539758685,
6.42735250497835));
#33018=CARTESIAN_POINT('Ctrl Pts',(-72.2420789287994,-2.33062157207041,
6.04883839375603));
#33019=CARTESIAN_POINT('Ctrl Pts',(-72.1429911435828,-4.93718066622978,
4.20053447729974));
#33020=CARTESIAN_POINT('Ctrl Pts',(-72.0632130279028,-6.06990209169191,
1.89064539902266));
#33021=CARTESIAN_POINT('Ctrl Pts',(-72.0164641739618,-6.21897289391461,
0.429055152133518));
#33022=CARTESIAN_POINT('Ctrl Pts',(-72.0027445817596,-6.21878348465591,
7.77291339506408E-5));
#33023=CARTESIAN_POINT('Ctrl Pts',(-73.0062554182403,-6.21874727498198,
5.02444159830237E-5));
#33024=CARTESIAN_POINT('Ctrl Pts',(-72.9879789585214,-6.21858534952317,
-0.571418576758583));
#33025=CARTESIAN_POINT('Ctrl Pts',(-72.9366732370636,-5.9993684942345,-2.17576897141618));
#33026=CARTESIAN_POINT('Ctrl Pts',(-72.8523382538668,-4.63711226892121,
-4.52961725564207));
#33027=CARTESIAN_POINT('Ctrl Pts',(-72.7532504686503,-1.90979667128091,
-6.19458790813032));
#33028=CARTESIAN_POINT('Ctrl Pts',(-72.6541626834335,1.28157491443408,-6.35435350101671));
#33029=CARTESIAN_POINT('Ctrl Pts',(-72.5550748982169,4.16154030589149,-4.97009305341768));
#33030=CARTESIAN_POINT('Ctrl Pts',(-72.4559871130002,6.03030501425848,-2.37816402129864));
#33031=CARTESIAN_POINT('Ctrl Pts',(-72.3568993277835,6.4337832898522,0.791628231184674));
#33032=CARTESIAN_POINT('Ctrl Pts',(-72.2578115425668,5.27393510953157,3.76906502167849));
#33033=CARTESIAN_POINT('Ctrl Pts',(-72.1587237573503,2.83258863931502,5.83066756706414));
#33034=CARTESIAN_POINT('Ctrl Pts',(-72.0596359721335,-0.297040379296998,
6.47549300750585));
#33035=CARTESIAN_POINT('Ctrl Pts',(-71.9605481869169,-3.35449241237668,
5.54685706797077));
#33036=CARTESIAN_POINT('Ctrl Pts',(-71.8614604017001,-5.59684600365713,
3.27040631856919));
#33037=CARTESIAN_POINT('Ctrl Pts',(-71.7933628121413,-6.20326561309311,
1.15979613005301));
#33038=CARTESIAN_POINT('Ctrl Pts',(-71.7582944843214,-6.21976122515642,
0.0637936904746014));
#33039=CARTESIAN_POINT('Ctrl Pts',(-71.7562554182403,-6.21972691674719,
6.50263875293274E-5));
#33040=CARTESIAN_POINT('Origin',(-88.8777445817596,0.,0.));
#33041=CARTESIAN_POINT('',(-74.5027445817596,-6.21939977619133,0.000150774270671845));
#33042=CARTESIAN_POINT('',(-74.2562554182403,-6.21945322821522,-0.00014406247351606));
#33043=CARTESIAN_POINT('',(-88.8777445817596,-6.21925,-6.18233832090354E-13));
#33044=CARTESIAN_POINT('Ctrl Pts',(-74.5027445817597,-6.21939977619133,
0.000150774270671963));
#33045=CARTESIAN_POINT('Ctrl Pts',(-74.4758331223618,-6.21854665466753,
-0.841063946683904));
#33046=CARTESIAN_POINT('Ctrl Pts',(-74.4158924012251,-5.83566021064195,
-2.71548027997294));
#33047=CARTESIAN_POINT('Ctrl Pts',(-74.3229224183495,-4.00970737006563,
-5.09337703615375));
#33048=CARTESIAN_POINT('Ctrl Pts',(-74.2238346331329,-1.08929218333971,
-6.39012404928824));
#33049=CARTESIAN_POINT('Ctrl Pts',(-74.1247468479162,2.09580697107931,-6.13415323952314));
#33050=CARTESIAN_POINT('Ctrl Pts',(-74.0256590626996,4.77165203085921,-4.38766221607524));
#33051=CARTESIAN_POINT('Ctrl Pts',(-73.9265712774829,6.2880471181749,-1.5750257983885));
#33052=CARTESIAN_POINT('Ctrl Pts',(-73.8274834922662,6.27652776184059,1.62032159796177));
#33053=CARTESIAN_POINT('Ctrl Pts',(-73.7283957070496,4.73989301704688,4.42195171987746));
#33054=CARTESIAN_POINT('Ctrl Pts',(-73.6293079218328,2.05152533100835,6.1491045398666));
#33055=CARTESIAN_POINT('Ctrl Pts',(-73.5302201366162,-1.13533658159241,
6.38210417280031));
#33056=CARTESIAN_POINT('Ctrl Pts',(-73.4311323513995,-4.04632633089381,
5.06433470950454));
#33057=CARTESIAN_POINT('Ctrl Pts',(-73.3386404997806,-5.84578490937601,
2.68563123354285));
#33058=CARTESIAN_POINT('Ctrl Pts',(-73.2791779099007,-6.21850577594525,
0.826131802093192));
#33059=CARTESIAN_POINT('Ctrl Pts',(-73.2527445817597,-6.21935292074379,
-0.000155149267012482));
#33060=CARTESIAN_POINT('Ctrl Pts',(-74.2562554182403,-6.21945322821522,
-0.000144062473516251));
#33061=CARTESIAN_POINT('Ctrl Pts',(-74.2506926944603,-6.2196254798594,-0.17402274329055));
#33062=CARTESIAN_POINT('Ctrl Pts',(-74.2121007089414,-6.17004795161988,
-1.38022658464286));
#33063=CARTESIAN_POINT('Ctrl Pts',(-74.1404794616836,-5.41525391029054,
-3.5630419256968));
#33064=CARTESIAN_POINT('Ctrl Pts',(-74.0413916764669,-3.05516163314319,
-5.71718725183634));
#33065=CARTESIAN_POINT('Ctrl Pts',(-73.9423038912502,0.047295562592674,
-6.48212972771674));
#33066=CARTESIAN_POINT('Ctrl Pts',(-73.8432161060336,3.13826054590585,-5.67199818610696));
#33067=CARTESIAN_POINT('Ctrl Pts',(-73.744128320817,5.4666686453549,-3.48364415506002));
#33068=CARTESIAN_POINT('Ctrl Pts',(-73.6450405356003,6.4667466886019,-0.448809472545249));
#33069=CARTESIAN_POINT('Ctrl Pts',(-73.5459527503835,5.89548859469092,2.6950801299886));
#33070=CARTESIAN_POINT('Ctrl Pts',(-73.446864965167,3.89170272118268,5.18409998043338));
#33071=CARTESIAN_POINT('Ctrl Pts',(-73.3477771799502,0.94228322147271,6.4134503200478));
#33072=CARTESIAN_POINT('Ctrl Pts',(-73.2486893947337,-2.23609896204665,
6.0844148534698));
#33073=CARTESIAN_POINT('Ctrl Pts',(-73.1496016095169,-4.87113790444004,
4.27694496026283));
#33074=CARTESIAN_POINT('Ctrl Pts',(-73.0687902840191,-6.05484369252271,
1.95530053641333));
#33075=CARTESIAN_POINT('Ctrl Pts',(-73.0210082202603,-6.21887798159982,
0.46134124437055));
#33076=CARTESIAN_POINT('Ctrl Pts',(-73.0062554182403,-6.21874727498198,
5.02444159830237E-5));
#33077=CARTESIAN_POINT('Origin',(-88.8777445817596,0.,0.));
#33078=CARTESIAN_POINT('',(-75.7527445817596,-6.21876477465699,-6.52826263097299E-5));
#33079=CARTESIAN_POINT('',(-75.5062554182403,-6.21929810910058,0.000158575904569969));
#33080=CARTESIAN_POINT('',(-88.8777445817596,-6.21925,-6.18233832090354E-13));
#33081=CARTESIAN_POINT('Ctrl Pts',(-75.7527445817597,-6.21876477465699,
-6.52826263093653E-5));
#33082=CARTESIAN_POINT('Ctrl Pts',(-75.7385468583008,-6.21892878036616,
-0.443996499890235));
#33083=CARTESIAN_POINT('Ctrl Pts',(-75.691319873103,-6.06300112700048,-1.92056570481116));
#33084=CARTESIAN_POINT('Ctrl Pts',(-75.6110636261662,-4.90676653851619,
-4.23602230429382));
#33085=CARTESIAN_POINT('Ctrl Pts',(-75.5119758409496,-2.28694894755983,
-6.06548492185348));
#33086=CARTESIAN_POINT('Ctrl Pts',(-75.4128880557329,0.888567775924808,
-6.42111284230117));
#33087=CARTESIAN_POINT('Ctrl Pts',(-75.3138002705162,3.84817397687645,-5.21649306236172));
#33088=CARTESIAN_POINT('Ctrl Pts',(-75.2147124852996,5.87272347573166,-2.7443326699887));
#33089=CARTESIAN_POINT('Ctrl Pts',(-75.1156247000829,6.47027682562396,0.394665207195212));
#33090=CARTESIAN_POINT('Ctrl Pts',(-75.0165369148663,5.49563626053907,3.43776452332399));
#33091=CARTESIAN_POINT('Ctrl Pts',(-74.9174491296495,3.18562688193913,5.64553134745027));
#33092=CARTESIAN_POINT('Ctrl Pts',(-74.8183613444329,0.101551210018007,
6.48150678297269));
#33093=CARTESIAN_POINT('Ctrl Pts',(-74.7192735592163,-3.00720009769922,
5.74255956855258));
#33094=CARTESIAN_POINT('Ctrl Pts',(-74.6201857739996,-5.38524052207403,
3.60824435777137));
#33095=CARTESIAN_POINT('Ctrl Pts',(-74.5480094481807,-6.16427011766636,
1.41495563973138));
#33096=CARTESIAN_POINT('Ctrl Pts',(-74.5088623841007,-6.21959371695011,
0.191384750590594));
#33097=CARTESIAN_POINT('Ctrl Pts',(-74.5027445817597,-6.21939977619133,
0.000150774270671963));
#33098=CARTESIAN_POINT('Ctrl Pts',(-75.5062554182403,-6.21929810910058,
0.000158575904569969));
#33099=CARTESIAN_POINT('Ctrl Pts',(-75.4803771686603,-6.21846650667767,
-0.808797549377969));
#33100=CARTESIAN_POINT('Ctrl Pts',(-75.4214696573415,-5.85738026136393,
-2.65097162487408));
#33101=CARTESIAN_POINT('Ctrl Pts',(-75.3295328842836,-4.08857452377673,
-5.03028836556254));
#33102=CARTESIAN_POINT('Ctrl Pts',(-75.230445099067,-1.18871686815845,-6.37237749074438));
#33103=CARTESIAN_POINT('Ctrl Pts',(-75.1313573138503,1.99998367272066,-6.1660609781319));
#33104=CARTESIAN_POINT('Ctrl Pts',(-75.0322695286336,4.70271394601358,-4.46147108240762));
#33105=CARTESIAN_POINT('Ctrl Pts',(-74.933181743417,6.26274531336161,-1.67280118877204));
#33106=CARTESIAN_POINT('Ctrl Pts',(-74.8340939582003,6.30101024967761,1.52233784379415));
#33107=CARTESIAN_POINT('Ctrl Pts',(-74.7350061729836,4.8082108683866,4.34756839190818));
#33108=CARTESIAN_POINT('Ctrl Pts',(-74.635918387767,2.14707818808318,6.11639582854541));
#33109=CARTESIAN_POINT('Ctrl Pts',(-74.5368306025503,-1.03576683208741,
6.39901787360667));
#33110=CARTESIAN_POINT('Ctrl Pts',(-74.4377428173336,-3.96693385537629,
5.1267610110341));
#33111=CARTESIAN_POINT('Ctrl Pts',(-74.344217755897,-5.82374674154208,2.75012579862636));
#33112=CARTESIAN_POINT('Ctrl Pts',(-74.2837219561992,-6.21860271747436,
0.858400344144813));
#33113=CARTESIAN_POINT('Ctrl Pts',(-74.2562554182403,-6.21945322821522,
-0.000144062473516251));
#33114=CARTESIAN_POINT('Origin',(-88.8777445817596,0.,0.));
#33115=CARTESIAN_POINT('',(-77.0027445817596,-6.21975224382197,-4.80951439556949E-5));
#33116=CARTESIAN_POINT('',(-76.7562554182403,-6.21880928941777,-9.14614924069079E-5));
#33117=CARTESIAN_POINT('',(-88.8777445817596,-6.21925,-6.18233832090354E-13));
#33118=CARTESIAN_POINT('Ctrl Pts',(-77.0027445817596,-6.21975224382197,
-4.80951439554757E-5));
#33119=CARTESIAN_POINT('Ctrl Pts',(-77.0012605942396,-6.21977142923684,
-0.0464278686673888));
#33120=CARTESIAN_POINT('Ctrl Pts',(-76.9667473449807,-6.20795725940526,
-1.12507719611085));
#33121=CARTESIAN_POINT('Ctrl Pts',(-76.899204833983,-5.6240241962828,-3.22344453428357));
#33122=CARTESIAN_POINT('Ctrl Pts',(-76.8001170487663,-3.40080370644699,
-5.51858468959146));
#33123=CARTESIAN_POINT('Ctrl Pts',(-76.7010292635497,-0.351231726960331,
-6.47277985875879));
#33124=CARTESIAN_POINT('Ctrl Pts',(-76.6019414783329,2.78368503741827,-5.85417290814259));
#33125=CARTESIAN_POINT('Ctrl Pts',(-76.5028536931163,5.24220219865931,-3.81307735750908));
#33126=CARTESIAN_POINT('Ctrl Pts',(-76.4037659078996,6.42693175854569,-0.845453131151542));
#33127=CARTESIAN_POINT('Ctrl Pts',(-76.304678122683,6.04999969635994,2.32760531448557));
#33128=CARTESIAN_POINT('Ctrl Pts',(-76.2055903374662,4.20299564736804,4.93508565418903));
#33129=CARTESIAN_POINT('Ctrl Pts',(-76.1065025522496,1.3347178013573,6.34340375640058));
#33130=CARTESIAN_POINT('Ctrl Pts',(-76.0074147670329,-1.85787927581762,
6.21035646500782));
#33131=CARTESIAN_POINT('Ctrl Pts',(-75.9083269818163,-4.59903562318709,
4.56827255783114));
#33132=CARTESIAN_POINT('Ctrl Pts',(-75.8234369200585,-5.99004202451095,
2.21049216915895));
#33133=CARTESIAN_POINT('Ctrl Pts',(-75.7715761200396,-6.21854724120529,
0.58875501210554));
#33134=CARTESIAN_POINT('Ctrl Pts',(-75.7527445817597,-6.21876477465699,
-6.52826263093653E-5));
#33135=CARTESIAN_POINT('Ctrl Pts',(-76.7562554182403,-6.21880928941777,
-9.14614924065957E-5));
#33136=CARTESIAN_POINT('Ctrl Pts',(-76.7430909045993,-6.2190242752516,-0.411708070281631));
#33137=CARTESIAN_POINT('Ctrl Pts',(-76.6968971292193,-6.07776826767591,
-1.85590942897543));
#33138=CARTESIAN_POINT('Ctrl Pts',(-76.6176740921003,-4.97216739135669,
-4.15906168618827));
#33139=CARTESIAN_POINT('Ctrl Pts',(-76.5185863068837,-2.38117045277481,
-6.02911850538885));
#33140=CARTESIAN_POINT('Ctrl Pts',(-76.419498521667,0.788420230289574,-6.43417719818628));
#33141=CARTESIAN_POINT('Ctrl Pts',(-76.3204107364504,3.76643495425477,-5.27581372041868));
#33142=CARTESIAN_POINT('Ctrl Pts',(-76.2213229512337,5.82925450561374,-2.83549547451091));
#33143=CARTESIAN_POINT('Ctrl Pts',(-76.122235166017,6.47564030775746,0.293811643297502));
#33144=CARTESIAN_POINT('Ctrl Pts',(-76.0231473808003,5.54852893786079,3.3517263168271));
#33145=CARTESIAN_POINT('Ctrl Pts',(-75.9240595955837,3.27319651525233,5.59521467414165));
#33146=CARTESIAN_POINT('Ctrl Pts',(-75.824971810367,0.202519506547572,6.47913794625935));
#33147=CARTESIAN_POINT('Ctrl Pts',(-75.7258840251503,-2.91736713328106,
5.78871416523925));
#33148=CARTESIAN_POINT('Ctrl Pts',(-75.6267962399337,-5.32837114284346,
3.69170741545199));
#33149=CARTESIAN_POINT('Ctrl Pts',(-75.553586704297,-6.15311687587124,1.47960248994997));
#33150=CARTESIAN_POINT('Ctrl Pts',(-75.5134064303992,-6.21952790822279,
0.2236997806532));
#33151=CARTESIAN_POINT('Ctrl Pts',(-75.5062554182403,-6.21929810910058,
0.000158575904569969));
#33152=CARTESIAN_POINT('Origin',(-88.8777445817596,0.,0.));
#33153=CARTESIAN_POINT('',(-78.2527445817596,-6.21893077709273,0.000131417006590163));
#33154=CARTESIAN_POINT('',(-78.0062554182403,-6.2197799278902,-1.48610517280989E-5));
#33155=CARTESIAN_POINT('',(-88.8777445817596,-6.21925,-6.18233832090354E-13));
#33156=CARTESIAN_POINT('Ctrl Pts',(-78.2527445817597,-6.21893077709273,
0.000131417006590355));
#33157=CARTESIAN_POINT('Ctrl Pts',(-78.2309450684397,-6.218405642012,-0.681438740356712));
#33158=CARTESIAN_POINT('Ctrl Pts',(-78.1761162933808,-5.93741656761277,
-2.39610387996943));
#33159=CARTESIAN_POINT('Ctrl Pts',(-78.088258256583,-4.39004082983858,-4.76946373697579));
#33160=CARTESIAN_POINT('Ctrl Pts',(-77.9891704713664,-1.57816084063661,
-6.2872610242504));
#33161=CARTESIAN_POINT('Ctrl Pts',(-77.8900826861497,1.61719190210787,-6.27733487857178));
#33162=CARTESIAN_POINT('Ctrl Pts',(-77.790994900933,4.41958784619184,-4.74209722546579));
#33163=CARTESIAN_POINT('Ctrl Pts',(-77.6919071157163,6.14808087920214,-2.05459103686501));
#33164=CARTESIAN_POINT('Ctrl Pts',(-77.5928193304997,6.3826694615111,1.13215430532706));
#33165=CARTESIAN_POINT('Ctrl Pts',(-77.493731545283,5.06635158971623,4.04380073635643));
#33166=CARTESIAN_POINT('Ctrl Pts',(-77.3946437600663,2.51897554913599,5.97285568290681));
#33167=CARTESIAN_POINT('Ctrl Pts',(-77.2955559748497,-0.640479099061789,
6.45058364410864));
#33168=CARTESIAN_POINT('Ctrl Pts',(-77.196468189633,-3.64430557719005,5.36090287974316));
#33169=CARTESIAN_POINT('Ctrl Pts',(-77.0988643919364,-5.73088793552195,
3.00442020811975));
#33170=CARTESIAN_POINT('Ctrl Pts',(-77.0342898559785,-6.21934441749918,
0.985851485745715));
#33171=CARTESIAN_POINT('Ctrl Pts',(-77.0027445817596,-6.21975224382197,
-4.80951439554757E-5));
#33172=CARTESIAN_POINT('Ctrl Pts',(-78.0062554182403,-6.2197799278902,-1.4861051727765E-5));
#33173=CARTESIAN_POINT('Ctrl Pts',(-78.0058046405381,-6.21978187756921,
-0.0141030499939625));
#33174=CARTESIAN_POINT('Ctrl Pts',(-77.9723246010971,-6.21630091181974,
-1.06045623693887));
#33175=CARTESIAN_POINT('Ctrl Pts',(-77.9058152999171,-5.67356222662317,
-3.13543208152));
#33176=CARTESIAN_POINT('Ctrl Pts',(-77.8067275147004,-3.48636941843915,
-5.46493101103411));
#33177=CARTESIAN_POINT('Ctrl Pts',(-77.7076397294838,-0.452033754894525,
-6.46652210710101));
#33178=CARTESIAN_POINT('Ctrl Pts',(-77.608551944267,2.69214028774311,-5.89683163642142));
#33179=CARTESIAN_POINT('Ctrl Pts',(-77.5094641590505,5.18215892208465,-3.89428704430587));
#33180=CARTESIAN_POINT('Ctrl Pts',(-77.4103763738337,6.41297969776877,-0.945480868762339));
#33181=CARTESIAN_POINT('Ctrl Pts',(-77.3112885886171,6.08552902241152,2.23306497768811));
#33182=CARTESIAN_POINT('Ctrl Pts',(-77.2122008034003,4.27937319172577,4.8690048021263));
#33183=CARTESIAN_POINT('Ctrl Pts',(-77.1131130181838,1.43338480467962,6.32183918483408));
#33184=CARTESIAN_POINT('Ctrl Pts',(-77.014025232967,-1.76089762425562,6.2385480870216));
#33185=CARTESIAN_POINT('Ctrl Pts',(-76.9149374477504,-4.52730461534429,
4.63937017245579));
#33186=CARTESIAN_POINT('Ctrl Pts',(-76.8290141761748,-5.9722511339069,2.2751179173021));
#33187=CARTESIAN_POINT('Ctrl Pts',(-76.7761201663381,-6.21848488400865,
0.621022274220235));
#33188=CARTESIAN_POINT('Ctrl Pts',(-76.7562554182403,-6.21880928941777,
-9.14614924065957E-5));
#33189=CARTESIAN_POINT('Origin',(-88.8777445817596,0.,0.));
#33190=CARTESIAN_POINT('',(-79.5027445817596,-6.21911133157867,-0.000156735226100492));
#33191=CARTESIAN_POINT('',(-79.2562554182404,-6.21886011839245,0.000111780172469961));
#33192=CARTESIAN_POINT('',(-88.8777445817596,-6.21925,-6.18233832090354E-13));
#33193=CARTESIAN_POINT('Ctrl Pts',(-79.5027445817596,-6.21911133157867,
-0.00015673522610081));
#33194=CARTESIAN_POINT('Ctrl Pts',(-79.4936588043785,-6.21938423771565,
-0.284203389274524));
#33195=CARTESIAN_POINT('Ctrl Pts',(-79.4515437652585,-6.13082844877969,
-1.60066773865356));
#33196=CARTESIAN_POINT('Ctrl Pts',(-79.3763994643998,-5.21841112433719,
-3.84557254038601));
#33197=CARTESIAN_POINT('Ctrl Pts',(-79.2773116791831,-2.7472604853497,-5.87135441372885));
#33198=CARTESIAN_POINT('Ctrl Pts',(-79.1782238939664,0.391439059863712,
-6.47047280253847));
#33199=CARTESIAN_POINT('Ctrl Pts',(-79.0791361087498,3.43502395626256,-5.49734965650533));
#33200=CARTESIAN_POINT('Ctrl Pts',(-78.980048323533,5.64394228314933,-3.18844136381023));
#33201=CARTESIAN_POINT('Ctrl Pts',(-78.8809605383164,6.48145534358615,-0.104782894956996));
#33202=CARTESIAN_POINT('Ctrl Pts',(-78.7818727530997,5.74405825318873,3.00433646750017));
#33203=CARTESIAN_POINT('Ctrl Pts',(-78.682784967883,3.61092900537051,5.38344077186245));
#33204=CARTESIAN_POINT('Ctrl Pts',(-78.5836971826664,0.600390527212153,
6.45443832109432));
#33205=CARTESIAN_POINT('Ctrl Pts',(-78.4846093974497,-2.55603511449917,
5.9570905079094));
#33206=CARTESIAN_POINT('Ctrl Pts',(-78.3855216122331,-5.09137715163132,
4.01224644380471));
#33207=CARTESIAN_POINT('Ctrl Pts',(-78.3082333403363,-6.10397284759602,
1.73483310960994));
#33208=CARTESIAN_POINT('Ctrl Pts',(-78.2639743301786,-6.21920129390455,
0.351233814784175));
#33209=CARTESIAN_POINT('Ctrl Pts',(-78.2527445817597,-6.21893077709273,
0.000131417006590355));
#33210=CARTESIAN_POINT('Ctrl Pts',(-79.2562554182403,-6.21886011839245,
0.000111780172470065));
#33211=CARTESIAN_POINT('Ctrl Pts',(-79.2354891147382,-6.21844119785085,
-0.649175810843478));
#33212=CARTESIAN_POINT('Ctrl Pts',(-79.181693549497,-5.95626667819782,-2.33150006579333));
#33213=CARTESIAN_POINT('Ctrl Pts',(-79.0948687225172,-4.46381531427285,
-4.7004888593904));
#33214=CARTESIAN_POINT('Ctrl Pts',(-78.9957809373004,-1.67592360331519,
-6.26191047149678));
#33215=CARTESIAN_POINT('Ctrl Pts',(-78.8966931520838,1.5191959530824,-6.30176850838938));
#33216=CARTESIAN_POINT('Ctrl Pts',(-78.797605366867,4.34517046399522,-4.81037798057634));
#33217=CARTESIAN_POINT('Ctrl Pts',(-78.6985175816505,6.11532452902266,-2.15012757340671));
#33218=CARTESIAN_POINT('Ctrl Pts',(-78.5994297964337,6.39953351445713,1.03257613497986));
#33219=CARTESIAN_POINT('Ctrl Pts',(-78.5003420112172,5.12873829817387,3.96437714477757));
#33220=CARTESIAN_POINT('Ctrl Pts',(-78.4012542260003,2.61172574664976,5.93288557967174));
#33221=CARTESIAN_POINT('Ctrl Pts',(-78.3021664407838,-0.539902515628905,
6.45977924938676));
#33222=CARTESIAN_POINT('Ctrl Pts',(-78.2030786555671,-3.5603414219296,5.41702977991466));
#33223=CARTESIAN_POINT('Ctrl Pts',(-78.1044416480526,-5.70585807478664,
3.06874368313118));
#33224=CARTESIAN_POINT('Ctrl Pts',(-78.038833902277,-6.21963902121677,1.01816291553709));
#33225=CARTESIAN_POINT('Ctrl Pts',(-78.0062554182403,-6.2197799278902,-1.4861051727765E-5));
#33226=CARTESIAN_POINT('Origin',(-88.8777445817596,0.,0.));
#33227=CARTESIAN_POINT('',(-80.7527445817596,-6.21962280111477,0.000107712410215426));
#33228=CARTESIAN_POINT('',(-80.5062554182403,-6.21920956565303,-0.00016035455149499));
#33229=CARTESIAN_POINT('',(-88.8777445817596,-6.21925,-6.18233832090354E-13));
#33230=CARTESIAN_POINT('Ctrl Pts',(-80.7527445817596,-6.21962280111477,
0.000107712410215288));
#33231=CARTESIAN_POINT('Ctrl Pts',(-80.7233432785786,-6.2188772365995,-0.91884081869823));
#33232=CARTESIAN_POINT('Ctrl Pts',(-80.6609127136587,-5.78087320937469,
-2.87081814951415));
#33233=CARTESIAN_POINT('Ctrl Pts',(-80.5654528869998,-3.81569066033551,
-5.24030033591639));
#33234=CARTESIAN_POINT('Ctrl Pts',(-80.4663651017831,-0.84865751236067,
-6.42650941434701));
#33235=CARTESIAN_POINT('Ctrl Pts',(-80.3672773165665,2.32458847824698,-6.05115949490496));
#33236=CARTESIAN_POINT('Ctrl Pts',(-80.2681895313497,4.9329894152624,-4.20545577255142));
#33237=CARTESIAN_POINT('Ctrl Pts',(-80.1691017461332,6.34273747384018,-1.33788047445222));
#33238=CARTESIAN_POINT('Ctrl Pts',(-80.0700139609164,6.21128203689244,1.85478254362996));
#33239=CARTESIAN_POINT('Ctrl Pts',(-79.9709261756998,4.57056508211651,4.59675729793451));
#33240=CARTESIAN_POINT('Ctrl Pts',(-79.871838390483,1.81925969290868,6.22177924678583));
#33241=CARTESIAN_POINT('Ctrl Pts',(-79.7727506052665,-1.37410236497632,
6.3349889910357));
#33242=CARTESIAN_POINT('Ctrl Pts',(-79.6736628200496,-4.23357525011125,
4.90887802126133));
#33243=CARTESIAN_POINT('Ctrl Pts',(-79.5836608122142,-5.89647298261668,
2.53011139605932));
#33244=CARTESIAN_POINT('Ctrl Pts',(-79.5266880661174,-6.21839214998882,
0.748383134600084));
#33245=CARTESIAN_POINT('Ctrl Pts',(-79.5027445817596,-6.21911133157867,
-0.00015673522610081));
#33246=CARTESIAN_POINT('Ctrl Pts',(-80.5062554182403,-6.21920956565303,
-0.000160354551495372));
#33247=CARTESIAN_POINT('Ctrl Pts',(-80.498202850677,-6.2194640039143,-0.251894566613715));
#33248=CARTESIAN_POINT('Ctrl Pts',(-80.4571210213749,-6.14295939465773,
-1.53601476073233));
#33249=CARTESIAN_POINT('Ctrl Pts',(-80.3830099303339,-5.27769101971328,
-3.76380395047722));
#33250=CARTESIAN_POINT('Ctrl Pts',(-80.2839221451171,-2.83840160478908,
-5.82783999498278));
#33251=CARTESIAN_POINT('Ctrl Pts',(-80.1848343599005,0.290582834254973,
-6.47578599813385));
#33252=CARTESIAN_POINT('Ctrl Pts',(-80.0857465746839,3.34895938802227,-5.55019942835999));
#33253=CARTESIAN_POINT('Ctrl Pts',(-79.9866587894671,5.59358195362901,-3.27598589820315));
#33254=CARTESIAN_POINT('Ctrl Pts',(-79.8875710042505,6.47903616408986,-0.205749997827326));
#33255=CARTESIAN_POINT('Ctrl Pts',(-79.7884832190337,5.79016805316885,2.91448050143638));
#33256=CARTESIAN_POINT('Ctrl Pts',(-79.6893954338172,3.69436369744359,5.32652978478494));
#33257=CARTESIAN_POINT('Ctrl Pts',(-79.5903076486004,0.700876556055815,
6.44430094970444));
#33258=CARTESIAN_POINT('Ctrl Pts',(-79.4912198633839,-2.46291455937789,
5.99619000285969));
#33259=CARTESIAN_POINT('Ctrl Pts',(-79.392132078167,-5.0282491654969,4.09108213152337));
#33260=CARTESIAN_POINT('Ctrl Pts',(-79.3138105964527,-6.09021294666528,
1.79949079884625));
#33261=CARTESIAN_POINT('Ctrl Pts',(-79.2685183764771,-6.21910750017158,
0.383530360730315));
#33262=CARTESIAN_POINT('Ctrl Pts',(-79.2562554182403,-6.21886011839245,
0.000111780172470065));
#33263=CARTESIAN_POINT('Origin',(-88.8777445817596,0.,0.));
#33264=CARTESIAN_POINT('',(-82.0027445817596,-6.21872329644988,5.01257785865963E-6));
#33265=CARTESIAN_POINT('',(-81.7562554182403,-6.21953636931397,0.000129532949082536));
#33266=CARTESIAN_POINT('',(-88.8777445817596,-6.21925,-6.18233832090354E-13));
#33267=CARTESIAN_POINT('Ctrl Pts',(-82.0027445817597,-6.21872329644988,
5.01257785858605E-6));
#33268=CARTESIAN_POINT('Ctrl Pts',(-81.9860570145175,-6.21870861559184,
-0.521788036686013));
#33269=CARTESIAN_POINT('Ctrl Pts',(-81.9363401855364,-6.02517739221427,
-2.07636300232439));
#33270=CARTESIAN_POINT('Ctrl Pts',(-81.8535940948165,-4.74430025497663,
-4.41722287377553));
#33271=CARTESIAN_POINT('Ctrl Pts',(-81.7545063095999,-2.0576562319405,-6.14705569009534));
#33272=CARTESIAN_POINT('Ctrl Pts',(-81.6554185243831,1.12897174760274,-6.3832331634597));
#33273=CARTESIAN_POINT('Ctrl Pts',(-81.5563307391665,4.04127413651083,-5.06836721040866));
#33274=CARTESIAN_POINT('Ctrl Pts',(-81.4572429539498,5.97159897215335,-2.52195331871032));
#33275=CARTESIAN_POINT('Ctrl Pts',(-81.3581551687331,6.45090218697082,0.637262740250864));
#33276=CARTESIAN_POINT('Ctrl Pts',(-81.2590673835165,5.36271927440909,3.64163216289869));
#33277=CARTESIAN_POINT('Ctrl Pts',(-81.1599795982997,2.97146466365244,5.76113188346196));
#33278=CARTESIAN_POINT('Ctrl Pts',(-81.0608918130833,-0.141817580336693,
6.48075077439986));
#33279=CARTESIAN_POINT('Ctrl Pts',(-80.9618040278663,-3.22063997927572,
5.62563071573915));
#33280=CARTESIAN_POINT('Ctrl Pts',(-80.8627162426499,-5.5168883532987,3.4035548656095));
#33281=CARTESIAN_POINT('Ctrl Pts',(-80.7930297606142,-6.18902423921956,
1.25918599373804));
#33282=CARTESIAN_POINT('Ctrl Pts',(-80.7563725403174,-6.21971479966146,
0.113500889818269));
#33283=CARTESIAN_POINT('Ctrl Pts',(-80.7527445817596,-6.21962280111477,
0.000107712410215288));
#33284=CARTESIAN_POINT('Ctrl Pts',(-81.7562554182403,-6.21953636931396,
0.000129532949082693));
#33285=CARTESIAN_POINT('Ctrl Pts',(-81.7278873248771,-6.21871470310021,
-0.886561297176356));
#33286=CARTESIAN_POINT('Ctrl Pts',(-81.6664899697749,-5.80403033309651,
-2.80637919144345));
#33287=CARTESIAN_POINT('Ctrl Pts',(-81.5720633529339,-3.89687039929076,
-5.18021657542632));
#33288=CARTESIAN_POINT('Ctrl Pts',(-81.4729755677172,-0.948678281001003,
-6.41250748119229));
#33289=CARTESIAN_POINT('Ctrl Pts',(-81.3738877825005,2.23003043817884,-6.08664167846161));
#33290=CARTESIAN_POINT('Ctrl Pts',(-81.274799997284,4.86687048935458,-4.28180035931612));
#33291=CARTESIAN_POINT('Ctrl Pts',(-81.1757122120671,6.32112370930806,-1.43653671335388));
#33292=CARTESIAN_POINT('Ctrl Pts',(-81.0766244268506,6.23942530007697,1.75778684770072));
#33293=CARTESIAN_POINT('Ctrl Pts',(-80.9775366416338,4.64162692262079,4.52499084953681));
#33294=CARTESIAN_POINT('Ctrl Pts',(-80.8784488564173,1.91597299894771,6.19268036834564));
#33295=CARTESIAN_POINT('Ctrl Pts',(-80.7793610712004,-1.27523768085627,
6.35562833514629));
#33296=CARTESIAN_POINT('Ctrl Pts',(-80.6802732859839,-4.15658203252233,
4.97424049319116));
#33297=CARTESIAN_POINT('Ctrl Pts',(-80.5892380683304,-5.87585161207603,
2.59466305334264));
#33298=CARTESIAN_POINT('Ctrl Pts',(-80.5312321124159,-6.21842037306466,
0.780645069160635));
#33299=CARTESIAN_POINT('Ctrl Pts',(-80.5062554182403,-6.21920956565303,
-0.000160354551495372));
#33300=CARTESIAN_POINT('Origin',(-88.8777445817596,0.,0.));
#33301=CARTESIAN_POINT('',(-83.2527445817597,-6.21959518121893,-0.000115596989317509));
#33302=CARTESIAN_POINT('',(-83.0062554182403,-6.21872885219791,-2.48421024784395E-5));
#33303=CARTESIAN_POINT('',(-88.8777445817596,-6.21925,-6.18233832090354E-13));
#33304=CARTESIAN_POINT('Ctrl Pts',(-83.2527445817596,-6.21959518121893,
-0.000115596989317054));
#33305=CARTESIAN_POINT('Ctrl Pts',(-83.2487707504564,-6.21970139409347,
-0.124320751295493));
#33306=CARTESIAN_POINT('Ctrl Pts',(-83.2117676574143,-6.18576408699328,
-1.2808228962477));
#33307=CARTESIAN_POINT('Ctrl Pts',(-83.1417353026332,-5.49906168580417,
-3.43228253523767));
#33308=CARTESIAN_POINT('Ctrl Pts',(-83.0426475174165,-3.19125505301957,
-5.64235181573731));
#33309=CARTESIAN_POINT('Ctrl Pts',(-82.9435597321999,-0.108014553846464,
-6.48140229287878));
#33310=CARTESIAN_POINT('Ctrl Pts',(-82.8444719469832,3.0014720904087,-5.7455555098245));
#33311=CARTESIAN_POINT('Ctrl Pts',(-82.7453841617665,5.38163968330173,-3.61361275527539));
#33312=CARTESIAN_POINT('Ctrl Pts',(-82.6462963765498,6.45413816238201,-0.603608653732817));
#33313=CARTESIAN_POINT('Ctrl Pts',(-82.5472085913332,5.95836421374577,2.5530645746496));
#33314=CARTESIAN_POINT('Ctrl Pts',(-82.4481208061165,4.01478452008011,5.08937600136816));
#33315=CARTESIAN_POINT('Ctrl Pts',(-82.3490330208998,1.0956639086878,6.38903462388301));
#33316=CARTESIAN_POINT('Ctrl Pts',(-82.2499452356833,-2.08968891757316,
6.13624013983718));
#33317=CARTESIAN_POINT('Ctrl Pts',(-82.1508574504665,-4.76727425738086,
4.39241835221678));
#33318=CARTESIAN_POINT('Ctrl Pts',(-82.068457232492,-6.03062208101894,2.05472217656536));
#33319=CARTESIAN_POINT('Ctrl Pts',(-82.0190862762564,-6.21873767302698,
0.510983184401946));
#33320=CARTESIAN_POINT('Ctrl Pts',(-82.0027445817597,-6.21872329644988,
5.01257785858605E-6));
#33321=CARTESIAN_POINT('Ctrl Pts',(-83.0062554182404,-6.21872885219791,
-2.48421024784395E-5));
#33322=CARTESIAN_POINT('Ctrl Pts',(-82.990601060816,-6.21879717894966,-0.489509848776858));
#33323=CARTESIAN_POINT('Ctrl Pts',(-82.9419174416527,-6.04125906635289,
-2.01171468559772));
#33324=CARTESIAN_POINT('Ctrl Pts',(-82.8602045607506,-4.8125438968831,-4.34277145585205));
#33325=CARTESIAN_POINT('Ctrl Pts',(-82.7611167755339,-2.15317642419824,
-6.11425170920097));
#33326=CARTESIAN_POINT('Ctrl Pts',(-82.6620289903173,1.02938518116893,-6.40004756435293));
#33327=CARTESIAN_POINT('Ctrl Pts',(-82.5629412051006,3.96181944861569,-5.13071431028474));
#33328=CARTESIAN_POINT('Ctrl Pts',(-82.4638534198839,5.93158262837659,-2.61468357548884));
#33329=CARTESIAN_POINT('Ctrl Pts',(-82.3647656346672,6.46004764333774,0.536681584365129));
#33330=CARTESIAN_POINT('Ctrl Pts',(-82.2656778494506,5.41880430283928,3.55764003304445));
#33331=CARTESIAN_POINT('Ctrl Pts',(-82.1665900642338,3.06086132475543,5.71413778516117));
#33332=CARTESIAN_POINT('Ctrl Pts',(-82.0675022790172,-0.0408315235521791,
6.4821736681359));
#33333=CARTESIAN_POINT('Ctrl Pts',(-81.9684144938005,-3.13260283765064,
5.67512485666467));
#33334=CARTESIAN_POINT('Ctrl Pts',(-81.8693267085839,-5.46319201810528,
3.48909381509022));
#33335=CARTESIAN_POINT('Ctrl Pts',(-81.7986070167305,-6.17911475814637,
1.32382249712401));
#33336=CARTESIAN_POINT('Ctrl Pts',(-81.760916586616,-6.219671377491,0.145821920640187));
#33337=CARTESIAN_POINT('Ctrl Pts',(-81.7562554182403,-6.21953636931396,
0.000129532949082693));
#33338=CARTESIAN_POINT('Origin',(-88.8777445817596,0.,0.));
#33339=CARTESIAN_POINT('',(-84.5027445817596,-6.21914365535479,0.000158605856680488));
#33340=CARTESIAN_POINT('',(-84.2562554182403,-6.21967289644367,-9.04560928893794E-5));
#33341=CARTESIAN_POINT('',(-88.8777445817596,-6.21925,-6.18233832090354E-13));
#33342=CARTESIAN_POINT('Ctrl Pts',(-84.5027445817596,-6.21914365535479,
0.000158605856680621));
#33343=CARTESIAN_POINT('Ctrl Pts',(-84.4784552246564,-6.21839883607971,
-0.759182867613572));
#33344=CARTESIAN_POINT('Ctrl Pts',(-84.4211366058144,-5.8896347122068,-2.55172269859188));
#33345=CARTESIAN_POINT('Ctrl Pts',(-84.3307887252331,-4.20791485226097,
-4.93089194986176));
#33346=CARTESIAN_POINT('Ctrl Pts',(-84.2317009400167,-1.34104281493249,
-6.34206961449874));
#33347=CARTESIAN_POINT('Ctrl Pts',(-84.1326131547998,1.85168535032901,-6.21220606459603));
#33348=CARTESIAN_POINT('Ctrl Pts',(-84.0335253695833,4.59447782990876,-4.57285647015062));
#33349=CARTESIAN_POINT('Ctrl Pts',(-83.9344375843666,6.22087138538862,-1.82236166344391));
#33350=CARTESIAN_POINT('Ctrl Pts',(-83.8353497991498,6.33567333489668,1.37094355079113));
#33351=CARTESIAN_POINT('Ctrl Pts',(-83.7362620139334,4.91098828363557,4.23112714344313));
#33352=CARTESIAN_POINT('Ctrl Pts',(-83.6371742287164,2.29299634549289,6.06320134792872));
#33353=CARTESIAN_POINT('Ctrl Pts',(-83.5380864435,-0.8821641649706,6.4219957343511));
#33354=CARTESIAN_POINT('Ctrl Pts',(-83.4389986582831,-3.84297014786777,
5.22032788899049));
#33355=CARTESIAN_POINT('Ctrl Pts',(-83.3438847043698,-5.78869223083908,
2.84925049123928));
#33356=CARTESIAN_POINT('Ctrl Pts',(-83.2818000121953,-6.21881858539693,
0.908034232556073));
#33357=CARTESIAN_POINT('Ctrl Pts',(-83.2527445817596,-6.21959518121893,
-0.000115596989317054));
#33358=CARTESIAN_POINT('Ctrl Pts',(-84.2562554182403,-6.21967289644367,
-9.04560928895008E-5));
#33359=CARTESIAN_POINT('Ctrl Pts',(-84.2533147967549,-6.2197379703033,-0.0919985144304947));
#33360=CARTESIAN_POINT('Ctrl Pts',(-84.2173449135305,-6.19533287709085,
-1.21618959255704));
#33361=CARTESIAN_POINT('Ctrl Pts',(-84.1483457685672,-5.55186853905296,
-3.34619162665173));
#33362=CARTESIAN_POINT('Ctrl Pts',(-84.0492579833507,-3.27877446672824,
-5.59194784252432));
#33363=CARTESIAN_POINT('Ctrl Pts',(-83.950170198134,-0.208980437956675,
-6.47893277120133));
#33364=CARTESIAN_POINT('Ctrl Pts',(-83.8510824129173,2.91159314503785,-5.79162050163479));
#33365=CARTESIAN_POINT('Ctrl Pts',(-83.7519946277006,5.32468710252559,-3.6970190609988));
#33366=CARTESIAN_POINT('Ctrl Pts',(-83.652906842484,6.44395068963483,-0.704089615563853));
#33367=CARTESIAN_POINT('Ctrl Pts',(-83.5538190572673,5.9974172736645,2.4599245359849));
#33368=CARTESIAN_POINT('Ctrl Pts',(-83.4547312720506,4.09358872220742,5.02620871538443));
#33369=CARTESIAN_POINT('Ctrl Pts',(-83.3556434868339,1.19507084710563,6.37118892731869));
#33370=CARTESIAN_POINT('Ctrl Pts',(-83.2565557016173,-1.99383384828571,
6.16805230705936));
#33371=CARTESIAN_POINT('Ctrl Pts',(-83.1574679164006,-4.69826260420316,
4.46615843641225));
#33372=CARTESIAN_POINT('Ctrl Pts',(-83.0740344886083,-6.01417371817795,
2.11936688207577));
#33373=CARTESIAN_POINT('Ctrl Pts',(-83.0236303225549,-6.2186530157556,0.543258725776869));
#33374=CARTESIAN_POINT('Ctrl Pts',(-83.0062554182404,-6.21872885219791,
-2.48421024784395E-5));
#33375=CARTESIAN_POINT('Origin',(-88.8777445817596,0.,0.));
#33376=CARTESIAN_POINT('',(-85.7527445817596,-6.21890566139956,-0.00012576145485806));
#33377=CARTESIAN_POINT('',(-85.5062554182403,-6.21904930984993,0.000151106537523982));
#33378=CARTESIAN_POINT('',(-88.8777445817596,-6.21925,-6.18233832090354E-13));
#33379=CARTESIAN_POINT('Ctrl Pts',(-85.7527445817596,-6.21890566139956,
-0.00012576145485773));
#33380=CARTESIAN_POINT('Ctrl Pts',(-85.7411689605953,-6.21917016689645,
-0.362045793825795));
#33381=CARTESIAN_POINT('Ctrl Pts',(-85.696564077692,-6.09942646984245,-1.75647613111435));
#33382=CARTESIAN_POINT('Ctrl Pts',(-85.6189299330499,-5.07038134923681,
-4.03874760456303));
#33383=CARTESIAN_POINT('Ctrl Pts',(-85.5198421478334,-2.52493057070103,
-5.97034024796873));
#33384=CARTESIAN_POINT('Ctrl Pts',(-85.4207543626165,0.634046276949095,
-6.45121938687785));
#33385=CARTESIAN_POINT('Ctrl Pts',(-85.3216665774001,3.63895781668574,-5.36453420729772));
#33386=CARTESIAN_POINT('Ctrl Pts',(-85.2225787921832,5.75964959979071,-2.97433687429733));
#33387=CARTESIAN_POINT('Ctrl Pts',(-85.1234910069667,6.48082067300681,0.138586273355216));
#33388=CARTESIAN_POINT('Ctrl Pts',(-85.0244032217499,5.62723583982488,3.21783460818738));
#33389=CARTESIAN_POINT('Ctrl Pts',(-84.9253154365333,3.40630517705998,5.51519065308138));
#33390=CARTESIAN_POINT('Ctrl Pts',(-84.8262276513165,0.357686244883394,
6.47242638646756));
#33391=CARTESIAN_POINT('Ctrl Pts',(-84.7271398660999,-2.77784584020579,
5.85694590531591));
#33392=CARTESIAN_POINT('Ctrl Pts',(-84.6280520808834,-5.23839717022127,
3.81830301365183));
#33393=CARTESIAN_POINT('Ctrl Pts',(-84.5532536527698,-6.13494781882954,
1.57902449778438));
#33394=CARTESIAN_POINT('Ctrl Pts',(-84.5114844863953,-6.2194116595431,0.273388236258902));
#33395=CARTESIAN_POINT('Ctrl Pts',(-84.5027445817596,-6.21914365535479,
0.000158605856680621));
#33396=CARTESIAN_POINT('Ctrl Pts',(-85.5062554182403,-6.21904930984993,
0.000151106537523774));
#33397=CARTESIAN_POINT('Ctrl Pts',(-85.4829992709549,-6.21838659122049,
-0.726921510317828));
#33398=CARTESIAN_POINT('Ctrl Pts',(-85.4267138619306,-5.90986944813889,
-2.48715788437484));
#33399=CARTESIAN_POINT('Ctrl Pts',(-85.3373991911673,-4.28422646215156,
-4.86473497443532));
#33400=CARTESIAN_POINT('Ctrl Pts',(-85.2383114059508,-1.43968826503564,
-6.32040665848384));
#33401=CARTESIAN_POINT('Ctrl Pts',(-85.139223620734,1.75467563421941,-6.24030096387333));
#33402=CARTESIAN_POINT('Ctrl Pts',(-85.0401358355174,4.52267595876155,-4.64388251792204));
#33403=CARTESIAN_POINT('Ctrl Pts',(-84.9410480503007,6.19172428905613,-1.919060449145));
#33404=CARTESIAN_POINT('Ctrl Pts',(-84.8419602650839,6.35626338222264,1.27206858835509));
#33405=CARTESIAN_POINT('Ctrl Pts',(-84.7428724798673,4.9763123584096,4.15410134539831));
#33406=CARTESIAN_POINT('Ctrl Pts',(-84.6437846946507,2.38718153906689,6.02674099139694));
#33407=CARTESIAN_POINT('Ctrl Pts',(-84.544696909434,-0.782003641280745,
6.43496021602791));
#33408=CARTESIAN_POINT('Ctrl Pts',(-84.4456091242173,-3.76117201100048,
5.27956700696203));
#33409=CARTESIAN_POINT('Ctrl Pts',(-84.3494619604861,-5.76513369117889,
2.91366710550249));
#33410=CARTESIAN_POINT('Ctrl Pts',(-84.2863440584938,-6.2190070562591,0.940319085696299));
#33411=CARTESIAN_POINT('Ctrl Pts',(-84.2562554182403,-6.21967289644367,
-9.04560928895008E-5));
#33412=CARTESIAN_POINT('Origin',(28.1999754182402,0.,0.));
#33413=CARTESIAN_POINT('',(108.82497541824,-6.21455514838355,-0.00757742687950716));
#33414=CARTESIAN_POINT('',(109.067,-6.21925,5.68729293530136E-12));
#33415=CARTESIAN_POINT('',(28.1999754182402,-6.21925,5.68729293530136E-12));
#33416=CARTESIAN_POINT('',(109.067,-2.15736603634146,-5.83308171961789));
#33417=CARTESIAN_POINT('Ctrl Pts',(108.82497541824,-6.21455514838355,-0.00757742687950716));
#33418=CARTESIAN_POINT('Ctrl Pts',(108.844499925929,-6.21989172346176,-0.619498065585236));
#33419=CARTESIAN_POINT('Ctrl Pts',(108.864024433619,-6.13743667878425,-1.2297196011537));
#33420=CARTESIAN_POINT('Ctrl Pts',(108.883548941308,-5.96152933675784,-1.81073897317348));
#33421=CARTESIAN_POINT('Ctrl Pts',(108.944699294205,-5.41059119207356,-3.63047958865122));
#33422=CARTESIAN_POINT('Ctrl Pts',(109.005849647103,-3.94295198716987,-5.16376759627442));
#33423=CARTESIAN_POINT('Ctrl Pts',(109.067,-2.15756780909074,-5.83789702209062));
#33424=CARTESIAN_POINT('Origin',(109.067,0.,0.));
#33425=CARTESIAN_POINT('Origin',(28.1999754182402,0.,0.));
#33426=CARTESIAN_POINT('',(107.57497541824,-6.21197113448905,0.00272930593023462));
#33427=CARTESIAN_POINT('',(107.821464581759,-6.21681811402912,-0.00341565526005089));
#33428=CARTESIAN_POINT('',(28.1999754182402,-6.21925,5.68729293530136E-12));
#33429=CARTESIAN_POINT('Ctrl Pts',(107.57497541824,-6.21197113448905,0.00272930593023461));
#33430=CARTESIAN_POINT('Ctrl Pts',(107.614143383712,-6.20682472272673,-1.22554755889008));
#33431=CARTESIAN_POINT('Ctrl Pts',(107.719481883998,-5.25859683548935,-4.53616070271995));
#33432=CARTESIAN_POINT('Ctrl Pts',(107.890990919097,0.136997792198854,-7.35133649303282));
#33433=CARTESIAN_POINT('Ctrl Pts',(108.056417256132,5.21425114731496,-4.45398626681165));
#33434=CARTESIAN_POINT('Ctrl Pts',(108.18875832576,6.46158639258335,-0.360283155660035));
#33435=CARTESIAN_POINT('Ctrl Pts',(108.288014127981,5.8651082250223,2.77856311405613));
#33436=CARTESIAN_POINT('Ctrl Pts',(108.387269930202,3.81258651774621,5.23074243008551));
#33437=CARTESIAN_POINT('Ctrl Pts',(108.519610999831,-0.144983932043383,
6.8528582990123));
#33438=CARTESIAN_POINT('Ctrl Pts',(108.665512829176,-4.95903172843287,5.01362006060166));
#33439=CARTESIAN_POINT('Ctrl Pts',(108.778329391115,-6.20180552981113,1.45436297979792));
#33440=CARTESIAN_POINT('Ctrl Pts',(108.82497541824,-6.21455514838355,-0.00757742687950737));
#33441=CARTESIAN_POINT('',(109.067,-6.21768400249992,0.139557183823105));
#33442=CARTESIAN_POINT('Origin',(109.067,0.,0.));
#33443=CARTESIAN_POINT('Ctrl Pts',(107.821464581759,-6.21681811402912,-0.00341565526005082));
#33444=CARTESIAN_POINT('Ctrl Pts',(107.839619845622,-6.21808736455384,-0.570723268463156));
#33445=CARTESIAN_POINT('Ctrl Pts',(107.890860376892,-6.0060659270755,-2.16948211616312));
#33446=CARTESIAN_POINT('Ctrl Pts',(107.975186175568,-4.63696157612732,-4.51609008620458));
#33447=CARTESIAN_POINT('Ctrl Pts',(108.107527245197,-1.00805461892616,-6.77986084607601));
#33448=CARTESIAN_POINT('Ctrl Pts',(108.272953582231,4.72291868063634,-5.64086832996922));
#33449=CARTESIAN_POINT('Ctrl Pts',(108.471465186674,7.29544819300465,0.934110138162679));
#33450=CARTESIAN_POINT('Ctrl Pts',(108.636891523709,3.86681832161873,5.66141617959935));
#33451=CARTESIAN_POINT('Ctrl Pts',(108.769232593337,-0.340764604699964,
6.46373036659584));
#33452=CARTESIAN_POINT('Ctrl Pts',(108.868488395558,-3.38799745293929,5.53147877557648));
#33453=CARTESIAN_POINT('Ctrl Pts',(108.967744197779,-5.62418538167471,3.22542302469746));
#33454=CARTESIAN_POINT('Ctrl Pts',(109.033914732593,-6.19447498791001,1.17358721206399));
#33455=CARTESIAN_POINT('Ctrl Pts',(109.067,-6.21768400249992,0.139557183822751));
#33456=CARTESIAN_POINT('Origin',(28.1999754182402,0.,0.));
#33457=CARTESIAN_POINT('',(106.32497541824,-6.22618423365076,0.00404232319106064));
#33458=CARTESIAN_POINT('',(106.57146458176,-6.21560315594324,0.00241033447495986));
#33459=CARTESIAN_POINT('',(28.1999754182402,-6.21925,5.68729293530136E-12));
#33460=CARTESIAN_POINT('Ctrl Pts',(106.32497541824,-6.22618423365075,0.004042323191061));
#33461=CARTESIAN_POINT('Ctrl Pts',(106.383786841494,-6.21175399018336,-1.82954563581619));
#33462=CARTESIAN_POINT('Ctrl Pts',(106.508768799563,-4.38464470241311,-5.75083267620402));
#33463=CARTESIAN_POINT('Ctrl Pts',(106.666836025037,1.10798790665508,-6.76730712296029));
#33464=CARTESIAN_POINT('Ctrl Pts',(106.799177094666,4.70262135634261,-4.44608868040009));
#33465=CARTESIAN_POINT('Ctrl Pts',(106.898432896887,6.2736721784315,-1.66275690292686));
#33466=CARTESIAN_POINT('Ctrl Pts',(106.997688699108,6.28738997577458,1.53331465981352));
#33467=CARTESIAN_POINT('Ctrl Pts',(107.130029768736,4.31428373900651,5.33021287136194));
#33468=CARTESIAN_POINT('Ctrl Pts',(107.295456105771,-1.20636992374352,7.25309034469861));
#33469=CARTESIAN_POINT('Ctrl Pts',(107.454799744741,-5.65798516834366,3.76690557215357));
#33470=CARTESIAN_POINT('Ctrl Pts',(107.547972848898,-6.21551909361338,0.849508831356341));
#33471=CARTESIAN_POINT('Ctrl Pts',(107.57497541824,-6.21197113448905,0.00272930593023461));
#33472=CARTESIAN_POINT('Ctrl Pts',(106.57146458176,-6.21560315594324,0.00241033447496005));
#33473=CARTESIAN_POINT('Ctrl Pts',(106.576178035998,-6.21571381863042,-0.145160143453014));
#33474=CARTESIAN_POINT('Ctrl Pts',(106.613976757643,-6.1753255886943,-1.32900497305834));
#33475=CARTESIAN_POINT('Ctrl Pts',(106.717946014101,-5.14823859197666,-4.5298844173743));
#33476=CARTESIAN_POINT('Ctrl Pts',(106.883372351137,-0.0289675534008062,
-7.35267358327051));
#33477=CARTESIAN_POINT('Ctrl Pts',(107.081883955579,6.1675620574163,-4.00271286495399));
#33478=CARTESIAN_POINT('Ctrl Pts',(107.280395560021,6.70875004256005,3.00890426696354));
#33479=CARTESIAN_POINT('Ctrl Pts',(107.478907164463,1.09964973772579,7.26991658020799));
#33480=CARTESIAN_POINT('Ctrl Pts',(107.644333501498,-4.39210610522649,5.26648010085043));
#33481=CARTESIAN_POINT('Ctrl Pts',(107.758519307264,-6.04627559345864,1.96530621919418));
#33482=CARTESIAN_POINT('Ctrl Pts',(107.806534578215,-6.21577434430061,0.463110457495906));
#33483=CARTESIAN_POINT('Ctrl Pts',(107.821464581759,-6.21681811402912,-0.00341565526005082));
#33484=CARTESIAN_POINT('Origin',(28.1999754182402,0.,0.));
#33485=CARTESIAN_POINT('',(105.07497541824,-6.22210088067886,-0.00776764447856886));
#33486=CARTESIAN_POINT('',(105.321464581759,-6.21925,5.80383180751043E-12));
#33487=CARTESIAN_POINT('',(28.1999754182402,-6.21925,5.68729293530136E-12));
#33488=CARTESIAN_POINT('Ctrl Pts',(105.07497541824,-6.22210088067886,-0.00776764447856897));
#33489=CARTESIAN_POINT('Ctrl Pts',(105.087259764463,-6.22564393247865,-0.391088311636573));
#33490=CARTESIAN_POINT('Ctrl Pts',(105.165714645499,-6.01911196292566,-2.83449884888709));
#33491=CARTESIAN_POINT('Ctrl Pts',(105.277254793943,-3.52167204419261,-5.88403957747914));
#33492=CARTESIAN_POINT('Ctrl Pts',(105.409595863571,0.722150160936881,-6.43123931018474));
#33493=CARTESIAN_POINT('Ctrl Pts',(105.508851665792,3.71862112089202,-5.3193600409715));
#33494=CARTESIAN_POINT('Ctrl Pts',(105.608107468013,5.79200698135239,-2.88703913835982));
#33495=CARTESIAN_POINT('Ctrl Pts',(105.740448537641,6.73563905550354,1.2865699056858));
#33496=CARTESIAN_POINT('Ctrl Pts',(105.905874874676,3.76008989159166,6.31860060108252));
#33497=CARTESIAN_POINT('Ctrl Pts',(106.104386479118,-3.27915422052681,6.58083808626542));
#33498=CARTESIAN_POINT('Ctrl Pts',(106.244086660306,-6.11378249632262,2.52412807553831));
#33499=CARTESIAN_POINT('Ctrl Pts',(106.31761630668,-6.22798989938095,0.233480374486457));
#33500=CARTESIAN_POINT('Ctrl Pts',(106.32497541824,-6.22618423365075,0.004042323191061));
#33501=CARTESIAN_POINT('Ctrl Pts',(105.321464581759,-6.22149027562554,0.00277977264042391));
#33502=CARTESIAN_POINT('Ctrl Pts',(105.378906761187,-6.205339920575,-1.79044338804944));
#33503=CARTESIAN_POINT('Ctrl Pts',(105.502519475428,-4.46474788533615,-5.66066214127837));
#33504=CARTESIAN_POINT('Ctrl Pts',(105.692302724484,2.12728060596421,-7.03810766777042));
#33505=CARTESIAN_POINT('Ctrl Pts',(105.890814328926,7.06620582008108,-2.03199906838922));
#33506=CARTESIAN_POINT('Ctrl Pts',(106.089325933368,5.53238437901881,4.84311030515874));
#33507=CARTESIAN_POINT('Ctrl Pts',(106.254752270403,0.0443617744349961,
6.85726730780797));
#33508=CARTESIAN_POINT('Ctrl Pts',(106.387093340032,-3.88907072626489,5.1727633873222));
#33509=CARTESIAN_POINT('Ctrl Pts',(106.481635688015,-5.80953565783217,2.81060433023539));
#33510=CARTESIAN_POINT('Ctrl Pts',(106.543092768591,-6.21493704125813,0.890685008966381));
#33511=CARTESIAN_POINT('Ctrl Pts',(106.57146458176,-6.21560315594324,0.00241033447496005));
#33512=CARTESIAN_POINT('Origin',(28.1999754182402,0.,0.));
#33513=CARTESIAN_POINT('',(103.82497541824,-6.2174167363618,0.000391862094605458));
#33514=CARTESIAN_POINT('',(104.07146458176,-6.21925,5.31621332200516E-12));
#33515=CARTESIAN_POINT('',(28.1999754182402,-6.21925,5.68729293530136E-12));
#33516=CARTESIAN_POINT('Ctrl Pts',(103.82497541824,-6.20679593735384,0.00266206938908144));
#33517=CARTESIAN_POINT('Ctrl Pts',(103.856903222245,-6.20668924563014,-0.998325940866833));
#33518=CARTESIAN_POINT('Ctrl Pts',(103.921916293657,-5.74038997171335,-3.03807828006894));
#33519=CARTESIAN_POINT('Ctrl Pts',(104.020014632476,-3.59946059997928,-5.37831045715732));
#33520=CARTESIAN_POINT('Ctrl Pts',(104.119270434697,-0.593085485580851,
-6.46312492323568));
#33521=CARTESIAN_POINT('Ctrl Pts',(104.218526236918,2.56051311720067,-5.94357742119504));
#33522=CARTESIAN_POINT('Ctrl Pts',(104.350867306546,5.97511638043491,-3.364829852218));
#33523=CARTESIAN_POINT('Ctrl Pts',(104.516293643581,6.95030565375228,2.39921649231612));
#33524=CARTESIAN_POINT('Ctrl Pts',(104.714805248023,1.74297217383987,7.14299183158766));
#33525=CARTESIAN_POINT('Ctrl Pts',(104.901032506243,-4.63366916893313,5.45146242636149));
#33526=CARTESIAN_POINT('Ctrl Pts',(105.021089229649,-6.20655902326007,1.67369666688253));
#33527=CARTESIAN_POINT('Ctrl Pts',(105.07497541824,-6.22210088067886,-0.00776764447856897));
#33528=CARTESIAN_POINT('Ctrl Pts',(104.07146458176,-6.21925,5.31621332200516E-12));
#33529=CARTESIAN_POINT('Ctrl Pts',(104.130264333233,-6.21925000000157,-1.83816020915209));
#33530=CARTESIAN_POINT('Ctrl Pts',(104.189064084707,-5.35502977485331,-3.6580814134549));
#33531=CARTESIAN_POINT('Ctrl Pts',(104.247863836181,-3.93049712176249,-4.81977830800513));
#33532=CARTESIAN_POINT('Ctrl Pts',(104.306663587654,-2.50596446867168,-5.98147520255536));
#33533=CARTESIAN_POINT('Ctrl Pts',(104.365463339128,-0.549389021424183,
-6.46189408921008));
#33534=CARTESIAN_POINT('Ctrl Pts',(104.424263090602,1.25118869866398,-6.09209302316007));
#33535=CARTESIAN_POINT('Ctrl Pts',(104.483062842075,3.05176641875214,-5.72229195711005));
#33536=CARTESIAN_POINT('Ctrl Pts',(104.541862593549,4.66061422074842,-4.50960958425308));
#33537=CARTESIAN_POINT('Ctrl Pts',(104.600662345023,5.51197192302482,-2.88049233331493));
#33538=CARTESIAN_POINT('Ctrl Pts',(104.659462096496,6.36332962530122,-1.25137508237678));
#33539=CARTESIAN_POINT('Ctrl Pts',(104.71826184797,6.44030216377344,0.761847462635921));
#33540=CARTESIAN_POINT('Ctrl Pts',(104.777061599444,5.71582172177643,2.45121451679953));
#33541=CARTESIAN_POINT('Ctrl Pts',(104.835861350918,4.99134127977942,4.14058157096314));
#33542=CARTESIAN_POINT('Ctrl Pts',(104.894661102391,3.47978506146911,5.47256790209185));
#33543=CARTESIAN_POINT('Ctrl Pts',(104.953460853865,1.71270012776144,5.97877318811025));
#33544=CARTESIAN_POINT('Ctrl Pts',(105.012260605339,-0.0543848059462324,
6.48497847412864));
#33545=CARTESIAN_POINT('Ctrl Pts',(105.071060356812,-2.04193092336917,6.15535714814489));
#33546=CARTESIAN_POINT('Ctrl Pts',(105.129860108286,-3.55100669662017,5.10582236305365));
#33547=CARTESIAN_POINT('Ctrl Pts',(105.18865985976,-5.06008246987117,4.05628757796241));
#33548=CARTESIAN_POINT('Ctrl Pts',(105.247459611233,-6.06074051980635,2.30766719190768));
#33549=CARTESIAN_POINT('Ctrl Pts',(105.306259362707,-6.20109393743633,0.474873184745606));
#33550=CARTESIAN_POINT('Ctrl Pts',(105.311327769058,-6.21319208641554,0.31689046283348));
#33551=CARTESIAN_POINT('Ctrl Pts',(105.316396175409,-6.21924999999985,0.158445276462653));
#33552=CARTESIAN_POINT('Ctrl Pts',(105.321464581759,-6.21925,5.80383131895764E-12));
#33553=CARTESIAN_POINT('Origin',(28.1999754182402,0.,0.));
#33554=CARTESIAN_POINT('',(102.57497541824,-6.21925,5.30358233294917E-12));
#33555=CARTESIAN_POINT('',(102.82146458176,-6.20834130759024,0.000316658844899398));
#33556=CARTESIAN_POINT('',(28.1999754182402,-6.21925,5.68729293530136E-12));
#33557=CARTESIAN_POINT('Ctrl Pts',(102.57497541824,-6.21925,5.30358233294917E-12));
#33558=CARTESIAN_POINT('Ctrl Pts',(102.633775169714,-6.21925000000157,-1.83816020915211));
#33559=CARTESIAN_POINT('Ctrl Pts',(102.692574921188,-5.3550297748533,-3.65808141345491));
#33560=CARTESIAN_POINT('Ctrl Pts',(102.751374672661,-3.93049712176248,-4.81977830800514));
#33561=CARTESIAN_POINT('Ctrl Pts',(102.810174424135,-2.50596446867166,-5.98147520255537));
#33562=CARTESIAN_POINT('Ctrl Pts',(102.868974175609,-0.549389021424171,
-6.46189408921008));
#33563=CARTESIAN_POINT('Ctrl Pts',(102.927773927082,1.25118869866399,-6.09209302316006));
#33564=CARTESIAN_POINT('Ctrl Pts',(102.986573678556,3.05176641875215,-5.72229195711004));
#33565=CARTESIAN_POINT('Ctrl Pts',(103.04537343003,4.66061422074843,-4.50960958425307));
#33566=CARTESIAN_POINT('Ctrl Pts',(103.104173181503,5.51197192302482,-2.88049233331492));
#33567=CARTESIAN_POINT('Ctrl Pts',(103.162972932977,6.36332962530122,-1.25137508237677));
#33568=CARTESIAN_POINT('Ctrl Pts',(103.221772684451,6.44030216377344,0.761847462635935));
#33569=CARTESIAN_POINT('Ctrl Pts',(103.280572435925,5.71582172177642,2.45121451679954));
#33570=CARTESIAN_POINT('Ctrl Pts',(103.339372187398,4.99134127977941,4.14058157096315));
#33571=CARTESIAN_POINT('Ctrl Pts',(103.398171938872,3.4797850614691,5.47256790209186));
#33572=CARTESIAN_POINT('Ctrl Pts',(103.456971690346,1.71270012776143,5.97877318811025));
#33573=CARTESIAN_POINT('Ctrl Pts',(103.515771441819,-0.0543848059462451,
6.48497847412864));
#33574=CARTESIAN_POINT('Ctrl Pts',(103.574571193293,-2.04193092336918,6.15535714814488));
#33575=CARTESIAN_POINT('Ctrl Pts',(103.633370944767,-3.55100669662018,5.10582236305364));
#33576=CARTESIAN_POINT('Ctrl Pts',(103.69217069624,-5.06008246987118,4.0562875779624));
#33577=CARTESIAN_POINT('Ctrl Pts',(103.750970447714,-6.06074051980636,2.30766719190766));
#33578=CARTESIAN_POINT('Ctrl Pts',(103.809770199188,-6.20109393743633,0.474873184745594));
#33579=CARTESIAN_POINT('Ctrl Pts',(103.814838605539,-6.21319208641554,0.316890462833468));
#33580=CARTESIAN_POINT('Ctrl Pts',(103.819907011889,-6.21924999999985,0.15844527646264));
#33581=CARTESIAN_POINT('Ctrl Pts',(103.82497541824,-6.21925,5.79120032990165E-12));
#33582=CARTESIAN_POINT('Ctrl Pts',(102.82146458176,-6.20834130759024,0.000316658844898982));
#33583=CARTESIAN_POINT('Ctrl Pts',(102.852023141938,-6.21030615967812,-0.959220914400505));
#33584=CARTESIAN_POINT('Ctrl Pts',(102.94875223693,-5.55144391813371,-3.99518424091588));
#33585=CARTESIAN_POINT('Ctrl Pts',(103.111651866737,-0.82496606132839,-7.30614229910194));
#33586=CARTESIAN_POINT('Ctrl Pts',(103.310163471179,5.69801405622591,-4.64710923843941));
#33587=CARTESIAN_POINT('Ctrl Pts',(103.475589808214,6.76861424179842,1.09998042754471));
#33588=CARTESIAN_POINT('Ctrl Pts',(103.607930877842,4.45164816401902,4.69735761978553));
#33589=CARTESIAN_POINT('Ctrl Pts',(103.707186680063,1.67018130387269,6.27170061297181));
#33590=CARTESIAN_POINT('Ctrl Pts',(103.806442482284,-1.52587995074471,6.2891995008118));
#33591=CARTESIAN_POINT('Ctrl Pts',(103.927868449516,-5.01174531446683,4.48295294983669));
#33592=CARTESIAN_POINT('Ctrl Pts',(104.016209149341,-6.20768450607271,1.71559912667801));
#33593=CARTESIAN_POINT('Ctrl Pts',(104.071464581759,-6.22368981997608,-0.00517086289489384));
#33594=CARTESIAN_POINT('Origin',(28.1999754182402,0.,0.));
#33595=CARTESIAN_POINT('',(101.32497541824,-6.22105475706665,-0.00162676184122019));
#33596=CARTESIAN_POINT('',(101.57146458176,-6.21989505726344,0.0051066519576129));
#33597=CARTESIAN_POINT('',(28.1999754182402,-6.21925,5.68729293530136E-12));
#33598=CARTESIAN_POINT('Ctrl Pts',(101.32497541824,-6.22105475706665,-0.00162676184122041));
#33599=CARTESIAN_POINT('Ctrl Pts',(101.330019602996,-6.22143817055166,-0.158868376741796));
#33600=CARTESIAN_POINT('Ctrl Pts',(101.368149055159,-6.17819176943028,-1.34717661173896));
#33601=CARTESIAN_POINT('Ctrl Pts',(101.439363774729,-5.43325591434297,-3.51597357120765));
#33602=CARTESIAN_POINT('Ctrl Pts',(101.571704844356,-2.3211098600259,-6.45263858533859));
#33603=CARTESIAN_POINT('Ctrl Pts',(101.737131181392,3.52484809098738,-6.45278501071125));
#33604=CARTESIAN_POINT('Ctrl Pts',(101.935642785834,7.33364606630008,-0.527180871479639));
#33605=CARTESIAN_POINT('Ctrl Pts',(102.134154390276,4.42207903767292,5.87413834375616));
#33606=CARTESIAN_POINT('Ctrl Pts',(102.332665994718,-2.54733029566822,6.89739782988979));
#33607=CARTESIAN_POINT('Ctrl Pts',(102.479606337373,-5.95970016665688,2.98335614725549));
#33608=CARTESIAN_POINT('Ctrl Pts',(102.560376145214,-6.22546141667382,0.459170652905071));
#33609=CARTESIAN_POINT('Ctrl Pts',(102.57497541824,-6.22306105720208,0.00238369616239718));
#33610=CARTESIAN_POINT('Ctrl Pts',(101.57146458176,-6.21989505726344,0.00510665195761345));
#33611=CARTESIAN_POINT('Ctrl Pts',(101.62166659972,-6.2061803997074,-1.56410508432724));
#33612=CARTESIAN_POINT('Ctrl Pts',(101.738039152495,-4.80701918903245,-5.22328206966102));
#33613=CARTESIAN_POINT('Ctrl Pts',(101.920582240084,1.3526844941182,-7.22725626488847));
#33614=CARTESIAN_POINT('Ctrl Pts',(102.086008577119,5.87986878794746,-3.52863128306579));
#33615=CARTESIAN_POINT('Ctrl Pts',(102.218349646747,6.43208922602856,0.714540532497019));
#33616=CARTESIAN_POINT('Ctrl Pts',(102.317605448968,5.32375599492072,3.71232491487952));
#33617=CARTESIAN_POINT('Ctrl Pts',(102.416861251189,2.89388995296144,5.78858712677963));
#33618=CARTESIAN_POINT('Ctrl Pts',(102.549202320817,-1.27859977470671,6.73715654497048));
#33619=CARTESIAN_POINT('Ctrl Pts',(102.684070097674,-5.38395033335684,4.31612449633043));
#33620=CARTESIAN_POINT('Ctrl Pts',(102.785852607124,-6.20605153142578,1.11853124490405));
#33621=CARTESIAN_POINT('Ctrl Pts',(102.82146458176,-6.20834130759024,0.000316658844898982));
#33622=CARTESIAN_POINT('Origin',(28.1999754182402,0.,0.));
#33623=CARTESIAN_POINT('',(100.07497541824,-6.21925,5.38891630971761E-12));
#33624=CARTESIAN_POINT('',(100.32146458176,-6.22909731479716,-0.0014603442074157));
#33625=CARTESIAN_POINT('',(28.1999754182402,-6.21925,5.68729293530136E-12));
#33626=CARTESIAN_POINT('Ctrl Pts',(100.07497541824,-6.21823345339706,-0.000850643466643111));
#33627=CARTESIAN_POINT('Ctrl Pts',(100.099663060778,-6.22121061960845,-0.774526207076587));
#33628=CARTESIAN_POINT('Ctrl Pts',(100.190521238131,-5.71106097194565,-3.62193451684539));
#33629=CARTESIAN_POINT('Ctrl Pts',(100.347549950297,-1.47265859680333,-7.20376742519206));
#33630=CARTESIAN_POINT('Ctrl Pts',(100.546061554739,5.26119106866268,-5.13616129381046));
#33631=CARTESIAN_POINT('Ctrl Pts',(100.744573159181,7.16905691026357,1.63245438356331));
#33632=CARTESIAN_POINT('Ctrl Pts',(100.943084763623,2.50626464765636,6.91242547698743));
#33633=CARTESIAN_POINT('Ctrl Pts',(101.108511100658,-3.27215427013865,6.02636724135885));
#33634=CARTESIAN_POINT('Ctrl Pts',(101.235807985531,-5.8030391565124,2.78060935378298));
#33635=CARTESIAN_POINT('Ctrl Pts',(101.296934335589,-6.21892332656926,0.872493702243004));
#33636=CARTESIAN_POINT('Ctrl Pts',(101.32497541824,-6.22105475706665,-0.00162676184122041));
#33637=CARTESIAN_POINT('Ctrl Pts',(100.32146458176,-6.22909731479716,-0.00146034420741566));
#33638=CARTESIAN_POINT('Ctrl Pts',(100.325139522689,-6.22952837035362,-0.115891893155128));
#33639=CARTESIAN_POINT('Ctrl Pts',(100.394984998432,-6.17349008821943,-2.29036018435994));
#33640=CARTESIAN_POINT('Ctrl Pts',(100.531001008989,-3.63164551501983,-6.39328861480798));
#33641=CARTESIAN_POINT('Ctrl Pts',(100.696427346024,2.21350682387351,-6.49033768273847));
#33642=CARTESIAN_POINT('Ctrl Pts',(100.828768415652,5.37404798958258,-3.60582143066423));
#33643=CARTESIAN_POINT('Ctrl Pts',(100.928024217873,6.46241869027549,-0.600731919134315));
#33644=CARTESIAN_POINT('Ctrl Pts',(101.027280020095,5.94660273312621,2.55347917918856));
#33645=CARTESIAN_POINT('Ctrl Pts',(101.159621089723,3.3718969584413,5.97113109862479));
#33646=CARTESIAN_POINT('Ctrl Pts',(101.325047426758,-2.39099155665315,6.95313942295208));
#33647=CARTESIAN_POINT('Ctrl Pts',(101.473357013239,-5.93970404826024,3.06689542039316));
#33648=CARTESIAN_POINT('Ctrl Pts',(101.555496064906,-6.22425748628952,0.504249616225492));
#33649=CARTESIAN_POINT('Ctrl Pts',(101.57146458176,-6.21989505726344,0.00510665195761345));
#33650=CARTESIAN_POINT('Origin',(28.1999754182402,0.,0.));
#33651=CARTESIAN_POINT('',(98.8249754182402,-6.21788518063575,0.00023803869261306));
#33652=CARTESIAN_POINT('',(99.0714645817595,-6.21907165140323,-0.00016453540808593));
#33653=CARTESIAN_POINT('',(28.1999754182402,-6.21925,5.68729293530136E-12));
#33654=CARTESIAN_POINT('Ctrl Pts',(98.8249754182402,-6.21925,5.25482207309205E-12));
#33655=CARTESIAN_POINT('Ctrl Pts',(98.8837751697139,-6.21925000000155,-1.83816020915227));
#33656=CARTESIAN_POINT('Ctrl Pts',(98.9425749211876,-5.35502977485315,-3.65808141345518));
#33657=CARTESIAN_POINT('Ctrl Pts',(99.0013746726613,-3.93049712176217,-4.81977830800539));
#33658=CARTESIAN_POINT('Ctrl Pts',(99.060174424135,-2.50596446867118,-5.9814752025556));
#33659=CARTESIAN_POINT('Ctrl Pts',(99.1189741756087,-0.549389021423501,
-6.46189408921017));
#33660=CARTESIAN_POINT('Ctrl Pts',(99.1777739270824,1.25118869866473,-6.09209302315991));
#33661=CARTESIAN_POINT('Ctrl Pts',(99.2365736785561,3.05176641875296,-5.72229195710965));
#33662=CARTESIAN_POINT('Ctrl Pts',(99.2953734300298,4.66061422074918,-4.50960958425234));
#33663=CARTESIAN_POINT('Ctrl Pts',(99.3541731815035,5.51197192302534,-2.88049233331393));
#33664=CARTESIAN_POINT('Ctrl Pts',(99.4129729329772,6.3633296253015,-1.25137508237553));
#33665=CARTESIAN_POINT('Ctrl Pts',(99.4717726844509,6.4403021637733,0.761847462637341));
#33666=CARTESIAN_POINT('Ctrl Pts',(99.5305724359246,5.71582172177585,2.45121451680089));
#33667=CARTESIAN_POINT('Ctrl Pts',(99.5893721873983,4.99134127977839,4.14058157096443));
#33668=CARTESIAN_POINT('Ctrl Pts',(99.648171938872,3.47978506146762,5.47256790209284));
#33669=CARTESIAN_POINT('Ctrl Pts',(99.7069716903457,1.71270012775968,5.97877318811075));
#33670=CARTESIAN_POINT('Ctrl Pts',(99.7657714418194,-0.0543848059482521,
6.48497847412865));
#33671=CARTESIAN_POINT('Ctrl Pts',(99.8245711932931,-2.04193092337123,6.15535714814424));
#33672=CARTESIAN_POINT('Ctrl Pts',(99.8833709447668,-3.55100669662196,5.1058223630524));
#33673=CARTESIAN_POINT('Ctrl Pts',(99.9421706962405,-5.06008246987269,4.05628757796056));
#33674=CARTESIAN_POINT('Ctrl Pts',(100.000970447714,-6.06074051980728,2.30766719190532));
#33675=CARTESIAN_POINT('Ctrl Pts',(100.059770199188,-6.20109393743652,0.474873184743078));
#33676=CARTESIAN_POINT('Ctrl Pts',(100.064838605539,-6.21319208641561,0.316890462831652));
#33677=CARTESIAN_POINT('Ctrl Pts',(100.069907011889,-6.21924999999986,0.158445276461531));
#33678=CARTESIAN_POINT('Ctrl Pts',(100.07497541824,-6.21925,5.38891663729445E-12));
#33679=CARTESIAN_POINT('Ctrl Pts',(99.0714645817595,-6.21191492285883,-0.00676697184800665));
#33680=CARTESIAN_POINT('Ctrl Pts',(99.0947829804711,-6.2167521851182,-0.737717910543499));
#33681=CARTESIAN_POINT('Ctrl Pts',(99.1842719139968,-5.76013513448276,-3.5356653242606));
#33682=CARTESIAN_POINT('Ctrl Pts',(99.3068461149296,-2.49850315059143,-6.3860455449202));
#33683=CARTESIAN_POINT('Ctrl Pts',(99.4391871845576,1.77733710574879,-6.22281389700046));
#33684=CARTESIAN_POINT('Ctrl Pts',(99.5384429867787,4.54827162108827,-4.63000641769442));
#33685=CARTESIAN_POINT('Ctrl Pts',(99.6376987889997,6.19017426763678,-1.8878777821833));
#33686=CARTESIAN_POINT('Ctrl Pts',(99.7700398586277,6.4295287824728,2.38437734653381));
#33687=CARTESIAN_POINT('Ctrl Pts',(99.9354661956629,2.66165501182151,6.85409228541916));
#33688=CARTESIAN_POINT('Ctrl Pts',(100.130302859176,-4.19448567590115,5.96364365419648));
#33689=CARTESIAN_POINT('Ctrl Pts',(100.258968987875,-6.22176683696992,1.94454851646174));
#33690=CARTESIAN_POINT('Ctrl Pts',(100.32146458176,-6.22909731479716,-0.00146034420741566));
#33691=CARTESIAN_POINT('Origin',(28.1999754182402,0.,0.));
#33692=CARTESIAN_POINT('',(97.5749754182402,-6.22946104778866,0.003031573280016));
#33693=CARTESIAN_POINT('',(97.8214645817595,-6.21908492321965,0.000146043508555585));
#33694=CARTESIAN_POINT('',(28.1999754182402,-6.21925,5.68729293530136E-12));
#33695=CARTESIAN_POINT('Ctrl Pts',(97.5749754182402,-6.22946104778865,0.00303157328001538));
#33696=CARTESIAN_POINT('Ctrl Pts',(97.6389499763434,-6.22390252582942,-1.98595495917002));
#33697=CARTESIAN_POINT('Ctrl Pts',(97.7690950692605,-4.10935756144167,-6.05247427775012));
#33698=CARTESIAN_POINT('Ctrl Pts',(97.9654106969916,2.80531182390014,-6.79636004547279));
#33699=CARTESIAN_POINT('Ctrl Pts',(98.1639223014338,7.23361860234148,-1.31823760182156));
#33700=CARTESIAN_POINT('Ctrl Pts',(98.3293486384688,5.39619172482621,4.2314548992311));
#33701=CARTESIAN_POINT('Ctrl Pts',(98.4616897080969,1.63023388960724,6.26296075744928));
#33702=CARTESIAN_POINT('Ctrl Pts',(98.5609455103179,-1.56567653366841,6.29860231789631));
#33703=CARTESIAN_POINT('Ctrl Pts',(98.6602013125392,-4.37293411252434,4.77072187742011));
#33704=CARTESIAN_POINT('Ctrl Pts',(98.7482112818464,-5.95333417220565,2.40432899867917));
#33705=CARTESIAN_POINT('Ctrl Pts',(98.8031359837468,-6.21472755727631,0.685712634539138));
#33706=CARTESIAN_POINT('Ctrl Pts',(98.8249754182402,-6.21007513781392,0.00160019136293106));
#33707=CARTESIAN_POINT('Ctrl Pts',(97.8214645817595,-6.21925,4.99926393374325E-12));
#33708=CARTESIAN_POINT('Ctrl Pts',(97.8802643332332,-6.21925000000148,-1.83816020915241));
#33709=CARTESIAN_POINT('Ctrl Pts',(97.9390640847069,-5.35502977485312,-3.65808141345517));
#33710=CARTESIAN_POINT('Ctrl Pts',(97.9978638361806,-3.93049712176224,-4.81977830800533));
#33711=CARTESIAN_POINT('Ctrl Pts',(98.0566635876543,-2.50596446867137,-5.98147520255549));
#33712=CARTESIAN_POINT('Ctrl Pts',(98.115463339128,-0.549389021423854,-6.46189408921011));
#33713=CARTESIAN_POINT('Ctrl Pts',(98.1742630906017,1.25118869866429,-6.09209302316));
#33714=CARTESIAN_POINT('Ctrl Pts',(98.2330628420754,3.05176641875243,-5.72229195710989));
#33715=CARTESIAN_POINT('Ctrl Pts',(98.2918625935491,4.66061422074865,-4.50960958425284));
#33716=CARTESIAN_POINT('Ctrl Pts',(98.3506623450228,5.51197192302497,-2.88049233331465));
#33717=CARTESIAN_POINT('Ctrl Pts',(98.4094620964965,6.36332962530128,-1.25137508237646));
#33718=CARTESIAN_POINT('Ctrl Pts',(98.4682618479702,6.4403021637734,0.761847462636249));
#33719=CARTESIAN_POINT('Ctrl Pts',(98.5270615994439,5.7158217217763,2.45121451679982));
#33720=CARTESIAN_POINT('Ctrl Pts',(98.5858613509176,4.99134127977921,4.14058157096339));
#33721=CARTESIAN_POINT('Ctrl Pts',(98.6446611023913,3.47978506146883,5.47256790209203));
#33722=CARTESIAN_POINT('Ctrl Pts',(98.703460853865,1.71270012776114,5.97877318811033));
#33723=CARTESIAN_POINT('Ctrl Pts',(98.7622606053387,-0.0543848059465626,
6.48497847412864));
#33724=CARTESIAN_POINT('Ctrl Pts',(98.8210603568124,-2.04193092336948,6.15535714814478));
#33725=CARTESIAN_POINT('Ctrl Pts',(98.8798601082861,-3.55100669662043,5.10582236305346));
#33726=CARTESIAN_POINT('Ctrl Pts',(98.9386598597598,-5.06008246987137,4.05628757796215));
#33727=CARTESIAN_POINT('Ctrl Pts',(98.9974596112335,-6.06074051980647,2.30766719190737));
#33728=CARTESIAN_POINT('Ctrl Pts',(99.0562593627072,-6.20109393743635,0.47487318474529));
#33729=CARTESIAN_POINT('Ctrl Pts',(99.061327769058,-6.21319208641557,0.316890462832929));
#33730=CARTESIAN_POINT('Ctrl Pts',(99.0663961754087,-6.21924999999988,0.158445276461865));
#33731=CARTESIAN_POINT('Ctrl Pts',(99.0714645817595,-6.21925,4.77983506519556E-12));
#33732=CARTESIAN_POINT('Origin',(28.1999754182402,0.,0.));
#33733=CARTESIAN_POINT('',(96.3249754182403,-6.21661354691106,-0.00511547088340806));
#33734=CARTESIAN_POINT('',(96.5714645817595,-6.22727089829113,0.000782417097775698));
#33735=CARTESIAN_POINT('',(28.1999754182402,-6.21925,5.68729293530136E-12));
#33736=CARTESIAN_POINT('Ctrl Pts',(96.3249754182403,-6.21661354691106,-0.00511547088340718));
#33737=CARTESIAN_POINT('Ctrl Pts',(96.3424228993118,-6.22171682457446,-0.551217455118361));
#33738=CARTESIAN_POINT('Ctrl Pts',(96.4260409151973,-5.90739062850722,-3.16292774537146));
#33739=CARTESIAN_POINT('Ctrl Pts',(96.5758294658966,-2.24400282214668,-7.00176660787908));
#33740=CARTESIAN_POINT('Ctrl Pts',(96.7743410703392,4.67420254334854,-5.67580999001474));
#33741=CARTESIAN_POINT('Ctrl Pts',(96.9397674073738,6.85281755654995,-0.250972572108975));
#33742=CARTESIAN_POINT('Ctrl Pts',(97.0721084770024,5.28760290966167,3.73143343152621));
#33743=CARTESIAN_POINT('Ctrl Pts',(97.171364279223,2.86956225427671,5.82145571450295));
#33744=CARTESIAN_POINT('Ctrl Pts',(97.2706200814443,-0.260798927335446,
6.46639960903085));
#33745=CARTESIAN_POINT('Ctrl Pts',(97.4029611510722,-4.37268362577514,5.28239847078841));
#33746=CARTESIAN_POINT('Ctrl Pts',(97.5044129300043,-6.19766708457246,2.19647310644682));
#33747=CARTESIAN_POINT('Ctrl Pts',(97.5727794415293,-6.22965184839958,0.0713050906459493));
#33748=CARTESIAN_POINT('Ctrl Pts',(97.5749754182402,-6.22946104778865,0.00303157328001538));
#33749=CARTESIAN_POINT('Ctrl Pts',(96.5714645817595,-6.22727089829113,0.000782417097776149));
#33750=CARTESIAN_POINT('Ctrl Pts',(96.600984628629,-6.22650045475056,-0.92035981733023));
#33751=CARTESIAN_POINT('Ctrl Pts',(96.6635899429056,-5.76619445014441,-2.87893556911145));
#33752=CARTESIAN_POINT('Ctrl Pts',(96.7592805245889,-3.80654732511578,-5.25679861025155));
#33753=CARTESIAN_POINT('Ctrl Pts',(96.8585363268103,-0.828976761999734,
-6.41834382938761));
#33754=CARTESIAN_POINT('Ctrl Pts',(96.990877396438,3.4233566459321,-5.94177793005278));
#33755=CARTESIAN_POINT('Ctrl Pts',(97.1563037334735,7.20202000654271,-1.48118070617854));
#33756=CARTESIAN_POINT('Ctrl Pts',(97.3548153379154,5.14238247907462,5.25511053508099));
#33757=CARTESIAN_POINT('Ctrl Pts',(97.5533269423575,-1.62397116860792,7.17098333149248));
#33758=CARTESIAN_POINT('Ctrl Pts',(97.7088766903056,-5.76557152816693,3.52220956672017));
#33759=CARTESIAN_POINT('Ctrl Pts',(97.7982559034396,-6.2172889394232,0.732667319618331));
#33760=CARTESIAN_POINT('Ctrl Pts',(97.8214645817595,-6.21180884511622,0.0065831931557591));
#33761=CARTESIAN_POINT('Origin',(28.1999754182402,0.,0.));
#33762=CARTESIAN_POINT('',(95.0749754182402,-6.21121305788863,0.0018572188690421));
#33763=CARTESIAN_POINT('',(95.3214645817595,-6.21743435837855,-0.00353071204778788));
#33764=CARTESIAN_POINT('',(28.1999754182402,-6.21925,5.68729293530136E-12));
#33765=CARTESIAN_POINT('Ctrl Pts',(95.0749754182402,-6.21121305788863,0.00185721886904223));
#33766=CARTESIAN_POINT('Ctrl Pts',(95.1120663570942,-6.2079342228646,-1.16163168635908));
#33767=CARTESIAN_POINT('Ctrl Pts',(95.2153278307623,-5.33382860132951,-4.40534107097937));
#33768=CARTESIAN_POINT('Ctrl Pts',(95.384759839244,-0.0932801621545284,
-7.35216208134352));
#33769=CARTESIAN_POINT('Ctrl Pts',(95.5501861762794,5.07221142391009,-4.61484203049959));
#33770=CARTESIAN_POINT('Ctrl Pts',(95.6825272459072,6.44713844549368,-0.562801784655363));
#33771=CARTESIAN_POINT('Ctrl Pts',(95.7817830481286,5.94923618490345,2.59428660392868));
#33772=CARTESIAN_POINT('Ctrl Pts',(95.8810388503493,3.97453618501874,5.10738701276399));
#33773=CARTESIAN_POINT('Ctrl Pts',(96.0133799199776,0.069653856197323,6.85705797231051));
#33774=CARTESIAN_POINT('Ctrl Pts',(96.161358775941,-4.86882509062783,5.13720229160962));
#33775=CARTESIAN_POINT('Ctrl Pts',(96.2762523644977,-6.2023623624084,1.51990445707891));
#33776=CARTESIAN_POINT('Ctrl Pts',(96.3249754182403,-6.21661354691106,-0.00511547088340718));
#33777=CARTESIAN_POINT('Ctrl Pts',(95.3214645817595,-6.21743435837855,-0.00353071204778815));
#33778=CARTESIAN_POINT('Ctrl Pts',(95.3375428190044,-6.2188023314762,-0.505805742142214));
#33779=CARTESIAN_POINT('Ctrl Pts',(95.3867063236564,-6.03922426887351,-2.03954346570472));
#33780=CARTESIAN_POINT('Ctrl Pts',(95.4689550957154,-4.77589237691392,-4.36728657043583));
#33781=CARTESIAN_POINT('Ctrl Pts',(95.6012961653434,-1.22034872738306,-6.74795114674706));
#33782=CARTESIAN_POINT('Ctrl Pts',(95.7667225023786,4.544895881605,-5.77987109582617));
#33783=CARTESIAN_POINT('Ctrl Pts',(95.9652341068206,7.31967546924895,0.694719599470295));
#33784=CARTESIAN_POINT('Ctrl Pts',(96.1637457112627,3.388114636821,6.52540906800271));
#33785=CARTESIAN_POINT('Ctrl Pts',(96.3622573157049,-3.65451648904094,6.38024276108088));
#33786=CARTESIAN_POINT('Ctrl Pts',(96.4981636058704,-6.16747960465473,2.28738448867254));
#33787=CARTESIAN_POINT('Ctrl Pts',(96.567899361222,-6.22736394696229,0.112031400768883));
#33788=CARTESIAN_POINT('Ctrl Pts',(96.5714645817595,-6.22727089829113,0.000782417097776149));
#33789=CARTESIAN_POINT('Origin',(28.1999754182402,0.,0.));
#33790=CARTESIAN_POINT('',(93.8249754182403,-6.22441105920928,0.00468493321960073));
#33791=CARTESIAN_POINT('',(94.0714645817596,-6.21573536891404,0.00197485669535868));
#33792=CARTESIAN_POINT('',(28.1999754182402,-6.21925,5.68729293530136E-12));
#33793=CARTESIAN_POINT('Ctrl Pts',(93.8249754182403,-6.22441105920928,0.00468493321960094));
#33794=CARTESIAN_POINT('Ctrl Pts',(93.8817098148766,-6.20866265984911,-1.76545450189424));
#33795=CARTESIAN_POINT('Ctrl Pts',(94.0046147463269,-4.49086526416891,-5.62631371215349));
#33796=CARTESIAN_POINT('Ctrl Pts',(94.1606049451846,0.895521517553394,-6.7986864103964));
#33797=CARTESIAN_POINT('Ctrl Pts',(94.2929460148125,4.56108251734731,-4.59117264477413));
#33798=CARTESIAN_POINT('Ctrl Pts',(94.3922018170336,6.21852484226242,-1.85840871534061));
#33799=CARTESIAN_POINT('Ctrl Pts',(94.4914576192548,6.33232305163478,1.33567389504654));
#33800=CARTESIAN_POINT('Ctrl Pts',(94.6237986888826,4.47908725340983,5.19248236122677));
#33801=CARTESIAN_POINT('Ctrl Pts',(94.7892250259181,-0.978642878797454,
7.28733466877817));
#33802=CARTESIAN_POINT('Ctrl Pts',(94.9506456915058,-5.59666748377655,3.89861203888041));
#33803=CARTESIAN_POINT('Ctrl Pts',(95.04589582228,-6.21378369105847,0.914041927951374));
#33804=CARTESIAN_POINT('Ctrl Pts',(95.0749754182402,-6.21121305788863,0.00185721886904223));
#33805=CARTESIAN_POINT('Ctrl Pts',(94.0714645817595,-6.21573536891404,0.00197485669535951));
#33806=CARTESIAN_POINT('Ctrl Pts',(94.0741010093799,-6.21584226203414,-0.0805910237340283));
#33807=CARTESIAN_POINT('Ctrl Pts',(94.1098227044073,-6.1954099144712,-1.19952608424165));
#33808=CARTESIAN_POINT('Ctrl Pts',(94.2117149342486,-5.2875683157848,-4.36643069350914));
#33809=CARTESIAN_POINT('Ctrl Pts',(94.3771412712839,-0.259211159662201,
-7.34818331519461));
#33810=CARTESIAN_POINT('Ctrl Pts',(94.5756528757259,6.03919547739302,-4.19385291621541));
#33811=CARTESIAN_POINT('Ctrl Pts',(94.7741644801679,6.79967439427966,2.79726874447026));
#33812=CARTESIAN_POINT('Ctrl Pts',(94.9726760846102,1.32679513771092,7.23205386605656));
#33813=CARTESIAN_POINT('Ctrl Pts',(95.1381024216451,-4.22506743128341,5.40119439535534));
#33814=CARTESIAN_POINT('Ctrl Pts',(95.2543652540283,-6.01367690893417,2.09488009192008));
#33815=CARTESIAN_POINT('Ctrl Pts',(95.3044575515974,-6.21598736146102,0.527759283015377));
#33816=CARTESIAN_POINT('Ctrl Pts',(95.3214645817595,-6.21743435837855,-0.00353071204778815));
#33817=CARTESIAN_POINT('Origin',(28.1999754182402,0.,0.));
#33818=CARTESIAN_POINT('',(92.5749754182402,-6.22408856974339,-0.00719918589093503));
#33819=CARTESIAN_POINT('',(92.8214645817595,-6.21925,4.46288405536732E-12));
#33820=CARTESIAN_POINT('',(28.1999754182402,-6.21925,5.68729293530136E-12));
#33821=CARTESIAN_POINT('Ctrl Pts',(92.5749754182402,-6.22408856974339,-0.00719918589093541));
#33822=CARTESIAN_POINT('Ctrl Pts',(92.585182737845,-6.2268665635629,-0.325414501277245));
#33823=CARTESIAN_POINT('Ctrl Pts',(92.6615605922639,-6.06021962183329,-2.70283095786737));
#33824=CARTESIAN_POINT('Ctrl Pts',(92.7710237140898,-3.7042076507531,-5.7708700709176));
#33825=CARTESIAN_POINT('Ctrl Pts',(92.9033647837178,0.520397198382932,-6.45069970934075));
#33826=CARTESIAN_POINT('Ctrl Pts',(93.0026205859388,3.55021779910258,-5.43320234723718));
#33827=CARTESIAN_POINT('Ctrl Pts',(93.10187638816,5.69875659207993,-3.06700395963218));
#33828=CARTESIAN_POINT('Ctrl Pts',(93.2342174577878,6.77262535525563,1.0750076709765));
#33829=CARTESIAN_POINT('Ctrl Pts',(93.3996437948232,3.95611714926058,6.19775165365016));
#33830=CARTESIAN_POINT('Ctrl Pts',(93.5981553992651,-3.07146236840367,6.6802996352329));
#33831=CARTESIAN_POINT('Ctrl Pts',(93.739932607071,-6.07575174174706,2.65538258240216));
#33832=CARTESIAN_POINT('Ctrl Pts',(93.8155392800626,-6.22703035334564,0.29909681196911));
#33833=CARTESIAN_POINT('Ctrl Pts',(93.8249754182403,-6.22441105920928,0.00468493321960094));
#33834=CARTESIAN_POINT('Ctrl Pts',(92.8214645817596,-6.2195957732021,0.00304117013771654));
#33835=CARTESIAN_POINT('Ctrl Pts',(92.8768297345694,-6.20322707436264,-1.72625245001619));
#33836=CARTESIAN_POINT('Ctrl Pts',(92.9983654221932,-4.56818868445748,-5.53539594499472));
#33837=CARTESIAN_POINT('Ctrl Pts',(93.1860716446312,1.90583395511156,-7.10127321207659));
#33838=CARTESIAN_POINT('Ctrl Pts',(93.3845832490731,6.99910671440612,-2.25228539429799));
#33839=CARTESIAN_POINT('Ctrl Pts',(93.5830948535154,5.68133630187344,4.66748393505667));
#33840=CARTESIAN_POINT('Ctrl Pts',(93.7485211905503,0.259080310101639,6.85251582181516));
#33841=CARTESIAN_POINT('Ctrl Pts',(93.8808622601785,-3.72517479045193,5.29201405560826));
#33842=CARTESIAN_POINT('Ctrl Pts',(93.9774816347792,-5.76246549727055,2.94061004980632));
#33843=CARTESIAN_POINT('Ctrl Pts',(94.0410157419728,-6.21450083038052,0.955551296889638));
#33844=CARTESIAN_POINT('Ctrl Pts',(94.0714645817595,-6.21573536891404,0.00197485669535951));
#33845=CARTESIAN_POINT('Origin',(28.1999754182402,0.,0.));
#33846=CARTESIAN_POINT('',(91.3249754182403,-6.21873749421801,7.04867538213377E-5));
#33847=CARTESIAN_POINT('',(91.5714645817596,-6.21925,3.97526767998117E-12));
#33848=CARTESIAN_POINT('',(28.1999754182402,-6.21925,5.68729293530136E-12));
#33849=CARTESIAN_POINT('Ctrl Pts',(91.3249754182402,-6.20685969906364,0.00170408232238357));
#33850=CARTESIAN_POINT('Ctrl Pts',(91.3548261956275,-6.20822254272067,-0.934201698018358));
#33851=CARTESIAN_POINT('Ctrl Pts',(91.4177622404217,-5.78895833438908,-2.90776862535172));
#33852=CARTESIAN_POINT('Ctrl Pts',(91.513783552623,-3.76612079172275,-5.26295298918085));
#33853=CARTESIAN_POINT('Ctrl Pts',(91.613039354844,-0.795191902178077,-6.44138215026858));
#33854=CARTESIAN_POINT('Ctrl Pts',(91.7122951570653,2.37312999160159,-6.02084662046249));
#33855=CARTESIAN_POINT('Ctrl Pts',(91.844636226693,5.86681383167074,-3.55029451733617));
#33856=CARTESIAN_POINT('Ctrl Pts',(92.0100625637283,7.0220299791157,2.18038607393216));
#33857=CARTESIAN_POINT('Ctrl Pts',(92.2085741681705,1.9658051306551,7.08490610278661));
#33858=CARTESIAN_POINT('Ctrl Pts',(92.3968784530076,-4.53235594076636,5.57726581121151));
#33859=CARTESIAN_POINT('Ctrl Pts',(92.519012203031,-6.20885778712949,1.73746570825861));
#33860=CARTESIAN_POINT('Ctrl Pts',(92.5749754182402,-6.22408856974339,-0.00719918589093541));
#33861=CARTESIAN_POINT('Ctrl Pts',(91.5714645817595,-6.21925,4.32879111273125E-12));
#33862=CARTESIAN_POINT('Ctrl Pts',(91.6302643332332,-6.21925000000128,-1.83816020915308));
#33863=CARTESIAN_POINT('Ctrl Pts',(91.6890640847069,-5.35502977485273,-3.65808141345575));
#33864=CARTESIAN_POINT('Ctrl Pts',(91.7478638361806,-3.93049712176173,-4.81977830800575));
#33865=CARTESIAN_POINT('Ctrl Pts',(91.8066635876543,-2.50596446867072,-5.98147520255576));
#33866=CARTESIAN_POINT('Ctrl Pts',(91.865463339128,-0.549389021423158,-6.46189408921017));
#33867=CARTESIAN_POINT('Ctrl Pts',(91.9242630906017,1.25118869866495,-6.09209302315987));
#33868=CARTESIAN_POINT('Ctrl Pts',(91.9830628420754,3.05176641875305,-5.72229195710956));
#33869=CARTESIAN_POINT('Ctrl Pts',(92.0418625935491,4.66061422074914,-4.50960958425234));
#33870=CARTESIAN_POINT('Ctrl Pts',(92.1006623450228,5.51197192302528,-2.88049233331405));
#33871=CARTESIAN_POINT('Ctrl Pts',(92.1594620964965,6.36332962530141,-1.25137508237577));
#33872=CARTESIAN_POINT('Ctrl Pts',(92.2182618479702,6.44030216377332,0.761847462636944));
#33873=CARTESIAN_POINT('Ctrl Pts',(92.2770615994439,5.71582172177604,2.45121451680044));
#33874=CARTESIAN_POINT('Ctrl Pts',(92.3358613509176,4.99134127977876,4.14058157096393));
#33875=CARTESIAN_POINT('Ctrl Pts',(92.3946611023913,3.47978506146824,5.4725679020924));
#33876=CARTESIAN_POINT('Ctrl Pts',(92.453460853865,1.71270012776049,5.97877318811052));
#33877=CARTESIAN_POINT('Ctrl Pts',(92.5122606053387,-0.0543848059472618,
6.48497847412863));
#33878=CARTESIAN_POINT('Ctrl Pts',(92.5710603568124,-2.04193092337015,6.15535714814456));
#33879=CARTESIAN_POINT('Ctrl Pts',(92.6298601082861,-3.55100669662098,5.10582236305308));
#33880=CARTESIAN_POINT('Ctrl Pts',(92.6886598597598,-5.06008246987181,4.0562875779616));
#33881=CARTESIAN_POINT('Ctrl Pts',(92.7474596112335,-6.06074051980672,2.30766719190671));
#33882=CARTESIAN_POINT('Ctrl Pts',(92.8062593627072,-6.2010939374364,0.474873184744622));
#33883=CARTESIAN_POINT('Ctrl Pts',(92.811327769058,-6.2131920864156,0.316890462832376));
#33884=CARTESIAN_POINT('Ctrl Pts',(92.8163961754088,-6.21924999999989,0.15844527646143));
#33885=CARTESIAN_POINT('Ctrl Pts',(92.8214645817595,-6.21925,4.46288567693365E-12));
#33886=CARTESIAN_POINT('Origin',(28.1999754182402,0.,0.));
#33887=CARTESIAN_POINT('',(90.0749754182402,-6.21925,3.96263669092518E-12));
#33888=CARTESIAN_POINT('',(90.3214645817596,-6.2089008876497,-0.000864123173838216));
#33889=CARTESIAN_POINT('',(28.1999754182402,-6.21925,5.68729293530136E-12));
#33890=CARTESIAN_POINT('Ctrl Pts',(90.0749754182402,-6.21925,4.31616012367526E-12));
#33891=CARTESIAN_POINT('Ctrl Pts',(90.1337751697139,-6.21925000000128,-1.83816020915309));
#33892=CARTESIAN_POINT('Ctrl Pts',(90.1925749211876,-5.35502977485272,-3.65808141345576));
#33893=CARTESIAN_POINT('Ctrl Pts',(90.2513746726613,-3.93049712176172,-4.81977830800576));
#33894=CARTESIAN_POINT('Ctrl Pts',(90.310174424135,-2.50596446867071,-5.98147520255577));
#33895=CARTESIAN_POINT('Ctrl Pts',(90.3689741756087,-0.549389021423145,
-6.46189408921017));
#33896=CARTESIAN_POINT('Ctrl Pts',(90.4277739270824,1.25118869866496,-6.09209302315986));
#33897=CARTESIAN_POINT('Ctrl Pts',(90.4865736785561,3.05176641875306,-5.72229195710956));
#33898=CARTESIAN_POINT('Ctrl Pts',(90.5453734300298,4.66061422074915,-4.50960958425233));
#33899=CARTESIAN_POINT('Ctrl Pts',(90.6041731815035,5.51197192302528,-2.88049233331404));
#33900=CARTESIAN_POINT('Ctrl Pts',(90.6629729329772,6.36332962530142,-1.25137508237576));
#33901=CARTESIAN_POINT('Ctrl Pts',(90.7217726844509,6.44030216377332,0.761847462636957));
#33902=CARTESIAN_POINT('Ctrl Pts',(90.7805724359246,5.71582172177603,2.45121451680045));
#33903=CARTESIAN_POINT('Ctrl Pts',(90.8393721873983,4.99134127977875,4.14058157096394));
#33904=CARTESIAN_POINT('Ctrl Pts',(90.898171938872,3.47978506146823,5.47256790209241));
#33905=CARTESIAN_POINT('Ctrl Pts',(90.9569716903457,1.71270012776048,5.97877318811052));
#33906=CARTESIAN_POINT('Ctrl Pts',(91.0157714418194,-0.0543848059472749,
6.48497847412863));
#33907=CARTESIAN_POINT('Ctrl Pts',(91.0745711932931,-2.04193092337016,6.15535714814456));
#33908=CARTESIAN_POINT('Ctrl Pts',(91.1333709447668,-3.55100669662099,5.10582236305308));
#33909=CARTESIAN_POINT('Ctrl Pts',(91.1921706962405,-5.06008246987182,4.05628757796159));
#33910=CARTESIAN_POINT('Ctrl Pts',(91.2509704477142,-6.06074051980672,2.3076671919067));
#33911=CARTESIAN_POINT('Ctrl Pts',(91.3097701991879,-6.2010939374364,0.474873184744609));
#33912=CARTESIAN_POINT('Ctrl Pts',(91.3148386055387,-6.21319208641561,0.316890462832246));
#33913=CARTESIAN_POINT('Ctrl Pts',(91.3199070118895,-6.2192499999999,0.158445276461182));
#33914=CARTESIAN_POINT('Ctrl Pts',(91.3249754182402,-6.21925,4.09673125512758E-12));
#33915=CARTESIAN_POINT('Ctrl Pts',(90.3214645817596,-6.2089008876497,-0.000864123173838147));
#33916=CARTESIAN_POINT('Ctrl Pts',(90.3499461153202,-6.2120955723698,-0.895010566629414));
#33917=CARTESIAN_POINT('Ctrl Pts',(90.444598183695,-5.61492052568028,-3.86345977911135));
#33918=CARTESIAN_POINT('Ctrl Pts',(90.6054207868836,-1.05335843212328,-7.27672455920159));
#33919=CARTESIAN_POINT('Ctrl Pts',(90.8039323913257,5.54969193399755,-4.82326734659396));
#33920=CARTESIAN_POINT('Ctrl Pts',(90.9693587283609,6.79974118846012,0.887477022389232));
#33921=CARTESIAN_POINT('Ctrl Pts',(91.1016997979888,4.59656587779412,4.55564727731113));
#33922=CARTESIAN_POINT('Ctrl Pts',(91.20095560021,1.86576486459037,6.21632171280966));
#33923=CARTESIAN_POINT('Ctrl Pts',(91.300211402431,-1.32818086979205,6.33389892256676));
#33924=CARTESIAN_POINT('Ctrl Pts',(91.4237143962808,-4.92946548902491,4.60868661393506));
#33925=CARTESIAN_POINT('Ctrl Pts',(91.5141321227237,-6.21048370270169,1.78002491689768));
#33926=CARTESIAN_POINT('Ctrl Pts',(91.5714645817596,-6.22556524348756,-0.00419006153428332));
#33927=CARTESIAN_POINT('Origin',(28.1999754182402,0.,0.));
#33928=CARTESIAN_POINT('',(88.8249754182402,-6.22149727412722,-0.000986937928962441));
#33929=CARTESIAN_POINT('',(89.0714645817595,-6.21806379781386,0.00504561100484663));
#33930=CARTESIAN_POINT('',(28.1999754182402,-6.21925,5.68729293530136E-12));
#33931=CARTESIAN_POINT('Ctrl Pts',(88.8249754182402,-6.22149727412722,-0.00098693792896223));
#33932=CARTESIAN_POINT('Ctrl Pts',(88.8279425763783,-6.22164967457631,-0.0934599545148036));
#33933=CARTESIAN_POINT('Ctrl Pts',(88.8639950019234,-6.19761435895859,-1.21694528678682));
#33934=CARTESIAN_POINT('Ctrl Pts',(88.9331326948756,-5.54069632003458,-3.34410291009848));
#33935=CARTESIAN_POINT('Ctrl Pts',(89.0654737645036,-2.52204036811142,-6.37678665762986));
#33936=CARTESIAN_POINT('Ctrl Pts',(89.2309001015388,3.32104580709813,-6.56000329315107));
#33937=CARTESIAN_POINT('Ctrl Pts',(89.4294117059809,7.31354018950449,-0.7565805928752));
#33938=CARTESIAN_POINT('Ctrl Pts',(89.6279233104229,4.60386296928326,5.73277681905332));
#33939=CARTESIAN_POINT('Ctrl Pts',(89.8264349148652,-2.33008407920169,6.97378639211496));
#33940=CARTESIAN_POINT('Ctrl Pts',(89.9754522841373,-5.91329462628883,3.11473712707665));
#33941=CARTESIAN_POINT('Ctrl Pts',(90.0582991185959,-6.22469949224009,0.524291360883706));
#33942=CARTESIAN_POINT('Ctrl Pts',(90.0749754182403,-6.22196066299615,0.00227071514955785));
#33943=CARTESIAN_POINT('Ctrl Pts',(89.0714645817595,-6.21806379781386,0.0050456110048467));
#33944=CARTESIAN_POINT('Ctrl Pts',(89.1195895731026,-6.20545924076061,-1.50037252384037));
#33945=CARTESIAN_POINT('Ctrl Pts',(89.2338850992598,-4.89889388900873,-5.09517050824349));
#33946=CARTESIAN_POINT('Ctrl Pts',(89.4143511602309,1.12569445119592,-7.26607187285839));
#33947=CARTESIAN_POINT('Ctrl Pts',(89.5797774972661,5.76648339708804,-3.71103286517617));
#33948=CARTESIAN_POINT('Ctrl Pts',(89.7121185668941,6.45131090248977,0.512764686372355));
#33949=CARTESIAN_POINT('Ctrl Pts',(89.8113743691151,5.43739898593206,3.54378701883646));
#33950=CARTESIAN_POINT('Ctrl Pts',(89.9106301713363,3.07374429895899,5.69512387650968));
#33951=CARTESIAN_POINT('Ctrl Pts',(90.0429712409643,-1.06699388433329,6.77389251066956));
#33952=CARTESIAN_POINT('Ctrl Pts',(90.1799160444387,-5.31050817540945,4.44732299061749));
#33953=CARTESIAN_POINT('Ctrl Pts',(90.2837755805062,-6.20467343001778,1.18234064901073));
#33954=CARTESIAN_POINT('Ctrl Pts',(90.3214645817596,-6.2089008876497,-0.000864123173838147));
#33955=CARTESIAN_POINT('Origin',(28.1999754182402,0.,0.));
#33956=CARTESIAN_POINT('',(87.5749754182402,-6.21925,4.04797289438319E-12));
#33957=CARTESIAN_POINT('',(87.8214645817596,-6.22964168097674,-0.000350078226707407));
#33958=CARTESIAN_POINT('',(28.1999754182402,-6.21925,5.68729293530136E-12));
#33959=CARTESIAN_POINT('Ctrl Pts',(87.5749754182403,-6.21906914730504,-0.00133611460555415));
#33960=CARTESIAN_POINT('Ctrl Pts',(87.5975860341608,-6.22215116111062,-0.70980238469718));
#33961=CARTESIAN_POINT('Ctrl Pts',(87.6863671848953,-5.76713295026162,-3.49042167931515));
#33962=CARTESIAN_POINT('Ctrl Pts',(87.8413188704441,-1.69752736119953,-7.15411694879083));
#33963=CARTESIAN_POINT('Ctrl Pts',(88.0398304748858,5.0977681804467,-5.29840012413548));
#33964=CARTESIAN_POINT('Ctrl Pts',(88.2383420793283,7.21666225322758,1.40714967926411));
#33965=CARTESIAN_POINT('Ctrl Pts',(88.4368536837702,2.72150289496444,6.83054979131966));
#33966=CARTESIAN_POINT('Ctrl Pts',(88.6022800208054,-3.0818294938239,6.125881378733));
#33967=CARTESIAN_POINT('Ctrl Pts',(88.7316539322954,-5.75604940176151,2.90933191124067));
#33968=CARTESIAN_POINT('Ctrl Pts',(88.7948573089713,-6.2199503348794,0.93765950029407));
#33969=CARTESIAN_POINT('Ctrl Pts',(88.8249754182402,-6.22149727412722,-0.00098693792896223));
#33970=CARTESIAN_POINT('Ctrl Pts',(87.8214645817596,-6.22964168097674,-0.000350078226707528));
#33971=CARTESIAN_POINT('Ctrl Pts',(87.8230624960711,-6.22971496116889,-0.0500951023154418));
#33972=CARTESIAN_POINT('Ctrl Pts',(87.8908309451966,-6.20535244691635,-2.15974806597762));
#33973=CARTESIAN_POINT('Ctrl Pts',(88.0247699291361,-3.8300746758159,-6.27642545057859));
#33974=CARTESIAN_POINT('Ctrl Pts',(88.1901962661713,2.00917170803365,-6.55647197377879));
#33975=CARTESIAN_POINT('Ctrl Pts',(88.3225373357994,5.25849341829804,-3.77234502052638));
#33976=CARTESIAN_POINT('Ctrl Pts',(88.4217931380204,6.44043681020296,-0.802812469304661));
#33977=CARTESIAN_POINT('Ctrl Pts',(88.5210489402415,6.02365017597241,2.36600476366407));
#33978=CARTESIAN_POINT('Ctrl Pts',(88.6533900098694,3.55723335538306,5.86260919306929));
#33979=CARTESIAN_POINT('Ctrl Pts',(88.8188163469047,-2.17207643043537,7.02460478883646));
#33980=CARTESIAN_POINT('Ctrl Pts',(88.9692029600036,-5.89212743611744,3.19855472586929));
#33981=CARTESIAN_POINT('Ctrl Pts',(89.0534190382886,-6.22279015881442,0.56953586100025));
#33982=CARTESIAN_POINT('Ctrl Pts',(89.0714645817595,-6.21806379781386,0.0050456110048467));
#33983=CARTESIAN_POINT('Origin',(28.1999754182402,0.,0.));
#33984=CARTESIAN_POINT('',(86.3249754182403,-6.21883554189359,3.4186727807411E-5));
#33985=CARTESIAN_POINT('',(86.5714645817596,-6.21915084886221,-0.00012899831342565));
#33986=CARTESIAN_POINT('',(28.1999754182402,-6.21925,5.68729293530136E-12));
#33987=CARTESIAN_POINT('Ctrl Pts',(86.3249754182403,-6.21925,3.56035299831798E-12));
#33988=CARTESIAN_POINT('Ctrl Pts',(86.383775169714,-6.21925000000105,-1.83816020915385));
#33989=CARTESIAN_POINT('Ctrl Pts',(86.4425749211877,-5.35502977485227,-3.65808141345641));
#33990=CARTESIAN_POINT('Ctrl Pts',(86.5013746726614,-3.93049712176113,-4.81977830800624));
#33991=CARTESIAN_POINT('Ctrl Pts',(86.5601744241351,-2.50596446866999,-5.98147520255607));
#33992=CARTESIAN_POINT('Ctrl Pts',(86.6189741756087,-0.549389021422359,
-6.46189408921024));
#33993=CARTESIAN_POINT('Ctrl Pts',(86.6777739270824,1.2511886986657,-6.09209302315971));
#33994=CARTESIAN_POINT('Ctrl Pts',(86.7365736785561,3.05176641875376,-5.72229195710919));
#33995=CARTESIAN_POINT('Ctrl Pts',(86.7953734300298,4.66061422074969,-4.50960958425176));
#33996=CARTESIAN_POINT('Ctrl Pts',(86.8541731815035,5.51197192302563,-2.88049233331337));
#33997=CARTESIAN_POINT('Ctrl Pts',(86.9129729329772,6.36332962530157,-1.25137508237498));
#33998=CARTESIAN_POINT('Ctrl Pts',(86.9717726844509,6.44030216377322,0.76184746263774));
#33999=CARTESIAN_POINT('Ctrl Pts',(87.0305724359246,5.71582172177574,2.45121451680114));
#34000=CARTESIAN_POINT('Ctrl Pts',(87.0893721873983,4.99134127977825,4.14058157096455));
#34001=CARTESIAN_POINT('Ctrl Pts',(87.148171938872,3.47978506146757,5.47256790209283));
#34002=CARTESIAN_POINT('Ctrl Pts',(87.2069716903457,1.71270012775975,5.97877318811073));
#34003=CARTESIAN_POINT('Ctrl Pts',(87.2657714418194,-0.0543848059480628,
6.48497847412862));
#34004=CARTESIAN_POINT('Ctrl Pts',(87.3245711932931,-2.04193092337091,6.15535714814431));
#34005=CARTESIAN_POINT('Ctrl Pts',(87.3833709447668,-3.55100669662161,5.10582236305264));
#34006=CARTESIAN_POINT('Ctrl Pts',(87.4421706962405,-5.06008246987231,4.05628757796098));
#34007=CARTESIAN_POINT('Ctrl Pts',(87.5009704477142,-6.060740519807,2.30766719190597));
#34008=CARTESIAN_POINT('Ctrl Pts',(87.5597701991879,-6.20109393743646,0.474873184743856));
#34009=CARTESIAN_POINT('Ctrl Pts',(87.5648386055387,-6.21319208641563,0.316890462831726));
#34010=CARTESIAN_POINT('Ctrl Pts',(87.5699070118895,-6.2192499999999,0.158445276460897));
#34011=CARTESIAN_POINT('Ctrl Pts',(87.5749754182402,-6.21925,4.04797099527046E-12));
#34012=CARTESIAN_POINT('Ctrl Pts',(86.5714645817596,-6.21353584576935,-0.00743426924668888));
#34013=CARTESIAN_POINT('Ctrl Pts',(86.5927059538535,-6.21863854140484,-0.672800635959472));
#34014=CARTESIAN_POINT('Ctrl Pts',(86.6801178607615,-5.81430299723871,-3.40355548725215));
#34015=CARTESIAN_POINT('Ctrl Pts',(86.8006150350767,-2.69726124705009,-6.30467108265544));
#34016=CARTESIAN_POINT('Ctrl Pts',(86.9329561047044,1.58159360772959,-6.2754204356491));
#34017=CARTESIAN_POINT('Ctrl Pts',(87.0322119069257,4.40104898481893,-4.77016792160538));
#34018=CARTESIAN_POINT('Ctrl Pts',(87.1314677091467,6.1280180343697,-2.08080151735183));
#34019=CARTESIAN_POINT('Ctrl Pts',(87.2638087787747,6.501043828168,2.18186269951808));
#34020=CARTESIAN_POINT('Ctrl Pts',(87.4292351158099,2.87499030196175,6.76737905120017));
#34021=CARTESIAN_POINT('Ctrl Pts',(87.6261488059404,-4.07902303115758,6.0848730030111));
#34022=CARTESIAN_POINT('Ctrl Pts',(87.756891961257,-6.22668038699246,2.00987446213666));
#34023=CARTESIAN_POINT('Ctrl Pts',(87.8214645817596,-6.22964168097674,-0.000350078226707528));
#34024=CARTESIAN_POINT('Origin',(28.1999754182402,0.,0.));
#34025=CARTESIAN_POINT('',(85.0749754182403,-6.22858364363872,0.00435858369765019));
#34026=CARTESIAN_POINT('',(85.3214645817596,-6.21849213708592,0.0005147991858583));
#34027=CARTESIAN_POINT('',(28.1999754182402,-6.21925,5.68729293530136E-12));
#34028=CARTESIAN_POINT('Ctrl Pts',(85.0749754182403,-6.22858364363872,0.00435858369765025));
#34029=CARTESIAN_POINT('Ctrl Pts',(85.1368729497257,-6.21898881198671,-1.92103273188814));
#34030=CARTESIAN_POINT('Ctrl Pts',(85.2649410160251,-4.22400447196293,-5.93097583593628));
#34031=CARTESIAN_POINT('Ctrl Pts',(85.4591796171386,2.59110314784578,-6.88087703525041));
#34032=CARTESIAN_POINT('Ctrl Pts',(85.6576912215807,7.18878928721451,-1.54411691365224));
#34033=CARTESIAN_POINT('Ctrl Pts',(85.8231175586158,5.52605610955549,4.0603940165154));
#34034=CARTESIAN_POINT('Ctrl Pts',(85.9554586282439,1.82556334808452,6.2088371251229));
#34035=CARTESIAN_POINT('Ctrl Pts',(86.0547144304649,-1.36766347836997,6.34454338601461));
#34036=CARTESIAN_POINT('Ctrl Pts',(86.1539702326861,-4.22139086822476,4.90532354914965));
#34037=CARTESIAN_POINT('Ctrl Pts',(86.2440572286111,-5.91414893595505,2.5349313646869));
#34038=CARTESIAN_POINT('Ctrl Pts',(86.3010589571292,-6.21301106946328,0.75031761569158));
#34039=CARTESIAN_POINT('Ctrl Pts',(86.3249754182402,-6.20882463865616,0.000859939640229165));
#34040=CARTESIAN_POINT('Ctrl Pts',(85.3214645817596,-6.21925,3.65831829171925E-12));
#34041=CARTESIAN_POINT('Ctrl Pts',(85.3802643332333,-6.21925000000108,-1.83816020915375));
#34042=CARTESIAN_POINT('Ctrl Pts',(85.439064084707,-5.35502977485233,-3.65808141345632));
#34043=CARTESIAN_POINT('Ctrl Pts',(85.4978638361806,-3.93049712176121,-4.81977830800618));
#34044=CARTESIAN_POINT('Ctrl Pts',(85.5566635876543,-2.50596446867008,-5.98147520255603));
#34045=CARTESIAN_POINT('Ctrl Pts',(85.615463339128,-0.549389021422461,-6.46189408921023));
#34046=CARTESIAN_POINT('Ctrl Pts',(85.6742630906017,1.2511886986656,-6.09209302315973));
#34047=CARTESIAN_POINT('Ctrl Pts',(85.7330628420754,3.05176641875367,-5.72229195710924));
#34048=CARTESIAN_POINT('Ctrl Pts',(85.7918625935491,4.66061422074962,-4.50960958425183));
#34049=CARTESIAN_POINT('Ctrl Pts',(85.8506623450228,5.51197192302559,-2.88049233331346));
#34050=CARTESIAN_POINT('Ctrl Pts',(85.9094620964965,6.36332962530155,-1.25137508237509));
#34051=CARTESIAN_POINT('Ctrl Pts',(85.9682618479702,6.44030216377323,0.761847462637638));
#34052=CARTESIAN_POINT('Ctrl Pts',(86.0270615994439,5.71582172177577,2.45121451680105));
#34053=CARTESIAN_POINT('Ctrl Pts',(86.0858613509176,4.99134127977831,4.14058157096447));
#34054=CARTESIAN_POINT('Ctrl Pts',(86.1446611023913,3.47978506146765,5.47256790209278));
#34055=CARTESIAN_POINT('Ctrl Pts',(86.203460853865,1.71270012775985,5.9787731881107));
#34056=CARTESIAN_POINT('Ctrl Pts',(86.2622606053387,-0.0543848059479607,
6.48497847412862));
#34057=CARTESIAN_POINT('Ctrl Pts',(86.3210603568124,-2.04193092337081,6.15535714814434));
#34058=CARTESIAN_POINT('Ctrl Pts',(86.3798601082861,-3.55100669662153,5.1058223630527));
#34059=CARTESIAN_POINT('Ctrl Pts',(86.4386598597598,-5.06008246987225,4.05628757796106));
#34060=CARTESIAN_POINT('Ctrl Pts',(86.4974596112335,-6.06074051980697,2.30766719190606));
#34061=CARTESIAN_POINT('Ctrl Pts',(86.5562593627072,-6.20109393743645,0.474873184743953));
#34062=CARTESIAN_POINT('Ctrl Pts',(86.561327769058,-6.21319208641564,0.316890462831589));
#34063=CARTESIAN_POINT('Ctrl Pts',(86.5663961754088,-6.21924999999991,0.158445276460524));
#34064=CARTESIAN_POINT('Ctrl Pts',(86.5714645817596,-6.21925,3.43888942317157E-12));
#34065=CARTESIAN_POINT('Origin',(28.1999754182402,0.,0.));
#34066=CARTESIAN_POINT('',(83.8249754182403,-6.21863967025274,-0.0053269228922874));
#34067=CARTESIAN_POINT('',(84.0714645817596,-6.22691982511773,0.00134582525012354));
#34068=CARTESIAN_POINT('',(28.1999754182402,-6.21925,5.68729293530136E-12));
#34069=CARTESIAN_POINT('Ctrl Pts',(83.8249754182403,-6.21863967025274,-0.00532692289228712));
#34070=CARTESIAN_POINT('Ctrl Pts',(83.8403458726941,-6.22330610280407,-0.48602639124095));
#34071=CARTESIAN_POINT('Ctrl Pts',(83.921886861962,-5.95443652093343,-3.03117788366071));
#34072=CARTESIAN_POINT('Ctrl Pts',(84.0695983860438,-2.46216747788131,-6.92806001762949));
#34073=CARTESIAN_POINT('Ctrl Pts',(84.2681099904858,4.49416806949842,-5.81940218769057));
#34074=CARTESIAN_POINT('Ctrl Pts',(84.4335363275211,6.84159716243557,-0.465450279045067));
#34075=CARTESIAN_POINT('Ctrl Pts',(84.565877397149,5.4018620288319,3.56401832285386));
#34076=CARTESIAN_POINT('Ctrl Pts',(84.6651331993702,3.05045783488768,5.72873818258966));
#34077=CARTESIAN_POINT('Ctrl Pts',(84.7643890015912,-0.0581711681516334,
6.47139522045821));
#34078=CARTESIAN_POINT('Ctrl Pts',(84.8967300712192,-4.20511699218411,5.41674134303595));
#34079=CARTESIAN_POINT('Ctrl Pts',(85.000258876769,-6.16516640887946,2.32750288322991));
#34080=CARTESIAN_POINT('Ctrl Pts',(85.0707024149117,-6.22924600846334,0.137275087845278));
#34081=CARTESIAN_POINT('Ctrl Pts',(85.0749754182403,-6.22858364363872,0.00435858369765025));
#34082=CARTESIAN_POINT('Ctrl Pts',(84.0714645817596,-6.22691982511773,0.00134582525012326));
#34083=CARTESIAN_POINT('Ctrl Pts',(84.0989076020114,-6.22489235382799,-0.855356492542834));
#34084=CARTESIAN_POINT('Ctrl Pts',(84.1594358896702,-5.81262401081619,-2.74987092752364));
#34085=CARTESIAN_POINT('Ctrl Pts',(84.253049444736,-3.96930072085848,-5.13501567227216));
#34086=CARTESIAN_POINT('Ctrl Pts',(84.3523052469571,-1.02956513266701,-6.38923591846239));
#34087=CARTESIAN_POINT('Ctrl Pts',(84.4846463165852,3.23560668510475,-6.04606856350603));
#34088=CARTESIAN_POINT('Ctrl Pts',(84.6500726536202,7.15210351133029,-1.70599056920427));
#34089=CARTESIAN_POINT('Ctrl Pts',(84.8485842580625,5.30442784199376,5.09149580831549));
#34090=CARTESIAN_POINT('Ctrl Pts',(85.0470958625043,-1.39861029772509,7.21832207179135));
#34091=CARTESIAN_POINT('Ctrl Pts',(85.2047226370703,-5.7092439301469,3.65406932462159));
#34092=CARTESIAN_POINT('Ctrl Pts',(85.296178876822,-6.21531076597404,0.797672369212536));
#34093=CARTESIAN_POINT('Ctrl Pts',(85.3214645817596,-6.21024711481797,0.00611545682707264));
#34094=CARTESIAN_POINT('Origin',(28.1999754182402,0.,0.));
#34095=CARTESIAN_POINT('',(82.5749754182402,-6.21075901980729,0.000909742482199126));
#34096=CARTESIAN_POINT('',(82.8214645817596,-6.21810878279376,-0.00339757865050971));
#34097=CARTESIAN_POINT('',(28.1999754182402,-6.21925,5.68729293530136E-12));
#34098=CARTESIAN_POINT('Ctrl Pts',(82.5749754182403,-6.21075901980729,0.000909742482198966));
#34099=CARTESIAN_POINT('Ctrl Pts',(82.6099893304765,-6.20925005302336,-1.09762679373399));
#34100=CARTESIAN_POINT('Ctrl Pts',(82.7111737775268,-5.40608907411339,-4.27426631199952));
#34101=CARTESIAN_POINT('Ctrl Pts',(82.8785287593912,-0.323472535169768,
-7.34563502891261));
#34102=CARTESIAN_POINT('Ctrl Pts',(83.0439550964262,4.92520670119462,-4.77141851505581));
#34103=CARTESIAN_POINT('Ctrl Pts',(83.1762961660544,6.42635186854234,-0.7644224263167));
#34104=CARTESIAN_POINT('Ctrl Pts',(83.2755519682753,6.02756024934152,2.40670970572829));
#34105=CARTESIAN_POINT('Ctrl Pts',(83.3748077704965,4.13252826027979,4.98041666551734));
#34106=CARTESIAN_POINT('Ctrl Pts',(83.5071488401245,0.284353283747686,6.85151362148041));
#34107=CARTESIAN_POINT('Ctrl Pts',(83.6572047227057,-4.77560033766816,5.26519608353924));
#34108=CARTESIAN_POINT('Ctrl Pts',(83.7741753378801,-6.20321688953303,1.58340759986397));
#34109=CARTESIAN_POINT('Ctrl Pts',(83.8249754182403,-6.21863967025274,-0.00532692289228712));
#34110=CARTESIAN_POINT('Ctrl Pts',(82.8214645817596,-6.21810878279376,-0.00339757865050951));
#34111=CARTESIAN_POINT('Ctrl Pts',(82.8354657923868,-6.21944953262559,-0.4405939671335));
#34112=CARTESIAN_POINT('Ctrl Pts',(82.882552270421,-6.07008559218604,-1.90917328702513));
#34113=CARTESIAN_POINT('Ctrl Pts',(82.9627240158624,-4.91031465598665,-4.2155841781865));
#34114=CARTESIAN_POINT('Ctrl Pts',(83.0950650854904,-1.43106703177257,-6.70642548947526));
#34115=CARTESIAN_POINT('Ctrl Pts',(83.2604914225255,4.36166608043273,-5.91936292702175));
#34116=CARTESIAN_POINT('Ctrl Pts',(83.4590030269676,7.33784111646791,0.465158087628112));
#34117=CARTESIAN_POINT('Ctrl Pts',(83.6575146314097,3.59080068386597,6.41610744499814));
#34118=CARTESIAN_POINT('Ctrl Pts',(83.8560262358518,-3.45292231992367,6.49155727938758));
#34119=CARTESIAN_POINT('Ctrl Pts',(83.9940095526351,-6.13316871367438,2.4180846706705));
#34120=CARTESIAN_POINT('Ctrl Pts',(84.0658223346043,-6.22733667042163,0.177482641499614));
#34121=CARTESIAN_POINT('Ctrl Pts',(84.0714645817596,-6.22691982511773,0.00134582525012326));
#34122=CARTESIAN_POINT('Origin',(28.1999754182402,0.,0.));
#34123=CARTESIAN_POINT('',(81.3249754182402,-6.22245972074542,0.00511829929418269));
#34124=CARTESIAN_POINT('',(81.5714645817596,-6.21597937799738,0.00149266041878204));
#34125=CARTESIAN_POINT('',(28.1999754182402,-6.21925,5.68729293530136E-12));
#34126=CARTESIAN_POINT('Ctrl Pts',(81.3249754182402,-6.22245972074542,0.00511829929418263));
#34127=CARTESIAN_POINT('Ctrl Pts',(81.379632788259,-6.2062119306234,-1.7015911957153));
#34128=CARTESIAN_POINT('Ctrl Pts',(81.5004606930918,-4.59365834777172,-5.50076823327935));
#34129=CARTESIAN_POINT('Ctrl Pts',(81.6543738653314,0.682176659571807,-6.82339583348686));
#34130=CARTESIAN_POINT('Ctrl Pts',(81.7867149349596,4.41506970477836,-4.73175437719689));
#34131=CARTESIAN_POINT('Ctrl Pts',(81.8859707371805,6.1572775488005,-2.05223472198617));
#34132=CARTESIAN_POINT('Ctrl Pts',(81.9852265394016,6.37104488690502,1.13671765765088));
#34133=CARTESIAN_POINT('Ctrl Pts',(82.1175676090297,4.63949668876505,5.04966990705815));
#34134=CARTESIAN_POINT('Ctrl Pts',(82.2829939460648,-0.749954889722087,
7.3144074348083));
#34135=CARTESIAN_POINT('Ctrl Pts',(82.4464916382707,-5.53259199941689,4.03024244694824));
#34136=CARTESIAN_POINT('Ctrl Pts',(82.5438187956625,-6.21210175204047,0.978426565390665));
#34137=CARTESIAN_POINT('Ctrl Pts',(82.5749754182403,-6.21075901980729,0.000909742482198966));
#34138=CARTESIAN_POINT('Ctrl Pts',(81.5714645817596,-6.21597937799738,0.00149266041878201));
#34139=CARTESIAN_POINT('Ctrl Pts',(81.5720239827622,-6.216009963232,-0.0160310956563993));
#34140=CARTESIAN_POINT('Ctrl Pts',(81.6056686511719,-6.21346008847608,-1.07002792270585));
#34141=CARTESIAN_POINT('Ctrl Pts',(81.7054838543957,-5.42171283747731,-4.19870522938243));
#34142=CARTESIAN_POINT('Ctrl Pts',(81.8709101914306,-0.48919755281723,-7.33646196836831));
#34143=CARTESIAN_POINT('Ctrl Pts',(82.069421795873,5.90490006067872,-4.38091766304837));
#34144=CARTESIAN_POINT('Ctrl Pts',(82.2679334003147,6.88393788382687,2.58296022203711));
#34145=CARTESIAN_POINT('Ctrl Pts',(82.4664450047572,1.55262125162276,7.18695733311437));
#34146=CARTESIAN_POINT('Ctrl Pts',(82.6318713417919,-4.05385301920155,5.53085629844241));
#34147=CARTESIAN_POINT('Ctrl Pts',(82.7502112007931,-5.97891224336876,2.22413772225872));
#34148=CARTESIAN_POINT('Ctrl Pts',(82.8023805249798,-6.21628130182804,0.592513798148406));
#34149=CARTESIAN_POINT('Ctrl Pts',(82.8214645817596,-6.21810878279376,-0.00339757865050951));
#34150=CARTESIAN_POINT('Origin',(28.1999754182402,0.,0.));
#34151=CARTESIAN_POINT('',(80.0749754182403,-6.22591546342771,-0.00639606690001471));
#34152=CARTESIAN_POINT('',(80.3214645817596,-6.21925,3.12193847162856E-12));
#34153=CARTESIAN_POINT('',(28.1999754182402,-6.21925,5.68729293530136E-12));
#34154=CARTESIAN_POINT('Ctrl Pts',(80.0749754182403,-6.22591546342771,-0.00639606690001581));
#34155=CARTESIAN_POINT('Ctrl Pts',(80.0831057112274,-6.22789577682199,-0.259639247857812));
#34156=CARTESIAN_POINT('Ctrl Pts',(80.1574065390285,-6.09902881688988,-2.57131173126798));
#34157=CARTESIAN_POINT('Ctrl Pts',(80.2647926342366,-3.88310974879154,-5.65203984187573));
#34158=CARTESIAN_POINT('Ctrl Pts',(80.3971337038648,0.318133770830362,-6.46383252320411));
#34159=CARTESIAN_POINT('Ctrl Pts',(80.4963895060858,3.37833202016725,-5.5417151612656));
#34160=CARTESIAN_POINT('Ctrl Pts',(80.5956453083068,5.59991621302585,-3.24396029434143));
#34161=CARTESIAN_POINT('Ctrl Pts',(80.7279863779349,6.80296829521341,0.862390903031537));
#34162=CARTESIAN_POINT('Ctrl Pts',(80.89341271497,4.14826379333761,6.07082333459648));
#34163=CARTESIAN_POINT('Ctrl Pts',(81.0919243194122,-2.86075767029707,6.77320823899939));
#34164=CARTESIAN_POINT('Ctrl Pts',(81.2357785538355,-6.035454250839,2.78678910832403));
#34165=CARTESIAN_POINT('Ctrl Pts',(81.3134622534449,-6.22588219579629,0.364623845702632));
#34166=CARTESIAN_POINT('Ctrl Pts',(81.3249754182402,-6.22245972074542,0.00511829929418263));
#34167=CARTESIAN_POINT('Ctrl Pts',(80.3214645817596,-6.21763963428012,0.00313466642206932));
#34168=CARTESIAN_POINT('Ctrl Pts',(80.3747527079517,-6.20169098464531,-1.66223637650542));
#34169=CARTESIAN_POINT('Ctrl Pts',(80.4942113689577,-4.66823370288436,-5.40918680826147));
#34170=CARTESIAN_POINT('Ctrl Pts',(80.6798405647781,1.68251786406567,-7.15747287344582));
#34171=CARTESIAN_POINT('Ctrl Pts',(80.8783521692202,6.92514205415142,-2.4703626913545));
#34172=CARTESIAN_POINT('Ctrl Pts',(81.0768637736622,5.82471539119074,4.48727969605447));
#34173=CARTESIAN_POINT('Ctrl Pts',(81.2422901106974,0.473544591506288,6.84104167617517));
#34174=CARTESIAN_POINT('Ctrl Pts',(81.3746311803253,-3.55762461323784,5.40607501755736));
#34175=CARTESIAN_POINT('Ctrl Pts',(81.473327581544,-5.71290909288839,3.07047161723339));
#34176=CARTESIAN_POINT('Ctrl Pts',(81.5389387153552,-6.21420102713517,1.0203956411079));
#34177=CARTESIAN_POINT('Ctrl Pts',(81.5714645817596,-6.21597937799738,0.00149266041878201));
#34178=CARTESIAN_POINT('Origin',(28.1999754182402,0.,0.));
#34179=CARTESIAN_POINT('',(78.8249754182403,-6.21868393922028,3.57448842112454E-5));
#34180=CARTESIAN_POINT('',(79.0714645817596,-6.21925,2.63432203795717E-12));
#34181=CARTESIAN_POINT('',(28.1999754182402,-6.21925,5.68729293530136E-12));
#34182=CARTESIAN_POINT('Ctrl Pts',(78.8249754182403,-6.20725553121229,0.000757411355485488));
#34183=CARTESIAN_POINT('Ctrl Pts',(78.8527491690098,-6.20985090167876,-0.869958336885441));
#34184=CARTESIAN_POINT('Ctrl Pts',(78.9136081871864,-5.83503896856034,-2.77734718629318));
#34185=CARTESIAN_POINT('Ctrl Pts',(79.0075524727701,-3.92908674363906,-5.14243301805027));
#34186=CARTESIAN_POINT('Ctrl Pts',(79.106808274991,-0.996518304073061,-6.41332093667049));
#34187=CARTESIAN_POINT('Ctrl Pts',(79.2060640772121,2.18341903006714,-6.09220988831756));
#34188=CARTESIAN_POINT('Ctrl Pts',(79.33840514684,5.75275644429788,-3.73227664943248));
#34189=CARTESIAN_POINT('Ctrl Pts',(79.5038314838753,7.08686629844,1.95941688444093));
#34190=CARTESIAN_POINT('Ctrl Pts',(79.7023430883174,2.18670980208234,7.01987069243372));
#34191=CARTESIAN_POINT('Ctrl Pts',(79.8927243997723,-4.42763839203692,5.7020875320387));
#34192=CARTESIAN_POINT('Ctrl Pts',(80.0169351764133,-6.21177847371782,1.80144720358636));
#34193=CARTESIAN_POINT('Ctrl Pts',(80.0749754182403,-6.22591546342771,-0.00639606690001581));
#34194=CARTESIAN_POINT('Ctrl Pts',(79.0714645817596,-6.21925,2.98784547070725E-12));
#34195=CARTESIAN_POINT('Ctrl Pts',(79.1302643332333,-6.21925000000088,-1.83816020915454));
#34196=CARTESIAN_POINT('Ctrl Pts',(79.189064084707,-5.35502977485182,-3.65808141345713));
#34197=CARTESIAN_POINT('Ctrl Pts',(79.2478638361807,-3.93049712176041,-4.81977830800682));
#34198=CARTESIAN_POINT('Ctrl Pts',(79.3066635876544,-2.505964468669,-5.98147520255652));
#34199=CARTESIAN_POINT('Ctrl Pts',(79.3654633391281,-0.549389021421145,
-6.46189408921037));
#34200=CARTESIAN_POINT('Ctrl Pts',(79.4242630906018,1.25118869866695,-6.09209302315946));
#34201=CARTESIAN_POINT('Ctrl Pts',(79.4830628420755,3.05176641875505,-5.72229195710854));
#34202=CARTESIAN_POINT('Ctrl Pts',(79.5418625935492,4.66061422075082,-4.50960958425064));
#34203=CARTESIAN_POINT('Ctrl Pts',(79.6006623450229,5.51197192302639,-2.88049233331193));
#34204=CARTESIAN_POINT('Ctrl Pts',(79.6594620964966,6.36332962530195,-1.25137508237321));
#34205=CARTESIAN_POINT('Ctrl Pts',(79.7182618479703,6.44030216377303,0.761847462639688));
#34206=CARTESIAN_POINT('Ctrl Pts',(79.777061599444,5.71582172177495,2.45121451680297));
#34207=CARTESIAN_POINT('Ctrl Pts',(79.8358613509177,4.99134127977688,4.14058157096625));
#34208=CARTESIAN_POINT('Ctrl Pts',(79.8946611023914,3.47978506146562,5.47256790209411));
#34209=CARTESIAN_POINT('Ctrl Pts',(79.9534608538651,1.7127001277575,5.97877318811137));
#34210=CARTESIAN_POINT('Ctrl Pts',(80.0122606053388,-0.0543848059506163,
6.48497847412863));
#34211=CARTESIAN_POINT('Ctrl Pts',(80.0710603568125,-2.04193092337348,6.15535714814349));
#34212=CARTESIAN_POINT('Ctrl Pts',(80.1298601082862,-3.55100669662382,5.10582236305111));
#34213=CARTESIAN_POINT('Ctrl Pts',(80.1886598597599,-5.06008246987417,4.05628757795872));
#34214=CARTESIAN_POINT('Ctrl Pts',(80.2474596112336,-6.06074051980812,2.30766719190311));
#34215=CARTESIAN_POINT('Ctrl Pts',(80.3062593627073,-6.20109393743669,0.474873184740817));
#34216=CARTESIAN_POINT('Ctrl Pts',(80.3113277690581,-6.21319208641573,0.316890462829387));
#34217=CARTESIAN_POINT('Ctrl Pts',(80.3163961754088,-6.21924999999992,0.158445276459264));
#34218=CARTESIAN_POINT('Ctrl Pts',(80.3214645817596,-6.21925,3.12194003490965E-12));
#34219=CARTESIAN_POINT('Origin',(28.1999754182402,0.,0.));
#34220=CARTESIAN_POINT('',(77.5749754182403,-6.21925,2.62169104890118E-12));
#34221=CARTESIAN_POINT('',(77.8214645817596,-6.20978691806976,-0.00197117650404144));
#34222=CARTESIAN_POINT('',(28.1999754182402,-6.21925,5.68729293530136E-12));
#34223=CARTESIAN_POINT('Ctrl Pts',(77.5749754182403,-6.21925,2.97521448165126E-12));
#34224=CARTESIAN_POINT('Ctrl Pts',(77.633775169714,-6.21925000000088,-1.83816020915432));
#34225=CARTESIAN_POINT('Ctrl Pts',(77.6925749211877,-5.35502977485205,-3.65808141345668));
#34226=CARTESIAN_POINT('Ctrl Pts',(77.7513746726614,-3.93049712176095,-4.81977830800639));
#34227=CARTESIAN_POINT('Ctrl Pts',(77.8101744241351,-2.50596446866985,-5.98147520255609));
#34228=CARTESIAN_POINT('Ctrl Pts',(77.8689741756087,-0.549389021422371,
-6.4618940892102));
#34229=CARTESIAN_POINT('Ctrl Pts',(77.9277739270824,1.25118869866558,-6.09209302315974));
#34230=CARTESIAN_POINT('Ctrl Pts',(77.9865736785561,3.05176641875353,-5.72229195710927));
#34231=CARTESIAN_POINT('Ctrl Pts',(78.0453734300298,4.6606142207494,-4.50960958425201));
#34232=CARTESIAN_POINT('Ctrl Pts',(78.1041731815035,5.51197192302541,-2.88049233331379));
#34233=CARTESIAN_POINT('Ctrl Pts',(78.1629729329772,6.36332962530142,-1.25137508237558));
#34234=CARTESIAN_POINT('Ctrl Pts',(78.2217726844509,6.44030216377328,0.76184746263699));
#34235=CARTESIAN_POINT('Ctrl Pts',(78.2805724359246,5.71582172177606,2.45121451680038));
#34236=CARTESIAN_POINT('Ctrl Pts',(78.3393721873983,4.99134127977885,4.14058157096377));
#34237=CARTESIAN_POINT('Ctrl Pts',(78.398171938872,3.4797850614685,5.47256790209221));
#34238=CARTESIAN_POINT('Ctrl Pts',(78.4569716903457,1.71270012776089,5.9787731881104));
#34239=CARTESIAN_POINT('Ctrl Pts',(78.5157714418194,-0.0543848059467164,
6.4849784741286));
#34240=CARTESIAN_POINT('Ctrl Pts',(78.5745711932931,-2.04193092336948,6.15535714814475));
#34241=CARTESIAN_POINT('Ctrl Pts',(78.6333709447668,-3.55100669662035,5.10582236305352));
#34242=CARTESIAN_POINT('Ctrl Pts',(78.6921706962405,-5.06008246987121,4.0562875779623));
#34243=CARTESIAN_POINT('Ctrl Pts',(78.7509704477142,-6.06074051980631,2.30766719190769));
#34244=CARTESIAN_POINT('Ctrl Pts',(78.8097701991879,-6.20109393743632,0.47487318474574));
#34245=CARTESIAN_POINT('Ctrl Pts',(78.8148386055387,-6.2131920864156,0.316890462832674));
#34246=CARTESIAN_POINT('Ctrl Pts',(78.8199070118895,-6.21924999999992,0.158445276460901));
#34247=CARTESIAN_POINT('Ctrl Pts',(78.8249754182403,-6.21925,3.10930904585366E-12));
#34248=CARTESIAN_POINT('Ctrl Pts',(77.8214645817596,-6.20978691806976,-0.00197117650404123));
#34249=CARTESIAN_POINT('Ctrl Pts',(77.8478690887026,-6.21394152490341,-0.830640096174487));
#34250=CARTESIAN_POINT('Ctrl Pts',(77.9404441304595,-5.67565032115918,-3.73163537846471));
#34251=CARTESIAN_POINT('Ctrl Pts',(78.0991897070306,-1.28071754910471,-7.24016897982555));
#34252=CARTESIAN_POINT('Ctrl Pts',(78.2977013114727,5.39592604241165,-4.99469424527876));
#34253=CARTESIAN_POINT('Ctrl Pts',(78.4631276485078,6.82419817520737,0.674103078769445));
#34254=CARTESIAN_POINT('Ctrl Pts',(78.5954687181358,4.73697475670672,4.40946823761063));
#34255=CARTESIAN_POINT('Ctrl Pts',(78.6947245203569,2.0595182708145,6.1548451369039));
#34256=CARTESIAN_POINT('Ctrl Pts',(78.793980322578,-1.12917895789654,6.37238533558803));
#34257=CARTESIAN_POINT('Ctrl Pts',(78.9195603430456,-4.8441674685037,4.73369282734356));
#34258=CARTESIAN_POINT('Ctrl Pts',(79.012055096106,-6.21390045877809,1.84473924277232));
#34259=CARTESIAN_POINT('Ctrl Pts',(79.0714645817595,-6.22720257754346,-0.00302929506990259));
#34260=CARTESIAN_POINT('Origin',(28.1999754182402,0.,0.));
#34261=CARTESIAN_POINT('',(76.3249754182403,-6.22173704813553,-0.000300768587064016));
#34262=CARTESIAN_POINT('',(76.5714645817596,-6.21633441253698,0.00478628877724901));
#34263=CARTESIAN_POINT('',(28.1999754182402,-6.21925,5.68729293530136E-12));
#34264=CARTESIAN_POINT('Ctrl Pts',(76.3249754182403,-6.22173704813553,-0.000300768587063625));
#34265=CARTESIAN_POINT('Ctrl Pts',(76.3258655497607,-6.22175262900424,-0.0280386865486988));
#34266=CARTESIAN_POINT('Ctrl Pts',(76.3598409486881,-6.2149600094303,-1.08675627772139));
#34267=CARTESIAN_POINT('Ctrl Pts',(76.4269016150225,-5.64270178030442,-3.1689519723282));
#34268=CARTESIAN_POINT('Ctrl Pts',(76.5592426846506,-2.72049697200563,-6.29467965193754));
#34269=CARTESIAN_POINT('Ctrl Pts',(76.7246690216857,3.1139858635671,-6.66078677788813));
#34270=CARTESIAN_POINT('Ctrl Pts',(76.9231806261278,7.28626036027289,-0.985238173931595));
#34271=CARTESIAN_POINT('Ctrl Pts',(77.1216922305699,4.78113090820971,5.58579193450243));
#34272=CARTESIAN_POINT('Ctrl Pts',(77.3202038350121,-2.11055225112471,7.0433342710871));
#34273=CARTESIAN_POINT('Ctrl Pts',(77.4712982309021,-5.86445747246485,3.2461908392673));
#34274=CARTESIAN_POINT('Ctrl Pts',(77.5562220919782,-6.22385504227548,0.589316613379467));
#34275=CARTESIAN_POINT('Ctrl Pts',(77.5749754182403,-6.22088517383465,0.00203704096300435));
#34276=CARTESIAN_POINT('Ctrl Pts',(76.5714645817596,-6.21633441253698,0.00478628877724929));
#34277=CARTESIAN_POINT('Ctrl Pts',(76.6175125464849,-6.20517767444331,-1.43667693955316));
#34278=CARTESIAN_POINT('Ctrl Pts',(76.7297310460244,-4.98752806823633,-4.96640378610114));
#34279=CARTESIAN_POINT('Ctrl Pts',(76.9081200803781,0.897600199059924,-7.29776009071585));
#34280=CARTESIAN_POINT('Ctrl Pts',(77.0735464174129,5.64744158313445,-3.88979424396703));
#34281=CARTESIAN_POINT('Ctrl Pts',(77.2058874870412,6.46420439911098,0.31048586229469));
#34282=CARTESIAN_POINT('Ctrl Pts',(77.3051432892621,5.54570835728657,3.37177297323113));
#34283=CARTESIAN_POINT('Ctrl Pts',(77.4043990914832,3.2505835667813,5.59607420068252));
#34284=CARTESIAN_POINT('Ctrl Pts',(77.5367401611112,-0.854341364942577,
6.80398387178119));
#34285=CARTESIAN_POINT('Ctrl Pts',(77.6757619912035,-5.23406692997655,4.57819005869191));
#34286=CARTESIAN_POINT('Ctrl Pts',(77.7816985538885,-6.20352994794352,1.24603059178104));
#34287=CARTESIAN_POINT('Ctrl Pts',(77.8214645817596,-6.20978691806976,-0.00197117650404123));
#34288=CARTESIAN_POINT('Origin',(28.1999754182402,0.,0.));
#34289=CARTESIAN_POINT('',(75.0749754182403,-6.21925,2.53026332525108E-12));
#34290=CARTESIAN_POINT('',(75.3214645817596,-6.22966011066701,0.000792207867037114));
#34291=CARTESIAN_POINT('',(28.1999754182402,-6.21925,5.68729293530136E-12));
#34292=CARTESIAN_POINT('Ctrl Pts',(75.0749754182403,-6.22001023982655,-0.00175185933932603));
#34293=CARTESIAN_POINT('Ctrl Pts',(75.0955090075431,-6.22308363120507,-0.644970145081011));
#34294=CARTESIAN_POINT('Ctrl Pts',(75.18221313166,-5.82062366491697,-3.35890160914945));
#34295=CARTESIAN_POINT('Ctrl Pts',(75.3350877905908,-1.92073099598895,-7.09744889988669));
#34296=CARTESIAN_POINT('Ctrl Pts',(75.533599395033,4.92934482030065,-5.45544168096722));
#34297=CARTESIAN_POINT('Ctrl Pts',(75.7321109994751,7.25718867309859,1.18046468258034));
#34298=CARTESIAN_POINT('Ctrl Pts',(75.9306226039172,2.93407158228261,6.74197392506965));
#34299=CARTESIAN_POINT('Ctrl Pts',(76.0960489409524,-2.88848170832391,6.21938655461771));
#34300=CARTESIAN_POINT('Ctrl Pts',(76.22749987906,-5.70664773980729,3.03788962666509));
#34301=CARTESIAN_POINT('Ctrl Pts',(76.2927802823537,-6.22117350423921,1.00295101784076));
#34302=CARTESIAN_POINT('Ctrl Pts',(76.3249754182403,-6.22173704813553,-0.000300768587063625));
#34303=CARTESIAN_POINT('Ctrl Pts',(75.3214645817596,-6.22966011066701,0.000792207867037168));
#34304=CARTESIAN_POINT('Ctrl Pts',(75.3871560042675,-6.22706287267145,-2.04425958841946));
#34305=CARTESIAN_POINT('Ctrl Pts',(75.5190179615893,-4.00786877131307,-6.15474593912649));
#34306=CARTESIAN_POINT('Ctrl Pts',(75.6839651863182,1.80286576781962,-6.61617493105383));
#34307=CARTESIAN_POINT('Ctrl Pts',(75.8163062559463,5.13778071835795,-3.93516826512113));
#34308=CARTESIAN_POINT('Ctrl Pts',(75.9155620581673,6.41213741680385,-1.0041055296563));
#34309=CARTESIAN_POINT('Ctrl Pts',(76.0148178603885,6.09478893729921,2.1762095014379));
#34310=CARTESIAN_POINT('Ctrl Pts',(76.1471589300164,3.73908041305424,5.74833657329857));
#34311=CARTESIAN_POINT('Ctrl Pts',(76.3125852670516,-1.95103068448381,7.08917962300208));
#34312=CARTESIAN_POINT('Ctrl Pts',(76.4650489067683,-5.84208075630458,3.330294435224));
#34313=CARTESIAN_POINT('Ctrl Pts',(76.5513420116709,-6.22120981247244,0.634693495648045));
#34314=CARTESIAN_POINT('Ctrl Pts',(76.5714645817596,-6.21633441253698,0.00478628877724929));
#34315=CARTESIAN_POINT('Origin',(28.1999754182402,0.,0.));
#34316=CARTESIAN_POINT('',(73.8249754182403,-6.21908946014578,2.83535676061311E-7));
#34317=CARTESIAN_POINT('',(74.0714645817596,-6.21923049956772,-3.95732063914942E-5));
#34318=CARTESIAN_POINT('',(28.1999754182402,-6.21925,5.68729293530136E-12));
#34319=CARTESIAN_POINT('Ctrl Pts',(73.8249754182403,-6.21925,2.57293078904406E-12));
#34320=CARTESIAN_POINT('Ctrl Pts',(73.883775169714,-6.21925000000076,-1.83816020915484));
#34321=CARTESIAN_POINT('Ctrl Pts',(73.9425749211877,-5.35502977485169,-3.65808141345726));
#34322=CARTESIAN_POINT('Ctrl Pts',(74.0013746726614,-3.93049712176036,-4.81977830800686));
#34323=CARTESIAN_POINT('Ctrl Pts',(74.0601744241351,-2.50596446866904,-5.98147520255647));
#34324=CARTESIAN_POINT('Ctrl Pts',(74.1189741756088,-0.549389021421334,
-6.46189408921033));
#34325=CARTESIAN_POINT('Ctrl Pts',(74.1777739270825,1.25118869866667,-6.09209302315951));
#34326=CARTESIAN_POINT('Ctrl Pts',(74.2365736785562,3.05176641875466,-5.7222919571087));
#34327=CARTESIAN_POINT('Ctrl Pts',(74.2953734300299,4.66061422075041,-4.50960958425102));
#34328=CARTESIAN_POINT('Ctrl Pts',(74.3541731815036,5.51197192302609,-2.8804923333125));
#34329=CARTESIAN_POINT('Ctrl Pts',(74.4129729329773,6.36332962530177,-1.25137508237398));
#34330=CARTESIAN_POINT('Ctrl Pts',(74.471772684451,6.4403021637731,0.761847462638762));
#34331=CARTESIAN_POINT('Ctrl Pts',(74.5305724359247,5.71582172177535,2.45121451680205));
#34332=CARTESIAN_POINT('Ctrl Pts',(74.5893721873984,4.99134127977759,4.14058157096534));
#34333=CARTESIAN_POINT('Ctrl Pts',(74.648171938872,3.4797850614667,5.47256790209339));
#34334=CARTESIAN_POINT('Ctrl Pts',(74.7069716903457,1.7127001277588,5.978773188111));
#34335=CARTESIAN_POINT('Ctrl Pts',(74.7657714418194,-0.0543848059490926,
6.48497847412861));
#34336=CARTESIAN_POINT('Ctrl Pts',(74.8245711932931,-2.04193092337188,6.15535714814398));
#34337=CARTESIAN_POINT('Ctrl Pts',(74.8833709447668,-3.55100669662242,5.10582236305208));
#34338=CARTESIAN_POINT('Ctrl Pts',(74.9421706962405,-5.06008246987296,4.05628757796018));
#34339=CARTESIAN_POINT('Ctrl Pts',(75.0009704477142,-6.06074051980737,2.307667191905));
#34340=CARTESIAN_POINT('Ctrl Pts',(75.0597701991879,-6.20109393743654,0.474873184742871));
#34341=CARTESIAN_POINT('Ctrl Pts',(75.0648386055387,-6.21319208641569,0.316890462830563));
#34342=CARTESIAN_POINT('Ctrl Pts',(75.0699070118895,-6.21924999999994,0.158445276459556));
#34343=CARTESIAN_POINT('Ctrl Pts',(75.0749754182403,-6.21925,2.53026363687142E-12));
#34344=CARTESIAN_POINT('Ctrl Pts',(74.0714645817596,-6.21535782541014,-0.00789858458239298));
#34345=CARTESIAN_POINT('Ctrl Pts',(74.0906289272359,-6.22045708227677,-0.607720104182565));
#34346=CARTESIAN_POINT('Ctrl Pts',(74.1759638075261,-5.86589957661036,-3.27147217734002));
#34347=CARTESIAN_POINT('Ctrl Pts',(74.2943839552234,-2.89337352700839,-6.21711227638719));
#34348=CARTESIAN_POINT('Ctrl Pts',(74.4267250248515,1.38429868618496,-6.32187133024273));
#34349=CARTESIAN_POINT('Ctrl Pts',(74.5259808270725,4.24950930786462,-4.9056503007122));
#34350=CARTESIAN_POINT('Ctrl Pts',(74.6252366292937,6.05985073959253,-2.27168416620927));
#34351=CARTESIAN_POINT('Ctrl Pts',(74.7575776989216,6.5661819132465,1.9772078337143));
#34352=CARTESIAN_POINT('Ctrl Pts',(74.9230040359569,3.08550547279318,6.67402760129288));
#34353=CARTESIAN_POINT('Ctrl Pts',(75.1215156403989,-3.94304652828918,6.20585758518567));
#34354=CARTESIAN_POINT('Ctrl Pts',(75.2543358223332,-6.22415247288678,2.09056984967631));
#34355=CARTESIAN_POINT('Ctrl Pts',(75.3209854694534,-6.22967905330272,0.0157075414827555));
#34356=CARTESIAN_POINT('Ctrl Pts',(75.3214645817596,-6.22966011066701,0.000792207867037168));
#34357=CARTESIAN_POINT('Origin',(28.1999754182402,0.,0.));
#34358=CARTESIAN_POINT('',(72.5749754182403,-6.22725864519176,0.00554552405307109));
#34359=CARTESIAN_POINT('',(72.8214645817596,-6.217957588601,0.000688194671020262));
#34360=CARTESIAN_POINT('',(28.1999754182402,-6.21925,5.68729293530136E-12));
#34361=CARTESIAN_POINT('Ctrl Pts',(72.5749754182403,-6.22725864519176,0.00554552405307093));
#34362=CARTESIAN_POINT('Ctrl Pts',(72.634795923108,-6.21476230695049,-1.85648529413867));
#34363=CARTESIAN_POINT('Ctrl Pts',(72.7607869627898,-4.33519792882598,-5.80824127579764));
#34364=CARTESIAN_POINT('Ctrl Pts',(72.9529485372856,2.37438354046372,-6.95863454231163));
#34365=CARTESIAN_POINT('Ctrl Pts',(73.1514601417277,7.13688992541174,-1.76848755210188));
#34366=CARTESIAN_POINT('Ctrl Pts',(73.3168864787627,5.65050896588544,3.88535316654217));
#34367=CARTESIAN_POINT('Ctrl Pts',(73.4492275483909,2.01909789486699,6.14862180311659));
#34368=CARTESIAN_POINT('Ctrl Pts',(73.5484833506118,-1.16830659219089,6.38426173854624));
#34369=CARTESIAN_POINT('Ctrl Pts',(73.647739152833,-4.06570784309721,5.0351131850683));
#34370=CARTESIAN_POINT('Ctrl Pts',(73.7399031753757,-5.87258511218837,2.66549161737149));
#34371=CARTESIAN_POINT('Ctrl Pts',(73.7989819305115,-6.2112958543,0.814794971644609));
#34372=CARTESIAN_POINT('Ctrl Pts',(73.8249754182403,-6.2078499707538,2.01338545920832E-5));
#34373=CARTESIAN_POINT('Ctrl Pts',(72.8214645817596,-6.21925,1.96384921694517E-12));
#34374=CARTESIAN_POINT('Ctrl Pts',(72.8802643332333,-6.21925000000058,-1.83816020915533));
#34375=CARTESIAN_POINT('Ctrl Pts',(72.939064084707,-5.35502977485145,-3.65808141345755));
#34376=CARTESIAN_POINT('Ctrl Pts',(72.9978638361807,-3.93049712176017,-4.81977830800702));
#34377=CARTESIAN_POINT('Ctrl Pts',(73.0566635876544,-2.50596446866888,-5.9814752025565));
#34378=CARTESIAN_POINT('Ctrl Pts',(73.1154633391281,-0.54938902142132,-6.46189408921029));
#34379=CARTESIAN_POINT('Ctrl Pts',(73.1742630906018,1.25118869866657,-6.09209302315953));
#34380=CARTESIAN_POINT('Ctrl Pts',(73.2330628420755,3.05176641875446,-5.72229195710877));
#34381=CARTESIAN_POINT('Ctrl Pts',(73.2918625935492,4.66061422075014,-4.50960958425125));
#34382=CARTESIAN_POINT('Ctrl Pts',(73.3506623450229,5.51197192302588,-2.8804923333129));
#34383=CARTESIAN_POINT('Ctrl Pts',(73.4094620964966,6.36332962530162,-1.25137508237454));
#34384=CARTESIAN_POINT('Ctrl Pts',(73.4682618479702,6.44030216377315,0.761847462638037));
#34385=CARTESIAN_POINT('Ctrl Pts',(73.5270615994439,5.71582172177566,2.45121451680131));
#34386=CARTESIAN_POINT('Ctrl Pts',(73.5858613509176,4.99134127977817,4.14058157096459));
#34387=CARTESIAN_POINT('Ctrl Pts',(73.6446611023913,3.4797850614676,5.47256790209277));
#34388=CARTESIAN_POINT('Ctrl Pts',(73.703460853865,1.71270012775992,5.97877318811068));
#34389=CARTESIAN_POINT('Ctrl Pts',(73.7622606053387,-0.0543848059477714,
6.48497847412859));
#34390=CARTESIAN_POINT('Ctrl Pts',(73.8210603568124,-2.04193092337049,6.15535714814441));
#34391=CARTESIAN_POINT('Ctrl Pts',(73.8798601082861,-3.55100669662118,5.10582236305294));
#34392=CARTESIAN_POINT('Ctrl Pts',(73.9386598597598,-5.06008246987187,4.05628757796147));
#34393=CARTESIAN_POINT('Ctrl Pts',(73.9974596112335,-6.06074051980669,2.3076671919067));
#34394=CARTESIAN_POINT('Ctrl Pts',(74.0562593627072,-6.20109393743639,0.474873184744731));
#34395=CARTESIAN_POINT('Ctrl Pts',(74.061327769058,-6.21319208641565,0.316890462831781));
#34396=CARTESIAN_POINT('Ctrl Pts',(74.0663961754088,-6.21924999999994,0.158445276460126));
#34397=CARTESIAN_POINT('Ctrl Pts',(74.0714645817596,-6.21925,2.45146721389765E-12));
#34398=CARTESIAN_POINT('Origin',(28.1999754182402,0.,0.));
#34399=CARTESIAN_POINT('',(71.3249754182403,-6.22194821980233,-0.00360940077133112));
#34400=CARTESIAN_POINT('',(71.5714645817596,-6.22570420439633,0.00188724029056356));
#34401=CARTESIAN_POINT('',(28.1999754182402,-6.21925,5.68729293530136E-12));
#34402=CARTESIAN_POINT('Ctrl Pts',(71.3249754182403,-6.22194821980233,-0.00360940077133092));
#34403=CARTESIAN_POINT('Ctrl Pts',(71.3382688460764,-6.22445124236017,-0.418740319735753));
#34404=CARTESIAN_POINT('Ctrl Pts',(71.4177328087265,-5.98942607440445,-2.89665130682511));
#34405=CARTESIAN_POINT('Ctrl Pts',(71.563367306191,-2.68617674612466,-6.85019204663737));
#34406=CARTESIAN_POINT('Ctrl Pts',(71.7618789106327,4.31461801077602,-5.95570943739811));
#34407=CARTESIAN_POINT('Ctrl Pts',(71.9273052476681,6.82127674849029,-0.680243620698351));
#34408=CARTESIAN_POINT('Ctrl Pts',(72.059646317296,5.51192719551105,3.39346452184477));
#34409=CARTESIAN_POINT('Ctrl Pts',(72.1589021195172,3.22776268544752,5.63020767552143));
#34410=CARTESIAN_POINT('Ctrl Pts',(72.2581579217381,0.144787652460555,6.47013157578351));
#34411=CARTESIAN_POINT('Ctrl Pts',(72.3904989913663,-4.03362152721484,5.54570745472594));
#34412=CARTESIAN_POINT('Ctrl Pts',(72.4961048235336,-6.13049964680174,2.45871254298357));
#34413=CARTESIAN_POINT('Ctrl Pts',(72.568625388294,-6.22858514890861,0.20320268998025));
#34414=CARTESIAN_POINT('Ctrl Pts',(72.5749754182403,-6.22725864519176,0.00554552405307093));
#34415=CARTESIAN_POINT('Ctrl Pts',(71.5714645817596,-6.22570420439633,0.00188724029056342));
#34416=CARTESIAN_POINT('Ctrl Pts',(71.5968305753937,-6.22320179469496,-0.79041573268228));
#34417=CARTESIAN_POINT('Ctrl Pts',(71.6552818364349,-5.85767767178159,-2.62081709736886));
#34418=CARTESIAN_POINT('Ctrl Pts',(71.7468183648829,-4.12753807040063,-5.00810542026236));
#34419=CARTESIAN_POINT('Ctrl Pts',(71.8460741671042,-1.22942858196295,-6.35390206362266));
#34420=CARTESIAN_POINT('Ctrl Pts',(71.978415236732,3.04488676341186,-6.14439894507291));
#34421=CARTESIAN_POINT('Ctrl Pts',(72.1438415737674,7.09505541724423,-1.92914383180871));
#34422=CARTESIAN_POINT('Ctrl Pts',(72.3423531782092,5.46132883333844,4.92289529580099));
#34423=CARTESIAN_POINT('Ctrl Pts',(72.5408647826516,-1.17190946057312,7.25857562521031));
#34424=CARTESIAN_POINT('Ctrl Pts',(72.7005685838348,-5.65024837779282,3.78590359445975));
#34425=CARTESIAN_POINT('Ctrl Pts',(72.7941018502042,-6.21330002205454,0.862522468085002));
#34426=CARTESIAN_POINT('Ctrl Pts',(72.8214645817596,-6.20893906029042,0.0054904605059336));
#34427=CARTESIAN_POINT('Origin',(28.1999754182402,0.,0.));
#34428=CARTESIAN_POINT('',(70.0749754182403,-6.21806317550423,-0.000299885513699476));
#34429=CARTESIAN_POINT('',(70.3214645817596,-6.22327189076832,-0.00449888440332335));
#34430=CARTESIAN_POINT('',(28.1999754182402,-6.21925,5.68729293530136E-12));
#34431=CARTESIAN_POINT('Ctrl Pts',(70.0749754182403,-6.20699959075668,-0.00309542000869176));
#34432=CARTESIAN_POINT('Ctrl Pts',(70.1079123038589,-6.20822260668311,-1.03541925636434));
#34433=CARTESIAN_POINT('Ctrl Pts',(70.2070197242914,-5.47881021611929,-4.13832027487605));
#34434=CARTESIAN_POINT('Ctrl Pts',(70.3722976795382,-0.557063823628739,
-7.3341557210225));
#34435=CARTESIAN_POINT('Ctrl Pts',(70.5708092839802,5.85298547448848,-4.44184497426088));
#34436=CARTESIAN_POINT('Ctrl Pts',(70.7693208884224,6.91261030511504,2.50813707913662));
#34437=CARTESIAN_POINT('Ctrl Pts',(70.9678324928645,1.6305555301296,7.17107975691506));
#34438=CARTESIAN_POINT('Ctrl Pts',(71.1332588298994,-3.99925385407112,5.57258592607248));
#34439=CARTESIAN_POINT('Ctrl Pts',(71.2523064716916,-5.96060023780131,2.26929551249555));
#34440=CARTESIAN_POINT('Ctrl Pts',(71.3051835786694,-6.21822160981746,0.614455755210577));
#34441=CARTESIAN_POINT('Ctrl Pts',(71.3249754182403,-6.22194821980233,-0.00360940077133092));
#34442=CARTESIAN_POINT('Ctrl Pts',(70.3214645817596,-6.22327189076832,-0.00449888440332329));
#34443=CARTESIAN_POINT('Ctrl Pts',(70.3333887657692,-6.22667288846678,-0.376563255007046));
#34444=CARTESIAN_POINT('Ctrl Pts',(70.4114834845927,-6.02678452208852,-2.81004110988959));
#34445=CARTESIAN_POINT('Ctrl Pts',(70.5557487382304,-2.81181884640884,-6.79534921779986));
#34446=CARTESIAN_POINT('Ctrl Pts',(70.7211750752654,3.00649289900833,-6.16512333542295));
#34447=CARTESIAN_POINT('Ctrl Pts',(70.8535161448936,5.77263950695759,-2.91134114312552));
#34448=CARTESIAN_POINT('Ctrl Pts',(70.9858572145215,6.74314937401964,1.2444879873417));
#34449=CARTESIAN_POINT('Ctrl Pts',(71.1512835515567,3.79854938863639,6.30172191780343));
#34450=CARTESIAN_POINT('Ctrl Pts',(71.3497951559988,-3.25302923561936,6.59577169661227));
#34451=CARTESIAN_POINT('Ctrl Pts',(71.4898554993997,-6.09535851688912,2.54913226163309));
#34452=CARTESIAN_POINT('Ctrl Pts',(71.5637453079867,-6.22646572731775,0.242997588565489));
#34453=CARTESIAN_POINT('Ctrl Pts',(71.5714645817596,-6.22570420439633,0.00188724029056342));
#34454=CARTESIAN_POINT('Origin',(28.1999754182402,0.,0.));
#34455=CARTESIAN_POINT('',(68.8249754182403,-6.21925,1.68302909948438E-12));
#34456=CARTESIAN_POINT('',(69.0714645817596,-6.21743748979354,0.000366195279979008));
#34457=CARTESIAN_POINT('',(28.1999754182402,-6.21925,5.68729293530136E-12));
#34458=CARTESIAN_POINT('Ctrl Pts',(68.8249754182403,-6.21925,2.03655253223446E-12));
#34459=CARTESIAN_POINT('Ctrl Pts',(68.883775169714,-6.2192500000006,-1.83816020915543));
#34460=CARTESIAN_POINT('Ctrl Pts',(68.9425749211877,-5.35502977485132,-3.65808141345784));
#34461=CARTESIAN_POINT('Ctrl Pts',(69.0013746726614,-3.93049712175981,-4.81977830800731));
#34462=CARTESIAN_POINT('Ctrl Pts',(69.0601744241351,-2.5059644686683,-5.98147520255679));
#34463=CARTESIAN_POINT('Ctrl Pts',(69.1189741756088,-0.549389021420466,
-6.46189408921042));
#34464=CARTESIAN_POINT('Ctrl Pts',(69.1777739270825,1.25118869866754,-6.09209302315934));
#34465=CARTESIAN_POINT('Ctrl Pts',(69.2365736785562,3.05176641875554,-5.72229195710825));
#34466=CARTESIAN_POINT('Ctrl Pts',(69.2953734300299,4.66061422075116,-4.50960958425027));
#34467=CARTESIAN_POINT('Ctrl Pts',(69.3541731815036,5.51197192302658,-2.88049233331155));
#34468=CARTESIAN_POINT('Ctrl Pts',(69.4129729329773,6.36332962530201,-1.25137508237283));
#34469=CARTESIAN_POINT('Ctrl Pts',(69.471772684451,6.44030216377297,0.761847462639996));
#34470=CARTESIAN_POINT('Ctrl Pts',(69.5305724359247,5.71582172177486,2.45121451680319));
#34471=CARTESIAN_POINT('Ctrl Pts',(69.5893721873984,4.99134127977674,4.14058157096639));
#34472=CARTESIAN_POINT('Ctrl Pts',(69.6481719388721,3.47978506146551,5.47256790209417));
#34473=CARTESIAN_POINT('Ctrl Pts',(69.7069716903458,1.71270012775744,5.97877318811139));
#34474=CARTESIAN_POINT('Ctrl Pts',(69.7657714418195,-0.0543848059506302,
6.48497847412862));
#34475=CARTESIAN_POINT('Ctrl Pts',(69.8245711932932,-2.04193092337342,6.1553571481435));
#34476=CARTESIAN_POINT('Ctrl Pts',(69.8833709447669,-3.55100669662373,5.10582236305117));
#34477=CARTESIAN_POINT('Ctrl Pts',(69.9421706962406,-5.06008246987404,4.05628757795884));
#34478=CARTESIAN_POINT('Ctrl Pts',(70.0009704477143,-6.06074051980802,2.30766719190333));
#34479=CARTESIAN_POINT('Ctrl Pts',(70.059770199188,-6.20109393743667,0.474873184741103));
#34480=CARTESIAN_POINT('Ctrl Pts',(70.0648386055388,-6.21319208641575,0.316890462829203));
#34481=CARTESIAN_POINT('Ctrl Pts',(70.0699070118895,-6.21924999999995,0.158445276458607));
#34482=CARTESIAN_POINT('Ctrl Pts',(70.0749754182403,-6.21925,1.99388538006182E-12));
#34483=CARTESIAN_POINT('Ctrl Pts',(69.0714645817596,-6.20678839560337,0.00251771313458389));
#34484=CARTESIAN_POINT('Ctrl Pts',(69.1030322235516,-6.20695393622908,-0.987187120888528));
#34485=CARTESIAN_POINT('Ctrl Pts',(69.1676851327505,-5.74899888494865,-3.01546442731683));
#34486=CARTESIAN_POINT('Ctrl Pts',(69.2654233093567,-3.62859134903107,-5.35878348065247));
#34487=CARTESIAN_POINT('Ctrl Pts',(69.3646791115776,-0.62823592000139,-6.45958714174554));
#34488=CARTESIAN_POINT('Ctrl Pts',(69.4639349137987,2.52830110610206,-5.95780469931484));
#34489=CARTESIAN_POINT('Ctrl Pts',(69.5962759834268,5.95652483419779,-3.3963489535312));
#34490=CARTESIAN_POINT('Ctrl Pts',(69.7617023204619,6.96369965258984,2.35963460035952));
#34491=CARTESIAN_POINT('Ctrl Pts',(69.9602139249039,1.78096623639146,7.13640802565527));
#34492=CARTESIAN_POINT('Ctrl Pts',(70.1468013453366,-4.61505740066332,5.46838819564559));
#34493=CARTESIAN_POINT('Ctrl Pts',(70.2672182309551,-6.20779982877329,1.68812296321986));
#34494=CARTESIAN_POINT('Ctrl Pts',(70.3214645817596,-6.22327189076832,-0.00449888440332329));
#34495=CARTESIAN_POINT('Origin',(28.1999754182402,0.,0.));
#34496=CARTESIAN_POINT('',(67.5749754182403,-6.22716903015256,-0.00354123602412358));
#34497=CARTESIAN_POINT('',(67.8214645817596,-6.21925,1.42747096013558E-12));
#34498=CARTESIAN_POINT('',(28.1999754182402,-6.21925,5.68729293530136E-12));
#34499=CARTESIAN_POINT('Ctrl Pts',(67.5749754182403,-6.22716903015256,-0.00354123602412323));
#34500=CARTESIAN_POINT('Ctrl Pts',(67.5810286846097,-6.22849064190086,-0.192188270096255));
#34501=CARTESIAN_POINT('Ctrl Pts',(67.6532524857932,-6.13655344587958,-2.44169010369456));
#34502=CARTESIAN_POINT('Ctrl Pts',(67.7916468217906,-3.40809791078333,-6.51499441152191));
#34503=CARTESIAN_POINT('Ctrl Pts',(67.9901584262328,3.63494514635811,-6.39141334988969));
#34504=CARTESIAN_POINT('Ctrl Pts',(68.1555847632678,6.70899997741019,-1.41894774382875));
#34505=CARTESIAN_POINT('Ctrl Pts',(68.2879258328959,5.84773120199377,2.77243208544916));
#34506=CARTESIAN_POINT('Ctrl Pts',(68.387181635117,3.82264019194717,5.24510836053448));
#34507=CARTESIAN_POINT('Ctrl Pts',(68.486437437338,0.848644543025793,6.4157715664878));
#34508=CARTESIAN_POINT('Ctrl Pts',(68.6187785069662,-3.40513155320004,5.95224512547316));
#34509=CARTESIAN_POINT('Ctrl Pts',(68.7316245006002,-5.99206689653167,2.91734514626186));
#34510=CARTESIAN_POINT('Ctrl Pts',(68.8113852268273,-6.22478355345344,0.432318045390996));
#34511=CARTESIAN_POINT('Ctrl Pts',(68.8249754182403,-6.22080542650654,0.00799904362253197));
#34512=CARTESIAN_POINT('Ctrl Pts',(67.8214645817596,-6.21925,1.42747096013558E-12));
#34513=CARTESIAN_POINT('Ctrl Pts',(67.8802643332333,-6.21925000000042,-1.83816020915604));
#34514=CARTESIAN_POINT('Ctrl Pts',(67.939064084707,-5.35502977485096,-3.65808141345836));
#34515=CARTESIAN_POINT('Ctrl Pts',(67.9978638361807,-3.93049712175934,-4.8197783080077));
#34516=CARTESIAN_POINT('Ctrl Pts',(68.0566635876544,-2.50596446866772,-5.98147520255704));
#34517=CARTESIAN_POINT('Ctrl Pts',(68.1154633391281,-0.549389021419833,
-6.46189408921047));
#34518=CARTESIAN_POINT('Ctrl Pts',(68.1742630906018,1.25118869866813,-6.09209302315921));
#34519=CARTESIAN_POINT('Ctrl Pts',(68.2330628420755,3.0517664187561,-5.72229195710796));
#34520=CARTESIAN_POINT('Ctrl Pts',(68.2918625935492,4.6606142207516,-4.50960958424982));
#34521=CARTESIAN_POINT('Ctrl Pts',(68.3506623450229,5.51197192302687,-2.88049233331101));
#34522=CARTESIAN_POINT('Ctrl Pts',(68.4094620964966,6.36332962530213,-1.25137508237221));
#34523=CARTESIAN_POINT('Ctrl Pts',(68.4682618479703,6.4403021637729,0.761847462640626));
#34524=CARTESIAN_POINT('Ctrl Pts',(68.527061599444,5.71582172177462,2.45121451680375));
#34525=CARTESIAN_POINT('Ctrl Pts',(68.5858613509177,4.99134127977633,4.14058157096688));
#34526=CARTESIAN_POINT('Ctrl Pts',(68.6446611023914,3.47978506146497,5.47256790209451));
#34527=CARTESIAN_POINT('Ctrl Pts',(68.7034608538651,1.71270012775685,5.97877318811156));
#34528=CARTESIAN_POINT('Ctrl Pts',(68.7622606053388,-0.054384805951265,
6.48497847412861));
#34529=CARTESIAN_POINT('Ctrl Pts',(68.8210603568125,-2.04193092337402,6.15535714814329));
#34530=CARTESIAN_POINT('Ctrl Pts',(68.8798601082862,-3.55100669662423,5.10582236305082));
#34531=CARTESIAN_POINT('Ctrl Pts',(68.9386598597599,-5.06008246987444,4.05628757795835));
#34532=CARTESIAN_POINT('Ctrl Pts',(68.9974596112336,-6.06074051980825,2.30766719190274));
#34533=CARTESIAN_POINT('Ctrl Pts',(69.0562593627073,-6.20109393743672,0.474873184740495));
#34534=CARTESIAN_POINT('Ctrl Pts',(69.0613277690581,-6.21319208641577,0.31689046282877));
#34535=CARTESIAN_POINT('Ctrl Pts',(69.0663961754089,-6.21924999999995,0.158445276458352));
#34536=CARTESIAN_POINT('Ctrl Pts',(69.0714645817596,-6.21925,1.91508895708806E-12));
#34537=CARTESIAN_POINT('Origin',(28.1999754182402,0.,0.));
#34538=CARTESIAN_POINT('',(66.3249754182403,-6.21259519566301,-0.00324245267844449));
#34539=CARTESIAN_POINT('',(66.5714645817596,-6.22114348643294,-0.0015202752725002));
#34540=CARTESIAN_POINT('',(28.1999754182402,-6.21925,5.68729293530136E-12));
#34541=CARTESIAN_POINT('Ctrl Pts',(66.3249754182403,-6.21259519566301,-0.003242452678444));
#34542=CARTESIAN_POINT('Ctrl Pts',(66.3506721423922,-6.21662143089998,-0.808861812537382));
#34543=CARTESIAN_POINT('Ctrl Pts',(66.4425394013581,-5.69514649096048,-3.68402373808155));
#34544=CARTESIAN_POINT('Ctrl Pts',(66.6005771951379,-1.34895379295012,-7.22795352199158));
#34545=CARTESIAN_POINT('Ctrl Pts',(66.7660035321732,4.20849394244699,-5.41411806724503));
#34546=CARTESIAN_POINT('Ctrl Pts',(66.8983446018011,6.25597908877345,-1.65682395344729));
#34547=CARTESIAN_POINT('Ctrl Pts',(66.9976004040223,6.30519641260689,1.53890622628911));
#34548=CARTESIAN_POINT('Ctrl Pts',(67.0968562062432,4.78925485703138,4.35262885196658));
#34549=CARTESIAN_POINT('Ctrl Pts',(67.2291972758714,1.24102420380131,6.74417930312503));
#34550=CARTESIAN_POINT('Ctrl Pts',(67.388570346537,-4.31609141344847,5.82855040460842));
#34551=CARTESIAN_POINT('Ctrl Pts',(67.5148581497957,-6.21404360605863,1.86998351846371));
#34552=CARTESIAN_POINT('Ctrl Pts',(67.5749754182403,-6.22716903015256,-0.00354123602412323));
#34553=CARTESIAN_POINT('Ctrl Pts',(66.5714645817596,-6.22114348643294,-0.00152027527249955));
#34554=CARTESIAN_POINT('Ctrl Pts',(66.5761486043024,-6.22148244516996,-0.147527676541695));
#34555=CARTESIAN_POINT('Ctrl Pts',(66.6139178942523,-6.18170946866711,-1.32459121785407));
#34556=CARTESIAN_POINT('Ctrl Pts',(66.6847724516092,-5.45227135475848,-3.4864132116906));
#34557=CARTESIAN_POINT('Ctrl Pts',(66.8171135212372,-2.35612050115225,-6.43993724590316));
#34558=CARTESIAN_POINT('Ctrl Pts',(66.9825398582723,3.48975044558929,-6.47183364038364));
#34559=CARTESIAN_POINT('Ctrl Pts',(67.1810514627144,7.33067472739079,-0.567002756194563));
#34560=CARTESIAN_POINT('Ctrl Pts',(67.3795630671566,4.45391682219975,5.85003491379102));
#34561=CARTESIAN_POINT('Ctrl Pts',(67.5780746715986,-2.50983236811194,6.91113104420389));
#34562=CARTESIAN_POINT('Ctrl Pts',(67.7253751764663,-5.95182529533825,3.00613154281414));
#34563=CARTESIAN_POINT('Ctrl Pts',(67.80650514652,-6.22533619653189,0.470469326291353));
#34564=CARTESIAN_POINT('Ctrl Pts',(67.8214645817596,-6.22287026600109,0.00237337644969353));
#34565=CARTESIAN_POINT('Origin',(28.1999754182402,0.,0.));
#34566=CARTESIAN_POINT('',(65.0749754182404,-6.21356978932969,0.00431476290370225));
#34567=CARTESIAN_POINT('',(65.3214645817596,-6.21925,1.15928100452578E-12));
#34568=CARTESIAN_POINT('',(28.1999754182402,-6.21925,5.68729293530136E-12));
#34569=CARTESIAN_POINT('Ctrl Pts',(65.0749754182404,-6.21356978932969,0.00431476290370186));
#34570=CARTESIAN_POINT('Ctrl Pts',(65.1203156001746,-6.20196410271433,-1.41654032948276));
#34571=CARTESIAN_POINT('Ctrl Pts',(65.2318263169229,-5.01369486695274,-4.92727852199253));
#34572=CARTESIAN_POINT('Ctrl Pts',(65.3764223010783,-0.280080766866481,
-6.8516896061695));
#34573=CARTESIAN_POINT('Ctrl Pts',(65.5087633707064,3.70893826617409,-5.30340616226556));
#34574=CARTESIAN_POINT('Ctrl Pts',(65.6080191729274,5.80921341909733,-2.89426564405251));
#34575=CARTESIAN_POINT('Ctrl Pts',(65.7072749751485,6.46744912735215,0.233327601020761));
#34576=CARTESIAN_POINT('Ctrl Pts',(65.8396160447766,5.30092577216001,4.35020478294281));
#34577=CARTESIAN_POINT('Ctrl Pts',(66.0050423818117,0.281730743593815,7.34735437050459));
#34578=CARTESIAN_POINT('Ctrl Pts',(66.1778572621018,-5.20975654679889,4.61816001860487));
#34579=CARTESIAN_POINT('Ctrl Pts',(66.2845016075781,-6.20625364482176,1.26565412900383));
#34580=CARTESIAN_POINT('Ctrl Pts',(66.3249754182403,-6.21259519566301,-0.003242452678444));
#34581=CARTESIAN_POINT('Ctrl Pts',(65.3214645817597,-6.21837015127254,-0.000938862326199455));
#34582=CARTESIAN_POINT('Ctrl Pts',(65.3457920620849,-6.22137299609146,-0.763310719959148));
#34583=CARTESIAN_POINT('Ctrl Pts',(65.4362900772242,-5.72097133082025,-3.5991317981514));
#34584=CARTESIAN_POINT('Ctrl Pts',(65.5929586271775,-1.51176119750446,-7.19566303681453));
#34585=CARTESIAN_POINT('Ctrl Pts',(65.7914702316198,5.23321851206271,-5.16465955355726));
#34586=CARTESIAN_POINT('Ctrl Pts',(65.9899818360617,7.17781718660405,1.59349450345578));
#34587=CARTESIAN_POINT('Ctrl Pts',(66.1884934405039,2.54376969957746,6.89871177591126));
#34588=CARTESIAN_POINT('Ctrl Pts',(66.353919777539,-3.23937625907777,6.04404973191034));
#34589=CARTESIAN_POINT('Ctrl Pts',(66.4815768246242,-5.79506225091564,2.80294095321662));
#34590=CARTESIAN_POINT('Ctrl Pts',(66.5430633368954,-6.21908823370923,0.883785445935368));
#34591=CARTESIAN_POINT('Ctrl Pts',(66.5714645817596,-6.22114348643294,-0.00152027527249955));
#34592=CARTESIAN_POINT('Origin',(28.1999754182402,0.,0.));
#34593=CARTESIAN_POINT('',(63.8249754182403,-6.22975058477463,-0.000685955996849441));
#34594=CARTESIAN_POINT('',(64.0714645817597,-6.21853427270105,0.000112577972291501));
#34595=CARTESIAN_POINT('',(28.1999754182402,-6.21925,5.68729293530136E-12));
#34596=CARTESIAN_POINT('Ctrl Pts',(63.8249754182403,-6.22975058477463,-0.000685955996849274));
#34597=CARTESIAN_POINT('Ctrl Pts',(63.889959057957,-6.22639346802808,-2.02031191703693));
#34598=CARTESIAN_POINT('Ctrl Pts',(63.9880279650808,-4.60005908095223,-5.06504725367468));
#34599=CARTESIAN_POINT('Ctrl Pts',(64.1191821396116,-0.590183859376729,
-6.44468951899971));
#34600=CARTESIAN_POINT('Ctrl Pts',(64.2184379418327,2.56899111035366,-5.9602029195333));
#34601=CARTESIAN_POINT('Ctrl Pts',(64.3176937440537,5.09045728081569,-3.99619627350351));
#34602=CARTESIAN_POINT('Ctrl Pts',(64.4500348136817,6.85670021738249,-0.098781700014005));
#34603=CARTESIAN_POINT('Ctrl Pts',(64.615461150717,4.95753380652983,5.43008720152017));
#34604=CARTESIAN_POINT('Ctrl Pts',(64.8139727551589,-1.8840609360603,7.10708088361284));
#34605=CARTESIAN_POINT('Ctrl Pts',(64.9671441776669,-5.82547528679035,3.37766727413955));
#34606=CARTESIAN_POINT('Ctrl Pts',(65.0541450653606,-6.21890171649222,0.657089227026568));
#34607=CARTESIAN_POINT('Ctrl Pts',(65.0749754182404,-6.21356978932969,0.00431476290370186));
#34608=CARTESIAN_POINT('Ctrl Pts',(64.0714645817596,-6.21925,1.20194898390342E-12));
#34609=CARTESIAN_POINT('Ctrl Pts',(64.1302643332333,-6.21925000000036,-1.83816020915627));
#34610=CARTESIAN_POINT('Ctrl Pts',(64.189064084707,-5.35502977485083,-3.65808141345855));
#34611=CARTESIAN_POINT('Ctrl Pts',(64.2478638361807,-3.93049712175916,-4.81977830800784));
#34612=CARTESIAN_POINT('Ctrl Pts',(64.3066635876544,-2.5059644686675,-5.98147520255713));
#34613=CARTESIAN_POINT('Ctrl Pts',(64.3654633391281,-0.549389021419599,
-6.46189408921049));
#34614=CARTESIAN_POINT('Ctrl Pts',(64.4242630906018,1.25118869866836,-6.09209302315917));
#34615=CARTESIAN_POINT('Ctrl Pts',(64.4830628420755,3.05176641875631,-5.72229195710785));
#34616=CARTESIAN_POINT('Ctrl Pts',(64.5418625935492,4.66061422075176,-4.50960958424965));
#34617=CARTESIAN_POINT('Ctrl Pts',(64.6006623450229,5.51197192302697,-2.88049233331081));
#34618=CARTESIAN_POINT('Ctrl Pts',(64.6594620964966,6.36332962530218,-1.25137508237198));
#34619=CARTESIAN_POINT('Ctrl Pts',(64.7182618479703,6.44030216377287,0.76184746264086));
#34620=CARTESIAN_POINT('Ctrl Pts',(64.777061599444,5.71582172177453,2.45121451680396));
#34621=CARTESIAN_POINT('Ctrl Pts',(64.8358613509177,4.99134127977619,4.14058157096706));
#34622=CARTESIAN_POINT('Ctrl Pts',(64.8946611023914,3.47978506146477,5.47256790209463));
#34623=CARTESIAN_POINT('Ctrl Pts',(64.9534608538651,1.71270012775664,5.97877318811162));
#34624=CARTESIAN_POINT('Ctrl Pts',(65.0122606053388,-0.0543848059515001,
6.48497847412861));
#34625=CARTESIAN_POINT('Ctrl Pts',(65.0710603568125,-2.04193092337424,6.15535714814322));
#34626=CARTESIAN_POINT('Ctrl Pts',(65.1298601082862,-3.55100669662442,5.10582236305069));
#34627=CARTESIAN_POINT('Ctrl Pts',(65.1886598597599,-5.06008246987459,4.05628757795816));
#34628=CARTESIAN_POINT('Ctrl Pts',(65.2474596112336,-6.06074051980833,2.30766719190252));
#34629=CARTESIAN_POINT('Ctrl Pts',(65.3062593627073,-6.20109393743674,0.47487318474027));
#34630=CARTESIAN_POINT('Ctrl Pts',(65.3113277690581,-6.21319208641579,0.316890462828369));
#34631=CARTESIAN_POINT('Ctrl Pts',(65.3163961754089,-6.21924999999997,0.158445276457773));
#34632=CARTESIAN_POINT('Ctrl Pts',(65.3214645817596,-6.21925,1.15928183173078E-12));
#34633=CARTESIAN_POINT('Origin',(28.1999754182402,0.,0.));
#34634=CARTESIAN_POINT('',(62.5749754182403,-6.21856955346695,-0.000259107838776135));
#34635=CARTESIAN_POINT('',(62.8214645817596,-6.22934305414637,0.00327033652799832));
#34636=CARTESIAN_POINT('',(28.1999754182402,-6.21925,5.68729293530136E-12));
#34637=CARTESIAN_POINT('Ctrl Pts',(62.5749754182404,-6.21260916379183,-0.00252876991957987));
#34638=CARTESIAN_POINT('Ctrl Pts',(62.5934319809255,-6.21745248917224,-0.580222709882177));
#34639=CARTESIAN_POINT('Ctrl Pts',(62.6449738110176,-6.01215797913732,-2.1915756033502));
#34640=CARTESIAN_POINT('Ctrl Pts',(62.7296009085167,-4.61050649279502,-4.54153827068194));
#34641=CARTESIAN_POINT('Ctrl Pts',(62.828856710738,-1.88480796006642,-6.2105742987874));
#34642=CARTESIAN_POINT('Ctrl Pts',(62.9281125129588,1.30876242173983,-6.33793979993621));
#34643=CARTESIAN_POINT('Ctrl Pts',(63.0604535825871,5.17340855136809,-4.50110427072531));
#34644=CARTESIAN_POINT('Ctrl Pts',(63.225879919622,7.29142614877463,0.947677780663159));
#34645=CARTESIAN_POINT('Ctrl Pts',(63.4243915240643,3.14821152092017,6.64447503694298));
#34646=CARTESIAN_POINT('Ctrl Pts',(63.6229031285063,-3.87306471768808,6.24977231502176));
#34647=CARTESIAN_POINT('Ctrl Pts',(63.7564310932317,-6.21295322572177,2.12964199441194));
#34648=CARTESIAN_POINT('Ctrl Pts',(63.823788523143,-6.22981190090628,0.0362015461805261));
#34649=CARTESIAN_POINT('Ctrl Pts',(63.8249754182403,-6.22975058477463,-0.000685955996849274));
#34650=CARTESIAN_POINT('Ctrl Pts',(62.8214645817596,-6.22934305414637,0.00327033652799856));
#34651=CARTESIAN_POINT('Ctrl Pts',(62.8850789776498,-6.22299644639126,-1.97466634164587));
#34652=CARTESIAN_POINT('Ctrl Pts',(63.014863908354,-4.12949038798452,-6.0315003317796));
#34653=CARTESIAN_POINT('Ctrl Pts',(63.2108193738721,2.7683587964008,-6.81149571470196));
#34654=CARTESIAN_POINT('Ctrl Pts',(63.4093309783144,7.22635244835865,-1.35750460444815));
#34655=CARTESIAN_POINT('Ctrl Pts',(63.5747573153493,5.41909355797858,4.20208528057022));
#34656=CARTESIAN_POINT('Ctrl Pts',(63.7070983849776,1.66422455917251,6.25401443880813));
#34657=CARTESIAN_POINT('Ctrl Pts',(63.8063541871984,-1.53144515668549,6.30701275558833));
#34658=CARTESIAN_POINT('Ctrl Pts',(63.9056099894197,-4.34695939124221,4.79440132186115));
#34659=CARTESIAN_POINT('Ctrl Pts',(63.99398012094,-5.94670819129815,2.42697794624009));
#34660=CARTESIAN_POINT('Ctrl Pts',(64.0492649850533,-6.21443109280533,0.696924413737985));
#34661=CARTESIAN_POINT('Ctrl Pts',(64.0714645817596,-6.20983994024725,0.00148012439544501));
#34662=CARTESIAN_POINT('Origin',(28.1999754182402,0.,0.));
#34663=CARTESIAN_POINT('',(61.3249754182403,-6.21925,8.78461714269987E-13));
#34664=CARTESIAN_POINT('',(61.5714645817597,-6.21695893348969,-0.00516800745213986));
#34665=CARTESIAN_POINT('',(28.1999754182402,-6.21925,5.68729293530136E-12));
#34666=CARTESIAN_POINT('Ctrl Pts',(61.3249754182403,-6.21925,8.78461714269987E-13));
#34667=CARTESIAN_POINT('Ctrl Pts',(61.383775169714,-6.21925000000026,-1.83816020915659));
#34668=CARTESIAN_POINT('Ctrl Pts',(61.4425749211877,-5.35502977485064,-3.65808141345883));
#34669=CARTESIAN_POINT('Ctrl Pts',(61.5013746726614,-3.93049712175891,-4.81977830800805));
#34670=CARTESIAN_POINT('Ctrl Pts',(61.5601744241351,-2.50596446866719,-5.98147520255726));
#34671=CARTESIAN_POINT('Ctrl Pts',(61.6189741756088,-0.549389021419263,
-6.46189408921052));
#34672=CARTESIAN_POINT('Ctrl Pts',(61.6777739270825,1.25118869866867,-6.0920930231591));
#34673=CARTESIAN_POINT('Ctrl Pts',(61.7365736785562,3.05176641875661,-5.72229195710769));
#34674=CARTESIAN_POINT('Ctrl Pts',(61.7953734300299,4.660614220752,-4.5096095842494));
#34675=CARTESIAN_POINT('Ctrl Pts',(61.8541731815036,5.51197192302712,-2.88049233331053));
#34676=CARTESIAN_POINT('Ctrl Pts',(61.9129729329773,6.36332962530224,-1.25137508237165));
#34677=CARTESIAN_POINT('Ctrl Pts',(61.971772684451,6.44030216377283,0.761847462641195));
#34678=CARTESIAN_POINT('Ctrl Pts',(62.0305724359247,5.7158217217744,2.45121451680426));
#34679=CARTESIAN_POINT('Ctrl Pts',(62.0893721873984,4.99134127977597,4.14058157096732));
#34680=CARTESIAN_POINT('Ctrl Pts',(62.1481719388721,3.47978506146449,5.47256790209481));
#34681=CARTESIAN_POINT('Ctrl Pts',(62.2069716903458,1.71270012775632,5.97877318811171));
#34682=CARTESIAN_POINT('Ctrl Pts',(62.2657714418195,-0.054384805951837,
6.48497847412861));
#34683=CARTESIAN_POINT('Ctrl Pts',(62.3245711932932,-2.04193092337456,6.15535714814311));
#34684=CARTESIAN_POINT('Ctrl Pts',(62.3833709447669,-3.55100669662468,5.10582236305051));
#34685=CARTESIAN_POINT('Ctrl Pts',(62.4421706962406,-5.0600824698748,4.0562875779579));
#34686=CARTESIAN_POINT('Ctrl Pts',(62.5009704477143,-6.06074051980845,2.3076671919022));
#34687=CARTESIAN_POINT('Ctrl Pts',(62.559770199188,-6.20109393743676,0.474873184739948));
#34688=CARTESIAN_POINT('Ctrl Pts',(62.5648386055388,-6.2131920864158,0.316890462828163));
#34689=CARTESIAN_POINT('Ctrl Pts',(62.5699070118896,-6.21924999999997,0.158445276457685));
#34690=CARTESIAN_POINT('Ctrl Pts',(62.5749754182403,-6.21925,1.18931799484743E-12));
#34691=CARTESIAN_POINT('Ctrl Pts',(61.5714645817597,-6.21695893348969,-0.00516800745214034));
#34692=CARTESIAN_POINT('Ctrl Pts',(61.5885519006182,-6.22200109994744,-0.53992295050933));
#34693=CARTESIAN_POINT('Ctrl Pts',(61.6718097542908,-5.91572340500266,-3.14007559790216));
#34694=CARTESIAN_POINT('Ctrl Pts',(61.8212381427774,-2.28199696173699,-6.98947595772644));
#34695=CARTESIAN_POINT('Ctrl Pts',(62.0197497472196,4.64330776244168,-5.70111230219558));
#34696=CARTESIAN_POINT('Ctrl Pts',(62.1851760842546,6.85135343285645,-0.288187149949455));
#34697=CARTESIAN_POINT('Ctrl Pts',(62.3175171538827,5.30779068198273,3.70266094321786));
#34698=CARTESIAN_POINT('Ctrl Pts',(62.4167729561038,2.90113679133094,5.80578500162336));
#34699=CARTESIAN_POINT('Ctrl Pts',(62.5160287583248,-0.225675472877136,
6.46772066226701));
#34700=CARTESIAN_POINT('Ctrl Pts',(62.6483698279529,-4.34392994578106,5.30606900835795));
#34701=CARTESIAN_POINT('Ctrl Pts',(62.7501817690978,-6.19218467788144,2.21918086720454));
#34702=CARTESIAN_POINT('Ctrl Pts',(62.8189084428357,-6.22959807206944,0.0827473300813655));
#34703=CARTESIAN_POINT('Ctrl Pts',(62.8214645817596,-6.22934305414637,0.00327033652799856));
#34704=CARTESIAN_POINT('Origin',(28.1999754182402,0.,0.));
#34705=CARTESIAN_POINT('',(60.0749754182404,-6.21925,7.44365506732958E-13));
#34706=CARTESIAN_POINT('',(60.3214645817597,-6.21111205730243,0.00169677517069255));
#34707=CARTESIAN_POINT('',(28.1999754182402,-6.21925,5.68729293530136E-12));
#34708=CARTESIAN_POINT('Ctrl Pts',(60.0749754182404,-6.22004574063539,0.00250981053279774));
#34709=CARTESIAN_POINT('Ctrl Pts',(60.0996336290834,-6.21761940426262,-0.766580500658636));
#34710=CARTESIAN_POINT('Ctrl Pts',(60.1573771073334,-5.87450282726596,-2.57066518997162));
#34711=CARTESIAN_POINT('Ctrl Pts',(60.2812911203974,-3.57518444437901,-5.85167940714288));
#34712=CARTESIAN_POINT('Ctrl Pts',(60.4467174574326,2.15053713527687,-7.03122880361549));
#34713=CARTESIAN_POINT('Ctrl Pts',(60.6452290618746,7.07649152718233,-1.99588375481379));
#34714=CARTESIAN_POINT('Ctrl Pts',(60.8437406663167,5.5162418506764,4.86120974057477));
#34715=CARTESIAN_POINT('Ctrl Pts',(61.0422522707589,-1.1034200191743,7.26948778940321));
#34716=CARTESIAN_POINT('Ctrl Pts',(61.2026638547334,-5.61407165712723,3.83602481861383));
#34717=CARTESIAN_POINT('Ctrl Pts',(61.2969049038939,-6.21974059825275,0.879711363588332));
#34718=CARTESIAN_POINT('Ctrl Pts',(61.3249754182403,-6.21712757775053,-3.09561547350186E-5));
#34719=CARTESIAN_POINT('Ctrl Pts',(60.3214645817597,-6.21111205730243,0.0016967751706929));
#34720=CARTESIAN_POINT('Ctrl Pts',(60.3581953584006,-6.20814873088829,-1.15054126823442));
#34721=CARTESIAN_POINT('Ctrl Pts',(60.4610966698556,-5.34657007883321,-4.38263206448972));
#34722=CARTESIAN_POINT('Ctrl Pts',(60.6301685161248,-0.133209051532416,
-7.35154703498433));
#34723=CARTESIAN_POINT('Ctrl Pts',(60.7955948531599,5.0470729870606,-4.64232161300714));
#34724=CARTESIAN_POINT('Ctrl Pts',(60.9279359227879,6.44398673196168,-0.597808483107745));
#34725=CARTESIAN_POINT('Ctrl Pts',(61.027191725009,5.96323825064499,2.56193749594574));
#34726=CARTESIAN_POINT('Ctrl Pts',(61.12644752723,4.00221625291053,5.08572561677413));
#34727=CARTESIAN_POINT('Ctrl Pts',(61.2587885968582,0.106894138300333,6.85657854461737));
#34728=CARTESIAN_POINT('Ctrl Pts',(61.4071276150346,-4.8528948701387,5.15944898606185));
#34729=CARTESIAN_POINT('Ctrl Pts',(61.5223813658041,-6.20247534205104,1.53091220329418));
#34730=CARTESIAN_POINT('Ctrl Pts',(61.5714645817597,-6.21695893348969,-0.00516800745214034));
#34731=CARTESIAN_POINT('Origin',(28.1999754182402,0.,0.));
#34732=CARTESIAN_POINT('',(58.8249754182404,-6.21925,6.10272585865188E-13));
#34733=CARTESIAN_POINT('',(59.0714645817597,-6.22408309271093,0.00477558807787742));
#34734=CARTESIAN_POINT('',(28.1999754182402,-6.21925,5.68729293530136E-12));
#34735=CARTESIAN_POINT('Ctrl Pts',(58.8249754182404,-6.21925,6.10272585865188E-13));
#34736=CARTESIAN_POINT('Ctrl Pts',(58.8837751697141,-6.21925000000018,-1.83816020915686));
#34737=CARTESIAN_POINT('Ctrl Pts',(58.9425749211877,-5.35502977485048,-3.65808141345906));
#34738=CARTESIAN_POINT('Ctrl Pts',(59.0013746726614,-3.93049712175871,-4.81977830800821));
#34739=CARTESIAN_POINT('Ctrl Pts',(59.0601744241351,-2.50596446866693,-5.98147520255737));
#34740=CARTESIAN_POINT('Ctrl Pts',(59.1189741756088,-0.549389021418984,
-6.46189408921054));
#34741=CARTESIAN_POINT('Ctrl Pts',(59.1777739270825,1.25118869866893,-6.09209302315905));
#34742=CARTESIAN_POINT('Ctrl Pts',(59.2365736785562,3.05176641875685,-5.72229195710755));
#34743=CARTESIAN_POINT('Ctrl Pts',(59.2953734300299,4.66061422075219,-4.5096095842492));
#34744=CARTESIAN_POINT('Ctrl Pts',(59.3541731815036,5.51197192302724,-2.88049233331029));
#34745=CARTESIAN_POINT('Ctrl Pts',(59.4129729329773,6.3633296253023,-1.25137508237137));
#34746=CARTESIAN_POINT('Ctrl Pts',(59.471772684451,6.4403021637728,0.761847462641473));
#34747=CARTESIAN_POINT('Ctrl Pts',(59.5305724359247,5.71582172177429,2.45121451680451));
#34748=CARTESIAN_POINT('Ctrl Pts',(59.5893721873984,4.99134127977579,4.14058157096754));
#34749=CARTESIAN_POINT('Ctrl Pts',(59.6481719388721,3.47978506146425,5.47256790209496));
#34750=CARTESIAN_POINT('Ctrl Pts',(59.7069716903458,1.71270012775607,5.97877318811178));
#34751=CARTESIAN_POINT('Ctrl Pts',(59.7657714418195,-0.0543848059521168,
6.48497847412861));
#34752=CARTESIAN_POINT('Ctrl Pts',(59.8245711932932,-2.04193092337483,6.15535714814303));
#34753=CARTESIAN_POINT('Ctrl Pts',(59.8833709447669,-3.5510066966249,5.10582236305035));
#34754=CARTESIAN_POINT('Ctrl Pts',(59.9421706962406,-5.06008246987498,4.05628757795768));
#34755=CARTESIAN_POINT('Ctrl Pts',(60.0009704477143,-6.06074051980855,2.30766719190194));
#34756=CARTESIAN_POINT('Ctrl Pts',(60.059770199188,-6.20109393743678,0.47487318473968));
#34757=CARTESIAN_POINT('Ctrl Pts',(60.0648386055388,-6.21319208641582,0.316890462827836));
#34758=CARTESIAN_POINT('Ctrl Pts',(60.0699070118896,-6.21924999999998,0.158445276457299));
#34759=CARTESIAN_POINT('Ctrl Pts',(60.0749754182404,-6.21925,7.44367150067587E-13));
#34760=CARTESIAN_POINT('Ctrl Pts',(59.0714645817597,-6.22408309271093,0.00477558807787732));
#34761=CARTESIAN_POINT('Ctrl Pts',(59.1278388161831,-6.20819293747344,-1.7543657142207));
#34762=CARTESIAN_POINT('Ctrl Pts',(59.2503835854205,-4.50893443442348,-5.60461480076411));
#34763=CARTESIAN_POINT('Ctrl Pts',(59.406013622065,0.858584021869272,-6.80344979938125));
#34764=CARTESIAN_POINT('Ctrl Pts',(59.5383546916932,4.53608016947545,-4.61587658850033));
#34765=CARTESIAN_POINT('Ctrl Pts',(59.6376104939142,6.20833994062302,-1.89215468415061));
#34766=CARTESIAN_POINT('Ctrl Pts',(59.7368662961353,6.33948382661728,1.30126276986307));
#34767=CARTESIAN_POINT('Ctrl Pts',(59.8692073657633,4.50722204056254,5.16807944718129));
#34768=CARTESIAN_POINT('Ctrl Pts',(60.0346337027984,-0.939050263787701,
7.2925422906609));
#34769=CARTESIAN_POINT('Ctrl Pts',(60.1964145305996,-5.58575588337288,3.92144569883786));
#34770=CARTESIAN_POINT('Ctrl Pts',(60.2920248235866,-6.21348716670654,0.925216843563736));
#34771=CARTESIAN_POINT('Ctrl Pts',(60.3214645817597,-6.21111205730243,0.0016967751706929));
#34772=CARTESIAN_POINT('Origin',(28.1999754182402,0.,0.));
#34773=CARTESIAN_POINT('',(57.5749754182404,-6.21812662533432,-0.000394576859186467));
#34774=CARTESIAN_POINT('',(57.8214645817597,-6.22441924678459,-0.00707629521854547));
#34775=CARTESIAN_POINT('',(28.1999754182402,-6.21925,5.68729293530136E-12));
#34776=CARTESIAN_POINT('Ctrl Pts',(57.5749754182404,-6.20740910248718,-0.00415902574651419));
#34777=CARTESIAN_POINT('Ctrl Pts',(57.6058352772412,-6.20996092781725,-0.971356541319267));
#34778=CARTESIAN_POINT('Ctrl Pts',(57.7028656710561,-5.544781642729,-4.00770145453599));
#34779=CARTESIAN_POINT('Ctrl Pts',(57.8660665996852,-0.787641354648353,
-7.31026028219656));
#34780=CARTESIAN_POINT('Ctrl Pts',(58.0645782041271,5.71316809273326,-4.6281740072287));
#34781=CARTESIAN_POINT('Ctrl Pts',(58.2630898085693,6.98362156225626,2.30043872645768));
#34782=CARTESIAN_POINT('Ctrl Pts',(58.4285161456044,2.71657121158352,6.29637487350503));
#34783=CARTESIAN_POINT('Ctrl Pts',(58.5608572152325,-1.56235319508776,6.28023825009631));
#34784=CARTESIAN_POINT('Ctrl Pts',(58.6601130174535,-4.38640864661985,4.78363390655549));
#34785=CARTESIAN_POINT('Ctrl Pts',(58.7481524184562,-5.92552534696238,2.40288525575302));
#34786=CARTESIAN_POINT('Ctrl Pts',(58.8031065520518,-6.22151982471558,0.68137012316749));
#34787=CARTESIAN_POINT('Ctrl Pts',(58.8249754182404,-6.22479259784097,-0.00228417281318501));
#34788=CARTESIAN_POINT('Ctrl Pts',(57.8214645817597,-6.22441924678459,-0.00707629521854609));
#34789=CARTESIAN_POINT('Ctrl Pts',(57.8313117391515,-6.22705934464582,-0.314015706705484));
#34790=CARTESIAN_POINT('Ctrl Pts',(57.9073294313574,-6.06711261063953,-2.68001408884272));
#34791=CARTESIAN_POINT('Ctrl Pts',(58.0164323909703,-3.73549514279114,-5.75066706856635));
#34792=CARTESIAN_POINT('Ctrl Pts',(58.1487734605983,0.485355182835179,-6.45343089609464));
#34793=CARTESIAN_POINT('Ctrl Pts',(58.2480292628194,3.52065721958024,-5.45240377350268));
#34794=CARTESIAN_POINT('Ctrl Pts',(58.3472850650405,5.68201536485552,-3.09790919455678));
#34795=CARTESIAN_POINT('Ctrl Pts',(58.4796261346685,6.77836393432703,1.03820906811895));
#34796=CARTESIAN_POINT('Ctrl Pts',(58.6450524717037,3.98971935895797,6.17617421190118));
#34797=CARTESIAN_POINT('Ctrl Pts',(58.8435640761457,-3.03513575029629,6.69688250414221));
#34798=CARTESIAN_POINT('Ctrl Pts',(58.9857014461645,-6.06892784062922,2.67815832873045));
#34799=CARTESIAN_POINT('Ctrl Pts',(59.0616682813691,-6.22684436717526,0.310466242737264));
#34800=CARTESIAN_POINT('Ctrl Pts',(59.0714645817597,-6.22408309271093,0.00477558807787732));
#34801=CARTESIAN_POINT('Origin',(28.1999754182402,0.,0.));
#34802=CARTESIAN_POINT('',(56.3249754182404,-6.21925,3.42083457460389E-13));
#34803=CARTESIAN_POINT('',(56.5714645817597,-6.21881043026408,5.47690459495173E-5));
#34804=CARTESIAN_POINT('',(28.1999754182402,-6.21925,5.68729293530136E-12));
#34805=CARTESIAN_POINT('Ctrl Pts',(56.3249754182404,-6.21925,3.42083457460389E-13));
#34806=CARTESIAN_POINT('Ctrl Pts',(56.3837751697141,-6.2192500000001,-1.83816020915713));
#34807=CARTESIAN_POINT('Ctrl Pts',(56.4425749211878,-5.35502977485032,-3.65808141345929));
#34808=CARTESIAN_POINT('Ctrl Pts',(56.5013746726615,-3.9304971217585,-4.81977830800838));
#34809=CARTESIAN_POINT('Ctrl Pts',(56.5601744241352,-2.50596446866667,-5.98147520255747));
#34810=CARTESIAN_POINT('Ctrl Pts',(56.6189741756089,-0.549389021418706,
-6.46189408921057));
#34811=CARTESIAN_POINT('Ctrl Pts',(56.6777739270826,1.2511886986692,-6.09209302315899));
#34812=CARTESIAN_POINT('Ctrl Pts',(56.7365736785563,3.0517664187571,-5.72229195710742));
#34813=CARTESIAN_POINT('Ctrl Pts',(56.79537343003,4.66061422075239,-4.509609584249));
#34814=CARTESIAN_POINT('Ctrl Pts',(56.8541731815037,5.51197192302737,-2.88049233331005));
#34815=CARTESIAN_POINT('Ctrl Pts',(56.9129729329774,6.36332962530235,-1.2513750823711));
#34816=CARTESIAN_POINT('Ctrl Pts',(56.9717726844511,6.44030216377277,0.76184746264175));
#34817=CARTESIAN_POINT('Ctrl Pts',(57.0305724359248,5.71582172177419,2.45121451680475));
#34818=CARTESIAN_POINT('Ctrl Pts',(57.0893721873985,4.99134127977561,4.14058157096775));
#34819=CARTESIAN_POINT('Ctrl Pts',(57.1481719388721,3.47978506146401,5.47256790209511));
#34820=CARTESIAN_POINT('Ctrl Pts',(57.2069716903459,1.71270012775581,5.97877318811186));
#34821=CARTESIAN_POINT('Ctrl Pts',(57.2657714418196,-0.0543848059523969,
6.4849784741286));
#34822=CARTESIAN_POINT('Ctrl Pts',(57.3245711932932,-2.04193092337509,6.15535714814294));
#34823=CARTESIAN_POINT('Ctrl Pts',(57.3833709447669,-3.55100669662512,5.1058223630502));
#34824=CARTESIAN_POINT('Ctrl Pts',(57.4421706962406,-5.06008246987515,4.05628757795746));
#34825=CARTESIAN_POINT('Ctrl Pts',(57.5009704477143,-6.06074051980865,2.30766719190168));
#34826=CARTESIAN_POINT('Ctrl Pts',(57.559770199188,-6.2010939374368,0.474873184739413));
#34827=CARTESIAN_POINT('Ctrl Pts',(57.5648386055388,-6.21319208641583,0.316890462827627));
#34828=CARTESIAN_POINT('Ctrl Pts',(57.5699070118896,-6.21924999999998,0.158445276457149));
#34829=CARTESIAN_POINT('Ctrl Pts',(57.5749754182404,-6.21925,6.52939738037828E-13));
#34830=CARTESIAN_POINT('Ctrl Pts',(56.5714645817596,-6.20690476956114,0.00153817820988812));
#34831=CARTESIAN_POINT('Ctrl Pts',(56.6009551969339,-6.20849907782506,-0.923070451156225));
#34832=CARTESIAN_POINT('Ctrl Pts',(56.6635310795152,-5.79712602908302,-2.88516041489965));
#34833=CARTESIAN_POINT('Ctrl Pts',(56.7591922295036,-3.7946488264813,-5.24242122190289));
#34834=CARTESIAN_POINT('Ctrl Pts',(56.8584480317246,-0.830163910262025,
-6.43696838963711));
#34835=CARTESIAN_POINT('Ctrl Pts',(56.9577038339457,2.34039522251466,-6.03364650825719));
#34836=CARTESIAN_POINT('Ctrl Pts',(57.0900449035737,5.84744533060766,-3.58210535870519));
#34837=CARTESIAN_POINT('Ctrl Pts',(57.2554712406089,7.03376829111499,2.14221662907907));
#34838=CARTESIAN_POINT('Ctrl Pts',(57.4539828450509,2.00425491144597,7.07412514357485));
#34839=CARTESIAN_POINT('Ctrl Pts',(57.6426472921013,-4.51444270971877,5.59898313484983));
#34840=CARTESIAN_POINT('Ctrl Pts',(57.7651412043375,-6.20931852051886,1.74854348732337));
#34841=CARTESIAN_POINT('Ctrl Pts',(57.8214645817597,-6.22441924678459,-0.00707629521854609));
#34842=CARTESIAN_POINT('Origin',(28.1999754182402,0.,0.));
#34843=CARTESIAN_POINT('',(55.0749754182404,-6.22846436199193,-0.00261261932939155));
#34844=CARTESIAN_POINT('',(55.3214645817597,-6.21925,8.65253181115805E-14));
#34845=CARTESIAN_POINT('',(28.1999754182402,-6.21925,5.68729293530136E-12));
#34846=CARTESIAN_POINT('Ctrl Pts',(55.0749754182404,-6.22846436199193,-0.00261261932939051));
#34847=CARTESIAN_POINT('Ctrl Pts',(55.0789516579921,-6.22911653311281,-0.126462013579355));
#34848=CARTESIAN_POINT('Ctrl Pts',(55.1490984325579,-6.17099271056379,-2.31070670859694));
#34849=CARTESIAN_POINT('Ctrl Pts',(55.2854157419376,-3.61044798336259,-6.4050721819856));
#34850=CARTESIAN_POINT('Ctrl Pts',(55.4839273463797,3.43301069967906,-6.50210934965618));
#34851=CARTESIAN_POINT('Ctrl Pts',(55.6493536834148,6.66127426453652,-1.62834912347856));
#34852=CARTESIAN_POINT('Ctrl Pts',(55.7816947530429,5.93168364981801,2.58794688172988));
#34853=CARTESIAN_POINT('Ctrl Pts',(55.880950555264,3.98501993711935,5.12282639446718));
#34854=CARTESIAN_POINT('Ctrl Pts',(55.980206357485,1.04914210494851,6.38605048741379));
#34855=CARTESIAN_POINT('Ctrl Pts',(56.1125474271131,-3.21706142470918,6.05595669444211));
#34856=CARTESIAN_POINT('Ctrl Pts',(56.2274704473648,-5.94711148533298,3.04922222251432));
#34857=CARTESIAN_POINT('Ctrl Pts',(56.3093082002096,-6.22328552490555,0.497795406618084));
#34858=CARTESIAN_POINT('Ctrl Pts',(56.3249754182404,-6.21872822153172,0.00816645970560553));
#34859=CARTESIAN_POINT('Ctrl Pts',(55.3214645817597,-6.21925,8.65253181115805E-14));
#34860=CARTESIAN_POINT('Ctrl Pts',(55.3802643332334,-6.21925000000003,-1.8381602091575));
#34861=CARTESIAN_POINT('Ctrl Pts',(55.4390640847071,-5.35502977485006,-3.65808141345974));
#34862=CARTESIAN_POINT('Ctrl Pts',(55.4978638361808,-3.93049712175803,-4.81977830800877));
#34863=CARTESIAN_POINT('Ctrl Pts',(55.5566635876545,-2.505964468666,-5.9814752025578));
#34864=CARTESIAN_POINT('Ctrl Pts',(55.6154633391282,-0.549389021417821,
-6.46189408921067));
#34865=CARTESIAN_POINT('Ctrl Pts',(55.6742630906019,1.25118869867014,-6.0920930231588));
#34866=CARTESIAN_POINT('Ctrl Pts',(55.7330628420756,3.0517664187581,-5.72229195710693));
#34867=CARTESIAN_POINT('Ctrl Pts',(55.7918625935493,4.66061422075329,-4.50960958424812));
#34868=CARTESIAN_POINT('Ctrl Pts',(55.850662345023,5.51197192302798,-2.88049233330888));
#34869=CARTESIAN_POINT('Ctrl Pts',(55.9094620964967,6.36332962530267,-1.25137508236965));
#34870=CARTESIAN_POINT('Ctrl Pts',(55.9682618479704,6.44030216377261,0.761847462643371));
#34871=CARTESIAN_POINT('Ctrl Pts',(56.0270615994441,5.71582172177353,2.45121451680629));
#34872=CARTESIAN_POINT('Ctrl Pts',(56.0858613509178,4.99134127977445,4.1405815709692));
#34873=CARTESIAN_POINT('Ctrl Pts',(56.1446611023915,3.47978506146235,5.47256790209621));
#34874=CARTESIAN_POINT('Ctrl Pts',(56.2034608538652,1.71270012775386,5.97877318811242));
#34875=CARTESIAN_POINT('Ctrl Pts',(56.2622606053389,-0.0543848059546201,
6.48497847412862));
#34876=CARTESIAN_POINT('Ctrl Pts',(56.3210603568126,-2.04193092337735,6.15535714814223));
#34877=CARTESIAN_POINT('Ctrl Pts',(56.3798601082863,-3.55100669662707,5.10582236304884));
#34878=CARTESIAN_POINT('Ctrl Pts',(56.43865985976,-5.0600824698768,4.05628757795546));
#34879=CARTESIAN_POINT('Ctrl Pts',(56.4974596112337,-6.06074051980966,2.30766719189914));
#34880=CARTESIAN_POINT('Ctrl Pts',(56.5562593627074,-6.20109393743701,0.474873184736691));
#34881=CARTESIAN_POINT('Ctrl Pts',(56.5613277690582,-6.21319208641591,0.316890462825663));
#34882=CARTESIAN_POINT('Ctrl Pts',(56.5663961754089,-6.21925,0.15844527645595));
#34883=CARTESIAN_POINT('Ctrl Pts',(56.5714645817597,-6.21925,2.20619882313981E-13));
#34884=CARTESIAN_POINT('Origin',(28.1999754182402,0.,0.));
#34885=CARTESIAN_POINT('',(53.8249754182404,-6.2138011505806,-0.0039455443126054));
#34886=CARTESIAN_POINT('',(54.0714645817597,-6.2215550358857,-0.000870493656277005));
#34887=CARTESIAN_POINT('',(28.1999754182402,-6.21925,5.68729293530136E-12));
#34888=CARTESIAN_POINT('Ctrl Pts',(53.8249754182404,-6.2138011505806,-0.00394554431260567));
#34889=CARTESIAN_POINT('Ctrl Pts',(53.8485951157745,-6.21836794550842,-0.744086608287605));
#34890=CARTESIAN_POINT('Ctrl Pts',(53.9383853481227,-5.75208740079896,-3.55221171660335));
#34891=CARTESIAN_POINT('Ctrl Pts',(54.094346115285,-1.57464063360658,-7.18216508679608));
#34892=CARTESIAN_POINT('Ctrl Pts',(54.2597724523201,4.03688294466771,-5.54325462037972));
#34893=CARTESIAN_POINT('Ctrl Pts',(54.3921135219481,6.20102619469151,-1.85192173617664));
#34894=CARTESIAN_POINT('Ctrl Pts',(54.4913693241692,6.35029591436066,1.34069980500598));
#34895=CARTESIAN_POINT('Ctrl Pts',(54.5906251263902,4.92321156794364,4.2005151876216));
#34896=CARTESIAN_POINT('Ctrl Pts',(54.7229661960184,1.45161424482283,6.70200804084397));
#34897=CARTESIAN_POINT('Ctrl Pts',(54.8844162933016,-4.20421056897935,5.95119407725046));
#34898=CARTESIAN_POINT('Ctrl Pts',(55.0127811231781,-6.21826343708397,1.93457584269618));
#34899=CARTESIAN_POINT('Ctrl Pts',(55.0749754182404,-6.22846436199193,-0.00261261932939051));
#34900=CARTESIAN_POINT('Ctrl Pts',(54.0714645817597,-6.2215550358857,-0.000870493656276667));
#34901=CARTESIAN_POINT('Ctrl Pts',(54.0740715776848,-6.22167540488534,-0.0821163961368401));
#34902=CARTESIAN_POINT('Ctrl Pts',(54.109763841017,-6.20077041387944,-1.1943670518483));
#34903=CARTESIAN_POINT('Ctrl Pts',(54.1785413717561,-5.55877673210131,-3.31396156085478));
#34904=CARTESIAN_POINT('Ctrl Pts',(54.3108824413843,-2.55663608376213,-6.36299517762788));
#34905=CARTESIAN_POINT('Ctrl Pts',(54.4763087784192,3.28536884845591,-6.57794344674629));
#34906=CARTESIAN_POINT('Ctrl Pts',(54.6748203828615,7.30932326741656,-0.796289940546589));
#34907=CARTESIAN_POINT('Ctrl Pts',(54.8733319873035,4.63493030483003,5.70768826815035));
#34908=CARTESIAN_POINT('Ctrl Pts',(55.0718435917456,-2.29217444186588,6.98633843920073));
#34909=CARTESIAN_POINT('Ctrl Pts',(55.2212211232311,-5.90500183263401,3.13752701480774));
#34910=CARTESIAN_POINT('Ctrl Pts',(55.3044281199024,-6.22455833697474,0.535573970350642));
#34911=CARTESIAN_POINT('Ctrl Pts',(55.3214645817597,-6.22177129455467,0.00223847925715545));
#34912=CARTESIAN_POINT('Origin',(28.1999754182402,0.,0.));
#34913=CARTESIAN_POINT('',(52.5749754182404,-6.21194719993059,0.00357180041802368));
#34914=CARTESIAN_POINT('',(52.8214645817597,-6.21925,8.34792304726939E-14));
#34915=CARTESIAN_POINT('',(28.1999754182402,-6.21925,5.68729293530136E-12));
#34916=CARTESIAN_POINT('Ctrl Pts',(52.5749754182404,-6.21194719993059,0.00357180041802359));
#34917=CARTESIAN_POINT('Ctrl Pts',(52.618238573557,-6.20225771496113,-1.35305654649645));
#34918=CARTESIAN_POINT('Ctrl Pts',(52.7276722636877,-5.09844079489878,-4.79761319256802));
#34919=CARTESIAN_POINT('Ctrl Pts',(52.8701912212252,-0.494508874927136,
-6.83955822169301));
#34920=CARTESIAN_POINT('Ctrl Pts',(53.0025322908534,3.54103930044635,-5.41695307870284));
#34921=CARTESIAN_POINT('Ctrl Pts',(53.1017880930744,5.71572828749395,-3.07476573264209));
#34922=CARTESIAN_POINT('Ctrl Pts',(53.2010438952954,6.47158394013595,0.0306804489560287));
#34923=CARTESIAN_POINT('Ctrl Pts',(53.3333849649236,5.43455561682152,4.18206897874528));
#34924=CARTESIAN_POINT('Ctrl Pts',(53.4988113019586,0.511680132839369,7.33492821373557));
#34925=CARTESIAN_POINT('Ctrl Pts',(53.6737032088666,-5.1295763542309,4.74832352785551));
#34926=CARTESIAN_POINT('Ctrl Pts',(53.7824245809605,-6.20557407876551,1.32941708371486));
#34927=CARTESIAN_POINT('Ctrl Pts',(53.8249754182404,-6.2138011505806,-0.00394554431260567));
#34928=CARTESIAN_POINT('Ctrl Pts',(52.8214645817597,-6.21922526303958,-0.00141380809610282));
#34929=CARTESIAN_POINT('Ctrl Pts',(52.8437150354673,-6.22231424961983,-0.698568023883329));
#34930=CARTESIAN_POINT('Ctrl Pts',(52.9321360239888,-5.77659188785169,-3.46761533849687));
#34931=CARTESIAN_POINT('Ctrl Pts',(53.0867275473246,-1.73635698912002,-7.14479200994201));
#34932=CARTESIAN_POINT('Ctrl Pts',(53.2852391517666,5.06891690010915,-5.32600842627953));
#34933=CARTESIAN_POINT('Ctrl Pts',(53.4837507562088,7.22419817707089,1.36793457278422));
#34934=CARTESIAN_POINT('Ctrl Pts',(53.6822623606508,2.75856009795156,6.81566831976048));
#34935=CARTESIAN_POINT('Ctrl Pts',(53.847688697686,-3.04851381910718,6.14252872927938));
#34936=CARTESIAN_POINT('Ctrl Pts',(53.9774227713888,-5.74765690702425,2.93163669228894));
#34937=CARTESIAN_POINT('Ctrl Pts',(54.0409863102778,-6.22014780735358,0.948971678600679));
#34938=CARTESIAN_POINT('Ctrl Pts',(54.0714645817597,-6.2215550358857,-0.000870493656276667));
#34939=CARTESIAN_POINT('Origin',(28.1999754182402,0.,0.));
#34940=CARTESIAN_POINT('',(51.3249754182404,-6.22918278048295,0.000765166614752994));
#34941=CARTESIAN_POINT('',(51.5714645817597,-6.21798365229328,8.59752551505447E-5));
#34942=CARTESIAN_POINT('',(28.1999754182402,-6.21925,5.68729293530136E-12));
#34943=CARTESIAN_POINT('Ctrl Pts',(51.3249754182404,-6.22918278048295,0.00076516661475276));
#34944=CARTESIAN_POINT('Ctrl Pts',(51.3878820313394,-6.22114725490248,-1.95451838237354));
#34945=CARTESIAN_POINT('Ctrl Pts',(51.4838739118454,-4.69363132187248,-4.94233563448507));
#34946=CARTESIAN_POINT('Ctrl Pts',(51.6129510597586,-0.791714381456252,
-6.42304665422641));
#34947=CARTESIAN_POINT('Ctrl Pts',(51.7122068619796,2.38108318749985,-6.03772945910084));
#34948=CARTESIAN_POINT('Ctrl Pts',(51.8114626642006,4.96281693597846,-4.15364755897021));
#34949=CARTESIAN_POINT('Ctrl Pts',(51.9438037338288,6.85024388311463,-0.313455638265433));
#34950=CARTESIAN_POINT('Ctrl Pts',(52.1092300708638,5.12514934704392,5.27217532234014));
#34951=CARTESIAN_POINT('Ctrl Pts',(52.307741675306,-1.66057365242597,7.16259585917574));
#34952=CARTESIAN_POINT('Ctrl Pts',(52.4629901244314,-5.77184773115307,3.5095666463159));
#34953=CARTESIAN_POINT('Ctrl Pts',(52.5520680387429,-6.21707767891914,0.721892046649002));
#34954=CARTESIAN_POINT('Ctrl Pts',(52.5749754182404,-6.21194719993059,0.00357180041802359));
#34955=CARTESIAN_POINT('Ctrl Pts',(51.5714645817597,-6.21925,3.77650582544623E-14));
#34956=CARTESIAN_POINT('Ctrl Pts',(51.6302643332334,-6.21925000000001,-1.83816020915746));
#34957=CARTESIAN_POINT('Ctrl Pts',(51.6890640847071,-5.35502977485011,-3.65808141345961));
#34958=CARTESIAN_POINT('Ctrl Pts',(51.7478638361808,-3.93049712175819,-4.81977830800863));
#34959=CARTESIAN_POINT('Ctrl Pts',(51.8066635876545,-2.50596446866627,-5.98147520255765));
#34960=CARTESIAN_POINT('Ctrl Pts',(51.8654633391282,-0.549389021418235,
-6.46189408921061));
#34961=CARTESIAN_POINT('Ctrl Pts',(51.9242630906019,1.25118869866967,-6.0920930231589));
#34962=CARTESIAN_POINT('Ctrl Pts',(51.9830628420756,3.05176641875757,-5.72229195710718));
#34963=CARTESIAN_POINT('Ctrl Pts',(52.0418625935493,4.66061422075278,-4.5096095842486));
#34964=CARTESIAN_POINT('Ctrl Pts',(52.100662345023,5.51197192302763,-2.88049233330955));
#34965=CARTESIAN_POINT('Ctrl Pts',(52.1594620964967,6.36332962530248,-1.25137508237049));
#34966=CARTESIAN_POINT('Ctrl Pts',(52.2182618479704,6.4403021637727,0.761847462642404));
#34967=CARTESIAN_POINT('Ctrl Pts',(52.2770615994441,5.71582172177393,2.45121451680536));
#34968=CARTESIAN_POINT('Ctrl Pts',(52.3358613509178,4.99134127977516,4.14058157096831));
#34969=CARTESIAN_POINT('Ctrl Pts',(52.3946611023915,3.47978506146339,5.47256790209552));
#34970=CARTESIAN_POINT('Ctrl Pts',(52.4534608538652,1.71270012775509,5.97877318811206));
#34971=CARTESIAN_POINT('Ctrl Pts',(52.5122606053389,-0.0543848059532034,
6.48497847412861));
#34972=CARTESIAN_POINT('Ctrl Pts',(52.5710603568126,-2.0419309233759,6.15535714814268));
#34973=CARTESIAN_POINT('Ctrl Pts',(52.6298601082863,-3.55100669662581,5.10582236304972));
#34974=CARTESIAN_POINT('Ctrl Pts',(52.68865985976,-5.06008246987572,4.05628757795677));
#34975=CARTESIAN_POINT('Ctrl Pts',(52.7474596112337,-6.06074051980899,2.30766719190081));
#34976=CARTESIAN_POINT('Ctrl Pts',(52.8062593627074,-6.20109393743687,0.474873184738493));
#34977=CARTESIAN_POINT('Ctrl Pts',(52.8113277690581,-6.21319208641587,0.316890462826823));
#34978=CARTESIAN_POINT('Ctrl Pts',(52.8163961754089,-6.21925,0.158445276456461));
#34979=CARTESIAN_POINT('Ctrl Pts',(52.8214645817597,-6.21925,8.34787642693416E-14));
#34980=CARTESIAN_POINT('Origin',(28.1999754182402,0.,0.));
#34981=CARTESIAN_POINT('',(50.0749754182403,-6.21439911675028,-0.00289789719525526));
#34982=CARTESIAN_POINT('',(50.3214645817597,-6.22838628080824,0.00457472256878852));
#34983=CARTESIAN_POINT('',(28.1999754182402,-6.21925,5.68729293530136E-12));
#34984=CARTESIAN_POINT('Ctrl Pts',(50.0749754182403,-6.21439911675028,-0.00289789719525507));
#34985=CARTESIAN_POINT('Ctrl Pts',(50.0913549543078,-6.2190407860767,-0.515297532616419));
#34986=CARTESIAN_POINT('Ctrl Pts',(50.1408197577822,-6.04526190938845,-2.06095057890313));
#34987=CARTESIAN_POINT('Ctrl Pts',(50.2233698286639,-4.75046670097809,-4.39492959068425));
#34988=CARTESIAN_POINT('Ctrl Pts',(50.3226256308848,-2.07837204216358,-6.14850419382157));
#34989=CARTESIAN_POINT('Ctrl Pts',(50.4218814331059,1.10964349084127,-6.37581612873264));
#34990=CARTESIAN_POINT('Ctrl Pts',(50.554222502734,5.02991597370948,-4.66090559792109));
#34991=CARTESIAN_POINT('Ctrl Pts',(50.719648839769,7.31752721429885,0.718876851061941));
#34992=CARTESIAN_POINT('Ctrl Pts',(50.9181604442113,3.35474386460336,6.54262775189899));
#34993=CARTESIAN_POINT('Ctrl Pts',(51.1166720486532,-3.6754491338023,6.36799481484125));
#34994=CARTESIAN_POINT('Ctrl Pts',(51.2522770399964,-6.18160088298851,2.26024312233628));
#34995=CARTESIAN_POINT('Ctrl Pts',(51.3217114965254,-6.22959970527259,0.102215429474412));
#34996=CARTESIAN_POINT('Ctrl Pts',(51.3249754182404,-6.22918278048295,0.00076516661475276));
#34997=CARTESIAN_POINT('Ctrl Pts',(50.3214645817597,-6.22838628080824,0.00457472256878885));
#34998=CARTESIAN_POINT('Ctrl Pts',(50.3830019510321,-6.21821227336961,-1.9098165579918));
#34999=CARTESIAN_POINT('Ctrl Pts',(50.5107098551187,-4.24352685123475,-5.90977734476775));
#35000=CARTESIAN_POINT('Ctrl Pts',(50.7045882940192,2.55369426009361,-6.89484807105841));
#35001=CARTESIAN_POINT('Ctrl Pts',(50.9030998984613,7.1802970231816,-1.58313711278791));
#35002=CARTESIAN_POINT('Ctrl Pts',(51.0685262354964,5.54802698009573,4.03032161538502));
#35003=CARTESIAN_POINT('Ctrl Pts',(51.2008673051245,1.8592571864357,6.19883075255818));
#35004=CARTESIAN_POINT('Ctrl Pts',(51.3001231073455,-1.33318551163412,6.35187771912034));
#35005=CARTESIAN_POINT('Ctrl Pts',(51.3993789095666,-4.19468734797827,4.92817796319135));
#35006=CARTESIAN_POINT('Ctrl Pts',(51.4898260677046,-5.90711317747617,2.55757447662341));
#35007=CARTESIAN_POINT('Ctrl Pts',(51.5471879584357,-6.21271273978697,0.761507326426199));
#35008=CARTESIAN_POINT('Ctrl Pts',(51.5714645817597,-6.20863502281416,0.000720675188000328));
#35009=CARTESIAN_POINT('Origin',(28.1999754182402,0.,0.));
#35010=CARTESIAN_POINT('',(48.8249754182404,-6.2166083149304,-0.000591004908469454));
#35011=CARTESIAN_POINT('',(49.0714645817597,-6.21899721478014,-0.005340755338481));
#35012=CARTESIAN_POINT('',(28.1999754182402,-6.21925,5.68729293530136E-12));
#35013=CARTESIAN_POINT('Ctrl Pts',(48.8249754182404,-6.2166083149304,-0.000591004908469146));
#35014=CARTESIAN_POINT('Ctrl Pts',(48.8279131446832,-6.21638226706522,-0.092651946701776));
#35015=CARTESIAN_POINT('Ctrl Pts',(48.8639361385331,-6.18899652759796,-1.22134599105756));
#35016=CARTESIAN_POINT('Ctrl Pts',(48.93304439979,-5.55601616227824,-3.3547605833489));
#35017=CARTESIAN_POINT('Ctrl Pts',(49.0323002020111,-3.26771921629748,-5.58608549053932));
#35018=CARTESIAN_POINT('Ctrl Pts',(49.1646412716392,0.833484420250366,-6.80657031231661));
#35019=CARTESIAN_POINT('Ctrl Pts',(49.3300676086743,6.05314692292063,-4.17401494828823));
#35020=CARTESIAN_POINT('Ctrl Pts',(49.5285792131164,6.78529949630181,2.83195957642392));
#35021=CARTESIAN_POINT('Ctrl Pts',(49.7270908175584,1.30290129179695,7.23620981735928));
#35022=CARTESIAN_POINT('Ctrl Pts',(49.9092228859333,-4.82912622707473,5.19479701430948));
#35023=CARTESIAN_POINT('Ctrl Pts',(50.0251844194937,-6.20028923288899,1.55470968704536));
#35024=CARTESIAN_POINT('Ctrl Pts',(50.0749754182403,-6.21439911675028,-0.00289789719525507));
#35025=CARTESIAN_POINT('Ctrl Pts',(49.0714645817597,-6.21899721478014,-0.00534075533848107));
#35026=CARTESIAN_POINT('Ctrl Pts',(49.0864748740005,-6.22356854582095,-0.474708533744452));
#35027=CARTESIAN_POINT('Ctrl Pts',(49.1676557010554,-5.96234790315834,-3.00834188896351));
#35028=CARTESIAN_POINT('Ctrl Pts',(49.3150070629244,-2.4997580926362,-6.91458558232614));
#35029=CARTESIAN_POINT('Ctrl Pts',(49.5135186673665,4.46249608146065,-5.84372459840002));
#35030=CARTESIAN_POINT('Ctrl Pts',(49.6789450044016,6.838968356171,-0.502600754676708));
#35031=CARTESIAN_POINT('Ctrl Pts',(49.8112860740297,5.42113886922714,3.53462775193207));
#35032=CARTESIAN_POINT('Ctrl Pts',(49.9105418762507,3.08152614660459,5.71208637669992));
#35033=CARTESIAN_POINT('Ctrl Pts',(50.0097976784718,-0.0230235705233395,
6.47161571011243));
#35034=CARTESIAN_POINT('Ctrl Pts',(50.1421387480999,-4.17563615511025,5.43949982952901));
#35035=CARTESIAN_POINT('Ctrl Pts',(50.2460277158625,-6.15931160573698,2.35024230288155));
#35036=CARTESIAN_POINT('Ctrl Pts',(50.3168314162181,-6.22915228464041,0.148709771223719));
#35037=CARTESIAN_POINT('Ctrl Pts',(50.3214645817597,-6.22838628080824,0.00457472256878885));
#35038=CARTESIAN_POINT('Origin',(28.1999754182402,0.,0.));
#35039=CARTESIAN_POINT('',(47.5749754182404,-6.21925,3.75611000635878E-13));
#35040=CARTESIAN_POINT('',(47.8214645817597,-6.21071229255457,0.000741149837754085));
#35041=CARTESIAN_POINT('',(28.1999754182402,-6.21925,5.68729293530136E-12));
#35042=CARTESIAN_POINT('Ctrl Pts',(47.5749754182404,-6.21933081007893,0.00292931974371469));
#35043=CARTESIAN_POINT('Ctrl Pts',(47.5975566024657,-6.2170155757593,-0.701663893040958));
#35044=CARTESIAN_POINT('Ctrl Pts',(47.653223054098,-5.91532415731919,-2.44161599281549));
#35045=CARTESIAN_POINT('Ctrl Pts',(47.7750600405443,-3.756680423898,-5.73684999699412));
#35046=CARTESIAN_POINT('Ctrl Pts',(47.9404863775796,1.92929451774911,-7.09512587082007));
#35047=CARTESIAN_POINT('Ctrl Pts',(48.1389979820215,7.01051831056036,-2.21651016562319));
#35048=CARTESIAN_POINT('Ctrl Pts',(48.3375095864638,5.66576857146238,4.68608053618823));
#35049=CARTESIAN_POINT('Ctrl Pts',(48.5360211909057,-0.875229719861018,
7.30047679240671));
#35050=CARTESIAN_POINT('Ctrl Pts',(48.6985098014981,-5.55095834388157,3.96734594113617));
#35051=CARTESIAN_POINT('Ctrl Pts',(48.7948278772762,-6.21892806369116,0.94415693805931));
#35052=CARTESIAN_POINT('Ctrl Pts',(48.8249754182404,-6.2166083149304,-0.000591004908469146));
#35053=CARTESIAN_POINT('Ctrl Pts',(47.8214645817597,-6.21071229255457,0.000741149837754154));
#35054=CARTESIAN_POINT('Ctrl Pts',(47.856118331783,-6.20949620099682,-1.08651601273864));
#35055=CARTESIAN_POINT('Ctrl Pts',(47.9569426166203,-5.41832110916315,-4.25151146531121));
#35056=CARTESIAN_POINT('Ctrl Pts',(48.1239374362717,-0.363362580539744,
-7.34376988297294));
#35057=CARTESIAN_POINT('Ctrl Pts',(48.2893637733068,4.89922005122494,-4.79809739219469));
#35058=CARTESIAN_POINT('Ctrl Pts',(48.4217048429349,6.42210544142411,-0.79931325736819));
#35059=CARTESIAN_POINT('Ctrl Pts',(48.5209606451559,6.04054241262091,2.37393797905852));
#35060=CARTESIAN_POINT('Ctrl Pts',(48.620216447377,4.1595164104518,4.95789907272788));
#35061=CARTESIAN_POINT('Ctrl Pts',(48.7525575170051,0.321560287482606,6.84986822331817));
#35062=CARTESIAN_POINT('Ctrl Pts',(48.9029735617993,-4.75909947860206,5.28731370912977));
#35063=CARTESIAN_POINT('Ctrl Pts',(49.0203043391865,-6.20341654511846,1.59442619216282));
#35064=CARTESIAN_POINT('Ctrl Pts',(49.0714645817597,-6.21899721478014,-0.00534075533848107));
#35065=CARTESIAN_POINT('Origin',(28.1999754182402,0.,0.));
#35066=CARTESIAN_POINT('',(46.3249754182404,-6.21925,3.29897242091433E-13));
#35067=CARTESIAN_POINT('',(46.5714645817596,-6.22210936345043,0.0051709891022092));
#35068=CARTESIAN_POINT('',(28.1999754182402,-6.21925,5.68729293530136E-12));
#35069=CARTESIAN_POINT('Ctrl Pts',(46.3249754182404,-6.21925,3.29897242091433E-13));
#35070=CARTESIAN_POINT('Ctrl Pts',(46.3837751697141,-6.2192500000001,-1.83816020915711));
#35071=CARTESIAN_POINT('Ctrl Pts',(46.4425749211878,-5.35502977485034,-3.65808141345925));
#35072=CARTESIAN_POINT('Ctrl Pts',(46.5013746726615,-3.93049712175856,-4.81977830800834));
#35073=CARTESIAN_POINT('Ctrl Pts',(46.5601744241352,-2.50596446866677,-5.98147520255743));
#35074=CARTESIAN_POINT('Ctrl Pts',(46.6189741756089,-0.549389021418848,
-6.46189408921054));
#35075=CARTESIAN_POINT('Ctrl Pts',(46.6777739270826,1.25118869866904,-6.09209302315903));
#35076=CARTESIAN_POINT('Ctrl Pts',(46.7365736785563,3.05176641875692,-5.72229195710751));
#35077=CARTESIAN_POINT('Ctrl Pts',(46.7953734300299,4.66061422075222,-4.50960958424917));
#35078=CARTESIAN_POINT('Ctrl Pts',(46.8541731815036,5.51197192302725,-2.88049233331027));
#35079=CARTESIAN_POINT('Ctrl Pts',(46.9129729329773,6.36332962530229,-1.25137508237138));
#35080=CARTESIAN_POINT('Ctrl Pts',(46.971772684451,6.4403021637728,0.761847462641424));
#35081=CARTESIAN_POINT('Ctrl Pts',(47.0305724359247,5.71582172177432,2.45121451680444));
#35082=CARTESIAN_POINT('Ctrl Pts',(47.0893721873984,4.99134127977585,4.14058157096745));
#35083=CARTESIAN_POINT('Ctrl Pts',(47.1481719388721,3.47978506146436,5.47256790209488));
#35084=CARTESIAN_POINT('Ctrl Pts',(47.2069716903458,1.71270012775622,5.97877318811174));
#35085=CARTESIAN_POINT('Ctrl Pts',(47.2657714418195,-0.0543848059519203,
6.4849784741286));
#35086=CARTESIAN_POINT('Ctrl Pts',(47.3245711932932,-2.04193092337461,6.15535714814309));
#35087=CARTESIAN_POINT('Ctrl Pts',(47.3833709447669,-3.5510066966247,5.1058223630505));
#35088=CARTESIAN_POINT('Ctrl Pts',(47.4421706962406,-5.06008246987479,4.0562875779579));
#35089=CARTESIAN_POINT('Ctrl Pts',(47.5009704477143,-6.06074051980843,2.30766719190224));
#35090=CARTESIAN_POINT('Ctrl Pts',(47.559770199188,-6.20109393743675,0.474873184740018));
#35091=CARTESIAN_POINT('Ctrl Pts',(47.5648386055388,-6.21319208641582,0.316890462827939));
#35092=CARTESIAN_POINT('Ctrl Pts',(47.5699070118896,-6.21924999999999,0.158445276457166));
#35093=CARTESIAN_POINT('Ctrl Pts',(47.5749754182404,-6.21925,3.75610948106313E-13));
#35094=CARTESIAN_POINT('Ctrl Pts',(46.5714645817596,-6.22210936345043,0.00517098910220969));
#35095=CARTESIAN_POINT('Ctrl Pts',(46.6257617895654,-6.20584908536478,-1.6905361365724));
#35096=CARTESIAN_POINT('Ctrl Pts',(46.7462295321853,-4.61113712656708,-5.47890052593373));
#35097=CARTESIAN_POINT('Ctrl Pts',(46.899782542212,0.645108111263187,-6.82700016259648));
#35098=CARTESIAN_POINT('Ctrl Pts',(47.0321236118402,4.38930599811985,-4.75566323860751));
#35099=CARTESIAN_POINT('Ctrl Pts',(47.1313794140611,6.14604086368536,-2.08564519249999));
#35100=CARTESIAN_POINT('Ctrl Pts',(47.2306352162823,6.37712454126565,1.10209916493979));
#35101=CARTESIAN_POINT('Ctrl Pts',(47.3629762859102,4.66685348261288,5.0243979009563));
#35102=CARTESIAN_POINT('Ctrl Pts',(47.5284026229454,-0.710218612843849,
7.31837263201097));
#35103=CARTESIAN_POINT('Ctrl Pts',(47.6922604773642,-5.52119639342655,4.05305379686667));
#35104=CARTESIAN_POINT('Ctrl Pts',(47.7899477969689,-6.21181829972221,0.98957641245848));
#35105=CARTESIAN_POINT('Ctrl Pts',(47.8214645817597,-6.21071229255457,0.000741149837754154));
#35106=CARTESIAN_POINT('Origin',(28.1999754182402,0.,0.));
#35107=CARTESIAN_POINT('',(45.0749754182404,-6.21854788291297,-0.000317205416753715));
#35108=CARTESIAN_POINT('',(45.3214645817596,-6.22620958835039,-0.00623427698102752));
#35109=CARTESIAN_POINT('',(28.1999754182402,-6.21925,5.68729293530136E-12));
#35110=CARTESIAN_POINT('Ctrl Pts',(45.0749754182404,-6.20821420870357,-0.00498579630805643));
#35111=CARTESIAN_POINT('Ctrl Pts',(45.1037582506235,-6.2119349975194,-0.906770203246303));
#35112=CARTESIAN_POINT('Ctrl Pts',(45.1987116178207,-5.6083688757905,-3.87600348080113));
#35113=CARTESIAN_POINT('Ctrl Pts',(45.3598355198321,-1.01618098913832,-7.2820093720296));
#35114=CARTESIAN_POINT('Ctrl Pts',(45.5583471242741,5.56543150817819,-4.80481596159418));
#35115=CARTESIAN_POINT('Ctrl Pts',(45.7568587287163,7.05223625244414,2.08061344288397));
#35116=CARTESIAN_POINT('Ctrl Pts',(45.9222850657513,2.91241425495877,6.20821543624437));
#35117=CARTESIAN_POINT('Ctrl Pts',(46.0546261353794,-1.3649168534335,6.32608425231493));
#35118=CARTESIAN_POINT('Ctrl Pts',(46.1538819376005,-4.23445444437469,4.9186512099969));
#35119=CARTESIAN_POINT('Ctrl Pts',(46.2439983652208,-5.88542304071439,2.5322667313354));
#35120=CARTESIAN_POINT('Ctrl Pts',(46.3010295254341,-6.22263107846942,0.746134257446151));
#35121=CARTESIAN_POINT('Ctrl Pts',(46.3249754182404,-6.22573560541529,-0.00204345304936147));
#35122=CARTESIAN_POINT('Ctrl Pts',(45.3214645817597,-6.22620958835039,-0.00623427698102683));
#35123=CARTESIAN_POINT('Ctrl Pts',(45.3292347125338,-6.22805343704289,-0.248224525845919));
#35124=CARTESIAN_POINT('Ctrl Pts',(45.403175378122,-6.10552815017325,-2.54852208963383));
#35125=CARTESIAN_POINT('Ctrl Pts',(45.5102013111172,-3.91374922444537,-5.63086695842329));
#35126=CARTESIAN_POINT('Ctrl Pts',(45.6425423807454,0.283023412847933,-6.46546500508306));
#35127=CARTESIAN_POINT('Ctrl Pts',(45.7417981829663,3.34818463267598,-5.55998145973536));
#35128=CARTESIAN_POINT('Ctrl Pts',(45.8410539851874,5.58221537749888,-3.27432610828378));
#35129=CARTESIAN_POINT('Ctrl Pts',(45.9733950548155,6.80755168564738,0.825430640665489));
#35130=CARTESIAN_POINT('Ctrl Pts',(46.1388213918506,4.18117380984599,6.04820419883911));
#35131=CARTESIAN_POINT('Ctrl Pts',(46.3373329962928,-2.82392956463494,6.78864538114884));
#35132=CARTESIAN_POINT('Ctrl Pts',(46.481547392929,-6.02823238238414,2.80958978582469));
#35133=CARTESIAN_POINT('Ctrl Pts',(46.5595912547514,-6.22566504534934,0.375976156200805));
#35134=CARTESIAN_POINT('Ctrl Pts',(46.5714645817596,-6.22210936345043,0.00517098910220969));
#35135=CARTESIAN_POINT('Origin',(28.1999754182402,0.,0.));
#35136=CARTESIAN_POINT('',(43.8249754182404,-6.21925,4.15231546436714E-13));
#35137=CARTESIAN_POINT('',(44.0714645817597,-6.21730219627848,9.77522333141482E-5));
#35138=CARTESIAN_POINT('',(28.1999754182402,-6.21925,5.68729293530136E-12));
#35139=CARTESIAN_POINT('Ctrl Pts',(43.8249754182404,-6.21925,5.91993262811754E-13));
#35140=CARTESIAN_POINT('Ctrl Pts',(43.8837751697141,-6.21925000000018,-1.83816020915688));
#35141=CARTESIAN_POINT('Ctrl Pts',(43.9425749211877,-5.35502977485047,-3.65808141345908));
#35142=CARTESIAN_POINT('Ctrl Pts',(44.0013746726614,-3.93049712175869,-4.81977830800823));
#35143=CARTESIAN_POINT('Ctrl Pts',(44.0601744241351,-2.50596446866692,-5.98147520255737));
#35144=CARTESIAN_POINT('Ctrl Pts',(44.1189741756088,-0.549389021418965,
-6.46189408921054));
#35145=CARTESIAN_POINT('Ctrl Pts',(44.1777739270825,1.25118869866895,-6.09209302315904));
#35146=CARTESIAN_POINT('Ctrl Pts',(44.2365736785562,3.05176641875687,-5.72229195710755));
#35147=CARTESIAN_POINT('Ctrl Pts',(44.2953734300299,4.6606142207522,-4.50960958424919));
#35148=CARTESIAN_POINT('Ctrl Pts',(44.3541731815036,5.51197192302725,-2.88049233331027));
#35149=CARTESIAN_POINT('Ctrl Pts',(44.4129729329773,6.3633296253023,-1.25137508237135));
#35150=CARTESIAN_POINT('Ctrl Pts',(44.471772684451,6.4403021637728,0.761847462641492));
#35151=CARTESIAN_POINT('Ctrl Pts',(44.5305724359247,5.71582172177429,2.45121451680452));
#35152=CARTESIAN_POINT('Ctrl Pts',(44.5893721873984,4.99134127977578,4.14058157096755));
#35153=CARTESIAN_POINT('Ctrl Pts',(44.6481719388721,3.47978506146424,5.47256790209497));
#35154=CARTESIAN_POINT('Ctrl Pts',(44.7069716903458,1.71270012775605,5.97877318811179));
#35155=CARTESIAN_POINT('Ctrl Pts',(44.7657714418195,-0.0543848059521362,
6.48497847412861));
#35156=CARTESIAN_POINT('Ctrl Pts',(44.8245711932932,-2.04193092337485,6.15535714814302));
#35157=CARTESIAN_POINT('Ctrl Pts',(44.8833709447669,-3.55100669662492,5.10582236305034));
#35158=CARTESIAN_POINT('Ctrl Pts',(44.9421706962406,-5.06008246987499,4.05628757795767));
#35159=CARTESIAN_POINT('Ctrl Pts',(45.0009704477143,-6.06074051980856,2.30766719190193));
#35160=CARTESIAN_POINT('Ctrl Pts',(45.059770199188,-6.20109393743678,0.474873184739662));
#35161=CARTESIAN_POINT('Ctrl Pts',(45.0648386055388,-6.21319208641583,0.316890462827671));
#35162=CARTESIAN_POINT('Ctrl Pts',(45.0699070118896,-6.21924999999999,0.158445276456986));
#35163=CARTESIAN_POINT('Ctrl Pts',(45.0749754182404,-6.21925,2.84183536076554E-13));
#35164=CARTESIAN_POINT('Ctrl Pts',(44.0714645817597,-6.20735719350781,0.000596850939321783));
#35165=CARTESIAN_POINT('Ctrl Pts',(44.0988781703163,-6.21014037266732,-0.858805783627428));
#35166=CARTESIAN_POINT('Ctrl Pts',(44.1593770262799,-5.84277927858636,-2.75472237638653));
#35167=CARTESIAN_POINT('Ctrl Pts',(44.2529611496505,-3.9569578199035,-5.12101794526032));
#35168=CARTESIAN_POINT('Ctrl Pts',(44.3522169518716,-1.03133493987818,-6.40781416778569));
#35169=CARTESIAN_POINT('Ctrl Pts',(44.4514727540926,2.15029947849091,-6.10397838601804));
#35170=CARTESIAN_POINT('Ctrl Pts',(44.5838138237208,5.73240126379457,-3.76346535073147));
#35171=CARTESIAN_POINT('Ctrl Pts',(44.7492401607558,7.09740355031088,1.92089856656498));
#35172=CARTESIAN_POINT('Ctrl Pts',(44.9477517651979,2.22480311159819,7.00789093890849));
#35173=CARTESIAN_POINT('Ctrl Pts',(45.1384932388659,-4.40913087075351,5.72362536591463));
#35174=CARTESIAN_POINT('Ctrl Pts',(45.2630641777198,-6.21235119757683,1.81256758339546));
#35175=CARTESIAN_POINT('Ctrl Pts',(45.3214645817597,-6.22620958835039,-0.00623427698102683));
#35176=CARTESIAN_POINT('Origin',(28.1999754182402,0.,0.));
#35177=CARTESIAN_POINT('',(42.5749754182404,-6.22934530309283,-0.00155873460105957));
#35178=CARTESIAN_POINT('',(42.8214645817597,-6.21925,3.36435123462946E-13));
#35179=CARTESIAN_POINT('',(28.1999754182402,-6.21925,5.68729293530136E-12));
#35180=CARTESIAN_POINT('Ctrl Pts',(42.5749754182404,-6.22934530309283,-0.00155873460105878));
#35181=CARTESIAN_POINT('Ctrl Pts',(42.5768746313744,-6.22952614868411,-0.0606917412216028));
#35182=CARTESIAN_POINT('Ctrl Pts',(42.6449443793225,-6.20328599844248,-2.17990023331552));
#35183=CARTESIAN_POINT('Ctrl Pts',(42.7791846620846,-3.80925655132213,-6.2888670540267));
#35184=CARTESIAN_POINT('Ctrl Pts',(42.9776962665266,3.22770883173084,-6.60642748817874));
#35185=CARTESIAN_POINT('Ctrl Pts',(43.1431226035619,6.60701429937979,-1.83615297377451));
#35186=CARTESIAN_POINT('Ctrl Pts',(43.2754636731898,6.00981779016149,2.40092276286268));
#35187=CARTESIAN_POINT('Ctrl Pts',(43.3747194754109,4.14349036564128,4.9955201688039));
#35188=CARTESIAN_POINT('Ctrl Pts',(43.473975277632,1.24861120530404,6.35006378252714));
#35189=CARTESIAN_POINT('Ctrl Pts',(43.6063163472601,-3.02583705454058,6.15373104828925));
#35190=CARTESIAN_POINT('Ctrl Pts',(43.7233163941295,-5.89972442142763,3.18119516786605));
#35191=CARTESIAN_POINT('Ctrl Pts',(43.807231173592,-6.22164619015469,0.56313307617446));
#35192=CARTESIAN_POINT('Ctrl Pts',(43.8249754182404,-6.21669210645943,0.0080881789777975));
#35193=CARTESIAN_POINT('Ctrl Pts',(42.8214645817597,-6.21925,3.36435123462946E-13));
#35194=CARTESIAN_POINT('Ctrl Pts',(42.8802643332334,-6.2192500000001,-1.83816020915713));
#35195=CARTESIAN_POINT('Ctrl Pts',(42.9390640847071,-5.35502977485032,-3.6580814134593));
#35196=CARTESIAN_POINT('Ctrl Pts',(42.9978638361808,-3.93049712175849,-4.81977830800839));
#35197=CARTESIAN_POINT('Ctrl Pts',(43.0566635876545,-2.50596446866667,-5.98147520255748));
#35198=CARTESIAN_POINT('Ctrl Pts',(43.1154633391282,-0.5493890214187,-6.46189408921057));
#35199=CARTESIAN_POINT('Ctrl Pts',(43.1742630906019,1.2511886986692,-6.09209302315899));
#35200=CARTESIAN_POINT('Ctrl Pts',(43.2330628420756,3.05176641875711,-5.72229195710742));
#35201=CARTESIAN_POINT('Ctrl Pts',(43.2918625935493,4.66061422075239,-4.509609584249));
#35202=CARTESIAN_POINT('Ctrl Pts',(43.350662345023,5.51197192302737,-2.88049233331005));
#35203=CARTESIAN_POINT('Ctrl Pts',(43.4094620964967,6.36332962530235,-1.25137508237109));
#35204=CARTESIAN_POINT('Ctrl Pts',(43.4682618479704,6.44030216377276,0.761847462641756));
#35205=CARTESIAN_POINT('Ctrl Pts',(43.5270615994441,5.71582172177419,2.45121451680476));
#35206=CARTESIAN_POINT('Ctrl Pts',(43.5858613509178,4.99134127977561,4.14058157096776));
#35207=CARTESIAN_POINT('Ctrl Pts',(43.6446611023915,3.47978506146401,5.47256790209512));
#35208=CARTESIAN_POINT('Ctrl Pts',(43.7034608538652,1.7127001277558,5.97877318811186));
#35209=CARTESIAN_POINT('Ctrl Pts',(43.7622606053389,-0.0543848059524024,
6.4849784741286));
#35210=CARTESIAN_POINT('Ctrl Pts',(43.8210603568125,-2.0419309233751,6.15535714814294));
#35211=CARTESIAN_POINT('Ctrl Pts',(43.8798601082863,-3.55100669662513,5.1058223630502));
#35212=CARTESIAN_POINT('Ctrl Pts',(43.93865985976,-5.06008246987515,4.05628757795746));
#35213=CARTESIAN_POINT('Ctrl Pts',(43.9974596112336,-6.06074051980865,2.30766719190168));
#35214=CARTESIAN_POINT('Ctrl Pts',(44.0562593627073,-6.2010939374368,0.474873184739407));
#35215=CARTESIAN_POINT('Ctrl Pts',(44.0613277690581,-6.21319208641584,0.316890462827504));
#35216=CARTESIAN_POINT('Ctrl Pts',(44.0663961754089,-6.21924999999999,0.158445276456907));
#35217=CARTESIAN_POINT('Ctrl Pts',(44.0714645817597,-6.21925,2.93767971290306E-13));
#35218=CARTESIAN_POINT('Origin',(28.1999754182402,0.,0.));
#35219=CARTESIAN_POINT('',(41.3249754182403,-6.21523911303322,-0.00450227194547106));
#35220=CARTESIAN_POINT('',(41.5714645817597,-6.22175358549805,-0.000179260700348682));
#35221=CARTESIAN_POINT('',(28.1999754182402,-6.21925,5.68729293530136E-12));
#35222=CARTESIAN_POINT('Ctrl Pts',(41.3249754182403,-6.21523911303322,-0.00450227194547133));
#35223=CARTESIAN_POINT('Ctrl Pts',(41.3465180891568,-6.22007772484495,-0.679164296726016));
#35224=CARTESIAN_POINT('Ctrl Pts',(41.4342312948873,-5.80641375796907,-3.42039969603429));
#35225=CARTESIAN_POINT('Ctrl Pts',(41.5881150354319,-1.7987828877996,-7.12933156625193));
#35226=CARTESIAN_POINT('Ctrl Pts',(41.753541372467,3.86131211317401,-5.66695371958917));
#35227=CARTESIAN_POINT('Ctrl Pts',(41.8858824420951,6.13999062787377,-2.04520294195858));
#35228=CARTESIAN_POINT('Ctrl Pts',(41.9851382443162,6.38916632461915,1.14117826979005));
#35229=CARTESIAN_POINT('Ctrl Pts',(42.0843940465372,5.05233903023813,4.04428118553917));
#35230=CARTESIAN_POINT('Ctrl Pts',(42.2167351161653,1.66078038279294,6.65326267446582));
#35231=CARTESIAN_POINT('Ctrl Pts',(42.3802622400663,-4.08881072896843,6.07255729926071));
#35232=CARTESIAN_POINT('Ctrl Pts',(42.5107040965604,-6.22322530267627,1.99956289956022));
#35233=CARTESIAN_POINT('Ctrl Pts',(42.5749754182404,-6.22934530309283,-0.00155873460105878));
#35234=CARTESIAN_POINT('Ctrl Pts',(41.5714645817596,-6.22175358549805,-0.000179260700348691));
#35235=CARTESIAN_POINT('Ctrl Pts',(41.5719945510671,-6.22175922636749,-0.0166938072709939));
#35236=CARTESIAN_POINT('Ctrl Pts',(41.6056097877816,-6.21775797837456,-1.06418559288761));
#35237=CARTESIAN_POINT('Ctrl Pts',(41.6723102919031,-5.65982942715753,-3.13825920530084));
#35238=CARTESIAN_POINT('Ctrl Pts',(41.8046513615312,-2.7546438300705,-6.2798115469148));
#35239=CARTESIAN_POINT('Ctrl Pts',(41.9700776985662,3.07776459442245,-6.67760088357463));
#35240=CARTESIAN_POINT('Ctrl Pts',(42.1685893030084,7.280801980269,-1.02479599000183));
#35241=CARTESIAN_POINT('Ctrl Pts',(42.3671009074504,4.81139734096477,5.55974279300492));
#35242=CARTESIAN_POINT('Ctrl Pts',(42.5656125118927,-2.0722681306563,7.05469299499727));
#35243=CARTESIAN_POINT('Ctrl Pts',(42.7170670699956,-5.85573779370101,3.26899088665945));
#35244=CARTESIAN_POINT('Ctrl Pts',(42.8023510932847,-6.22370194316221,0.600581950735336));
#35245=CARTESIAN_POINT('Ctrl Pts',(42.8214645817597,-6.22070394341143,0.00198527999243369));
#35246=CARTESIAN_POINT('Origin',(28.1999754182402,0.,0.));
#35247=CARTESIAN_POINT('',(40.0749754182403,-6.21056889989778,0.00266732454412204));
#35248=CARTESIAN_POINT('',(40.3214645817597,-6.21925,5.98531640916278E-13));
#35249=CARTESIAN_POINT('',(28.1999754182402,-6.21925,5.68729293530136E-12));
#35250=CARTESIAN_POINT('Ctrl Pts',(40.0749754182403,-6.21056889989778,0.00266732454412187));
#35251=CARTESIAN_POINT('Ctrl Pts',(40.1161615469393,-6.20290591724236,-1.28951842298143));
#35252=CARTESIAN_POINT('Ctrl Pts',(40.2235182104523,-5.18004941908787,-4.66744415132467));
#35253=CARTESIAN_POINT('Ctrl Pts',(40.3639601413723,-0.708451912413997,
-6.82071782022295));
#35254=CARTESIAN_POINT('Ctrl Pts',(40.4963012110003,3.3696668804336,-5.52518643116073));
#35255=CARTESIAN_POINT('Ctrl Pts',(40.5955570132214,5.6166365191778,-3.25224974110642));
#35256=CARTESIAN_POINT('Ctrl Pts',(40.6948128154424,6.46937068698724,-0.17199679800523));
#35257=CARTESIAN_POINT('Ctrl Pts',(40.8271538850705,5.56285463090548,4.00983092545351));
#35258=CARTESIAN_POINT('Ctrl Pts',(40.9925802221055,0.741127608027151,7.3153071246269));
#35259=CARTESIAN_POINT('Ctrl Pts',(41.1695491556312,-5.04628844301002,4.87802538828724));
#35260=CARTESIAN_POINT('Ctrl Pts',(41.2803475543428,-6.20521542979432,1.39312967144128));
#35261=CARTESIAN_POINT('Ctrl Pts',(41.3249754182403,-6.21523911303322,-0.00450227194547133));
#35262=CARTESIAN_POINT('Ctrl Pts',(40.3214645817597,-6.22018273820767,-0.00181530436698364));
#35263=CARTESIAN_POINT('Ctrl Pts',(40.3416380088496,-6.22324239534247,-0.63371717248096));
#35264=CARTESIAN_POINT('Ctrl Pts',(40.4279819707534,-5.829640410661,-3.3360972611883));
#35265=CARTESIAN_POINT('Ctrl Pts',(40.5804964674716,-1.95924956424283,-7.08691255794874));
#35266=CARTESIAN_POINT('Ctrl Pts',(40.7790080719135,4.89964311770096,-5.48213294404453));
#35267=CARTESIAN_POINT('Ctrl Pts',(40.9775196763558,7.26349285183276,1.1410328165251));
#35268=CARTESIAN_POINT('Ctrl Pts',(41.1760312807977,2.97064458683377,6.72593927996026));
#35269=CARTESIAN_POINT('Ctrl Pts',(41.3414576178329,-2.85466105015735,6.23498243654499));
#35270=CARTESIAN_POINT('Ctrl Pts',(41.4732687181535,-5.69783323613032,3.06016323492747));
#35271=CARTESIAN_POINT('Ctrl Pts',(41.5389092836601,-6.22140707451404,1.01428700936641));
#35272=CARTESIAN_POINT('Ctrl Pts',(41.5714645817596,-6.22175358549805,-0.000179260700348691));
#35273=CARTESIAN_POINT('Origin',(28.1999754182402,0.,0.));
#35274=CARTESIAN_POINT('',(38.8249754182403,-6.22814110134059,0.00214874350932149));
#35275=CARTESIAN_POINT('',(39.0714645817597,-6.21833151244906,-1.0638405337316E-5));
#35276=CARTESIAN_POINT('',(28.1999754182402,-6.21925,5.68729293530136E-12));
#35277=CARTESIAN_POINT('Ctrl Pts',(38.8249754182403,-6.22814110134059,0.00214874350932153));
#35278=CARTESIAN_POINT('Ctrl Pts',(38.8858050047217,-6.216610570833,-1.88918205659997));
#35279=CARTESIAN_POINT('Ctrl Pts',(38.9797198586102,-4.7840918117624,-4.8187084571317));
#35280=CARTESIAN_POINT('Ctrl Pts',(39.1067199799055,-0.992468299979939,
-6.39510333440429));
#35281=CARTESIAN_POINT('Ctrl Pts',(39.2059757821266,2.19083962730784,-6.10933350657059));
#35282=CARTESIAN_POINT('Ctrl Pts',(39.3052315843476,4.83030849556222,-4.30702447425982));
#35283=CARTESIAN_POINT('Ctrl Pts',(39.4375726539757,6.83706805014439,-0.527822103558383));
#35284=CARTESIAN_POINT('Ctrl Pts',(39.6029989910108,5.28773755787813,5.10909189367368));
#35285=CARTESIAN_POINT('Ctrl Pts',(39.8015105954529,-1.43545748919326,7.2110849456744));
#35286=CARTESIAN_POINT('Ctrl Pts',(39.9588360711961,-5.71561946767958,3.6414683897976));
#35287=CARTESIAN_POINT('Ctrl Pts',(40.0499910121252,-6.21521743271123,0.786535449862077));
#35288=CARTESIAN_POINT('Ctrl Pts',(40.0749754182403,-6.21056889989778,0.00266732454412187));
#35289=CARTESIAN_POINT('Ctrl Pts',(39.0714645817597,-6.21925,4.64436579980868E-13));
#35290=CARTESIAN_POINT('Ctrl Pts',(39.1302643332334,-6.21925000000014,-1.83816020915697));
#35291=CARTESIAN_POINT('Ctrl Pts',(39.1890640847071,-5.35502977485042,-3.65808141345913));
#35292=CARTESIAN_POINT('Ctrl Pts',(39.2478638361808,-3.93049712175866,-4.81977830800825));
#35293=CARTESIAN_POINT('Ctrl Pts',(39.3066635876544,-2.5059644686669,-5.98147520255737));
#35294=CARTESIAN_POINT('Ctrl Pts',(39.3654633391281,-0.549389021418988,
-6.46189408921053));
#35295=CARTESIAN_POINT('Ctrl Pts',(39.4242630906018,1.2511886986689,-6.09209302315905));
#35296=CARTESIAN_POINT('Ctrl Pts',(39.4830628420755,3.0517664187568,-5.72229195710758));
#35297=CARTESIAN_POINT('Ctrl Pts',(39.5418625935492,4.66061422075212,-4.50960958424927));
#35298=CARTESIAN_POINT('Ctrl Pts',(39.6006623450229,5.51197192302719,-2.88049233331039));
#35299=CARTESIAN_POINT('Ctrl Pts',(39.6594620964966,6.36332962530226,-1.25137508237152));
#35300=CARTESIAN_POINT('Ctrl Pts',(39.7182618479703,6.44030216377281,0.761847462641284));
#35301=CARTESIAN_POINT('Ctrl Pts',(39.777061599444,5.71582172177438,2.45121451680431));
#35302=CARTESIAN_POINT('Ctrl Pts',(39.8358613509177,4.99134127977594,4.14058157096734));
#35303=CARTESIAN_POINT('Ctrl Pts',(39.8946611023914,3.47978506146448,5.47256790209481));
#35304=CARTESIAN_POINT('Ctrl Pts',(39.9534608538651,1.71270012775635,5.9787731881117));
#35305=CARTESIAN_POINT('Ctrl Pts',(40.0122606053388,-0.0543848059517801,
6.4849784741286));
#35306=CARTESIAN_POINT('Ctrl Pts',(40.0710603568125,-2.04193092337447,6.15535714814314));
#35307=CARTESIAN_POINT('Ctrl Pts',(40.1298601082862,-3.55100669662459,5.10582236305057));
#35308=CARTESIAN_POINT('Ctrl Pts',(40.1886598597599,-5.0600824698747,4.05628757795801));
#35309=CARTESIAN_POINT('Ctrl Pts',(40.2474596112336,-6.06074051980838,2.30766719190237));
#35310=CARTESIAN_POINT('Ctrl Pts',(40.3062593627073,-6.20109393743674,0.474873184740152));
#35311=CARTESIAN_POINT('Ctrl Pts',(40.3113277690581,-6.21319208641581,0.316890462828103));
#35312=CARTESIAN_POINT('Ctrl Pts',(40.3163961754089,-6.21924999999998,0.158445276457359));
#35313=CARTESIAN_POINT('Ctrl Pts',(40.3214645817597,-6.21925,5.98531144183268E-13));
#35314=CARTESIAN_POINT('Origin',(28.1999754182402,0.,0.));
#35315=CARTESIAN_POINT('',(37.5749754182404,-6.21630311580474,-0.00309819098741701));
#35316=CARTESIAN_POINT('',(37.8214645817596,-6.22702764812334,0.00572193935648446));
#35317=CARTESIAN_POINT('',(28.1999754182402,-6.21925,5.68729293530136E-12));
#35318=CARTESIAN_POINT('Ctrl Pts',(37.5749754182404,-6.21630311580474,-0.00309819098741684));
#35319=CARTESIAN_POINT('Ctrl Pts',(37.5892779276901,-6.22053647474818,-0.45026242937358));
#35320=CARTESIAN_POINT('Ctrl Pts',(37.6366657045469,-6.07611397572792,-1.93034435153842));
#35321=CARTESIAN_POINT('Ctrl Pts',(37.7171387488107,-4.88576711085616,-4.2440098636368));
#35322=CARTESIAN_POINT('Ctrl Pts',(37.8163945510318,-2.26989742046013,-6.08040293629282));
#35323=CARTESIAN_POINT('Ctrl Pts',(37.9156503532528,0.909436095338548,-6.40743833155411));
#35324=CARTESIAN_POINT('Ctrl Pts',(38.0479914228809,4.88148948210039,-4.81613497853341));
#35325=CARTESIAN_POINT('Ctrl Pts',(38.213417759916,7.33645041645639,0.489370765242909));
#35326=CARTESIAN_POINT('Ctrl Pts',(38.4119293643581,3.55798549376158,6.43436271305828));
#35327=CARTESIAN_POINT('Ctrl Pts',(38.6104409688003,-3.4742282511699,6.47997086072042));
#35328=CARTESIAN_POINT('Ctrl Pts',(38.748122986761,-6.14812552610466,2.39103132068625));
#35329=CARTESIAN_POINT('Ctrl Pts',(38.8196344699077,-6.2291535028914,0.168211027796827));
#35330=CARTESIAN_POINT('Ctrl Pts',(38.8249754182403,-6.22814110134059,0.00214874350932153));
#35331=CARTESIAN_POINT('Ctrl Pts',(37.8214645817596,-6.22702764812334,0.00572193935648436));
#35332=CARTESIAN_POINT('Ctrl Pts',(37.8809249244144,-6.214154207475,-1.84534440380487));
#35333=CARTESIAN_POINT('Ctrl Pts',(38.0065558018834,-4.3540617358176,-5.78681812394731));
#35334=CARTESIAN_POINT('Ctrl Pts',(38.1983572141661,2.33652476986658,-6.97143717584924));
#35335=CARTESIAN_POINT('Ctrl Pts',(38.3968688186083,7.12719834562496,-1.8072167000993));
#35336=CARTESIAN_POINT('Ctrl Pts',(38.5622951556433,5.67151826603053,3.85460455214176));
#35337=CARTESIAN_POINT('Ctrl Pts',(38.6946362252714,2.05246604268208,6.13756654772971));
#35338=CARTESIAN_POINT('Ctrl Pts',(38.7938920274925,-1.13361812652741,6.39051203819357));
#35339=CARTESIAN_POINT('Ctrl Pts',(38.8931478297135,-4.03830067804228,5.0571204867886));
#35340=CARTESIAN_POINT('Ctrl Pts',(38.9856720144692,-5.86513335389985,2.6881251712379));
#35341=CARTESIAN_POINT('Ctrl Pts',(39.045110931818,-6.21100116850847,0.82596242185995));
#35342=CARTESIAN_POINT('Ctrl Pts',(39.0714645817597,-6.20771145695589,-0.000133645472617031));
#35343=CARTESIAN_POINT('Origin',(28.1999754182402,0.,0.));
#35344=CARTESIAN_POINT('',(36.3249754182403,-6.2162013314378,-0.0011376377559993));
#35345=CARTESIAN_POINT('',(36.5714645817597,-6.2210655398886,-0.00528659965813971));
#35346=CARTESIAN_POINT('',(28.1999754182402,-6.21925,5.68729293530136E-12));
#35347=CARTESIAN_POINT('Ctrl Pts',(36.3249754182403,-6.2162013314378,-0.00113763775599949));
#35348=CARTESIAN_POINT('Ctrl Pts',(36.3258361180656,-6.21614725314266,-0.0281046714168168));
#35349=CARTESIAN_POINT('Ctrl Pts',(36.3597820852978,-6.20720164280366,-1.09161759141586));
#35350=CARTESIAN_POINT('Ctrl Pts',(36.426813319937,-5.65834786130082,-3.17912466680208));
#35351=CARTESIAN_POINT('Ctrl Pts',(36.526069122158,-3.44104873410895,-5.48101483247933));
#35352=CARTESIAN_POINT('Ctrl Pts',(36.6584101917862,0.619923098873849,-6.82933313338426));
#35353=CARTESIAN_POINT('Ctrl Pts',(36.8238365288212,5.919465903525,-4.36152632411429));
#35354=CARTESIAN_POINT('Ctrl Pts',(37.0223481332634,6.8706564039049,2.61808419966792));
#35355=CARTESIAN_POINT('Ctrl Pts',(37.2208597377055,1.52886927114417,7.19185949867951));
#35356=CARTESIAN_POINT('Ctrl Pts',(37.4050688326978,-4.73470315697655,5.32239779041791));
#35357=CARTESIAN_POINT('Ctrl Pts',(37.5231073928761,-6.20095084704205,1.61854213304384));
#35358=CARTESIAN_POINT('Ctrl Pts',(37.5749754182404,-6.21630311580474,-0.00309819098741684));
#35359=CARTESIAN_POINT('Ctrl Pts',(36.5714645817597,-6.2210655398886,-0.0052865996581393));
#35360=CARTESIAN_POINT('Ctrl Pts',(36.5843978473829,-6.2249967155556,-0.409366363204161));
#35361=CARTESIAN_POINT('Ctrl Pts',(36.6635016478201,-6.00657242484259,-2.87671415514283));
#35362=CARTESIAN_POINT('Ctrl Pts',(36.8087759830713,-2.71506717634408,-6.83291259456277));
#35363=CARTESIAN_POINT('Ctrl Pts',(37.0072875875135,4.27730707652595,-5.98060470455043));
#35364=CARTESIAN_POINT('Ctrl Pts',(37.1727139245486,6.81987484110359,-0.716521351391848));
#35365=CARTESIAN_POINT('Ctrl Pts',(37.3050549941766,5.52916938658696,3.36312739553527));
#35366=CARTESIAN_POINT('Ctrl Pts',(37.4043107963977,3.25889279038126,5.6127846874694));
#35367=CARTESIAN_POINT('Ctrl Pts',(37.5035665986187,0.179650915968158,6.46916266085227));
#35368=CARTESIAN_POINT('Ctrl Pts',(37.6359076682469,-4.00324642534526,5.56759497029643));
#35369=CARTESIAN_POINT('Ctrl Pts',(37.7418736626271,-6.12426506880607,2.48148226091111));
#35370=CARTESIAN_POINT('Ctrl Pts',(37.8147543896004,-6.22848043592516,0.214617655518784));
#35371=CARTESIAN_POINT('Ctrl Pts',(37.8214645817596,-6.22702764812334,0.00572193935648436));
#35372=CARTESIAN_POINT('Origin',(28.1999754182402,0.,0.));
#35373=CARTESIAN_POINT('',(35.0749754182404,-6.21859864471026,0.00324434653253106));
#35374=CARTESIAN_POINT('',(35.3214645817596,-6.210630471212,-0.000241035779820487));
#35375=CARTESIAN_POINT('',(28.1999754182402,-6.21925,5.68729293530136E-12));
#35376=CARTESIAN_POINT('Ctrl Pts',(35.0749754182404,-6.21859864471025,0.00324434653253113));
#35377=CARTESIAN_POINT('Ctrl Pts',(35.095479575848,-6.21654040868293,-0.636816772095382));
#35378=CARTESIAN_POINT('Ctrl Pts',(35.1490690008627,-5.95386142902179,-2.31247659416935));
#35379=CARTESIAN_POINT('Ctrl Pts',(35.2688289606914,-3.93449142709178,-5.61639323287909));
#35380=CARTESIAN_POINT('Ctrl Pts',(35.4342552977265,1.706159430506,-7.15206323045347));
#35381=CARTESIAN_POINT('Ctrl Pts',(35.6327669021685,6.93766837888352,-2.43496237142141));
#35382=CARTESIAN_POINT('Ctrl Pts',(35.8312785066107,5.80973766223456,4.50635469098045));
#35383=CARTESIAN_POINT('Ctrl Pts',(36.0297901110528,-0.646180895956555,
7.3243046569134));
#35384=CARTESIAN_POINT('Ctrl Pts',(36.1943557482627,-5.48506849708825,4.09851879072839));
#35385=CARTESIAN_POINT('Ctrl Pts',(36.2927508506585,-6.21822602067945,1.00850704118591));
#35386=CARTESIAN_POINT('Ctrl Pts',(36.3249754182403,-6.2162013314378,-0.00113763775599949));
#35387=CARTESIAN_POINT('Ctrl Pts',(35.3214645817596,-6.210630471212,-0.00024103577982007));
#35388=CARTESIAN_POINT('Ctrl Pts',(35.3540413051653,-6.21100194781226,-1.02236541662845));
#35389=CARTESIAN_POINT('Ctrl Pts',(35.452788563385,-5.48716606870768,-4.12015825613875));
#35390=CARTESIAN_POINT('Ctrl Pts',(35.6177063564187,-0.593159681851761,
-7.32878912572931));
#35391=CARTESIAN_POINT('Ctrl Pts',(35.7831326934538,4.74656140271064,-4.94916665150982));
#35392=CARTESIAN_POINT('Ctrl Pts',(35.9154737630819,6.39392461916095,-1.00003397421454));
#35393=CARTESIAN_POINT('Ctrl Pts',(36.0147295653029,6.1119213231936,2.18360983365812));
#35394=CARTESIAN_POINT('Ctrl Pts',(36.1139853675239,4.31273644099712,4.82520925710656));
#35395=CARTESIAN_POINT('Ctrl Pts',(36.2463264371521,0.535911013730674,6.83643877180359));
#35396=CARTESIAN_POINT('Ctrl Pts',(36.3988195085639,-4.66198719373343,5.41438603443864));
#35397=CARTESIAN_POINT('Ctrl Pts',(36.5182273125688,-6.20488362084988,1.65802905264626));
#35398=CARTESIAN_POINT('Ctrl Pts',(36.5714645817597,-6.2210655398886,-0.0052865996581393));
#35399=CARTESIAN_POINT('Origin',(28.1999754182402,0.,0.));
#35400=CARTESIAN_POINT('',(33.8249754182404,-6.22651516743638,-0.00167075726269435));
#35401=CARTESIAN_POINT('',(34.0714645817596,-6.22005335440933,0.0053417081121826));
#35402=CARTESIAN_POINT('',(28.1999754182402,-6.21925,5.68729293530136E-12));
#35403=CARTESIAN_POINT('Ctrl Pts',(33.8249754182403,-6.22651516743638,-0.0016707572626945));
#35404=CARTESIAN_POINT('Ctrl Pts',(33.8320377662234,-6.22722193989077,-0.222213824936918));
#35405=CARTESIAN_POINT('Ctrl Pts',(33.9052706490206,-6.10845944272299,-2.50753618971029));
#35406=CARTESIAN_POINT('Ctrl Pts',(34.0446740666317,-3.31312753510712,-6.56400641995886));
#35407=CARTESIAN_POINT('Ctrl Pts',(34.2431856710738,3.72736559794809,-6.33774649263565));
#35408=CARTESIAN_POINT('Ctrl Pts',(34.4416972755159,7.34611894960073,-0.307926448941118));
#35409=CARTESIAN_POINT('Ctrl Pts',(34.640208879958,4.233914906245,6.01140200914276));
#35410=CARTESIAN_POINT('Ctrl Pts',(34.8056352169931,-1.57434350116745,6.67424438783693));
#35411=CARTESIAN_POINT('Ctrl Pts',(34.9379762866212,-4.99945699673356,4.10947315312662));
#35412=CARTESIAN_POINT('Ctrl Pts',(35.0167279312346,-6.08991113296614,1.82004144531782));
#35413=CARTESIAN_POINT('Ctrl Pts',(35.062394308441,-6.21986155411372,0.395978316191532));
#35414=CARTESIAN_POINT('Ctrl Pts',(35.0749754182404,-6.21859864471025,0.00324434653253113));
#35415=CARTESIAN_POINT('Ctrl Pts',(34.0714645817596,-6.22005335440933,0.00534170811218225));
#35416=CARTESIAN_POINT('Ctrl Pts',(34.1236847629477,-6.20409670026243,-1.62686967844328));
#35417=CARTESIAN_POINT('Ctrl Pts',(34.2420754789499,-4.70995884997351,-5.35226492593367));
#35418=CARTESIAN_POINT('Ctrl Pts',(34.393551462359,0.430999447686097,-6.84385381815942));
#35419=CARTESIAN_POINT('Ctrl Pts',(34.5258925319871,4.23822627631683,-4.89078499723656));
#35420=CARTESIAN_POINT('Ctrl Pts',(34.6251483342081,6.07771306114946,-2.27708986044939));
#35421=CARTESIAN_POINT('Ctrl Pts',(34.7244041364292,6.40850984162318,0.901854494708191));
#35422=CARTESIAN_POINT('Ctrl Pts',(34.8567452060572,4.82190714720603,4.87578785427672));
#35423=CARTESIAN_POINT('Ctrl Pts',(35.0221715430924,-0.48069030065227,7.33702428029021));
#35424=CARTESIAN_POINT('Ctrl Pts',(35.1881064241288,-5.45381342879383,4.1845056440569));
#35425=CARTESIAN_POINT('Ctrl Pts',(35.2878707703512,-6.2102473966254,1.05379540792869));
#35426=CARTESIAN_POINT('Ctrl Pts',(35.3214645817596,-6.210630471212,-0.00024103577982007));
#35427=CARTESIAN_POINT('Origin',(28.1999754182402,0.,0.));
#35428=CARTESIAN_POINT('',(32.5749754182403,-6.21844556314562,-0.000466044233505376));
#35429=CARTESIAN_POINT('',(32.8214645817597,-6.22773255198024,-0.00518142285415191));
#35430=CARTESIAN_POINT('',(28.1999754182402,-6.21925,5.68729293530136E-12));
#35431=CARTESIAN_POINT('Ctrl Pts',(32.5749754182403,-6.20937279635969,-0.00572228109726187));
#35432=CARTESIAN_POINT('Ctrl Pts',(32.6016812240059,-6.21396328164207,-0.84203719014262));
#35433=CARTESIAN_POINT('Ctrl Pts',(32.6945575645854,-5.66911297578352,-3.74417462738773));
#35434=CARTESIAN_POINT('Ctrl Pts',(32.853604439979,-1.24379023624101,-7.2466418339485));
#35435=CARTESIAN_POINT('Ctrl Pts',(33.0521160444211,5.41227178463782,-4.97673046693937));
#35436=CARTESIAN_POINT('Ctrl Pts',(33.2506276488633,7.11391162562153,1.85873863792625));
#35437=CARTESIAN_POINT('Ctrl Pts',(33.4160539858983,3.10541110519021,6.11397050225541));
#35438=CARTESIAN_POINT('Ctrl Pts',(33.5483950555264,-1.16614656773419,6.36572295470293));
#35439=CARTESIAN_POINT('Ctrl Pts',(33.6476508577475,-4.07834394078075,5.04884480068));
#35440=CARTESIAN_POINT('Ctrl Pts',(33.7398443119854,-5.84299343888296,2.66154714325195));
#35441=CARTESIAN_POINT('Ctrl Pts',(33.7989524988164,-6.22391089437088,0.810973209496164));
#35442=CARTESIAN_POINT('Ctrl Pts',(33.8249754182403,-6.22651516743638,-0.0016707572626945));
#35443=CARTESIAN_POINT('Ctrl Pts',(32.8214645817597,-6.22773255198024,-0.00518142285415288));
#35444=CARTESIAN_POINT('Ctrl Pts',(32.8271576859162,-6.22883195533547,-0.182350455011576));
#35445=CARTESIAN_POINT('Ctrl Pts',(32.8990213248867,-6.14169081306461,-2.41719204780253));
#35446=CARTESIAN_POINT('Ctrl Pts',(33.0039702312642,-4.08817544863011,-5.50554583451141));
#35447=CARTESIAN_POINT('Ctrl Pts',(33.1363113008923,0.0804192017098835,
-6.47115594816462));
#35448=CARTESIAN_POINT('Ctrl Pts',(33.2355671031134,3.17242495854284,-5.66210588059523));
#35449=CARTESIAN_POINT('Ctrl Pts',(33.3348229053343,5.47694100310651,-3.44753091698999));
#35450=CARTESIAN_POINT('Ctrl Pts',(33.4671639749625,6.83006089629673,0.611842341327977));
#35451=CARTESIAN_POINT('Ctrl Pts',(33.6325903119975,4.36852741272638,5.91430153013899));
#35452=CARTESIAN_POINT('Ctrl Pts',(33.8311019164398,-2.60995361271077,6.87374912585412));
#35453=CARTESIAN_POINT('Ctrl Pts',(33.9773933396937,-5.98521297716978,2.94115569332543));
#35454=CARTESIAN_POINT('Ctrl Pts',(34.0575142281337,-6.22431609274099,0.441378610258281));
#35455=CARTESIAN_POINT('Ctrl Pts',(34.0714645817596,-6.22005335440933,0.00534170811218225));
#35456=CARTESIAN_POINT('Origin',(28.1999754182402,0.,0.));
#35457=CARTESIAN_POINT('',(31.3249754182403,-6.21925,7.0933178088184E-13));
#35458=CARTESIAN_POINT('',(31.5714645817597,-6.20816386984268,-0.000295703980951467));
#35459=CARTESIAN_POINT('',(28.1999754182402,-6.21925,5.68729293530136E-12));
#35460=CARTESIAN_POINT('Ctrl Pts',(31.3249754182403,-6.21925,6.65141351788081E-13));
#35461=CARTESIAN_POINT('Ctrl Pts',(31.383775169714,-6.2192500000002,-1.83816020915679));
#35462=CARTESIAN_POINT('Ctrl Pts',(31.4425749211877,-5.35502977485053,-3.65808141345899));
#35463=CARTESIAN_POINT('Ctrl Pts',(31.5013746726614,-3.93049712175878,-4.81977830800815));
#35464=CARTESIAN_POINT('Ctrl Pts',(31.5601744241351,-2.50596446866704,-5.98147520255732));
#35465=CARTESIAN_POINT('Ctrl Pts',(31.6189741756088,-0.549389021419119,
-6.46189408921052));
#35466=CARTESIAN_POINT('Ctrl Pts',(31.6777739270825,1.25118869866879,-6.09209302315908));
#35467=CARTESIAN_POINT('Ctrl Pts',(31.7365736785562,3.05176641875671,-5.72229195710763));
#35468=CARTESIAN_POINT('Ctrl Pts',(31.7953734300299,4.66061422075206,-4.50960958424933));
#35469=CARTESIAN_POINT('Ctrl Pts',(31.8541731815036,5.51197192302716,-2.88049233331045));
#35470=CARTESIAN_POINT('Ctrl Pts',(31.9129729329773,6.36332962530225,-1.25137508237158));
#35471=CARTESIAN_POINT('Ctrl Pts',(31.971772684451,6.44030216377282,0.761847462641246));
#35472=CARTESIAN_POINT('Ctrl Pts',(32.0305724359247,5.71582172177439,2.45121451680429));
#35473=CARTESIAN_POINT('Ctrl Pts',(32.0893721873984,4.99134127977595,4.14058157096734));
#35474=CARTESIAN_POINT('Ctrl Pts',(32.1481719388721,3.47978506146448,5.47256790209481));
#35475=CARTESIAN_POINT('Ctrl Pts',(32.2069716903458,1.71270012775633,5.97877318811171));
#35476=CARTESIAN_POINT('Ctrl Pts',(32.2657714418195,-0.0543848059518154,
6.4849784741286));
#35477=CARTESIAN_POINT('Ctrl Pts',(32.3245711932932,-2.04193092337452,6.15535714814312));
#35478=CARTESIAN_POINT('Ctrl Pts',(32.3833709447669,-3.55100669662464,5.10582236305054));
#35479=CARTESIAN_POINT('Ctrl Pts',(32.4421706962406,-5.06008246987476,4.05628757795795));
#35480=CARTESIAN_POINT('Ctrl Pts',(32.5009704477143,-6.06074051980842,2.30766719190228));
#35481=CARTESIAN_POINT('Ctrl Pts',(32.559770199188,-6.20109393743675,0.474873184740044));
#35482=CARTESIAN_POINT('Ctrl Pts',(32.5648386055388,-6.21319208641581,0.316890462828053));
#35483=CARTESIAN_POINT('Ctrl Pts',(32.5699070118896,-6.21924999999998,0.158445276457369));
#35484=CARTESIAN_POINT('Ctrl Pts',(32.5749754182403,-6.21925,6.666646287092E-13));
#35485=CARTESIAN_POINT('Ctrl Pts',(31.5714645817597,-6.20816386984268,-0.000295703980950981));
#35486=CARTESIAN_POINT('Ctrl Pts',(31.5968011436986,-6.21130704176283,-0.794297582896872));
#35487=CARTESIAN_POINT('Ctrl Pts',(31.6552229730446,-5.88436859534305,-2.6238606368355));
#35488=CARTESIAN_POINT('Ctrl Pts',(31.7467300697975,-4.11675109351076,-4.99488165618313));
#35489=CARTESIAN_POINT('Ctrl Pts',(31.8459858720185,-1.23075458232488,-6.37221708890274));
#35490=CARTESIAN_POINT('Ctrl Pts',(31.9452416742396,1.95775582174799,-6.16839483200312));
#35491=CARTESIAN_POINT('Ctrl Pts',(32.0775827438677,5.61197648499354,-3.94108216408908));
#35492=CARTESIAN_POINT('Ctrl Pts',(32.2430090809028,7.15393902550158,1.69766694268016));
#35493=CARTESIAN_POINT('Ctrl Pts',(32.4415206853449,2.4432388603139,6.93479746587837));
#35494=CARTESIAN_POINT('Ctrl Pts',(32.6343391856305,-4.30040480542789,5.84717018705371));
#35495=CARTESIAN_POINT('Ctrl Pts',(32.7609871511021,-6.21605367023959,1.87687229730388));
#35496=CARTESIAN_POINT('Ctrl Pts',(32.8214645817597,-6.22773255198024,-0.00518142285415288));
#35497=CARTESIAN_POINT('Origin',(-8.,0.,2.1));
#35498=CARTESIAN_POINT('',(0.,-9.,2.1));
#35499=CARTESIAN_POINT('',(-16.,9.,2.1));
#35500=CARTESIAN_POINT('Origin',(-16.,9.,0.));
#35501=CARTESIAN_POINT('',(-16.,9.,-2.1));
#35502=CARTESIAN_POINT('Origin',(-8.,0.,-2.1));
#35503=CARTESIAN_POINT('',(0.,-9.,-2.1));
#35504=CARTESIAN_POINT('Origin',(0.,-9.,0.));
#35505=CARTESIAN_POINT('Origin',(109.067,1.12618006296016E-15,0.));
#35506=CARTESIAN_POINT('',(109.067,6.85892174064777,1.01078264511681));
#35507=CARTESIAN_POINT('Ctrl Pts',(109.067,-2.15756780909041,-5.83789702209075));
#35508=CARTESIAN_POINT('Ctrl Pts',(109.067,-2.0135726607274,-5.9015965205511));
#35509=CARTESIAN_POINT('Ctrl Pts',(109.067,-1.86728073205768,-5.95949577427964));
#35510=CARTESIAN_POINT('Ctrl Pts',(109.067,-1.71893720698406,-6.01134642449991));
#35511=CARTESIAN_POINT('Ctrl Pts',(109.067,-1.55748216789094,-6.06777995440398));
#35512=CARTESIAN_POINT('Ctrl Pts',(109.067,-1.39359690962913,-6.11704974662805));
#35513=CARTESIAN_POINT('Ctrl Pts',(109.067,-1.22777124491188,-6.15927407685968));
#35514=CARTESIAN_POINT('Ctrl Pts',(109.067,-1.12095704707141,-6.18647226702362));
#35515=CARTESIAN_POINT('Ctrl Pts',(109.067,-1.01333719076962,-6.21074625738224));
#35516=CARTESIAN_POINT('Ctrl Pts',(109.067,-0.905038201094559,-6.2321171997402));
#35517=CARTESIAN_POINT('Ctrl Pts',(109.067,-0.842383954466684,-6.24448093736308));
#35518=CARTESIAN_POINT('Ctrl Pts',(109.067,-0.779502349592861,-6.25587288063033));
#35519=CARTESIAN_POINT('Ctrl Pts',(109.067,-0.716417544951752,-6.26629587236679));
#35520=CARTESIAN_POINT('Ctrl Pts',(109.067,-0.682837053570036,-6.2718441051967));
#35521=CARTESIAN_POINT('Ctrl Pts',(109.067,-0.64919898185994,-6.27711776920991));
#35522=CARTESIAN_POINT('Ctrl Pts',(109.067,-0.615506954172322,-6.28211718696264));
#35523=CARTESIAN_POINT('Ctrl Pts',(109.067,-0.590641187520192,-6.28580691310166));
#35524=CARTESIAN_POINT('Ctrl Pts',(109.067,-0.565749932528012,-6.28934664569366));
#35525=CARTESIAN_POINT('Ctrl Pts',(109.067,-0.540842974343021,-6.29273560102282));
#35526=CARTESIAN_POINT('Ctrl Pts',(109.067,-0.366963296689134,-6.31639446999596));
#35527=CARTESIAN_POINT('Ctrl Pts',(109.067,-0.192199995525417,-6.3327270073782));
#35528=CARTESIAN_POINT('Ctrl Pts',(109.067,-0.0170658993305209,-6.34185755124692));
#35529=CARTESIAN_POINT('Ctrl Pts',(109.067,0.159767917302458,-6.35107670933961));
#35530=CARTESIAN_POINT('Ctrl Pts',(109.067,0.336980514165373,-6.35295346928648));
#35531=CARTESIAN_POINT('Ctrl Pts',(109.067,0.514059064472075,-6.34756433866805));
#35532=CARTESIAN_POINT('Ctrl Pts',(109.067,0.663134169149158,-6.34302745258179));
#35533=CARTESIAN_POINT('Ctrl Pts',(109.067,0.812114778451582,-6.33334015175942));
#35534=CARTESIAN_POINT('Ctrl Pts',(109.067,0.960697048025707,-6.3185197289033));
#35535=CARTESIAN_POINT('Ctrl Pts',(109.067,0.986307215777789,-6.31596522817728));
#35536=CARTESIAN_POINT('Ctrl Pts',(109.067,1.01190554605928,-6.31325816427479));
#35537=CARTESIAN_POINT('Ctrl Pts',(109.067,1.03749047650535,-6.31039854793851));
#35538=CARTESIAN_POINT('Ctrl Pts',(109.067,1.06164020100599,-6.30769934393465));
#35539=CARTESIAN_POINT('Ctrl Pts',(109.067,1.08576977624899,-6.30486512412045));
#35540=CARTESIAN_POINT('Ctrl Pts',(109.067,1.10987372754823,-6.30189671902766));
#35541=CARTESIAN_POINT('Ctrl Pts',(109.067,1.20838784565032,-6.28976469111842));
#35542=CARTESIAN_POINT('Ctrl Pts',(109.067,1.30649618888237,-6.2753891231948));
#35543=CARTESIAN_POINT('Ctrl Pts',(109.067,1.40411036563822,-6.25879202047389));
#35544=CARTESIAN_POINT('Ctrl Pts',(109.067,1.57975009016904,-6.22892842230823));
#35545=CARTESIAN_POINT('Ctrl Pts',(109.067,1.75378995004789,-6.19187556201615));
#35546=CARTESIAN_POINT('Ctrl Pts',(109.067,1.9258564963741,-6.14786245476911));
#35547=CARTESIAN_POINT('Ctrl Pts',(109.067,2.09942770353434,-6.10346446853151));
#35548=CARTESIAN_POINT('Ctrl Pts',(109.067,2.27099158455466,-6.05198385933624));
#35549=CARTESIAN_POINT('Ctrl Pts',(109.067,2.44016284904198,-5.99360265655463));
#35550=CARTESIAN_POINT('Ctrl Pts',(109.067,2.61121284388512,-5.93457310171272));
#35551=CARTESIAN_POINT('Ctrl Pts',(109.067,2.7798174976817,-5.86848873919628));
#35552=CARTESIAN_POINT('Ctrl Pts',(109.067,2.94556620576367,-5.79548528379882));
#35553=CARTESIAN_POINT('Ctrl Pts',(109.067,3.06987773682515,-5.74073269225073));
#35554=CARTESIAN_POINT('Ctrl Pts',(109.067,3.1925826133881,-5.68208701342321));
#35555=CARTESIAN_POINT('Ctrl Pts',(109.067,3.31349941504197,-5.6195869992619));
#35556=CARTESIAN_POINT('Ctrl Pts',(109.067,3.34663878643761,-5.60245777360265));
#35557=CARTESIAN_POINT('Ctrl Pts',(109.067,3.37964379966736,-5.58503894784604));
#35558=CARTESIAN_POINT('Ctrl Pts',(109.067,3.4125105980543,-5.56733111927243));
#35559=CARTESIAN_POINT('Ctrl Pts',(109.067,3.43139568280936,-5.55715629665954));
#35560=CARTESIAN_POINT('Ctrl Pts',(109.067,3.45023242661829,-5.54688747547546));
#35561=CARTESIAN_POINT('Ctrl Pts',(109.067,3.46901112922455,-5.53652991792905));
#35562=CARTESIAN_POINT('Ctrl Pts',(109.067,3.62877163156698,-5.44841261657179));
#35563=CARTESIAN_POINT('Ctrl Pts',(109.067,3.78452202689656,-5.35377495289507));
#35564=CARTESIAN_POINT('Ctrl Pts',(109.067,3.93587605353499,-5.25282511603666));
#35565=CARTESIAN_POINT('Ctrl Pts',(109.067,4.07468561123279,-5.16024216654266));
#35566=CARTESIAN_POINT('Ctrl Pts',(109.067,4.20979769549856,-5.06234929407872));
#35567=CARTESIAN_POINT('Ctrl Pts',(109.067,4.34090372720216,-4.95927004899439));
#35568=CARTESIAN_POINT('Ctrl Pts',(109.067,4.48236568874247,-4.84804868095934));
#35569=CARTESIAN_POINT('Ctrl Pts',(109.067,4.61916464818014,-4.73078973445163));
#35570=CARTESIAN_POINT('Ctrl Pts',(109.067,4.75105064478682,-4.60792710833882));
#35571=CARTESIAN_POINT('Ctrl Pts',(109.067,4.88388391613822,-4.4841820180844));
#35572=CARTESIAN_POINT('Ctrl Pts',(109.067,5.01173392221482,-4.35475193857044));
#35573=CARTESIAN_POINT('Ctrl Pts',(109.067,5.13431262660541,-4.22003860820336));
#35574=CARTESIAN_POINT('Ctrl Pts',(109.067,5.19748221283924,-4.15061557602353));
#35575=CARTESIAN_POINT('Ctrl Pts',(109.067,5.25925129919297,-4.07978882346575));
#35576=CARTESIAN_POINT('Ctrl Pts',(109.067,5.31957640477001,-4.0076097744433));
#35577=CARTESIAN_POINT('Ctrl Pts',(109.067,5.33808213817268,-3.98546764595979));
#35578=CARTESIAN_POINT('Ctrl Pts',(109.067,5.35645196334427,-3.96319824319762));
#35579=CARTESIAN_POINT('Ctrl Pts',(109.067,5.3746845673014,-3.94080301147104));
#35580=CARTESIAN_POINT('Ctrl Pts',(109.067,5.38726994465937,-3.92534430667161));
#35581=CARTESIAN_POINT('Ctrl Pts',(109.067,5.39978828430919,-3.90982764047081));
#35582=CARTESIAN_POINT('Ctrl Pts',(109.067,5.41223383221326,-3.89426036487904));
#35583=CARTESIAN_POINT('Ctrl Pts',(109.067,5.52700188467733,-3.750704941236));
#35584=CARTESIAN_POINT('Ctrl Pts',(109.067,5.6357169848108,-3.60268437046879));
#35585=CARTESIAN_POINT('Ctrl Pts',(109.067,5.73814962803564,-3.45067190929303));
#35586=CARTESIAN_POINT('Ctrl Pts',(109.067,5.84145552549992,-3.29736351820676));
#35587=CARTESIAN_POINT('Ctrl Pts',(109.067,5.93837191258434,-3.13999433806236));
#35588=CARTESIAN_POINT('Ctrl Pts',(109.067,6.02863118663199,-2.97900751654019));
#35589=CARTESIAN_POINT('Ctrl Pts',(109.067,6.11884425326949,-2.81810311074946));
#35590=CARTESIAN_POINT('Ctrl Pts',(109.067,6.20240750924262,-2.65358415770578));
#35591=CARTESIAN_POINT('Ctrl Pts',(109.067,6.27901423903501,-2.48585980888858));
#35592=CARTESIAN_POINT('Ctrl Pts',(109.067,6.30202101264031,-2.43548830586537));
#35593=CARTESIAN_POINT('Ctrl Pts',(109.067,6.32440005144439,-2.38482750170827));
#35594=CARTESIAN_POINT('Ctrl Pts',(109.067,6.34614224786266,-2.33388801902908));
#35595=CARTESIAN_POINT('Ctrl Pts',(109.067,6.40204411734148,-2.20291632429923));
#35596=CARTESIAN_POINT('Ctrl Pts',(109.067,6.45373726838296,-2.07010281771283));
#35597=CARTESIAN_POINT('Ctrl Pts',(109.067,6.5011990215905,-1.93564346445603));
#35598=CARTESIAN_POINT('Ctrl Pts',(109.067,6.5219635386188,-1.87681749740618));
#35599=CARTESIAN_POINT('Ctrl Pts',(109.067,6.54191791372575,-1.81767642326058));
#35600=CARTESIAN_POINT('Ctrl Pts',(109.067,6.56105917890401,-1.75823633122607));
#35601=CARTESIAN_POINT('Ctrl Pts',(109.067,6.57150884537305,-1.72578658817798));
#35602=CARTESIAN_POINT('Ctrl Pts',(109.067,6.58171616720908,-1.69324772523769));
#35603=CARTESIAN_POINT('Ctrl Pts',(109.067,6.59168057800658,-1.66062234252173));
#35604=CARTESIAN_POINT('Ctrl Pts',(109.067,6.59948481623486,-1.63506977707871));
#35605=CARTESIAN_POINT('Ctrl Pts',(109.067,6.6071405710643,-1.60946211965833));
#35606=CARTESIAN_POINT('Ctrl Pts',(109.067,6.61464142664228,-1.58382220961391));
#35607=CARTESIAN_POINT('Ctrl Pts',(109.067,6.66647256761742,-1.40664964865927));
#35608=CARTESIAN_POINT('Ctrl Pts',(109.067,6.71098048972246,-1.22771717878011));
#35609=CARTESIAN_POINT('Ctrl Pts',(109.067,6.74821024821888,-1.04748636093756));
#35610=CARTESIAN_POINT('Ctrl Pts',(109.067,6.78607258251663,-0.8641932171862));
#35611=CARTESIAN_POINT('Ctrl Pts',(109.067,6.81640757241096,-0.679556633939157));
#35612=CARTESIAN_POINT('Ctrl Pts',(109.067,6.83921525633307,-0.494036516019991));
#35613=CARTESIAN_POINT('Ctrl Pts',(109.067,6.8620662536148,-0.308164082643737));
#35614=CARTESIAN_POINT('Ctrl Pts',(109.067,6.87736147631527,-0.121404073567072));
#35615=CARTESIAN_POINT('Ctrl Pts',(109.067,6.88505100358449,0.0657966891430848));
#35616=CARTESIAN_POINT('Ctrl Pts',(109.067,6.89266799101194,0.251231476750997));
#35617=CARTESIAN_POINT('Ctrl Pts',(109.067,6.89282216605126,0.437099421891961));
#35618=CARTESIAN_POINT('Ctrl Pts',(109.067,6.88541461247308,0.62297144031264));
#35619=CARTESIAN_POINT('Ctrl Pts',(109.067,6.88026095061278,0.752288295347639));
#35620=CARTESIAN_POINT('Ctrl Pts',(109.067,6.87144606107714,0.881607238796431));
#35621=CARTESIAN_POINT('Ctrl Pts',(109.067,6.85892174064777,1.01078264511681));
#35622=CARTESIAN_POINT('',(109.067,-6.933,-8.4904762584886E-16));
#35623=CARTESIAN_POINT('Origin',(109.067,0.,0.));
#35624=CARTESIAN_POINT('',(109.067,3.46348981423002,6.00884185984444));
#35625=CARTESIAN_POINT('Origin',(109.067,0.,0.));
#35626=CARTESIAN_POINT('Ctrl Pts',(109.067,3.46405146923353,6.01146880811302));
#35627=CARTESIAN_POINT('Ctrl Pts',(109.067,3.30912874255884,6.09212153599444));
#35628=CARTESIAN_POINT('Ctrl Pts',(109.067,3.1512484438972,6.16654224984595));
#35629=CARTESIAN_POINT('Ctrl Pts',(109.067,2.99061701977446,6.23440908312552));
#35630=CARTESIAN_POINT('Ctrl Pts',(109.067,2.81845433699699,6.30714787724899));
#35631=CARTESIAN_POINT('Ctrl Pts',(109.067,2.64313094670355,6.37235874611403));
#35632=CARTESIAN_POINT('Ctrl Pts',(109.067,2.46518012087715,6.43006589265));
#35633=CARTESIAN_POINT('Ctrl Pts',(109.067,2.35251751740855,6.4666009148242));
#35634=CARTESIAN_POINT('Ctrl Pts',(109.067,2.23880142696933,6.50012719452215));
#35635=CARTESIAN_POINT('Ctrl Pts',(109.067,2.1241655087431,6.53064026904539));
#35636=CARTESIAN_POINT('Ctrl Pts',(109.067,2.06495123148562,6.54640155645648));
#35637=CARTESIAN_POINT('Ctrl Pts',(109.067,2.00549151947031,6.56135873964514));
#35638=CARTESIAN_POINT('Ctrl Pts',(109.067,1.94580478784761,6.57551034809967));
#35639=CARTESIAN_POINT('Ctrl Pts',(109.067,1.90531981645002,6.58510925639864));
#35640=CARTESIAN_POINT('Ctrl Pts',(109.067,1.86473039837682,6.59433752490925));
#35641=CARTESIAN_POINT('Ctrl Pts',(109.067,1.82404229299711,6.60319454242566));
#35642=CARTESIAN_POINT('Ctrl Pts',(109.067,1.79431097931758,6.6096664772476));
#35643=CARTESIAN_POINT('Ctrl Pts',(109.067,1.76452539060412,6.61594044050794));
#35644=CARTESIAN_POINT('Ctrl Pts',(109.067,1.7347064700501,6.62201254137047));
#35645=CARTESIAN_POINT('Ctrl Pts',(109.067,1.55155509466467,6.65930811088765));
#35646=CARTESIAN_POINT('Ctrl Pts',(109.067,1.36699117500837,6.68902756324626));
#35647=CARTESIAN_POINT('Ctrl Pts',(109.067,1.18154536859613,6.71119870068649));
#35648=CARTESIAN_POINT('Ctrl Pts',(109.067,0.996051600557548,6.73337557222138));
#35649=CARTESIAN_POINT('Ctrl Pts',(109.067,0.809674689036533,6.74800018653563));
#35650=CARTESIAN_POINT('Ctrl Pts',(109.067,0.622944059228044,6.75504829234912));
#35651=CARTESIAN_POINT('Ctrl Pts',(109.067,0.460793212061621,6.76116863977015));
#35652=CARTESIAN_POINT('Ctrl Pts',(109.067,0.298375303328641,6.76157501218272));
#35653=CARTESIAN_POINT('Ctrl Pts',(109.067,0.136043018085803,6.75621996754557));
#35654=CARTESIAN_POINT('Ctrl Pts',(109.067,0.105092913226025,6.75519898029832));
#35655=CARTESIAN_POINT('Ctrl Pts',(109.067,0.074145947935451,6.75396847540538));
#35656=CARTESIAN_POINT('Ctrl Pts',(109.067,0.0432046090642379,6.75252800360357));
#35657=CARTESIAN_POINT('Ctrl Pts',(109.067,0.020305459140885,6.75146193532879));
#35658=CARTESIAN_POINT('Ctrl Pts',(109.067,-0.00258678730564892,6.75028101279484));
#35659=CARTESIAN_POINT('Ctrl Pts',(109.067,-0.0254628612165071,6.74898570654463));
#35660=CARTESIAN_POINT('Ctrl Pts',(109.067,-0.133799396937078,6.74285139379534));
#35661=CARTESIAN_POINT('Ctrl Pts',(109.067,-0.241828769116266,6.73414967973701));
#35662=CARTESIAN_POINT('Ctrl Pts',(109.067,-0.349448736226522,6.72288662725207));
#35663=CARTESIAN_POINT('Ctrl Pts',(109.067,-0.532719427466918,6.70370628860471));
#35664=CARTESIAN_POINT('Ctrl Pts',(109.067,-0.71480348606703,6.6771008732754));
#35665=CARTESIAN_POINT('Ctrl Pts',(109.067,-0.895302658472974,6.64322184101536));
#35666=CARTESIAN_POINT('Ctrl Pts',(109.067,-1.07613522511967,6.60928023187983));
#35667=CARTESIAN_POINT('Ctrl Pts',(109.067,-1.25537769913326,6.56803789023454));
#35668=CARTESIAN_POINT('Ctrl Pts',(109.067,-1.43261590046417,6.51959676567458));
#35669=CARTESIAN_POINT('Ctrl Pts',(109.067,-1.6104255942165,6.4709994460316));
#35670=CARTESIAN_POINT('Ctrl Pts',(109.067,-1.78621873701221,6.41515664486632));
#35671=CARTESIAN_POINT('Ctrl Pts',(109.067,-1.95955339481228,6.35212381902113));
#35672=CARTESIAN_POINT('Ctrl Pts',(109.067,-2.08955438816234,6.30484919963723));
#35673=CARTESIAN_POINT('Ctrl Pts',(109.067,-2.21817205794986,6.25352919760746));
#35674=CARTESIAN_POINT('Ctrl Pts',(109.067,-2.34520781399991,6.19817078339132));
#35675=CARTESIAN_POINT('Ctrl Pts',(109.067,-2.38702415979058,6.17994846029692));
#35676=CARTESIAN_POINT('Ctrl Pts',(109.067,-2.42866900487268,6.16128845441856));
#35677=CARTESIAN_POINT('Ctrl Pts',(109.067,-2.47013496906611,6.14219069678272));
#35678=CARTESIAN_POINT('Ctrl Pts',(109.067,-2.49201710721469,6.13211255730026));
#35679=CARTESIAN_POINT('Ctrl Pts',(109.067,-2.51384261560681,6.12191561532782));
#35680=CARTESIAN_POINT('Ctrl Pts',(109.067,-2.53560342805358,6.11160351080748));
#35681=CARTESIAN_POINT('Ctrl Pts',(109.067,-2.69890086127494,6.03421944238624));
#35682=CARTESIAN_POINT('Ctrl Pts',(109.067,-2.85868286445364,5.95029614110067));
#35683=CARTESIAN_POINT('Ctrl Pts',(109.067,-3.01456652439573,5.8599486944075));
#35684=CARTESIAN_POINT('Ctrl Pts',(109.067,-3.15730235684114,5.77722149889608));
#35685=CARTESIAN_POINT('Ctrl Pts',(109.067,-3.29676987486409,5.68910744517844));
#35686=CARTESIAN_POINT('Ctrl Pts',(109.067,-3.43265613191939,5.59566156792999));
#35687=CARTESIAN_POINT('Ctrl Pts',(109.067,-3.58145554886069,5.49333560538265));
#35688=CARTESIAN_POINT('Ctrl Pts',(109.067,-3.72596163392383,5.38461635190157));
#35689=CARTESIAN_POINT('Ctrl Pts',(109.067,-3.86583639657926,5.26988938971029));
#35690=CARTESIAN_POINT('Ctrl Pts',(109.067,-4.00522968928239,5.15555733496311));
#35691=CARTESIAN_POINT('Ctrl Pts',(109.067,-4.1400239540109,5.03525822345385));
#35692=CARTESIAN_POINT('Ctrl Pts',(109.067,-4.26984353036136,4.90934272162992));
#35693=CARTESIAN_POINT('Ctrl Pts',(109.067,-4.33436650584876,4.84676015075681));
#35694=CARTESIAN_POINT('Ctrl Pts',(109.067,-4.39765990532932,4.78278974609324));
#35695=CARTESIAN_POINT('Ctrl Pts',(109.067,-4.45967325628869,4.71747243917582));
#35696=CARTESIAN_POINT('Ctrl Pts',(109.067,-4.477009225061,4.69921284224235));
#35697=CARTESIAN_POINT('Ctrl Pts',(109.067,-4.49424514026326,4.6808479786264));
#35698=CARTESIAN_POINT('Ctrl Pts',(109.067,-4.51137985542899,4.66237872705053));
#35699=CARTESIAN_POINT('Ctrl Pts',(109.067,-4.52593111622634,4.64669414205375));
#35700=CARTESIAN_POINT('Ctrl Pts',(109.067,-4.54040839081441,4.63093529486271));
#35701=CARTESIAN_POINT('Ctrl Pts',(109.067,-4.55480284574971,4.61511188698257));
#35702=CARTESIAN_POINT('Ctrl Pts',(109.067,-4.67524484062003,4.48271348639725));
#35703=CARTESIAN_POINT('Ctrl Pts',(109.067,-4.79005070725105,4.34562748465468));
#35704=CARTESIAN_POINT('Ctrl Pts',(109.067,-4.89892627992167,4.20425211433211));
#35705=CARTESIAN_POINT('Ctrl Pts',(109.067,-5.00772778645258,4.06297291919076));
#35706=CARTESIAN_POINT('Ctrl Pts',(109.067,-5.11060752150017,3.91740955440837));
#35707=CARTESIAN_POINT('Ctrl Pts',(109.067,-5.20723092161534,3.76792762612764));
#35708=CARTESIAN_POINT('Ctrl Pts',(109.067,-5.30260180511279,3.6203834127172));
#35709=CARTESIAN_POINT('Ctrl Pts',(109.067,-5.39187784502882,3.46902093588031));
#35710=CARTESIAN_POINT('Ctrl Pts',(109.067,-5.47469157281416,3.3141702583193));
#35711=CARTESIAN_POINT('Ctrl Pts',(109.067,-5.49803287402587,3.27052512357597));
#35712=CARTESIAN_POINT('Ctrl Pts',(109.067,-5.52086050257896,3.22660278126208));
#35713=CARTESIAN_POINT('Ctrl Pts',(109.067,-5.54316550433805,3.18241041195473));
#35714=CARTESIAN_POINT('Ctrl Pts',(109.067,-5.60230175559497,3.06524516430197));
#35715=CARTESIAN_POINT('Ctrl Pts',(109.067,-5.65776545712255,2.94618196012103));
#35716=CARTESIAN_POINT('Ctrl Pts',(109.067,-5.70950047684215,2.82539173952989));
#35717=CARTESIAN_POINT('Ctrl Pts',(109.067,-5.73213454796948,2.77254601802126));
#35718=CARTESIAN_POINT('Ctrl Pts',(109.067,-5.75405472907524,2.71936971398817));
#35719=CARTESIAN_POINT('Ctrl Pts',(109.067,-5.7752553910661,2.665877096622));
#35720=CARTESIAN_POINT('Ctrl Pts',(109.067,-5.78798264815911,2.63376421759534));
#35721=CARTESIAN_POINT('Ctrl Pts',(109.067,-5.80045058798087,2.60153734283538));
#35722=CARTESIAN_POINT('Ctrl Pts',(109.067,-5.81265789335266,2.56919956290054));
#35723=CARTESIAN_POINT('Ctrl Pts',(109.067,-5.82219808721407,2.54392709856629));
#35724=CARTESIAN_POINT('Ctrl Pts',(109.067,-5.83158011004563,2.5185839007308));
#35725=CARTESIAN_POINT('Ctrl Pts',(109.067,-5.84079494789832,2.49319504473949));
#35726=CARTESIAN_POINT('Ctrl Pts',(109.067,-5.90045856108198,2.32880898529301));
#35727=CARTESIAN_POINT('Ctrl Pts',(109.067,-5.95319307428684,2.16231505043118));
#35728=CARTESIAN_POINT('Ctrl Pts',(109.067,-5.99896322840551,1.99414444801905));
#35729=CARTESIAN_POINT('Ctrl Pts',(109.067,-6.04501451703568,1.82494088950119));
#35730=CARTESIAN_POINT('Ctrl Pts',(109.067,-6.08401576538923,1.65403930183469));
#35731=CARTESIAN_POINT('Ctrl Pts',(109.067,-6.11588044698519,1.48186537531838));
#35732=CARTESIAN_POINT('Ctrl Pts',(109.067,-6.14757987742922,1.31058434771906));
#35733=CARTESIAN_POINT('Ctrl Pts',(109.067,-6.17221661993806,1.13804344736959));
#35734=CARTESIAN_POINT('Ctrl Pts',(109.067,-6.18965430287559,0.96465894100687));
#35735=CARTESIAN_POINT('Ctrl Pts',(109.067,-6.20678035459018,0.794373012932948));
#35736=CARTESIAN_POINT('Ctrl Pts',(109.067,-6.21696230688685,0.6232727421406));
#35737=CARTESIAN_POINT('Ctrl Pts',(109.067,-6.22002164922363,0.451759430133508));
#35738=CARTESIAN_POINT('Ctrl Pts',(109.067,-6.22187578004815,0.347812867898749));
#35739=CARTESIAN_POINT('Ctrl Pts',(109.067,-6.22111280177593,0.243714769828713));
#35740=CARTESIAN_POINT('Ctrl Pts',(109.067,-6.21768400249992,0.139557183822751));
#35741=CARTESIAN_POINT('Ctrl Pts',(30.6549162453659,0.653767430832815,-6.1847925356379));
#35742=CARTESIAN_POINT('Ctrl Pts',(30.6880015127729,1.68232745378033,-6.07606794386137));
#35743=CARTESIAN_POINT('Ctrl Pts',(30.7541720475869,3.67991374771159,-5.3378881315643));
#35744=CARTESIAN_POINT('Ctrl Pts',(30.853427849808,5.79294729058132,-2.91848348878711));
#35745=CARTESIAN_POINT('Ctrl Pts',(30.9526836520291,6.46975467895848,0.195461407864942));
#35746=CARTESIAN_POINT('Ctrl Pts',(31.0850247216571,5.32189755126117,4.32218967016898));
#35747=CARTESIAN_POINT('Ctrl Pts',(31.2504510586922,0.326999582929717,7.34773416501965));
#35748=CARTESIAN_POINT('Ctrl Pts',(31.4489626631343,-6.0124639065617,4.23976817199318));
#35749=CARTESIAN_POINT('Ctrl Pts',(31.6143890001695,-6.67314725497242,-1.56582020690343));
#35750=CARTESIAN_POINT('Ctrl Pts',(31.7467300697975,-4.11675109351076,-4.99488165618313));
#35751=CARTESIAN_POINT('Ctrl Pts',(31.8459858720185,-1.23075458232488,-6.37221708890274));
#35752=CARTESIAN_POINT('Ctrl Pts',(31.9452416742396,1.95775582174799,-6.16839483200312));
#35753=CARTESIAN_POINT('Ctrl Pts',(32.0775827438677,5.61197648499354,-3.94108216408908));
#35754=CARTESIAN_POINT('Ctrl Pts',(32.2430090809028,7.15393902550158,1.69766694268016));
#35755=CARTESIAN_POINT('Ctrl Pts',(32.4415206853449,2.4432388603139,6.93479746587837));
#35756=CARTESIAN_POINT('Ctrl Pts',(32.640032289787,-4.49951570882378,5.81505721359621));
#35757=CARTESIAN_POINT('Ctrl Pts',(32.8385438942291,-7.32504123893786,-0.637509834538132));
#35758=CARTESIAN_POINT('Ctrl Pts',(33.0039702312642,-4.08817544863011,-5.50554583451141));
#35759=CARTESIAN_POINT('Ctrl Pts',(33.1363113008923,0.0804192017098835,
-6.47115594816462));
#35760=CARTESIAN_POINT('Ctrl Pts',(33.2355671031134,3.17242495854284,-5.66210588059523));
#35761=CARTESIAN_POINT('Ctrl Pts',(33.3348229053343,5.47694100310651,-3.44753091698999));
#35762=CARTESIAN_POINT('Ctrl Pts',(33.4671639749625,6.83006089629673,0.611842341327977));
#35763=CARTESIAN_POINT('Ctrl Pts',(33.6325903119975,4.36852741272638,5.91430153013899));
#35764=CARTESIAN_POINT('Ctrl Pts',(33.8311019164398,-2.60995361271077,6.87374912585412));
#35765=CARTESIAN_POINT('Ctrl Pts',(34.0296135208817,-7.19004543862418,1.53737728295951));
#35766=CARTESIAN_POINT('Ctrl Pts',(34.2281251253239,-5.18342127361679,-5.21489534401854));
#35767=CARTESIAN_POINT('Ctrl Pts',(34.393551462359,0.430999447686097,-6.84385381815942));
#35768=CARTESIAN_POINT('Ctrl Pts',(34.5258925319871,4.23822627631683,-4.89078499723656));
#35769=CARTESIAN_POINT('Ctrl Pts',(34.6251483342081,6.07771306114946,-2.27708986044939));
#35770=CARTESIAN_POINT('Ctrl Pts',(34.7244041364292,6.40850984162318,0.901854494708191));
#35771=CARTESIAN_POINT('Ctrl Pts',(34.8567452060572,4.82190714720603,4.87578785427672));
#35772=CARTESIAN_POINT('Ctrl Pts',(35.0221715430924,-0.48069030065227,7.33702428029021));
#35773=CARTESIAN_POINT('Ctrl Pts',(35.2206831475344,-6.43014857662837,3.56559582231111));
#35774=CARTESIAN_POINT('Ctrl Pts',(35.4191947519766,-6.48407686024324,-3.46655903964816));
#35775=CARTESIAN_POINT('Ctrl Pts',(35.6177063564187,-0.593159681851761,
-7.32878912572931));
#35776=CARTESIAN_POINT('Ctrl Pts',(35.7831326934538,4.74656140271064,-4.94916665150982));
#35777=CARTESIAN_POINT('Ctrl Pts',(35.9154737630819,6.39392461916095,-1.00003397421454));
#35778=CARTESIAN_POINT('Ctrl Pts',(36.0147295653029,6.1119213231936,2.18360983365812));
#35779=CARTESIAN_POINT('Ctrl Pts',(36.1139853675239,4.31273644099712,4.82520925710656));
#35780=CARTESIAN_POINT('Ctrl Pts',(36.2463264371521,0.535911013730674,6.83643877180359));
#35781=CARTESIAN_POINT('Ctrl Pts',(36.4117527741871,-5.10283212902811,5.29377868085695));
#35782=CARTESIAN_POINT('Ctrl Pts',(36.6102643786293,-7.21277826054165,-1.42692468663486));
#35783=CARTESIAN_POINT('Ctrl Pts',(36.8087759830713,-2.71506717634408,-6.83291259456277));
#35784=CARTESIAN_POINT('Ctrl Pts',(37.0072875875135,4.27730707652595,-5.98060470455043));
#35785=CARTESIAN_POINT('Ctrl Pts',(37.1727139245486,6.81987484110359,-0.716521351391848));
#35786=CARTESIAN_POINT('Ctrl Pts',(37.3050549941766,5.52916938658696,3.36312739553527));
#35787=CARTESIAN_POINT('Ctrl Pts',(37.4043107963977,3.25889279038126,5.6127846874694));
#35788=CARTESIAN_POINT('Ctrl Pts',(37.5035665986187,0.179650915968158,6.46916266085227));
#35789=CARTESIAN_POINT('Ctrl Pts',(37.6359076682469,-4.00324642534526,5.56759497029643));
#35790=CARTESIAN_POINT('Ctrl Pts',(37.8013340052818,-7.31442513907121,0.749782197655131));
#35791=CARTESIAN_POINT('Ctrl Pts',(37.9998456097241,-4.58813259367446,-5.74537410443173));
#35792=CARTESIAN_POINT('Ctrl Pts',(38.1983572141661,2.33652476986658,-6.97143717584924));
#35793=CARTESIAN_POINT('Ctrl Pts',(38.3968688186083,7.12719834562496,-1.8072167000993));
#35794=CARTESIAN_POINT('Ctrl Pts',(38.5622951556433,5.67151826603053,3.85460455214176));
#35795=CARTESIAN_POINT('Ctrl Pts',(38.6946362252714,2.05246604268208,6.13756654772971));
#35796=CARTESIAN_POINT('Ctrl Pts',(38.7938920274925,-1.13361812652741,6.39051203819357));
#35797=CARTESIAN_POINT('Ctrl Pts',(38.8931478297135,-4.03830067804228,5.0571204867886));
#35798=CARTESIAN_POINT('Ctrl Pts',(39.0254888993416,-6.65129306476565,1.66865103059635));
#35799=CARTESIAN_POINT('Ctrl Pts',(39.1909152363767,-6.07072539313457,-4.14840712323998));
#35800=CARTESIAN_POINT('Ctrl Pts',(39.3894268408188,0.203920765924685,-7.34974153411109));
#35801=CARTESIAN_POINT('Ctrl Pts',(39.5879384452609,6.28435572899307,-3.81669456054382));
#35802=CARTESIAN_POINT('Ctrl Pts',(39.786450049703,6.61024172910176,3.21989017543126));
#35803=CARTESIAN_POINT('Ctrl Pts',(39.9518763867381,1.8439687800484,6.60483722990331));
#35804=CARTESIAN_POINT('Ctrl Pts',(40.0842174563662,-2.39381056423673,6.01265423641858));
#35805=CARTESIAN_POINT('Ctrl Pts',(40.1834732585872,-4.99061430015067,4.14939791707426));
#35806=CARTESIAN_POINT('Ctrl Pts',(40.2827290608084,-6.34858204315922,1.25612341171161));
#35807=CARTESIAN_POINT('Ctrl Pts',(40.4150701304363,-6.15730676139607,-3.01855414749781));
#35808=CARTESIAN_POINT('Ctrl Pts',(40.5804964674716,-1.95924956424283,-7.08691255794874));
#35809=CARTESIAN_POINT('Ctrl Pts',(40.7790080719135,4.89964311770096,-5.48213294404453));
#35810=CARTESIAN_POINT('Ctrl Pts',(40.9775196763558,7.26349285183276,1.1410328165251));
#35811=CARTESIAN_POINT('Ctrl Pts',(41.1760312807977,2.97064458683377,6.72593927996026));
#35812=CARTESIAN_POINT('Ctrl Pts',(41.3414576178329,-2.85466105015735,6.23498243654499));
#35813=CARTESIAN_POINT('Ctrl Pts',(41.473798687461,-5.70926470123999,3.04739832567862));
#35814=CARTESIAN_POINT('Ctrl Pts',(41.573054489682,-6.49007271635678,-0.0518681355929193));
#35815=CARTESIAN_POINT('Ctrl Pts',(41.6723102919031,-5.65982942715753,-3.13825920530084));
#35816=CARTESIAN_POINT('Ctrl Pts',(41.8046513615312,-2.7546438300705,-6.2798115469148));
#35817=CARTESIAN_POINT('Ctrl Pts',(41.9700776985662,3.07776459442245,-6.67760088357463));
#35818=CARTESIAN_POINT('Ctrl Pts',(42.1685893030084,7.280801980269,-1.02479599000183));
#35819=CARTESIAN_POINT('Ctrl Pts',(42.3671009074504,4.81139734096477,5.55974279300492));
#35820=CARTESIAN_POINT('Ctrl Pts',(42.5656125118927,-2.0722681306563,7.05469299499727));
#35821=CARTESIAN_POINT('Ctrl Pts',(42.7310388489277,-6.20476526695897,2.91975746890894));
#35822=CARTESIAN_POINT('Ctrl Pts',(42.8633799185558,-6.32769472643081,-1.35743118914858));
#35823=CARTESIAN_POINT('Ctrl Pts',(42.9626357207768,-4.92365776368081,-4.22863197656575));
#35824=CARTESIAN_POINT('Ctrl Pts',(43.0618915229979,-2.29740564112336,-6.05014605644428));
#35825=CARTESIAN_POINT('Ctrl Pts',(43.1942325926259,1.94929714981741,-6.57452175576472));
#35826=CARTESIAN_POINT('Ctrl Pts',(43.3596589296611,6.6608602966818,-3.11382860271486));
#35827=CARTESIAN_POINT('Ctrl Pts',(43.5581705341031,6.22255147548853,3.9166487501317));
#35828=CARTESIAN_POINT('Ctrl Pts',(43.7566821385453,0.0864251429686191,
7.35206195510319));
#35829=CARTESIAN_POINT('Ctrl Pts',(43.9551937429874,-6.13625319161177,4.05084993889327));
#35830=CARTESIAN_POINT('Ctrl Pts',(44.1206200800225,-6.62377372820908,-1.77474428941108));
#35831=CARTESIAN_POINT('Ctrl Pts',(44.2529611496505,-3.9569578199035,-5.12101794526032));
#35832=CARTESIAN_POINT('Ctrl Pts',(44.3522169518716,-1.03133493987818,-6.40781416778569));
#35833=CARTESIAN_POINT('Ctrl Pts',(44.4514727540926,2.15029947849091,-6.10397838601804));
#35834=CARTESIAN_POINT('Ctrl Pts',(44.5838138237208,5.73240126379457,-3.76346535073147));
#35835=CARTESIAN_POINT('Ctrl Pts',(44.7492401607558,7.09740355031088,1.92089856656498));
#35836=CARTESIAN_POINT('Ctrl Pts',(44.9477517651979,2.22480311159819,7.00789093890849));
#35837=CARTESIAN_POINT('Ctrl Pts',(45.1462633696401,-4.67937380009033,5.67130894380136));
#35838=CARTESIAN_POINT('Ctrl Pts',(45.3447749740821,-7.30150721100801,-0.866591545421022));
#35839=CARTESIAN_POINT('Ctrl Pts',(45.5102013111172,-3.91374922444537,-5.63086695842329));
#35840=CARTESIAN_POINT('Ctrl Pts',(45.6425423807454,0.283023412847933,-6.46546500508306));
#35841=CARTESIAN_POINT('Ctrl Pts',(45.7417981829663,3.34818463267598,-5.55998145973536));
#35842=CARTESIAN_POINT('Ctrl Pts',(45.8410539851874,5.58221537749888,-3.27432610828378));
#35843=CARTESIAN_POINT('Ctrl Pts',(45.9733950548155,6.80755168564738,0.825430640665489));
#35844=CARTESIAN_POINT('Ctrl Pts',(46.1388213918506,4.18117380984599,6.04820419883911));
#35845=CARTESIAN_POINT('Ctrl Pts',(46.3373329962928,-2.82392956463494,6.78864538114884));
#35846=CARTESIAN_POINT('Ctrl Pts',(46.5358446007348,-7.23466322442155,1.31146190421813));
#35847=CARTESIAN_POINT('Ctrl Pts',(46.734356205177,-5.01757083003903,-5.37466012176944));
#35848=CARTESIAN_POINT('Ctrl Pts',(46.899782542212,0.645108111263187,-6.82700016259648));
#35849=CARTESIAN_POINT('Ctrl Pts',(47.0321236118402,4.38930599811985,-4.75566323860751));
#35850=CARTESIAN_POINT('Ctrl Pts',(47.1313794140611,6.14604086368536,-2.08564519249999));
#35851=CARTESIAN_POINT('Ctrl Pts',(47.2306352162823,6.37712454126565,1.10209916493979));
#35852=CARTESIAN_POINT('Ctrl Pts',(47.3629762859102,4.66685348261288,5.0243979009563));
#35853=CARTESIAN_POINT('Ctrl Pts',(47.5284026229454,-0.710218612843849,
7.31837263201097));
#35854=CARTESIAN_POINT('Ctrl Pts',(47.7269142273875,-6.5386540061078,3.36248242901333));
#35855=CARTESIAN_POINT('Ctrl Pts',(47.9254258318296,-6.37233896675448,-3.66791226582583));
#35856=CARTESIAN_POINT('Ctrl Pts',(48.1239374362717,-0.363362580539744,
-7.34376988297294));
#35857=CARTESIAN_POINT('Ctrl Pts',(48.2893637733068,4.89922005122494,-4.79809739219469));
#35858=CARTESIAN_POINT('Ctrl Pts',(48.4217048429349,6.42210544142411,-0.79931325736819));
#35859=CARTESIAN_POINT('Ctrl Pts',(48.5209606451559,6.04054241262091,2.37393797905852));
#35860=CARTESIAN_POINT('Ctrl Pts',(48.620216447377,4.1595164104518,4.95789907272788));
#35861=CARTESIAN_POINT('Ctrl Pts',(48.7525575170051,0.321560287482606,6.84986822331817));
#35862=CARTESIAN_POINT('Ctrl Pts',(48.9179838540402,-5.26610780985881,5.1313835360399));
#35863=CARTESIAN_POINT('Ctrl Pts',(49.1164954584823,-7.1645555542505,-1.65209806218378));
#35864=CARTESIAN_POINT('Ctrl Pts',(49.3150070629244,-2.4997580926362,-6.91458558232614));
#35865=CARTESIAN_POINT('Ctrl Pts',(49.5135186673665,4.46249608146065,-5.84372459840002));
#35866=CARTESIAN_POINT('Ctrl Pts',(49.6789450044016,6.838968356171,-0.502600754676708));
#35867=CARTESIAN_POINT('Ctrl Pts',(49.8112860740297,5.42113886922714,3.53462775193207));
#35868=CARTESIAN_POINT('Ctrl Pts',(49.9105418762507,3.08152614660459,5.71208637669992));
#35869=CARTESIAN_POINT('Ctrl Pts',(50.0097976784718,-0.0230235705233395,
6.47161571011243));
#35870=CARTESIAN_POINT('Ctrl Pts',(50.1421387480999,-4.17563615511025,5.43949982952901));
#35871=CARTESIAN_POINT('Ctrl Pts',(50.3075650851349,-7.33431768531273,0.52035809776168));
#35872=CARTESIAN_POINT('Ctrl Pts',(50.5060766895771,-4.40596188428978,-5.88623684294122));
#35873=CARTESIAN_POINT('Ctrl Pts',(50.7045882940192,2.55369426009361,-6.89484807105841));
#35874=CARTESIAN_POINT('Ctrl Pts',(50.9030998984613,7.1802970231816,-1.58313711278791));
#35875=CARTESIAN_POINT('Ctrl Pts',(51.0685262354964,5.54802698009573,4.03032161538502));
#35876=CARTESIAN_POINT('Ctrl Pts',(51.2008673051245,1.8592571864357,6.19883075255818));
#35877=CARTESIAN_POINT('Ctrl Pts',(51.3001231073455,-1.33318551163412,6.35187771912034));
#35878=CARTESIAN_POINT('Ctrl Pts',(51.3993789095666,-4.19468734797827,4.92817796319135));
#35879=CARTESIAN_POINT('Ctrl Pts',(51.5317199791946,-6.70028587202019,1.45954271212482));
#35880=CARTESIAN_POINT('Ctrl Pts',(51.6971463162298,-5.93783767930351,-4.33648154074716));
#35881=CARTESIAN_POINT('Ctrl Pts',(51.8956579206718,0.433983073355225,-7.33975088058538));
#35882=CARTESIAN_POINT('Ctrl Pts',(52.094169525114,6.40079599604896,-3.61802361987541));
#35883=CARTESIAN_POINT('Ctrl Pts',(52.2926811295561,6.50616656657558,3.42531532372877));
#35884=CARTESIAN_POINT('Ctrl Pts',(52.4581074665912,1.63622927289707,6.65934302028545));
#35885=CARTESIAN_POINT('Ctrl Pts',(52.5904485362193,-2.58092699663894,5.93474142841911));
#35886=CARTESIAN_POINT('Ctrl Pts',(52.6897043384402,-5.11810793105627,3.99107822187782));
#35887=CARTESIAN_POINT('Ctrl Pts',(52.7889601406614,-6.38480472479868,1.05669702865221));
#35888=CARTESIAN_POINT('Ctrl Pts',(52.9213012102894,-6.05975872316839,-3.20989406558761));
#35889=CARTESIAN_POINT('Ctrl Pts',(53.0867275473246,-1.73635698912002,-7.14479200994201));
#35890=CARTESIAN_POINT('Ctrl Pts',(53.2852391517666,5.06891690010915,-5.32600842627953));
#35891=CARTESIAN_POINT('Ctrl Pts',(53.4837507562088,7.22419817707089,1.36793457278422));
#35892=CARTESIAN_POINT('Ctrl Pts',(53.6822623606508,2.75856009795156,6.81566831976048));
#35893=CARTESIAN_POINT('Ctrl Pts',(53.847688697686,-3.04851381910718,6.14252872927938));
#35894=CARTESIAN_POINT('Ctrl Pts',(53.980029767314,-5.80189597337518,2.86711407138024));
#35895=CARTESIAN_POINT('Ctrl Pts',(54.0792855695351,-6.4852653283173,-0.255083885053564));
#35896=CARTESIAN_POINT('Ctrl Pts',(54.1785413717561,-5.55877673210131,-3.31396156085478));
#35897=CARTESIAN_POINT('Ctrl Pts',(54.3108824413843,-2.55663608376213,-6.36299517762788));
#35898=CARTESIAN_POINT('Ctrl Pts',(54.4763087784192,3.28536884845591,-6.57794344674629));
#35899=CARTESIAN_POINT('Ctrl Pts',(54.6748203828615,7.30932326741656,-0.796289940546589));
#35900=CARTESIAN_POINT('Ctrl Pts',(54.8733319873035,4.63493030483003,5.70768826815035));
#35901=CARTESIAN_POINT('Ctrl Pts',(55.0718435917456,-2.29217444186588,6.98633843920073));
#35902=CARTESIAN_POINT('Ctrl Pts',(55.2372699287808,-6.29315635428496,2.72401886847961));
#35903=CARTESIAN_POINT('Ctrl Pts',(55.3696109984087,-6.28208235318225,-1.55492163532759));
#35904=CARTESIAN_POINT('Ctrl Pts',(55.4688668006299,-4.78882033941213,-4.38074581822788));
#35905=CARTESIAN_POINT('Ctrl Pts',(55.5681226028509,-2.10681428668835,-6.11912359293222));
#35906=CARTESIAN_POINT('Ctrl Pts',(55.700463672479,2.1542268731561,-6.51025362595669));
#35907=CARTESIAN_POINT('Ctrl Pts',(55.865890009514,6.75510516300982,-2.90371188234558));
#35908=CARTESIAN_POINT('Ctrl Pts',(56.0644016139562,6.09684697384953,4.10959137560839));
#35909=CARTESIAN_POINT('Ctrl Pts',(56.2629132183983,-0.143852232229424,
7.35116254971248));
#35910=CARTESIAN_POINT('Ctrl Pts',(56.4614248228404,-6.26009883682339,3.85670209015414));
#35911=CARTESIAN_POINT('Ctrl Pts',(56.6268511598755,-6.56494768793653,-1.98130198353674));
#35912=CARTESIAN_POINT('Ctrl Pts',(56.7591922295036,-3.7946488264813,-5.24242122190289));
#35913=CARTESIAN_POINT('Ctrl Pts',(56.8584480317246,-0.830163910262025,
-6.43696838963711));
#35914=CARTESIAN_POINT('Ctrl Pts',(56.9577038339457,2.34039522251466,-6.03364650825719));
#35915=CARTESIAN_POINT('Ctrl Pts',(57.0900449035737,5.84744533060766,-3.58210535870519));
#35916=CARTESIAN_POINT('Ctrl Pts',(57.2554712406089,7.03376829111499,2.14221662907907));
#35917=CARTESIAN_POINT('Ctrl Pts',(57.4539828450509,2.00425491144597,7.07412514357485));
#35918=CARTESIAN_POINT('Ctrl Pts',(57.6524944494932,-4.85467979449576,5.52198953185602));
#35919=CARTESIAN_POINT('Ctrl Pts',(57.8510060539352,-7.27078821313233,-1.09481834966948));
#35920=CARTESIAN_POINT('Ctrl Pts',(58.0164323909703,-3.73549514279114,-5.75066706856635));
#35921=CARTESIAN_POINT('Ctrl Pts',(58.1487734605983,0.485355182835179,-6.45343089609464));
#35922=CARTESIAN_POINT('Ctrl Pts',(58.2480292628194,3.52065721958024,-5.45240377350268));
#35923=CARTESIAN_POINT('Ctrl Pts',(58.3472850650405,5.68201536485552,-3.09790919455678));
#35924=CARTESIAN_POINT('Ctrl Pts',(58.4796261346685,6.77836393432703,1.03820906811895));
#35925=CARTESIAN_POINT('Ctrl Pts',(58.6450524717037,3.98971935895797,6.17617421190118));
#35926=CARTESIAN_POINT('Ctrl Pts',(58.8435640761457,-3.03513575029629,6.69688250414221));
#35927=CARTESIAN_POINT('Ctrl Pts',(59.0420756805879,-7.27218428522181,1.08426012505574));
#35928=CARTESIAN_POINT('Ctrl Pts',(59.2405872850299,-4.84679866862674,-5.52915283970294));
#35929=CARTESIAN_POINT('Ctrl Pts',(59.406013622065,0.858584021869272,-6.80344979938125));
#35930=CARTESIAN_POINT('Ctrl Pts',(59.5383546916932,4.53608016947545,-4.61587658850033));
#35931=CARTESIAN_POINT('Ctrl Pts',(59.6376104939142,6.20833994062302,-1.89215468415061));
#35932=CARTESIAN_POINT('Ctrl Pts',(59.7368662961353,6.33948382661728,1.30126276986307));
#35933=CARTESIAN_POINT('Ctrl Pts',(59.8692073657633,4.50722204056254,5.16807944718129));
#35934=CARTESIAN_POINT('Ctrl Pts',(60.0346337027984,-0.939050263787701,
7.2925422906609));
#35935=CARTESIAN_POINT('Ctrl Pts',(60.2331453072406,-6.64074557868628,3.15607073054002));
#35936=CARTESIAN_POINT('Ctrl Pts',(60.4316569116826,-6.25435035863348,-3.86566758639099));
#35937=CARTESIAN_POINT('Ctrl Pts',(60.6301685161248,-0.133209051532416,
-7.35154703498433));
#35938=CARTESIAN_POINT('Ctrl Pts',(60.7955948531599,5.0470729870606,-4.64232161300714));
#35939=CARTESIAN_POINT('Ctrl Pts',(60.9279359227879,6.44398673196168,-0.597808483107745));
#35940=CARTESIAN_POINT('Ctrl Pts',(61.027191725009,5.96323825064499,2.56193749594574));
#35941=CARTESIAN_POINT('Ctrl Pts',(61.12644752723,4.00221625291053,5.08572561677413));
#35942=CARTESIAN_POINT('Ctrl Pts',(61.2587885968582,0.106894138300333,6.85657854461737));
#35943=CARTESIAN_POINT('Ctrl Pts',(61.4242149338931,-5.42421789290193,4.96395494634262));
#35944=CARTESIAN_POINT('Ctrl Pts',(61.6227265383354,-7.10930503660753,-1.87565087195877));
#35945=CARTESIAN_POINT('Ctrl Pts',(61.8212381427774,-2.28199696173699,-6.98947595772644));
#35946=CARTESIAN_POINT('Ctrl Pts',(62.0197497472196,4.64330776244168,-5.70111230219558));
#35947=CARTESIAN_POINT('Ctrl Pts',(62.1851760842546,6.85135343285645,-0.288187149949455));
#35948=CARTESIAN_POINT('Ctrl Pts',(62.3175171538827,5.30779068198273,3.70266094321786));
#35949=CARTESIAN_POINT('Ctrl Pts',(62.4167729561038,2.90113679133094,5.80578500162336));
#35950=CARTESIAN_POINT('Ctrl Pts',(62.5160287583248,-0.225675472877136,
6.46772066226701));
#35951=CARTESIAN_POINT('Ctrl Pts',(62.6483698279529,-4.34392994578106,5.30606900835795));
#35952=CARTESIAN_POINT('Ctrl Pts',(62.813796164988,-7.34701589818293,0.29042357143327));
#35953=CARTESIAN_POINT('Ctrl Pts',(63.0123077694301,-4.21946930612633,-6.02132569054943));
#35954=CARTESIAN_POINT('Ctrl Pts',(63.2108193738721,2.7683587964008,-6.81149571470196));
#35955=CARTESIAN_POINT('Ctrl Pts',(63.4093309783144,7.22635244835865,-1.35750460444815));
#35956=CARTESIAN_POINT('Ctrl Pts',(63.5747573153493,5.41909355797858,4.20208528057022));
#35957=CARTESIAN_POINT('Ctrl Pts',(63.7070983849776,1.66422455917251,6.25401443880813));
#35958=CARTESIAN_POINT('Ctrl Pts',(63.8063541871984,-1.53144515668549,6.30701275558833));
#35959=CARTESIAN_POINT('Ctrl Pts',(63.9056099894197,-4.34695939124221,4.79440132186115));
#35960=CARTESIAN_POINT('Ctrl Pts',(64.0379510590476,-6.74270627645356,1.24900270807729));
#35961=CARTESIAN_POINT('Ctrl Pts',(64.2033773960828,-5.79912545859896,-4.52030224370326));
#35962=CARTESIAN_POINT('Ctrl Pts',(64.4018890005248,0.663619680803454,-7.32256056419159));
#35963=CARTESIAN_POINT('Ctrl Pts',(64.600400604967,6.5109576340338,-3.4158037099402));
#35964=CARTESIAN_POINT('Ctrl Pts',(64.798912209409,6.39570941553163,3.62738053298608));
#35965=CARTESIAN_POINT('Ctrl Pts',(64.9643385464442,1.42688476588627,6.70731656925046));
#35966=CARTESIAN_POINT('Ctrl Pts',(65.0966796160723,-2.76551176215596,5.8510071507069));
#35967=CARTESIAN_POINT('Ctrl Pts',(65.1959354182932,-5.24058113930113,3.82884362299698));
#35968=CARTESIAN_POINT('Ctrl Pts',(65.2951912205144,-6.4147644634311,0.856234116925767));
#35969=CARTESIAN_POINT('Ctrl Pts',(65.4275322901425,-5.95626658402133,-3.39808535436641));
#35970=CARTESIAN_POINT('Ctrl Pts',(65.5929586271775,-1.51176119750446,-7.19566303681453));
#35971=CARTESIAN_POINT('Ctrl Pts',(65.7914702316198,5.23321851206271,-5.16465955355726));
#35972=CARTESIAN_POINT('Ctrl Pts',(65.9899818360617,7.17781718660405,1.59349450345578));
#35973=CARTESIAN_POINT('Ctrl Pts',(66.1884934405039,2.54376969957746,6.89871177591126));
#35974=CARTESIAN_POINT('Ctrl Pts',(66.353919777539,-3.23937625907777,6.04404973191034));
#35975=CARTESIAN_POINT('Ctrl Pts',(66.486260847167,-5.88883608535315,2.68401742388717));
#35976=CARTESIAN_POINT('Ctrl Pts',(66.5855166493881,-6.47409645489935,-0.45804941602601));
#35977=CARTESIAN_POINT('Ctrl Pts',(66.6847724516092,-5.45227135475848,-3.4864132116906));
#35978=CARTESIAN_POINT('Ctrl Pts',(66.8171135212372,-2.35612050115225,-6.43993724590316));
#35979=CARTESIAN_POINT('Ctrl Pts',(66.9825398582723,3.48975044558929,-6.47183364038364));
#35980=CARTESIAN_POINT('Ctrl Pts',(67.1810514627144,7.33067472739079,-0.567002756194563));
#35981=CARTESIAN_POINT('Ctrl Pts',(67.3795630671566,4.45391682219975,5.85003491379102));
#35982=CARTESIAN_POINT('Ctrl Pts',(67.5780746715986,-2.50983236811194,6.91113104420389));
#35983=CARTESIAN_POINT('Ctrl Pts',(67.7435010086337,-6.37537432645889,2.5256079652503));
#35984=CARTESIAN_POINT('Ctrl Pts',(67.8758420782619,-6.23030789835879,-1.75088645287108));
#35985=CARTESIAN_POINT('Ctrl Pts',(67.9750978804828,-4.64928527757637,-4.52856336585343));
#35986=CARTESIAN_POINT('Ctrl Pts',(68.074353682704,-1.91415673077897,-6.18209724638608));
#35987=CARTESIAN_POINT('Ctrl Pts',(68.2066947523319,2.35704435361657,-6.43960284826646));
#35988=CARTESIAN_POINT('Ctrl Pts',(68.3721210893672,6.84272208387396,-2.69074004151496));
#35989=CARTESIAN_POINT('Ctrl Pts',(68.5706326938092,5.96516493496265,4.29849148457416));
#35990=CARTESIAN_POINT('Ctrl Pts',(68.7691442982513,-0.373993920311934,
7.34307320266848));
#35991=CARTESIAN_POINT('Ctrl Pts',(68.9676559026935,-6.37779317569966,3.65872989786245));
#35992=CARTESIAN_POINT('Ctrl Pts',(69.1330822397285,-6.49970078748444,-2.18584368611994));
#35993=CARTESIAN_POINT('Ctrl Pts',(69.2654233093567,-3.62859134903107,-5.35878348065247));
#35994=CARTESIAN_POINT('Ctrl Pts',(69.3646791115776,-0.62823592000139,-6.45958714174554));
#35995=CARTESIAN_POINT('Ctrl Pts',(69.4639349137987,2.52830110610206,-5.95780469931484));
#35996=CARTESIAN_POINT('Ctrl Pts',(69.5962759834268,5.95652483419779,-3.3963489535312));
#35997=CARTESIAN_POINT('Ctrl Pts',(69.7617023204619,6.96369965258984,2.35963460035952));
#35998=CARTESIAN_POINT('Ctrl Pts',(69.9602139249039,1.78096623639146,7.13640802565527));
#35999=CARTESIAN_POINT('Ctrl Pts',(70.1587255293462,-5.02380608586829,5.3617905732631));
#36000=CARTESIAN_POINT('Ctrl Pts',(70.3572371337882,-7.23566990141503,-1.31149301022891));
#36001=CARTESIAN_POINT('Ctrl Pts',(70.5557487382304,-2.81181884640884,-6.79534921779986));
#36002=CARTESIAN_POINT('Ctrl Pts',(70.7211750752654,3.00649289900833,-6.16512333542295));
#36003=CARTESIAN_POINT('Ctrl Pts',(70.8535161448936,5.77263950695759,-2.91134114312552));
#36004=CARTESIAN_POINT('Ctrl Pts',(70.9858572145215,6.74314937401964,1.2444879873417));
#36005=CARTESIAN_POINT('Ctrl Pts',(71.1512835515567,3.79854938863639,6.30172191780343));
#36006=CARTESIAN_POINT('Ctrl Pts',(71.3497951559988,-3.25302923561936,6.59577169661227));
#36007=CARTESIAN_POINT('Ctrl Pts',(71.5152214930338,-6.6101259714308,1.81625507702285));
#36008=CARTESIAN_POINT('Ctrl Pts',(71.647562562662,-6.00358031277986,-2.41949711668263));
#36009=CARTESIAN_POINT('Ctrl Pts',(71.7468183648829,-4.12753807040063,-5.00810542026236));
#36010=CARTESIAN_POINT('Ctrl Pts',(71.8460741671042,-1.22942858196295,-6.35390206362266));
#36011=CARTESIAN_POINT('Ctrl Pts',(71.978415236732,3.04488676341186,-6.14439894507291));
#36012=CARTESIAN_POINT('Ctrl Pts',(72.1438415737674,7.09505541724423,-1.92914383180871));
#36013=CARTESIAN_POINT('Ctrl Pts',(72.3423531782092,5.46132883333844,4.92289529580099));
#36014=CARTESIAN_POINT('Ctrl Pts',(72.5408647826516,-1.17190946057312,7.25857562521031));
#36015=CARTESIAN_POINT('Ctrl Pts',(72.7393763870934,-6.73847855351414,2.94204908409314));
#36016=CARTESIAN_POINT('Ctrl Pts',(72.9048027241288,-6.22280912928604,-2.88112258378322));
#36017=CARTESIAN_POINT('Ctrl Pts',(73.0371437937567,-3.02311377228348,-5.72215776666869));
#36018=CARTESIAN_POINT('Ctrl Pts',(73.1363995959778,0.0794348410866285,
-6.48979416820313));
#36019=CARTESIAN_POINT('Ctrl Pts',(73.2356553981989,3.16227467098884,-5.6464470206576));
#36020=CARTESIAN_POINT('Ctrl Pts',(73.367996467827,6.29145571547599,-2.72794273270417));
#36021=CARTESIAN_POINT('Ctrl Pts',(73.533422804862,6.66446686956165,3.10610303551645));
#36022=CARTESIAN_POINT('Ctrl Pts',(73.7319344093041,0.993858002836962,7.28508954315968));
#36023=CARTESIAN_POINT('Ctrl Pts',(73.9304460137462,-5.58013110682443,4.78773641119374));
#36024=CARTESIAN_POINT('Ctrl Pts',(74.1289576181884,-7.04582651485609,-2.10221746089843));
#36025=CARTESIAN_POINT('Ctrl Pts',(74.2943839552234,-2.89337352700839,-6.21711227638719));
#36026=CARTESIAN_POINT('Ctrl Pts',(74.4267250248515,1.38429868618496,-6.32187133024273));
#36027=CARTESIAN_POINT('Ctrl Pts',(74.5259808270725,4.24950930786462,-4.9056503007122));
#36028=CARTESIAN_POINT('Ctrl Pts',(74.6252366292937,6.05985073959253,-2.27168416620927));
#36029=CARTESIAN_POINT('Ctrl Pts',(74.7575776989216,6.5661819132465,1.9772078337143));
#36030=CARTESIAN_POINT('Ctrl Pts',(74.9230040359569,3.08550547279318,6.67402760129288));
#36031=CARTESIAN_POINT('Ctrl Pts',(75.1215156403989,-3.94304652828918,6.20585758518567));
#36032=CARTESIAN_POINT('Ctrl Pts',(75.3200272448411,-7.35236275094442,0.0551931363052712));
#36033=CARTESIAN_POINT('Ctrl Pts',(75.5185388492831,-4.02474686326202,-6.15340565402118));
#36034=CARTESIAN_POINT('Ctrl Pts',(75.6839651863182,1.80286576781962,-6.61617493105383));
#36035=CARTESIAN_POINT('Ctrl Pts',(75.8163062559463,5.13778071835795,-3.93516826512113));
#36036=CARTESIAN_POINT('Ctrl Pts',(75.9155620581673,6.41213741680385,-1.0041055296563));
#36037=CARTESIAN_POINT('Ctrl Pts',(76.0148178603885,6.09478893729921,2.1762095014379));
#36038=CARTESIAN_POINT('Ctrl Pts',(76.1471589300164,3.73908041305424,5.74833657329857));
#36039=CARTESIAN_POINT('Ctrl Pts',(76.3125852670516,-1.95103068448381,7.08917962300208));
#36040=CARTESIAN_POINT('Ctrl Pts',(76.5110968714937,-7.01727857255056,2.19501383418843));
#36041=CARTESIAN_POINT('Ctrl Pts',(76.7096084759358,-5.65138000548379,-4.70342304397645));
#36042=CARTESIAN_POINT('Ctrl Pts',(76.9081200803781,0.897600199059924,-7.29776009071585));
#36043=CARTESIAN_POINT('Ctrl Pts',(77.0735464174129,5.64744158313445,-3.88979424396703));
#36044=CARTESIAN_POINT('Ctrl Pts',(77.2058874870412,6.46420439911098,0.31048586229469));
#36045=CARTESIAN_POINT('Ctrl Pts',(77.3051432892621,5.54570835728657,3.37177297323113));
#36046=CARTESIAN_POINT('Ctrl Pts',(77.4043990914832,3.2505835667813,5.59607420068252));
#36047=CARTESIAN_POINT('Ctrl Pts',(77.5367401611112,-0.854341364942577,
6.80398387178119));
#36048=CARTESIAN_POINT('Ctrl Pts',(77.7021664981465,-6.06591106563178,4.15544358677189));
#36049=CARTESIAN_POINT('Ctrl Pts',(77.9006781025884,-6.7765882047847,-2.85274194412771));
#36050=CARTESIAN_POINT('Ctrl Pts',(78.0991897070306,-1.28071754910471,-7.24016897982555));
#36051=CARTESIAN_POINT('Ctrl Pts',(78.2977013114727,5.39592604241165,-4.99469424527876));
#36052=CARTESIAN_POINT('Ctrl Pts',(78.4631276485078,6.82419817520737,0.674103078769445));
#36053=CARTESIAN_POINT('Ctrl Pts',(78.5954687181358,4.73697475670672,4.40946823761063));
#36054=CARTESIAN_POINT('Ctrl Pts',(78.6947245203569,2.0595182708145,6.1548451369039));
#36055=CARTESIAN_POINT('Ctrl Pts',(78.793980322578,-1.12917895789654,6.37238533558803));
#36056=CARTESIAN_POINT('Ctrl Pts',(78.9263213922061,-5.04417715043781,4.64546796031478));
#36057=CARTESIAN_POINT('Ctrl Pts',(79.091747729241,-7.31528962469706,-0.741300320920373));
#36058=CARTESIAN_POINT('Ctrl Pts',(79.2902593336834,-3.33467618405536,-6.55287868379289));
#36059=CARTESIAN_POINT('Ctrl Pts',(79.4887709381253,3.69494857957145,-6.35670034619658));
#36060=CARTESIAN_POINT('Ctrl Pts',(79.6872825425675,7.34524717088535,-0.332163299594867));
#36061=CARTESIAN_POINT('Ctrl Pts',(79.8527088796025,4.77724243558189,4.91955794833087));
#36062=CARTESIAN_POINT('Ctrl Pts',(79.9850499492307,0.772025231896089,6.42544294391362));
#36063=CARTESIAN_POINT('Ctrl Pts',(80.0843057514517,-2.39957651105506,6.03040353000374));
#36064=CARTESIAN_POINT('Ctrl Pts',(80.1835615536727,-4.97552377725469,4.13841794966956));
#36065=CARTESIAN_POINT('Ctrl Pts',(80.3159026233009,-6.85117239325693,0.292459455625172));
#36066=CARTESIAN_POINT('Ctrl Pts',(80.4813289603358,-5.10896704970656,-5.28785818115516));
#36067=CARTESIAN_POINT('Ctrl Pts',(80.6798405647781,1.68251786406567,-7.15747287344582));
#36068=CARTESIAN_POINT('Ctrl Pts',(80.8783521692202,6.92514205415142,-2.4703626913545));
#36069=CARTESIAN_POINT('Ctrl Pts',(81.0768637736622,5.82471539119074,4.48727969605447));
#36070=CARTESIAN_POINT('Ctrl Pts',(81.2422901106974,0.473544591506288,6.84104167617517));
#36071=CARTESIAN_POINT('Ctrl Pts',(81.3746311803253,-3.55762461323784,5.40607501755736));
#36072=CARTESIAN_POINT('Ctrl Pts',(81.4738869825466,-5.72512502258832,3.05723365852555));
#36073=CARTESIAN_POINT('Ctrl Pts',(81.5731427847674,-6.47145951622151,-0.0505144937619511));
#36074=CARTESIAN_POINT('Ctrl Pts',(81.7054838543957,-5.42171283747731,-4.19870522938243));
#36075=CARTESIAN_POINT('Ctrl Pts',(81.8709101914306,-0.48919755281723,-7.33646196836831));
#36076=CARTESIAN_POINT('Ctrl Pts',(82.069421795873,5.90490006067872,-4.38091766304837));
#36077=CARTESIAN_POINT('Ctrl Pts',(82.2679334003147,6.88393788382687,2.58296022203711));
#36078=CARTESIAN_POINT('Ctrl Pts',(82.4664450047572,1.55262125162276,7.18695733311437));
#36079=CARTESIAN_POINT('Ctrl Pts',(82.6318713417919,-4.05385301920155,5.53085629844241));
#36080=CARTESIAN_POINT('Ctrl Pts',(82.7642124114203,-6.20667286345935,1.83290805829735));
#36081=CARTESIAN_POINT('Ctrl Pts',(82.8634682136412,-6.34615709688077,-1.36015597223205));
#36082=CARTESIAN_POINT('Ctrl Pts',(82.9627240158624,-4.91031465598665,-4.2155841781865));
#36083=CARTESIAN_POINT('Ctrl Pts',(83.0950650854904,-1.43106703177257,-6.70642548947526));
#36084=CARTESIAN_POINT('Ctrl Pts',(83.2604914225255,4.36166608043273,-5.91936292702175));
#36085=CARTESIAN_POINT('Ctrl Pts',(83.4590030269676,7.33784111646791,0.465158087628112));
#36086=CARTESIAN_POINT('Ctrl Pts',(83.6575146314097,3.59080068386597,6.41610744499814));
#36087=CARTESIAN_POINT('Ctrl Pts',(83.8560262358518,-3.45292231992367,6.49155727938758));
#36088=CARTESIAN_POINT('Ctrl Pts',(84.0214525728869,-6.66623356367417,1.60792592175586));
#36089=CARTESIAN_POINT('Ctrl Pts',(84.1537936425151,-5.92372422041267,-2.6061142232585));
#36090=CARTESIAN_POINT('Ctrl Pts',(84.253049444736,-3.96930072085848,-5.13501567227216));
#36091=CARTESIAN_POINT('Ctrl Pts',(84.3523052469571,-1.02956513266701,-6.38923591846239));
#36092=CARTESIAN_POINT('Ctrl Pts',(84.4846463165852,3.23560668510475,-6.04606856350603));
#36093=CARTESIAN_POINT('Ctrl Pts',(84.6500726536202,7.15210351133029,-1.70599056920427));
#36094=CARTESIAN_POINT('Ctrl Pts',(84.8485842580625,5.30442784199376,5.09149580831549));
#36095=CARTESIAN_POINT('Ctrl Pts',(85.0470958625043,-1.39861029772509,7.21832207179135));
#36096=CARTESIAN_POINT('Ctrl Pts',(85.2456074669468,-6.82732506329547,2.72958255766234));
#36097=CARTESIAN_POINT('Ctrl Pts',(85.4110338039816,-6.12952335880773,-3.07457949793802));
#36098=CARTESIAN_POINT('Ctrl Pts',(85.5433748736098,-2.84244201074919,-5.8140229961449));
#36099=CARTESIAN_POINT('Ctrl Pts',(85.6426306758308,0.282630697465553,-6.48412322954603));
#36100=CARTESIAN_POINT('Ctrl Pts',(85.7418864780519,3.3375450925625,-5.54464901858413));
#36101=CARTESIAN_POINT('Ctrl Pts',(85.8742275476799,6.37379824136797,-2.52958330039638));
#36102=CARTESIAN_POINT('Ctrl Pts',(86.0396538847151,6.56392799824454,3.313282012274));
#36103=CARTESIAN_POINT('Ctrl Pts',(86.2381654891571,0.765233081136916,7.31263992198074));
#36104=CARTESIAN_POINT('Ctrl Pts',(86.4366770935993,-5.72732574435958,4.61064248397214));
#36105=CARTESIAN_POINT('Ctrl Pts',(86.6351886980413,-6.97653835085342,-2.321831410346));
#36106=CARTESIAN_POINT('Ctrl Pts',(86.8006150350767,-2.69726124705009,-6.30467108265544));
#36107=CARTESIAN_POINT('Ctrl Pts',(86.9329561047044,1.58159360772959,-6.2754204356491));
#36108=CARTESIAN_POINT('Ctrl Pts',(87.0322119069257,4.40104898481893,-4.77016792160538));
#36109=CARTESIAN_POINT('Ctrl Pts',(87.1314677091467,6.1280180343697,-2.08080151735183));
#36110=CARTESIAN_POINT('Ctrl Pts',(87.2638087787747,6.501043828168,2.18186269951808));
#36111=CARTESIAN_POINT('Ctrl Pts',(87.4292351158099,2.87499030196175,6.76737905120017));
#36112=CARTESIAN_POINT('Ctrl Pts',(87.6277467202519,-4.1354534267282,6.07933460605474));
#36113=CARTESIAN_POINT('Ctrl Pts',(87.8262583246941,-7.35048514532909,-0.175078340491695));
#36114=CARTESIAN_POINT('Ctrl Pts',(88.0247699291361,-3.8300746758159,-6.27642545057859));
#36115=CARTESIAN_POINT('Ctrl Pts',(88.1901962661713,2.00917170803365,-6.55647197377879));
#36116=CARTESIAN_POINT('Ctrl Pts',(88.3225373357994,5.25849341829804,-3.77234502052638));
#36117=CARTESIAN_POINT('Ctrl Pts',(88.4217931380204,6.44043681020296,-0.802812469304661));
#36118=CARTESIAN_POINT('Ctrl Pts',(88.5210489402415,6.02365017597241,2.36600476366407));
#36119=CARTESIAN_POINT('Ctrl Pts',(88.6533900098694,3.55723335538306,5.86260919306929));
#36120=CARTESIAN_POINT('Ctrl Pts',(88.8188163469047,-2.17207643043537,7.02460478883646));
#36121=CARTESIAN_POINT('Ctrl Pts',(89.0173279513466,-7.08257530082506,1.974186264048));
#36122=CARTESIAN_POINT('Ctrl Pts',(89.2158395557889,-5.50131724885063,-4.87809315455458));
#36123=CARTESIAN_POINT('Ctrl Pts',(89.4143511602309,1.12569445119592,-7.26607187285839));
#36124=CARTESIAN_POINT('Ctrl Pts',(89.5797774972661,5.76648339708804,-3.71103286517617));
#36125=CARTESIAN_POINT('Ctrl Pts',(89.7121185668941,6.45131090248977,0.512764686372355));
#36126=CARTESIAN_POINT('Ctrl Pts',(89.8113743691151,5.43739898593206,3.54378701883646));
#36127=CARTESIAN_POINT('Ctrl Pts',(89.9106301713363,3.07374429895899,5.69512387650968));
#36128=CARTESIAN_POINT('Ctrl Pts',(90.0429712409643,-1.06699388433329,6.77389251066956));
#36129=CARTESIAN_POINT('Ctrl Pts',(90.2083975779993,-6.19306663421924,3.96344725247069));
#36130=CARTESIAN_POINT('Ctrl Pts',(90.4069091824416,-6.68392896138932,-3.06355641960676));
#36131=CARTESIAN_POINT('Ctrl Pts',(90.6054207868836,-1.05335843212328,-7.27672455920159));
#36132=CARTESIAN_POINT('Ctrl Pts',(90.8039323913257,5.54969193399755,-4.82326734659396));
#36133=CARTESIAN_POINT('Ctrl Pts',(90.9693587283609,6.79974118846012,0.887477022389232));
#36134=CARTESIAN_POINT('Ctrl Pts',(91.1016997979888,4.59656587779412,4.55564727731113));
#36135=CARTESIAN_POINT('Ctrl Pts',(91.20095560021,1.86576486459037,6.21632171280966));
#36136=CARTESIAN_POINT('Ctrl Pts',(91.300211402431,-1.32818086979205,6.33389892256676));
#36137=CARTESIAN_POINT('Ctrl Pts',(91.432552472059,-5.18717929313224,4.48522760584228));
#36138=CARTESIAN_POINT('Ctrl Pts',(91.5979788090943,-7.28848744989553,-0.970020181085168));
#36139=CARTESIAN_POINT('Ctrl Pts',(91.7964904135362,-3.12783266756751,-6.6540925076761));
#36140=CARTESIAN_POINT('Ctrl Pts',(91.9950020179784,3.89220090559598,-6.23787274697798));
#36141=CARTESIAN_POINT('Ctrl Pts',(92.1935136224206,7.35204657094004,-0.101978810180762));
#36142=CARTESIAN_POINT('Ctrl Pts',(92.3589399594556,4.62083998930958,5.06674782168087));
#36143=CARTESIAN_POINT('Ctrl Pts',(92.4912810290838,0.570429324999648,6.44646805385352));
#36144=CARTESIAN_POINT('Ctrl Pts',(92.5905368313047,-2.58724594711247,5.9523014520636));
#36145=CARTESIAN_POINT('Ctrl Pts',(92.6897926335258,-5.10268096401501,3.98057621000437));
#36146=CARTESIAN_POINT('Ctrl Pts',(92.8221337031539,-6.85697076191429,0.0777667381484085));
#36147=CARTESIAN_POINT('Ctrl Pts',(92.9875600401889,-4.9408683261657,-5.44525560855407));
#36148=CARTESIAN_POINT('Ctrl Pts',(93.1860716446312,1.90583395511156,-7.10127321207659));
#36149=CARTESIAN_POINT('Ctrl Pts',(93.3845832490731,6.99910671440612,-2.25228539429799));
#36150=CARTESIAN_POINT('Ctrl Pts',(93.5830948535154,5.68133630187344,4.66748393505667));
#36151=CARTESIAN_POINT('Ctrl Pts',(93.7485211905503,0.259080310101639,6.85251582181516));
#36152=CARTESIAN_POINT('Ctrl Pts',(93.8808622601785,-3.72517479045193,5.29201405560826));
#36153=CARTESIAN_POINT('Ctrl Pts',(93.9801180623995,-5.81805651628024,2.87644790331024));
#36154=CARTESIAN_POINT('Ctrl Pts',(94.0793738646206,-6.46670364739967,-0.253148021681272));
#36155=CARTESIAN_POINT('Ctrl Pts',(94.2117149342486,-5.2875683157848,-4.36643069350914));
#36156=CARTESIAN_POINT('Ctrl Pts',(94.3771412712839,-0.259211159662201,
-7.34818331519461));
#36157=CARTESIAN_POINT('Ctrl Pts',(94.5756528757259,6.03919547739302,-4.19385291621541));
#36158=CARTESIAN_POINT('Ctrl Pts',(94.7741644801679,6.79967439427966,2.79726874447026));
#36159=CARTESIAN_POINT('Ctrl Pts',(94.9726760846102,1.32679513771092,7.23205386605656));
#36160=CARTESIAN_POINT('Ctrl Pts',(95.1381024216451,-4.22506743128341,5.40119439535534));
#36161=CARTESIAN_POINT('Ctrl Pts',(95.2704434912733,-6.26102756202529,1.63764277293116));
#36162=CARTESIAN_POINT('Ctrl Pts',(95.3696992934943,-6.30045034013798,-1.55822324412883));
#36163=CARTESIAN_POINT('Ctrl Pts',(95.4689550957154,-4.77589237691392,-4.36728657043583));
#36164=CARTESIAN_POINT('Ctrl Pts',(95.6012961653434,-1.22034872738306,-6.74795114674706));
#36165=CARTESIAN_POINT('Ctrl Pts',(95.7667225023786,4.544895881605,-5.77987109582617));
#36166=CARTESIAN_POINT('Ctrl Pts',(95.9652341068206,7.31967546924895,0.694719599470295));
#36167=CARTESIAN_POINT('Ctrl Pts',(96.1637457112627,3.388114636821,6.52540906800271));
#36168=CARTESIAN_POINT('Ctrl Pts',(96.3622573157049,-3.65451648904094,6.38024276108088));
#36169=CARTESIAN_POINT('Ctrl Pts',(96.5276836527399,-6.71331739379509,1.39837951410866));
#36170=CARTESIAN_POINT('Ctrl Pts',(96.6600247223681,-5.83920659045662,-2.79034162391308));
#36171=CARTESIAN_POINT('Ctrl Pts',(96.7592805245889,-3.80654732511578,-5.25679861025155));
#36172=CARTESIAN_POINT('Ctrl Pts',(96.8585363268103,-0.828976761999734,
-6.41834382938761));
#36173=CARTESIAN_POINT('Ctrl Pts',(96.990877396438,3.4233566459321,-5.94177793005278));
#36174=CARTESIAN_POINT('Ctrl Pts',(97.1563037334735,7.20202000654271,-1.48118070617854));
#36175=CARTESIAN_POINT('Ctrl Pts',(97.3548153379154,5.14238247907462,5.25511053508099));
#36176=CARTESIAN_POINT('Ctrl Pts',(97.5533269423575,-1.62397116860792,7.17098333149248));
#36177=CARTESIAN_POINT('Ctrl Pts',(97.7518385467997,-6.90945535086944,2.51444133225228));
#36178=CARTESIAN_POINT('Ctrl Pts',(97.9172648838347,-6.03023447391599,-3.26502188122914));
#36179=CARTESIAN_POINT('Ctrl Pts',(98.0496059534629,-2.65897769905643,-5.90018453779998));
#36180=CARTESIAN_POINT('Ctrl Pts',(98.1488617556838,0.485546955475345,-6.47209226766101));
#36181=CARTESIAN_POINT('Ctrl Pts',(98.2481175579051,3.50954275153179,-5.43741203692939));
#36182=CARTESIAN_POINT('Ctrl Pts',(98.3804586275328,6.44988784699202,-2.32874267718317));
#36183=CARTESIAN_POINT('Ctrl Pts',(98.5458849645682,6.45695091959748,3.51721100886858));
#36184=CARTESIAN_POINT('Ctrl Pts',(98.7443965690102,0.535857308578908,7.33301719906992));
#36185=CARTESIAN_POINT('Ctrl Pts',(98.9429081734524,-5.8689022478471,4.42902593153709));
#36186=CARTESIAN_POINT('Ctrl Pts',(99.1414197778944,-6.90040687703648,-2.5391678539131));
#36187=CARTESIAN_POINT('Ctrl Pts',(99.3068461149296,-2.49850315059143,-6.3860455449202));
#36188=CARTESIAN_POINT('Ctrl Pts',(99.4391871845576,1.77733710574879,-6.22281389700046));
#36189=CARTESIAN_POINT('Ctrl Pts',(99.5384429867787,4.54827162108827,-4.63000641769442));
#36190=CARTESIAN_POINT('Ctrl Pts',(99.6376987889997,6.19017426763678,-1.8878777821833));
#36191=CARTESIAN_POINT('Ctrl Pts',(99.7700398586277,6.4295287824728,2.38437734653381));
#36192=CARTESIAN_POINT('Ctrl Pts',(99.9354661956629,2.66165501182151,6.85409228541916));
#36193=CARTESIAN_POINT('Ctrl Pts',(100.133977800105,-4.32380380101862,5.94684832388633));
#36194=CARTESIAN_POINT('Ctrl Pts',(100.332489404547,-7.34139734791796,-0.405178080596634));
#36195=CARTESIAN_POINT('Ctrl Pts',(100.531001008989,-3.63164551501983,-6.39328861480798));
#36196=CARTESIAN_POINT('Ctrl Pts',(100.696427346024,2.21350682387351,-6.49033768273847));
#36197=CARTESIAN_POINT('Ctrl Pts',(100.828768415652,5.37404798958258,-3.60582143066423));
#36198=CARTESIAN_POINT('Ctrl Pts',(100.928024217873,6.46241869027549,-0.600731919134315));
#36199=CARTESIAN_POINT('Ctrl Pts',(101.027280020095,5.94660273312621,2.55347917918856));
#36200=CARTESIAN_POINT('Ctrl Pts',(101.159621089723,3.3718969584413,5.97113109862479));
#36201=CARTESIAN_POINT('Ctrl Pts',(101.325047426758,-2.39099155665315,6.95313942295208));
#36202=CARTESIAN_POINT('Ctrl Pts',(101.5235590312,-7.1409246333084,1.75142218737291));
#36203=CARTESIAN_POINT('Ctrl Pts',(101.722070635642,-5.34585817425296,-5.04797827627917));
#36204=CARTESIAN_POINT('Ctrl Pts',(101.920582240084,1.3526844941182,-7.22725626488847));
#36205=CARTESIAN_POINT('Ctrl Pts',(102.086008577119,5.87986878794746,-3.52863128306579));
#36206=CARTESIAN_POINT('Ctrl Pts',(102.218349646747,6.43208922602856,0.714540532497019));
#36207=CARTESIAN_POINT('Ctrl Pts',(102.317605448968,5.32375599492072,3.71232491487952));
#36208=CARTESIAN_POINT('Ctrl Pts',(102.416861251189,2.89388995296144,5.78858712677963));
#36209=CARTESIAN_POINT('Ctrl Pts',(102.549202320817,-1.27859977470671,6.73715654497048));
#36210=CARTESIAN_POINT('Ctrl Pts',(102.714628657853,-6.31414733833159,3.76756311809497));
#36211=CARTESIAN_POINT('Ctrl Pts',(102.913140262295,-6.58471335989169,-3.27136581033968));
#36212=CARTESIAN_POINT('Ctrl Pts',(103.111651866737,-0.82496606132839,-7.30614229910194));
#36213=CARTESIAN_POINT('Ctrl Pts',(103.310163471179,5.69801405622591,-4.64710923843941));
#36214=CARTESIAN_POINT('Ctrl Pts',(103.475589808214,6.76861424179842,1.09998042754471));
#36215=CARTESIAN_POINT('Ctrl Pts',(103.607930877842,4.45164816401902,4.69735761978553));
#36216=CARTESIAN_POINT('Ctrl Pts',(103.707186680063,1.67018130387269,6.27170061297181));
#36217=CARTESIAN_POINT('Ctrl Pts',(103.806442482284,-1.52587995074471,6.2891995008118));
#36218=CARTESIAN_POINT('Ctrl Pts',(103.938783551912,-5.32509326013816,4.32058762958816));
#36219=CARTESIAN_POINT('Ctrl Pts',(104.104209888947,-7.2545358971902,-1.19778853474281));
#36220=CARTESIAN_POINT('Ctrl Pts',(104.302721493389,-2.91792101694804,-6.7487792410007));
#36221=CARTESIAN_POINT('Ctrl Pts',(104.501233097831,4.08563531820164,-6.11292633132952));
#36222=CARTESIAN_POINT('Ctrl Pts',(104.699744702274,7.35163424685847,0.128305709641857));
#36223=CARTESIAN_POINT('Ctrl Pts',(104.865171039309,4.4599048978128,5.20896765575043));
#36224=CARTESIAN_POINT('Ctrl Pts',(104.997512108937,0.368273875481132,6.4611697294255));
#36225=CARTESIAN_POINT('Ctrl Pts',(105.096767911158,-2.77237751656084,5.86836069033733));
#36226=CARTESIAN_POINT('Ctrl Pts',(105.196023713379,-5.22483286318278,3.81882984829934));
#36227=CARTESIAN_POINT('Ctrl Pts',(105.328364783007,-6.85604302789201,-0.137002218719652));
#36228=CARTESIAN_POINT('Ctrl Pts',(105.493791120042,-4.76792304793109,-5.59731179744855));
#36229=CARTESIAN_POINT('Ctrl Pts',(105.692302724484,2.12728060596421,-7.03810766777042));
#36230=CARTESIAN_POINT('Ctrl Pts',(105.890814328926,7.06620582008108,-2.03199906838922));
#36231=CARTESIAN_POINT('Ctrl Pts',(106.089325933368,5.53238437901881,4.84311030515874));
#36232=CARTESIAN_POINT('Ctrl Pts',(106.254752270403,0.0443617744349961,
6.85726730780797));
#36233=CARTESIAN_POINT('Ctrl Pts',(106.387093340032,-3.88907072626489,5.1727633873222));
#36234=CARTESIAN_POINT('Ctrl Pts',(106.486349142253,-5.90528136083011,2.69283775413386));
#36235=CARTESIAN_POINT('Ctrl Pts',(106.585604944474,-6.4556038302783,-0.455527979344725));
#36236=CARTESIAN_POINT('Ctrl Pts',(106.717946014101,-5.14823859197666,-4.5298844173743));
#36237=CARTESIAN_POINT('Ctrl Pts',(106.883372351137,-0.0289675534008062,
-7.35267358327051));
#36238=CARTESIAN_POINT('Ctrl Pts',(107.081883955579,6.1675620574163,-4.00271286495399));
#36239=CARTESIAN_POINT('Ctrl Pts',(107.280395560021,6.70875004256005,3.00890426696354));
#36240=CARTESIAN_POINT('Ctrl Pts',(107.478907164463,1.09964973772579,7.26991658020799));
#36241=CARTESIAN_POINT('Ctrl Pts',(107.644333501498,-4.39210610522649,5.26648010085043));
#36242=CARTESIAN_POINT('Ctrl Pts',(107.776674571126,-6.30928449663211,1.44042764539869));
#36243=CARTESIAN_POINT('Ctrl Pts',(107.875930373347,-6.2484678151464,-1.75401181099146));
#36244=CARTESIAN_POINT('Ctrl Pts',(107.975186175568,-4.63696157612732,-4.51609008620458));
#36245=CARTESIAN_POINT('Ctrl Pts',(108.107527245197,-1.00805461892616,-6.77986084607601));
#36246=CARTESIAN_POINT('Ctrl Pts',(108.272953582231,4.72291868063634,-5.64086832996922));
#36247=CARTESIAN_POINT('Ctrl Pts',(108.471465186674,7.29544819300465,0.934110138162679));
#36248=CARTESIAN_POINT('Ctrl Pts',(108.636891523709,3.86681832161873,5.66141617959935));
#36249=CARTESIAN_POINT('Ctrl Pts',(108.769232593337,-0.340764604699964,
6.46373036659584));
#36250=CARTESIAN_POINT('Ctrl Pts',(108.868488395558,-3.38799745293929,5.53147877557648));
#36251=CARTESIAN_POINT('Ctrl Pts',(108.967744197779,-5.62418538167471,3.22542302469746));
#36252=CARTESIAN_POINT('Ctrl Pts',(109.033914732593,-6.19447498791001,1.17358721206399));
#36253=CARTESIAN_POINT('Ctrl Pts',(109.067,-6.21768400249992,0.139557183822751));
#36254=CARTESIAN_POINT('Ctrl Pts',(30.7922774969106,0.678777225891756,-6.42139103611685));
#36255=CARTESIAN_POINT('Ctrl Pts',(30.8253627643176,1.74668468978894,-6.30850719805494));
#36256=CARTESIAN_POINT('Ctrl Pts',(30.8915332991316,3.82068840904174,-5.54208840511827));
#36257=CARTESIAN_POINT('Ctrl Pts',(30.9907891013527,6.01455579796589,-3.03012972641587));
#36258=CARTESIAN_POINT('Ctrl Pts',(31.0900449035738,6.71725437222838,0.202938760700514));
#36259=CARTESIAN_POINT('Ctrl Pts',(31.2223859732018,5.52548610707363,4.48753452027612));
#36260=CARTESIAN_POINT('Ctrl Pts',(31.387812310237,0.339508912956707,7.62882085876798));
#36261=CARTESIAN_POINT('Ctrl Pts',(31.586323914679,-6.24246999589781,4.40195999752177));
#36262=CARTESIAN_POINT('Ctrl Pts',(31.7517502517141,-6.92842770696881,-1.62572047208448));
#36263=CARTESIAN_POINT('Ctrl Pts',(31.8840913213422,-4.27423691538049,-5.18596025794933));
#36264=CARTESIAN_POINT('Ctrl Pts',(31.9833471235632,-1.27783695201738,-6.61598549330334));
#36265=CARTESIAN_POINT('Ctrl Pts',(32.0826029257843,2.03264953710899,-6.40436604028605));
#36266=CARTESIAN_POINT('Ctrl Pts',(32.2149439954124,5.82666197580389,-4.09184779202466));
#36267=CARTESIAN_POINT('Ctrl Pts',(32.3803703324475,7.42761210931129,1.76261098900636));
#36268=CARTESIAN_POINT('Ctrl Pts',(32.5788819368895,2.53670467138675,7.2000873154729));
#36269=CARTESIAN_POINT('Ctrl Pts',(32.7773935413318,-4.67164414538107,6.03751153344729));
#36270=CARTESIAN_POINT('Ctrl Pts',(32.9759051457738,-7.60525981750663,-0.661897697190728));
#36271=CARTESIAN_POINT('Ctrl Pts',(33.1413314828089,-4.24456811261457,-5.71615983348691));
#36272=CARTESIAN_POINT('Ctrl Pts',(33.273672552437,0.083495628675871,-6.7187092468208));
#36273=CARTESIAN_POINT('Ctrl Pts',(33.3729283546581,3.29378569679711,-5.87870906545261));
#36274=CARTESIAN_POINT('Ctrl Pts',(33.4721841568791,5.68646072766973,-3.57941580085851));
#36275=CARTESIAN_POINT('Ctrl Pts',(33.6045252265072,7.09134406091902,0.635248297090446));
#36276=CARTESIAN_POINT('Ctrl Pts',(33.7699515635422,4.53564490764562,6.14055242947785));
#36277=CARTESIAN_POINT('Ctrl Pts',(33.9684631679845,-2.70979707674458,7.13670357848515));
#36278=CARTESIAN_POINT('Ctrl Pts',(34.1669747724264,-7.46509976895978,1.59618946747842));
#36279=CARTESIAN_POINT('Ctrl Pts',(34.3654863768686,-5.38171243595097,-5.4143905431608));
#36280=CARTESIAN_POINT('Ctrl Pts',(34.5309127139037,0.447487280130549,-7.10566462936179));
#36281=CARTESIAN_POINT('Ctrl Pts',(34.6632537835318,4.40035911681068,-5.07788139373532));
#36282=CARTESIAN_POINT('Ctrl Pts',(34.7625095857528,6.31021524910873,-2.36419966135741));
#36283=CARTESIAN_POINT('Ctrl Pts',(34.8617653879739,6.65366662094855,0.936354830793845));
#36284=CARTESIAN_POINT('Ctrl Pts',(34.994106457602,5.00636862977039,5.06231053686134));
#36285=CARTESIAN_POINT('Ctrl Pts',(35.159532794637,-0.499079050747831,7.61770126867609));
#36286=CARTESIAN_POINT('Ctrl Pts',(35.3580443990792,-6.67613314317957,3.70199726504512));
#36287=CARTESIAN_POINT('Ctrl Pts',(35.5565560035213,-6.73212444684914,-3.59917184207896));
#36288=CARTESIAN_POINT('Ctrl Pts',(35.7550676079633,-0.6158509347047,-7.60915107926013));
#36289=CARTESIAN_POINT('Ctrl Pts',(35.9204939449985,4.92814054280995,-5.13849643122668));
#36290=CARTESIAN_POINT('Ctrl Pts',(36.0528350146265,6.63852344254141,-1.03829015457345));
#36291=CARTESIAN_POINT('Ctrl Pts',(36.1520908168476,6.34573214413546,2.26714356729575));
#36292=CARTESIAN_POINT('Ctrl Pts',(36.2513466190686,4.4777196589499,5.00979706149147));
#36293=CARTESIAN_POINT('Ctrl Pts',(36.3836876886968,0.556412225615593,7.09796592129242));
#36294=CARTESIAN_POINT('Ctrl Pts',(36.5491140257318,-5.29804036325235,5.49629155263721));
#36295=CARTESIAN_POINT('Ctrl Pts',(36.747625630174,-7.48870223226711,-1.48151152026111));
#36296=CARTESIAN_POINT('Ctrl Pts',(36.946137234616,-2.81893174721201,-7.09430485056207));
#36297=CARTESIAN_POINT('Ctrl Pts',(37.1446488390581,4.44093494836871,-6.20939202391477));
#36298=CARTESIAN_POINT('Ctrl Pts',(37.3100751760933,7.08076833939991,-0.743931790193501));
#36299=CARTESIAN_POINT('Ctrl Pts',(37.4424162457213,5.74068710172808,3.49178343276199));
#36300=CARTESIAN_POINT('Ctrl Pts',(37.5416720479424,3.38356134522474,5.827501095969));
#36301=CARTESIAN_POINT('Ctrl Pts',(37.6409278501634,0.186523440322275,6.71663970654018));
#36302=CARTESIAN_POINT('Ctrl Pts',(37.7732689197915,-4.15639013967811,5.78058265155737));
#36303=CARTESIAN_POINT('Ctrl Pts',(37.9386952568266,-7.59423760000636,0.778465026161879));
#36304=CARTESIAN_POINT('Ctrl Pts',(38.1372068612687,-4.76365105858751,-5.96516270525666));
#36305=CARTESIAN_POINT('Ctrl Pts',(38.3357184657108,2.42590824614302,-7.23812867317666));
#36306=CARTESIAN_POINT('Ctrl Pts',(38.5342300701529,7.39984846791683,-1.87635155932356));
#36307=CARTESIAN_POINT('Ctrl Pts',(38.6996564071881,5.88848152056962,4.00206198935123));
#36308=CARTESIAN_POINT('Ctrl Pts',(38.8319974768161,2.13098288624362,6.37235842367635));
#36309=CARTESIAN_POINT('Ctrl Pts',(38.9312532790372,-1.17698455269417,6.63498031369624));
#36310=CARTESIAN_POINT('Ctrl Pts',(39.0305090812582,-4.19278538862937,5.25058002759297));
#36311=CARTESIAN_POINT('Ctrl Pts',(39.1628501508863,-6.90573748732343,1.73248507666748));
#36312=CARTESIAN_POINT('Ctrl Pts',(39.3282764879214,-6.30296026868749,-4.30710394275017));
#36313=CARTESIAN_POINT('Ctrl Pts',(39.5267880923636,0.211721730493496,-7.63090501952448));
#36314=CARTESIAN_POINT('Ctrl Pts',(39.7252996968055,6.52476300755405,-3.96270175554772));
#36315=CARTESIAN_POINT('Ctrl Pts',(39.9238113012478,6.86311573771183,3.34306668989407));
#36316=CARTESIAN_POINT('Ctrl Pts',(40.0892376382828,1.91450958570585,6.85750449004156));
#36317=CARTESIAN_POINT('Ctrl Pts',(40.221578707911,-2.4853855017414,6.24266760680046));
#36318=CARTESIAN_POINT('Ctrl Pts',(40.3208345101319,-5.18152965472103,4.30813263928398));
#36319=CARTESIAN_POINT('Ctrl Pts',(40.4200903123531,-6.59144629170504,1.30417626294528));
#36320=CARTESIAN_POINT('Ctrl Pts',(40.552431381981,-6.39285379686092,-3.1340285762355));
#36321=CARTESIAN_POINT('Ctrl Pts',(40.7178577190163,-2.03420042254427,-7.35802155223996));
#36322=CARTESIAN_POINT('Ctrl Pts',(40.9163693234582,5.08707838054148,-5.69185128568854));
#36323=CARTESIAN_POINT('Ctrl Pts',(41.1148809279005,7.54135690419678,1.18468289077305));
#36324=CARTESIAN_POINT('Ctrl Pts',(41.3133925323425,3.08428624104439,6.98323928457356));
#36325=CARTESIAN_POINT('Ctrl Pts',(41.4788188693776,-2.96386576801207,6.47350094569438));
#36326=CARTESIAN_POINT('Ctrl Pts',(41.6111599390057,-5.92767194115434,3.1639761850105));
#36327=CARTESIAN_POINT('Ctrl Pts',(41.7104157412268,-6.738349673723,-0.0538523449313299));
#36328=CARTESIAN_POINT('Ctrl Pts',(41.8096715434477,-5.87634552656026,-3.25831293674151));
#36329=CARTESIAN_POINT('Ctrl Pts',(41.9420126130759,-2.86002240110445,-6.52004498833256));
#36330=CARTESIAN_POINT('Ctrl Pts',(42.1074389501108,3.19550411174225,-6.93305170860172));
#36331=CARTESIAN_POINT('Ctrl Pts',(42.3059505545532,7.55932819127609,-1.06399943832004));
#36332=CARTESIAN_POINT('Ctrl Pts',(42.5044621589951,4.99545677214538,5.77243009016082));
#36333=CARTESIAN_POINT('Ctrl Pts',(42.7029737634373,-2.15154250073096,7.3245694337521));
#36334=CARTESIAN_POINT('Ctrl Pts',(42.8684001004724,-6.44212782189157,3.03145244249525));
#36335=CARTESIAN_POINT('Ctrl Pts',(43.0007411701004,-6.56975993316737,-1.40935955732047));
#36336=CARTESIAN_POINT('Ctrl Pts',(43.0999969723215,-5.1120117039375,-4.39039778826742));
#36337=CARTESIAN_POINT('Ctrl Pts',(43.1992527745426,-2.38529261979699,-6.28159367192785));
#36338=CARTESIAN_POINT('Ctrl Pts',(43.3315938441706,2.02386727969302,-6.82602930105693));
#36339=CARTESIAN_POINT('Ctrl Pts',(43.4970201812058,6.91567071255501,-3.23294774436825));
#36340=CARTESIAN_POINT('Ctrl Pts',(43.6955317856478,6.46059443970595,4.06647968073216));
#36341=CARTESIAN_POINT('Ctrl Pts',(43.8940433900899,0.0897313265003367,
7.63331420794476));
#36342=CARTESIAN_POINT('Ctrl Pts',(44.0925549945321,-6.37099482527689,4.20581471995643));
#36343=CARTESIAN_POINT('Ctrl Pts',(44.2579813315672,-6.8771654018304,-1.84263692043955));
#36344=CARTESIAN_POINT('Ctrl Pts',(44.3903224011952,-4.10833076915798,-5.31692187571454));
#36345=CARTESIAN_POINT('Ctrl Pts',(44.4895782034163,-1.07078853494371,-6.65294433419148));
#36346=CARTESIAN_POINT('Ctrl Pts',(44.5888340056373,2.23255892846622,-6.337485350846));
#36347=CARTESIAN_POINT('Ctrl Pts',(44.7211750752654,5.95169359014882,-3.90743626866535));
#36348=CARTESIAN_POINT('Ctrl Pts',(44.8866014123005,7.368913876263,1.99438231202681));
#36349=CARTESIAN_POINT('Ctrl Pts',(45.0851130167426,2.30991268916776,7.27597697059224));
#36350=CARTESIAN_POINT('Ctrl Pts',(45.2836246211847,-4.85838268646827,5.88826419074352));
#36351=CARTESIAN_POINT('Ctrl Pts',(45.4821362256269,-7.58082549814641,-0.899742901589314));
#36352=CARTESIAN_POINT('Ctrl Pts',(45.6475625626619,-4.06346923403625,-5.84627510204067));
#36353=CARTESIAN_POINT('Ctrl Pts',(45.7799036322901,0.293850439736193,-6.7128005973907));
#36354=CARTESIAN_POINT('Ctrl Pts',(45.879159434511,3.4762690362925,-5.77267788705827));
#36355=CARTESIAN_POINT('Ctrl Pts',(45.9784152367322,5.7957623606931,-3.39958506286211));
#36356=CARTESIAN_POINT('Ctrl Pts',(46.1107563063601,7.06797376310207,0.857007391333677));
#36357=CARTESIAN_POINT('Ctrl Pts',(46.2761826433955,4.34112411504214,6.27957752879176));
#36358=CARTESIAN_POINT('Ctrl Pts',(46.4746942478373,-2.9319586531779,7.04834420018078));
#36359=CARTESIAN_POINT('Ctrl Pts',(46.6732058522796,-7.51142440282901,1.3616317228796));
#36360=CARTESIAN_POINT('Ctrl Pts',(46.8717174567216,-5.20951740344347,-5.58026710342137));
#36361=CARTESIAN_POINT('Ctrl Pts',(47.0371437937567,0.669786645085241,-7.08816623921626));
#36362=CARTESIAN_POINT('Ctrl Pts',(47.1694848633848,4.55721837534439,-4.93759056835269));
#36363=CARTESIAN_POINT('Ctrl Pts',(47.2687406656058,6.38115692357772,-2.16543130047887));
#36364=CARTESIAN_POINT('Ctrl Pts',(47.3679964678269,6.62108067967075,1.14425983699188));
#36365=CARTESIAN_POINT('Ctrl Pts',(47.5003375374549,4.84538340573927,5.21660564314443));
#36366=CARTESIAN_POINT('Ctrl Pts',(47.6657638744901,-0.737387941134879,
7.59833610381744));
#36367=CARTESIAN_POINT('Ctrl Pts',(47.8642754789322,-6.78878943491683,3.4911137931223));
#36368=CARTESIAN_POINT('Ctrl Pts',(48.0627870833743,-6.61611203357758,-3.8082278118985));
#36369=CARTESIAN_POINT('Ctrl Pts',(48.2612986878164,-0.377262972701469,
-7.6247049235846));
#36370=CARTESIAN_POINT('Ctrl Pts',(48.4267250248515,5.08663912970787,-4.98164803542207));
#36371=CARTESIAN_POINT('Ctrl Pts',(48.5590660944796,6.66778231879769,-0.82989089065422));
#36372=CARTESIAN_POINT('Ctrl Pts',(48.6583218967007,6.27162264185577,2.46475269318842));
#36373=CARTESIAN_POINT('Ctrl Pts',(48.7575776989217,4.31863821441834,5.14756291017678));
#36374=CARTESIAN_POINT('Ctrl Pts',(48.8899187685498,0.333861537911319,7.11190911487227));
#36375=CARTESIAN_POINT('Ctrl Pts',(49.0553451055849,-5.46756213577111,5.32768400093223));
#36376=CARTESIAN_POINT('Ctrl Pts',(49.253856710027,-7.43863477210073,-1.71529887642388));
#36377=CARTESIAN_POINT('Ctrl Pts',(49.452368314469,-2.59538604019765,-7.17910222872708));
#36378=CARTESIAN_POINT('Ctrl Pts',(49.6508799189113,4.63320833659035,-6.06727558563615));
#36379=CARTESIAN_POINT('Ctrl Pts',(49.8163062559462,7.10059227460798,-0.521827686576112));
#36380=CARTESIAN_POINT('Ctrl Pts',(49.9486473255744,5.6285238898169,3.66984451482926));
#36381=CARTESIAN_POINT('Ctrl Pts',(50.0479031277954,3.19940956165385,5.93060155947232));
#36382=CARTESIAN_POINT('Ctrl Pts',(50.1471589300164,-0.0239043344667595,
6.71918659690707));
#36383=CARTESIAN_POINT('Ctrl Pts',(50.2794999996446,-4.33537461798565,5.64758724646426));
#36384=CARTESIAN_POINT('Ctrl Pts',(50.4449263366796,-7.61489113323075,0.540264334701967));
#36385=CARTESIAN_POINT('Ctrl Pts',(50.6434379411218,-4.57451143045198,-6.11141413102002));
#36386=CARTESIAN_POINT('Ctrl Pts',(50.8419495455638,2.65138552930593,-7.15860966132069));
#36387=CARTESIAN_POINT('Ctrl Pts',(51.040461150006,7.45497842904763,-1.64369983413683));
#36388=CARTESIAN_POINT('Ctrl Pts',(51.2058874870411,5.76026609022641,4.18450108788224));
#36389=CARTESIAN_POINT('Ctrl Pts',(51.3382285566691,1.93038284825529,6.43596628335045));
#36390=CARTESIAN_POINT('Ctrl Pts',(51.4374843588902,-1.3841863643057,6.59486804335672));
#36391=CARTESIAN_POINT('Ctrl Pts',(51.5367401611112,-4.35515461196362,5.11670482314096));
#36392=CARTESIAN_POINT('Ctrl Pts',(51.6690812307394,-6.95660450857366,1.51537734442372));
#36393=CARTESIAN_POINT('Ctrl Pts',(51.8345075677744,-6.16498895122,-4.50237312465798));
#36394=CARTESIAN_POINT('Ctrl Pts',(52.0330191722166,0.450585044043654,-7.62053217474022));
#36395=CARTESIAN_POINT('Ctrl Pts',(52.2315307766586,6.64565768313247,-3.75643068174953));
#36396=CARTESIAN_POINT('Ctrl Pts',(52.4300423811008,6.75505919226148,3.55635035272829));
#36397=CARTESIAN_POINT('Ctrl Pts',(52.5954687181358,1.698823028496,6.91409539293113));
#36398=CARTESIAN_POINT('Ctrl Pts',(52.727809787764,-2.67966005093835,6.16177425362753));
#36399=CARTESIAN_POINT('Ctrl Pts',(52.8270655899849,-5.31390053926433,4.14375644303857));
#36400=CARTESIAN_POINT('Ctrl Pts',(52.9263213922061,-6.62905466770849,1.09712084739758));
#36401=CARTESIAN_POINT('Ctrl Pts',(53.0586624618341,-6.29157407007032,-3.33268818006107));
#36402=CARTESIAN_POINT('Ctrl Pts',(53.2240887988692,-1.80278111855577,-7.41811517576303));
#36403=CARTESIAN_POINT('Ctrl Pts',(53.4226004033114,5.26282771129787,-5.52975424312528));
#36404=CARTESIAN_POINT('Ctrl Pts',(53.6211120077534,7.50055901634054,1.42026474664386));
#36405=CARTESIAN_POINT('Ctrl Pts',(53.8196236121956,2.864088485346,7.0764008980848));
#36406=CARTESIAN_POINT('Ctrl Pts',(53.9850499492306,-3.16513435150749,6.37751043288894));
#36407=CARTESIAN_POINT('Ctrl Pts',(54.1173910188587,-6.02384681155226,2.97679517807551));
#36408=CARTESIAN_POINT('Ctrl Pts',(54.2166468210798,-6.73335837962768,-0.264842088639801));
#36409=CARTESIAN_POINT('Ctrl Pts',(54.3159026233008,-5.77142707271232,-3.44073676494229));
#36410=CARTESIAN_POINT('Ctrl Pts',(54.448243692929,-2.65443989208741,-6.60641079891305));
#36411=CARTESIAN_POINT('Ctrl Pts',(54.6136700299639,3.41105024174233,-6.82958188841868));
#36412=CARTESIAN_POINT('Ctrl Pts',(54.8121816344061,7.58894055686031,-0.826751917208314));
#36413=CARTESIAN_POINT('Ctrl Pts',(55.0106932388483,4.81223901059941,5.926035201805));
#36414=CARTESIAN_POINT('Ctrl Pts',(55.2092048432903,-2.37986130163657,7.25359998257966));
#36415=CARTESIAN_POINT('Ctrl Pts',(55.3746311803254,-6.53390029971636,2.82822588526208));
#36416=CARTESIAN_POINT('Ctrl Pts',(55.5069722499535,-6.52240266402268,-1.6144049769534));
#36417=CARTESIAN_POINT('Ctrl Pts',(55.6062280521746,-4.97201609009227,-4.54833072679206));
#36418=CARTESIAN_POINT('Ctrl Pts',(55.7054838543956,-2.18741021583949,-6.3532099358437));
#36419=CARTESIAN_POINT('Ctrl Pts',(55.8378249240237,2.23663656514571,-6.75930260161158));
#36420=CARTESIAN_POINT('Ctrl Pts',(56.0032512610587,7.01352090499909,-3.01479303393244));
#36421=CARTESIAN_POINT('Ctrl Pts',(56.2017628655009,6.33008112735583,4.26680330332445));
#36422=CARTESIAN_POINT('Ctrl Pts',(56.400274469943,-0.149355282209104,7.63238039590815));
#36423=CARTESIAN_POINT('Ctrl Pts',(56.5987860743851,-6.49957817086878,4.00423976842957));
#36424=CARTESIAN_POINT('Ctrl Pts',(56.7642124114202,-6.81608897840635,-2.05709645450743));
#36425=CARTESIAN_POINT('Ctrl Pts',(56.8965534810482,-3.93981266455918,-5.44296942021918));
#36426=CARTESIAN_POINT('Ctrl Pts',(56.9958092832694,-0.861921731593391,
-6.68321384732111));
#36427=CARTESIAN_POINT('Ctrl Pts',(57.0950650854903,2.4299267624953,-6.26446293549345));
#36428=CARTESIAN_POINT('Ctrl Pts',(57.2274061551185,6.07113865401073,-3.71913837178403));
#36429=CARTESIAN_POINT('Ctrl Pts',(57.3928324921535,7.30284425781954,2.2241668706146));
#36430=CARTESIAN_POINT('Ctrl Pts',(57.5913440965957,2.08092744393462,7.34474495685501));
#36431=CARTESIAN_POINT('Ctrl Pts',(57.7898557010377,-5.04039499077211,5.73323258251105));
#36432=CARTESIAN_POINT('Ctrl Pts',(57.98836730548,-7.54893134867238,-1.13670049500218));
#36433=CARTESIAN_POINT('Ctrl Pts',(58.1537936425149,-3.87839606375768,-5.97065815110265));
#36434=CARTESIAN_POINT('Ctrl Pts',(58.2861347121431,0.503922387441998,-6.70030612499883));
#36435=CARTESIAN_POINT('Ctrl Pts',(58.3853905143641,3.65533954142928,-5.66098482927496));
#36436=CARTESIAN_POINT('Ctrl Pts',(58.4846463165852,5.89938018465789,-3.21641934115063));
#36437=CARTESIAN_POINT('Ctrl Pts',(58.6169873862132,7.03766943783764,1.07792563214058));
#36438=CARTESIAN_POINT('Ctrl Pts',(58.7824137232483,4.14234559697983,6.41244301943407));
#36439=CARTESIAN_POINT('Ctrl Pts',(58.9809253276904,-3.15124450627053,6.95307094526344));
#36440=CARTESIAN_POINT('Ctrl Pts',(59.1794369321325,-7.55038082733314,1.12573836676515));
#36441=CARTESIAN_POINT('Ctrl Pts',(59.3779485365747,-5.03221237337296,-5.74066992184528));
#36442=CARTESIAN_POINT('Ctrl Pts',(59.5433748736097,0.891429051179542,-7.06371495966627));
#36443=CARTESIAN_POINT('Ctrl Pts',(59.6757159432379,4.70960737511203,-4.79245639662505));
#36444=CARTESIAN_POINT('Ctrl Pts',(59.7749717454588,6.44583924427009,-1.96453883581995));
#36445=CARTESIAN_POINT('Ctrl Pts',(59.8742275476801,6.5820000239748,1.35104242185723));
#36446=CARTESIAN_POINT('Ctrl Pts',(60.0065686173079,4.67964528192059,5.36578370977611));
#36447=CARTESIAN_POINT('Ctrl Pts',(60.1719949543433,-0.974973519581309,
7.57151762584112));
#36448=CARTESIAN_POINT('Ctrl Pts',(60.3705065587851,-6.89478650842269,3.276805839753));
#36449=CARTESIAN_POINT('Ctrl Pts',(60.5690181632275,-6.49360978533135,-4.01354823865563));
#36450=CARTESIAN_POINT('Ctrl Pts',(60.7675297676693,-0.138304947903981,
-7.63277958961821));
#36451=CARTESIAN_POINT('Ctrl Pts',(60.9329561047046,5.24014816196206,-4.81991307238892));
#36452=CARTESIAN_POINT('Ctrl Pts',(61.0652971743326,6.69050067549388,-0.620677575298068));
#36453=CARTESIAN_POINT('Ctrl Pts',(61.1645529765537,6.19136121838743,2.65994410916198));
#36454=CARTESIAN_POINT('Ctrl Pts',(61.2638087787748,4.15532055811943,5.2802794434132));
#36455=CARTESIAN_POINT('Ctrl Pts',(61.3961498484028,0.110983360806127,7.11887613871208));
#36456=CARTESIAN_POINT('Ctrl Pts',(61.5615761854379,-5.63172070117528,5.15385045051374));
#36457=CARTESIAN_POINT('Ctrl Pts',(61.76008778988,-7.38127065249784,-1.94740367226242));
#36458=CARTESIAN_POINT('Ctrl Pts',(61.9585993943222,-2.36929448321922,-7.25685752650235));
#36459=CARTESIAN_POINT('Ctrl Pts',(62.1571109987642,4.82093694685279,-5.91920767305697));
#36460=CARTESIAN_POINT('Ctrl Pts',(62.3225373357993,7.11345114092422,-0.299211714983929));
#36461=CARTESIAN_POINT('Ctrl Pts',(62.4548784054274,5.5108395811942,3.8443057957979));
#36462=CARTESIAN_POINT('Ctrl Pts',(62.5541342076485,3.01211943311833,6.02788461411204));
#36463=CARTESIAN_POINT('Ctrl Pts',(62.6533900098696,-0.234308661164597,
6.71514254447107));
#36464=CARTESIAN_POINT('Ctrl Pts',(62.7857310794975,-4.51010646753767,5.50905204515032));
#36465=CARTESIAN_POINT('Ctrl Pts',(62.9511574165328,-7.62807511471915,0.301533690504745));
#36466=CARTESIAN_POINT('Ctrl Pts',(63.1496690209747,-4.38088460096325,-6.25167078637463));
#36467=CARTESIAN_POINT('Ctrl Pts',(63.348180625417,2.87426203183569,-7.07206867051746));
#36468=CARTESIAN_POINT('Ctrl Pts',(63.546692229859,7.50279569901947,-1.40943578111309));
#36469=CARTESIAN_POINT('Ctrl Pts',(63.7121185668941,5.62640033543055,4.36283555158418));
#36470=CARTESIAN_POINT('Ctrl Pts',(63.8444596365222,1.72788927110751,6.49326101493335));
#36471=CARTESIAN_POINT('Ctrl Pts',(63.9437154387432,-1.59003040842209,6.54828677599809));
#36472=CARTESIAN_POINT('Ctrl Pts',(64.0429712409644,-4.51325180407346,4.97781057235896));
#36473=CARTESIAN_POINT('Ctrl Pts',(64.1753123105923,-7.000647700517,1.29678315764307));
#36474=CARTESIAN_POINT('Ctrl Pts',(64.3407386476275,-6.02097031106359,-4.69322586667211));
#36475=CARTESIAN_POINT('Ctrl Pts',(64.5392502520696,0.689006372509483,-7.60268424484393));
#36476=CARTESIAN_POINT('Ctrl Pts',(64.7377618565116,6.76003354143388,-3.54647487328871));
#36477=CARTESIAN_POINT('Ctrl Pts',(64.9362734609539,6.64037651608413,3.76614554245524));
#36478=CARTESIAN_POINT('Ctrl Pts',(65.1016997979887,1.48147007234857,6.96390416428755));
#36479=CARTESIAN_POINT('Ctrl Pts',(65.2340408676171,-2.8713060846355,6.07483673111265));
#36480=CARTESIAN_POINT('Ctrl Pts',(65.3332966698379,-5.44105894547704,3.97531557893542));
#36481=CARTESIAN_POINT('Ctrl Pts',(65.4325524720591,-6.66016051256749,0.888989250902352));
#36482=CARTESIAN_POINT('Ctrl Pts',(65.5648935416871,-6.1841228514889,-3.52807870413704));
#36483=CARTESIAN_POINT('Ctrl Pts',(65.7303198787223,-1.5695934417308,-7.4709322676986));
#36484=CARTESIAN_POINT('Ctrl Pts',(65.9288314831644,5.43341466181217,-5.36223298852923));
#36485=CARTESIAN_POINT('Ctrl Pts',(66.1273430876064,7.4524037266176,1.65445344554935));
#36486=CARTESIAN_POINT('Ctrl Pts',(66.3258546920486,2.64108130591095,7.16262117174185));
#36487=CARTESIAN_POINT('Ctrl Pts',(66.4912810290836,-3.36329821134536,6.27526413322609));
#36488=CARTESIAN_POINT('Ctrl Pts',(66.6236220987118,-6.11411280714021,2.78669419017976));
#36489=CARTESIAN_POINT('Ctrl Pts',(66.7228779009328,-6.7217622422898,-0.475572041781676));
#36490=CARTESIAN_POINT('Ctrl Pts',(66.8221337031539,-5.6608473448675,-3.61978553310384));
#36491=CARTESIAN_POINT('Ctrl Pts',(66.9544747727819,-2.44625360979039,-6.68629627682944));
#36492=CARTESIAN_POINT('Ctrl Pts',(67.1199011098171,3.62325043248716,-6.71941286407468));
#36493=CARTESIAN_POINT('Ctrl Pts',(67.3184127142591,7.61110881438817,-0.588693378977541));
#36494=CARTESIAN_POINT('Ctrl Pts',(67.5169243187013,4.62430087878972,6.07382730138981));
#36495=CARTESIAN_POINT('Ctrl Pts',(67.7154359231433,-2.60584570588013,7.17551553766098));
#36496=CARTESIAN_POINT('Ctrl Pts',(67.8808622601786,-6.6192635106055,2.6222247966042));
#36497=CARTESIAN_POINT('Ctrl Pts',(68.0132033298065,-6.46864758360768,-1.81786640520943));
#36498=CARTESIAN_POINT('Ctrl Pts',(68.1124591320277,-4.82714313111536,-4.70180301706438));
#36499=CARTESIAN_POINT('Ctrl Pts',(68.2117149342486,-1.98738256811678,-6.41859263889639));
#36500=CARTESIAN_POINT('Ctrl Pts',(68.3440560038768,2.44721280412095,-6.6859490868509));
#36501=CARTESIAN_POINT('Ctrl Pts',(68.5094823409118,7.10448960071639,-2.79367398074271));
#36502=CARTESIAN_POINT('Ctrl Pts',(68.7079939453539,6.1933616077837,4.46292976341907));
#36503=CARTESIAN_POINT('Ctrl Pts',(68.906505549796,-0.388301013108626,7.6239815918582));
#36504=CARTESIAN_POINT('Ctrl Pts',(69.1050171542382,-6.6217748926354,3.79869417354387));
#36505=CARTESIAN_POINT('Ctrl Pts',(69.2704434912732,-6.74834606556275,-2.26946287551695));
#36506=CARTESIAN_POINT('Ctrl Pts',(69.4027845609014,-3.76740267812313,-5.56378310329283));
#36507=CARTESIAN_POINT('Ctrl Pts',(69.5020403631223,-0.652269010159462,
-6.70669787709258));
#36508=CARTESIAN_POINT('Ctrl Pts',(69.6012961653433,2.62502096323833,-6.18571980719947));
#36509=CARTESIAN_POINT('Ctrl Pts',(69.7336372349716,6.18439098099528,-3.52627587749464));
#36510=CARTESIAN_POINT('Ctrl Pts',(69.8990635720066,7.23009515188822,2.44990214044399));
#36511=CARTESIAN_POINT('Ctrl Pts',(70.0975751764487,1.84909688725878,7.4094104631578));
#36512=CARTESIAN_POINT('Ctrl Pts',(70.2960867808908,-5.21599118824087,5.56690523187216));
#36513=CARTESIAN_POINT('Ctrl Pts',(70.4945983853329,-7.51246959013067,-1.36166401884761));
#36514=CARTESIAN_POINT('Ctrl Pts',(70.6931099897751,-2.91938464087065,-7.05530449130318));
#36515=CARTESIAN_POINT('Ctrl Pts',(70.8585363268101,3.12150592612419,-6.40096939299454));
#36516=CARTESIAN_POINT('Ctrl Pts',(70.9908773964382,5.99347114250277,-3.02271415117323));
#36517=CARTESIAN_POINT('Ctrl Pts',(71.1232184660663,7.0011077487275,1.29209572680489));
#36518=CARTESIAN_POINT('Ctrl Pts',(71.2886448031014,3.94386244225407,6.54279353784522));
#36519=CARTESIAN_POINT('Ctrl Pts',(71.4871564075435,-3.3774734808755,6.848092155856));
#36520=CARTESIAN_POINT('Ctrl Pts',(71.6525827445786,-6.86299555174514,1.88573569827787));
#36521=CARTESIAN_POINT('Ctrl Pts',(71.7849238142066,-6.23324656129562,-2.51205469018619));
#36522=CARTESIAN_POINT('Ctrl Pts',(71.8841796164277,-4.28543654678419,-5.19968989554554));
#36523=CARTESIAN_POINT('Ctrl Pts',(71.9834354186487,-1.27646022566982,-6.59696982891652));
#36524=CARTESIAN_POINT('Ctrl Pts',(72.1157764882769,3.16136854322932,-6.37945219356449));
#36525=CARTESIAN_POINT('Ctrl Pts',(72.2812028253119,7.36647591564621,-2.00294299890811));
#36526=CARTESIAN_POINT('Ctrl Pts',(72.4797144297541,5.67025131620974,5.11122006794026));
#36527=CARTESIAN_POINT('Ctrl Pts',(72.6782260341961,-1.2167407171549,7.53625156965662));
#36528=CARTESIAN_POINT('Ctrl Pts',(72.8767376386383,-6.99625824654105,3.05459682075844));
#36529=CARTESIAN_POINT('Ctrl Pts',(73.0421639756734,-6.46086195001876,-2.9913395844494));
#36530=CARTESIAN_POINT('Ctrl Pts',(73.1745050453014,-3.13876262892288,-5.94105822926261));
#36531=CARTESIAN_POINT('Ctrl Pts',(73.2737608475225,0.0824736114544292,
-6.73806046974298));
#36532=CARTESIAN_POINT('Ctrl Pts',(73.3730166497436,3.28324711120387,-5.86245117769648));
#36533=CARTESIAN_POINT('Ctrl Pts',(73.5053577193716,6.53213460317267,-2.83229985644436));
#36534=CARTESIAN_POINT('Ctrl Pts',(73.6707840564068,6.91941525444984,3.22492663651895));
#36535=CARTESIAN_POINT('Ctrl Pts',(73.8692956608488,1.0318779221477,7.56377977437356));
#36536=CARTESIAN_POINT('Ctrl Pts',(74.0678072652908,-5.79359835649274,4.97089069632919));
#36537=CARTESIAN_POINT('Ctrl Pts',(74.2663188697332,-7.31536376747108,-2.18263753902794));
#36538=CARTESIAN_POINT('Ctrl Pts',(74.4317452067681,-3.00405918604541,-6.45494716469223));
#36539=CARTESIAN_POINT('Ctrl Pts',(74.5640862763963,1.43725486725013,-6.56371376365296));
#36540=CARTESIAN_POINT('Ctrl Pts',(74.6633420786172,4.41207377938405,-5.0933153676217));
#36541=CARTESIAN_POINT('Ctrl Pts',(74.7625978808384,6.29166960657197,-2.35858717292915));
#36542=CARTESIAN_POINT('Ctrl Pts',(74.8949389504664,6.81737041885829,2.05284568347206));
#36543=CARTESIAN_POINT('Ctrl Pts',(75.0603652875016,3.20354111649094,6.92934173083288));
#36544=CARTESIAN_POINT('Ctrl Pts',(75.2588768919436,-4.09388730274326,6.44326192662146));
#36545=CARTESIAN_POINT('Ctrl Pts',(75.4573884963858,-7.63362651069499,0.0573045431487054));
#36546=CARTESIAN_POINT('Ctrl Pts',(75.6559001008278,-4.17871307428154,-6.38880345308914));
#36547=CARTESIAN_POINT('Ctrl Pts',(75.8213264378629,1.87183418264915,-6.86927591359667));
#36548=CARTESIAN_POINT('Ctrl Pts',(75.953667507491,5.33432590669687,-4.08570765755734));
#36549=CARTESIAN_POINT('Ctrl Pts',(76.052923309712,6.657432968585,-1.04251746688282));
#36550=CARTESIAN_POINT('Ctrl Pts',(76.1521791119332,6.32794436086292,2.25946013624946));
#36551=CARTESIAN_POINT('Ctrl Pts',(76.2845201815611,3.8821184881069,5.96823850301648));
#36552=CARTESIAN_POINT('Ctrl Pts',(76.4499465185964,-2.02566713052125,7.36037534359628));
#36553=CARTESIAN_POINT('Ctrl Pts',(76.6484581230383,-7.28572372703915,2.27898382650516));
#36554=CARTESIAN_POINT('Ctrl Pts',(76.8469697274806,-5.86757287326853,-4.8833519313097));
#36555=CARTESIAN_POINT('Ctrl Pts',(77.0454813319226,0.931937787573207,-7.57693503221458));
#36556=CARTESIAN_POINT('Ctrl Pts',(77.2109076689577,5.86348378704247,-4.03859785863803));
#36557=CARTESIAN_POINT('Ctrl Pts',(77.3432487385858,6.71149176708757,0.322363461909703));
#36558=CARTESIAN_POINT('Ctrl Pts',(77.4425045408068,5.75785876877837,3.50075974600101));
#36559=CARTESIAN_POINT('Ctrl Pts',(77.5417603430279,3.37493425326742,5.810151351504));
#36560=CARTESIAN_POINT('Ctrl Pts',(77.674101412656,-0.887024091918348,7.06426946294214));
#36561=CARTESIAN_POINT('Ctrl Pts',(77.8395277496911,-6.2979617696608,4.31440958535449));
#36562=CARTESIAN_POINT('Ctrl Pts',(78.0380393541331,-7.03582577797349,-2.96187324681027));
#36563=CARTESIAN_POINT('Ctrl Pts',(78.2365509585753,-1.32971124612974,-7.51714078024904));
#36564=CARTESIAN_POINT('Ctrl Pts',(78.4350625630174,5.60234654932029,-5.18576567766284));
#36565=CARTESIAN_POINT('Ctrl Pts',(78.6004889000525,7.08525706213391,0.699890811613769));
#36566=CARTESIAN_POINT('Ctrl Pts',(78.7328299696805,4.91818716080672,4.57815191890112));
#36567=CARTESIAN_POINT('Ctrl Pts',(78.8320857719017,2.13830489652176,6.39029800321771));
#36568=CARTESIAN_POINT('Ctrl Pts',(78.9313415741226,-1.17237556419702,6.61616017624541));
#36569=CARTESIAN_POINT('Ctrl Pts',(79.0636826437508,-5.23714154545479,4.82317978283739));
#36570=CARTESIAN_POINT('Ctrl Pts',(79.2291089807858,-7.59513515642661,-0.769658676245189));
#36571=CARTESIAN_POINT('Ctrl Pts',(79.4276205852279,-3.46224382358131,-6.80355827594947));
#36572=CARTESIAN_POINT('Ctrl Pts',(79.6261321896702,3.83629839660047,-6.59987515945624));
#36573=CARTESIAN_POINT('Ctrl Pts',(79.8246437941121,7.62623872496982,-0.344870166986757));
#36574=CARTESIAN_POINT('Ctrl Pts',(79.9900701311472,4.95999527493247,5.10775505064086));
#36575=CARTESIAN_POINT('Ctrl Pts',(80.1224112007753,0.8015589650237,6.67124749704671));
#36576=CARTESIAN_POINT('Ctrl Pts',(80.2216670029964,-2.49137202416728,6.26109589749385));
#36577=CARTESIAN_POINT('Ctrl Pts',(80.3209228052174,-5.16586184567227,4.29673263453635));
#36578=CARTESIAN_POINT('Ctrl Pts',(80.4532638748456,-7.11326317567643,0.303647457203498));
#36579=CARTESIAN_POINT('Ctrl Pts',(80.6186902118805,-5.30440997458895,-5.49014456492613));
#36580=CARTESIAN_POINT('Ctrl Pts',(80.8172018163229,1.74688238419706,-7.43128114418698));
#36581=CARTESIAN_POINT('Ctrl Pts',(81.0157134207648,7.19006253712243,-2.56486612134739));
#36582=CARTESIAN_POINT('Ctrl Pts',(81.214225025207,6.04753918347326,4.65894004540328));
#36583=CARTESIAN_POINT('Ctrl Pts',(81.3796513622421,0.491659983350608,7.10274490922151));
#36584=CARTESIAN_POINT('Ctrl Pts',(81.5119924318702,-3.6937211183203,5.61288377229892));
#36585=CARTESIAN_POINT('Ctrl Pts',(81.6112482340912,-5.94413899720338,3.17418776734193));
#36586=CARTESIAN_POINT('Ctrl Pts',(81.7105040363123,-6.7190244278375,-0.0524469196936317));
#36587=CARTESIAN_POINT('Ctrl Pts',(81.8428451059403,-5.62911981515396,-4.3593261969415));
#36588=CARTESIAN_POINT('Ctrl Pts',(82.0082714429754,-0.507911746828754,
-7.61711744557876));
#36589=CARTESIAN_POINT('Ctrl Pts',(82.2067830474175,6.13079130792516,-4.54850914551527));
#36590=CARTESIAN_POINT('Ctrl Pts',(82.4052946518595,7.14728210617843,2.68177105713156));
#36591=CARTESIAN_POINT('Ctrl Pts',(82.603806256302,1.61201659234397,7.46189352834217));
#36592=CARTESIAN_POINT('Ctrl Pts',(82.7692325933366,-4.20893268274398,5.74243854619525));
#36593=CARTESIAN_POINT('Ctrl Pts',(82.901573662965,-6.44410839326842,1.903025737364));
#36594=CARTESIAN_POINT('Ctrl Pts',(83.0008294651858,-6.58892857939596,-1.41218857665568));
#36595=CARTESIAN_POINT('Ctrl Pts',(83.1000852674072,-5.09815815725061,-4.37685084791804));
#36596=CARTESIAN_POINT('Ctrl Pts',(83.2324263370349,-1.48581233031733,-6.96297899636189));
#36597=CARTESIAN_POINT('Ctrl Pts',(83.3978526740704,4.5285210959042,-6.14580744949412));
#36598=CARTESIAN_POINT('Ctrl Pts',(83.5963642785122,7.61854935282431,0.482952654767742));
#36599=CARTESIAN_POINT('Ctrl Pts',(83.7948758829545,3.7281663355713,6.66155486973422));
#36600=CARTESIAN_POINT('Ctrl Pts',(83.9933874873964,-3.58501345126855,6.73989102853529));
#36601=CARTESIAN_POINT('Ctrl Pts',(84.1588138244318,-6.92124953323499,1.66943693603405));
#36602=CARTESIAN_POINT('Ctrl Pts',(84.2911548940596,-6.15033558364338,-2.7058108119069));
#36603=CARTESIAN_POINT('Ctrl Pts',(84.3904106962809,-4.12114584631622,-5.33145508410299));
#36604=CARTESIAN_POINT('Ctrl Pts',(84.4896664985016,-1.06895102396886,-6.63365537615708));
#36605=CARTESIAN_POINT('Ctrl Pts',(84.62200756813,3.3593844327698,-6.27736019498358));
#36606=CARTESIAN_POINT('Ctrl Pts',(84.7874339051648,7.42570637776451,-1.77125303486947));
#36607=CARTESIAN_POINT('Ctrl Pts',(84.9859455096072,5.50734809616266,5.28627037294353));
#36608=CARTESIAN_POINT('Ctrl Pts',(85.1844571140491,-1.4521139677821,7.49445812135466));
#36609=CARTESIAN_POINT('Ctrl Pts',(85.3829687184914,-7.08850356895284,2.83400241271063));
#36610=CARTESIAN_POINT('Ctrl Pts',(85.5483950555264,-6.36400754352169,-3.19219716977184));
#36611=CARTESIAN_POINT('Ctrl Pts',(85.6807361251545,-2.9511792907089,-6.03643775213103));
#36612=CARTESIAN_POINT('Ctrl Pts',(85.7799919273754,0.293442701073721,-6.73217259000419));
#36613=CARTESIAN_POINT('Ctrl Pts',(85.8792477295966,3.46522248184149,-5.75675890520026));
#36614=CARTESIAN_POINT('Ctrl Pts',(86.0115887992246,6.61762713256751,-2.62635220772195));
#36615=CARTESIAN_POINT('Ctrl Pts',(86.1770151362598,6.81503028060682,3.44003122031167));
#36616=CARTESIAN_POINT('Ctrl Pts',(86.3755267407018,0.794506981347646,7.5923840896491));
#36617=CARTESIAN_POINT('Ctrl Pts',(86.574038345144,-5.94642390732348,4.78702206205264));
#36618=CARTESIAN_POINT('Ctrl Pts',(86.7725499495861,-7.24342499302197,-2.41065279390719));
#36619=CARTESIAN_POINT('Ctrl Pts',(86.9379762866213,-2.80044465421751,-6.54585552264672));
#36620=CARTESIAN_POINT('Ctrl Pts',(87.0703173562492,1.64209728247714,-6.51548589562918));
#36621=CARTESIAN_POINT('Ctrl Pts',(87.1695731584704,4.56941058859847,-4.95265012626795));
#36622=CARTESIAN_POINT('Ctrl Pts',(87.2688289606913,6.36244463307709,-2.16040233111586));
#36623=CARTESIAN_POINT('Ctrl Pts',(87.4011700303195,6.7497404841074,2.26532959674766));
#36624=CARTESIAN_POINT('Ctrl Pts',(87.5665963673546,2.98497271291811,7.02626432931763));
#36625=CARTESIAN_POINT('Ctrl Pts',(87.7651079717966,-4.29365470412399,6.31189882602065));
#36626=CARTESIAN_POINT('Ctrl Pts',(87.9636195762388,-7.63167707750089,-0.181775941517044));
#36627=CARTESIAN_POINT('Ctrl Pts',(88.1621311806808,-3.97659372553301,-6.51652935728508));
#36628=CARTESIAN_POINT('Ctrl Pts',(88.327557517716,2.08603233198955,-6.80728902681484));
#36629=CARTESIAN_POINT('Ctrl Pts',(88.459898587344,5.45965645656968,-3.91665562916875));
#36630=CARTESIAN_POINT('Ctrl Pts',(88.5591543895652,6.68681495190187,-0.833523964525788));
#36631=CARTESIAN_POINT('Ctrl Pts',(88.658410191786,6.25408419470987,2.45651599358564));
#36632=CARTESIAN_POINT('Ctrl Pts',(88.7907512614142,3.69331489294256,6.08688260822147));
#36633=CARTESIAN_POINT('Ctrl Pts',(88.9561775984493,-2.25516895510891,7.29333020685474));
#36634=CARTESIAN_POINT('Ctrl Pts',(89.1546892028914,-7.35351837386254,2.04970852401823));
#36635=CARTESIAN_POINT('Ctrl Pts',(89.3532008073335,-5.71176948378593,-5.06470402612628));
#36636=CARTESIAN_POINT('Ctrl Pts',(89.5517124117756,1.16875775810838,-7.54403458536402));
#36637=CARTESIAN_POINT('Ctrl Pts',(89.7171387488108,5.98707953138472,-3.85299798463139));
#36638=CARTESIAN_POINT('Ctrl Pts',(89.8494798184388,6.69810503129157,0.532380438266475));
#36639=CARTESIAN_POINT('Ctrl Pts',(89.9487356206599,5.6454060353462,3.67935416839618));
#36640=CARTESIAN_POINT('Ctrl Pts',(90.047991422881,3.1913300203551,5.91299016086127));
#36641=CARTESIAN_POINT('Ctrl Pts',(90.1803324925089,-1.10781160806457,7.03302696040168));
#36642=CARTESIAN_POINT('Ctrl Pts',(90.3457588295443,-6.4299816593523,4.11506845419367));
#36643=CARTESIAN_POINT('Ctrl Pts',(90.544270433986,-6.93962186627816,-3.18075240489431));
#36644=CARTESIAN_POINT('Ctrl Pts',(90.7427820384285,-1.09365453325676,-7.55509478895228));
#36645=CARTESIAN_POINT('Ctrl Pts',(90.9412936428702,5.76199473674139,-5.00778086342357));
#36646=CARTESIAN_POINT('Ctrl Pts',(91.1067199799058,7.05986447627686,0.921427349986869));
#36647=CARTESIAN_POINT('Ctrl Pts',(91.2390610495334,4.77240695698494,4.72992302032322));
#36648=CARTESIAN_POINT('Ctrl Pts',(91.3383168517549,1.93713947686126,6.45412635819934));
#36649=CARTESIAN_POINT('Ctrl Pts',(91.4375726539756,-1.3789902704871,6.57620147008622));
#36650=CARTESIAN_POINT('Ctrl Pts',(91.5699137236039,-5.38561421805492,4.65680945272449));
#36651=CARTESIAN_POINT('Ctrl Pts',(91.7353400606388,-7.56730766762608,-1.00712818736965));
#36652=CARTESIAN_POINT('Ctrl Pts',(91.9338516650811,-3.24748753305086,-6.90864402258845));
#36653=CARTESIAN_POINT('Ctrl Pts',(92.132363269523,4.04109658682085,-6.47650182460808));
#36654=CARTESIAN_POINT('Ctrl Pts',(92.3308748739652,7.63329823526228,-0.105879997395819));
#36655=CARTESIAN_POINT('Ctrl Pts',(92.4963012110003,4.79760967174002,5.26057565503311));
#36656=CARTESIAN_POINT('Ctrl Pts',(92.6286422806284,0.592251030763429,6.69307692005863));
#36657=CARTESIAN_POINT('Ctrl Pts',(92.7278980828495,-2.68622073210826,6.18000603388127));
#36658=CARTESIAN_POINT('Ctrl Pts',(92.8271538850704,-5.29788341543967,4.132852677954));
#36659=CARTESIAN_POINT('Ctrl Pts',(92.9594949546987,-7.1192833602349,0.0807416954368796));
#36660=CARTESIAN_POINT('Ctrl Pts',(93.1249212917336,-5.12988065443664,-5.65356321212946));
#36661=CARTESIAN_POINT('Ctrl Pts',(93.3234328961759,1.97874140565975,-7.37293157147783));
#36662=CARTESIAN_POINT('Ctrl Pts',(93.5219445006178,7.26685670662967,-2.33844630331303));
#36663=CARTESIAN_POINT('Ctrl Pts',(93.7204561050601,5.89867514420218,4.84603797606646));
#36664=CARTESIAN_POINT('Ctrl Pts',(93.8858824420949,0.268991396450776,7.11465799693386));
#36665=CARTESIAN_POINT('Ctrl Pts',(94.0182235117233,-3.86768090757155,5.49445942186024));
#36666=CARTESIAN_POINT('Ctrl Pts',(94.1174793139442,-6.04062557409786,2.98648607463229));
#36667=CARTESIAN_POINT('Ctrl Pts',(94.2167351161653,-6.71408662382135,-0.262832169045199));
#36668=CARTESIAN_POINT('Ctrl Pts',(94.3490761857933,-5.48984361079027,-4.5334679786853));
#36669=CARTESIAN_POINT('Ctrl Pts',(94.5145025228285,-0.26912725164565,-7.62928719112931));
#36670=CARTESIAN_POINT('Ctrl Pts',(94.7130141272706,6.27022417978169,-4.35428825911284));
#36671=CARTESIAN_POINT('Ctrl Pts',(94.9115257317125,7.05979512689293,2.90427792651901));
#36672=CARTESIAN_POINT('Ctrl Pts',(95.110037336155,1.37755152739009,7.50871522377111));
#36673=CARTESIAN_POINT('Ctrl Pts',(95.2754636731897,-4.38669688173065,5.60781644247689));
#36674=CARTESIAN_POINT('Ctrl Pts',(95.4078047428181,-6.50054242434237,1.70029060180525));
#36675=CARTESIAN_POINT('Ctrl Pts',(95.5070605450389,-6.54147331612773,-1.61783288840539));
#36676=CARTESIAN_POINT('Ctrl Pts',(95.6063163472602,-4.95859356993127,-4.53435659708169));
#36677=CARTESIAN_POINT('Ctrl Pts',(95.738657416888,-1.26703302233638,-7.00609321269774));
#36678=CARTESIAN_POINT('Ctrl Pts',(95.9040837539233,4.71876033125727,-6.00097937494037));
#36679=CARTESIAN_POINT('Ctrl Pts',(96.1025953583653,7.5996887809385,0.721296014854075));
#36680=CARTESIAN_POINT('Ctrl Pts',(96.3011069628075,3.5177265579812,6.77503781328492));
#36681=CARTESIAN_POINT('Ctrl Pts',(96.4996185672496,-3.79431958127109,6.62431818661284));
#36682=CARTESIAN_POINT('Ctrl Pts',(96.6650449042846,-6.97013454965913,1.45187435556547));
#36683=CARTESIAN_POINT('Ctrl Pts',(96.7973859739128,-6.06258474183803,-2.89708580979144));
#36684=CARTESIAN_POINT('Ctrl Pts',(96.8966417761337,-3.95216633883919,-5.45789681384359));
#36685=CARTESIAN_POINT('Ctrl Pts',(96.995897578355,-0.860689169115976,-6.66387680674158));
#36686=CARTESIAN_POINT('Ctrl Pts',(97.1282386479826,3.55431674594619,-6.16907993579157));
#36687=CARTESIAN_POINT('Ctrl Pts',(97.2936649850182,7.47753242254522,-1.53784309735809));
#36688=CARTESIAN_POINT('Ctrl Pts',(97.4921765894599,5.33910370722034,5.45614416155886));
#36689=CARTESIAN_POINT('Ctrl Pts',(97.6906881939024,-1.68609599189039,7.44530844319415));
#36690=CARTESIAN_POINT('Ctrl Pts',(97.8891997983443,-7.17377574087814,2.61063098539322));
#36691=CARTESIAN_POINT('Ctrl Pts',(98.0546261353794,-6.26092037418559,-3.38992490371209));
#36692=CARTESIAN_POINT('Ctrl Pts',(98.1869672050076,-2.76069657366338,-6.1258953932813));
#36693=CARTESIAN_POINT('Ctrl Pts',(98.2862230072284,0.50412149632163,-6.7196813851078));
#36694=CARTESIAN_POINT('Ctrl Pts',(98.3854788094498,3.64379989073183,-5.64541958560787));
#36695=CARTESIAN_POINT('Ctrl Pts',(98.5178198790776,6.69662753697565,-2.4178284504321));
#36696=CARTESIAN_POINT('Ctrl Pts',(98.6832462161129,6.70396080658066,3.65176149633809));
#36697=CARTESIAN_POINT('Ctrl Pts',(98.8817578205549,0.556356465979633,7.6135408970419));
#36698=CARTESIAN_POINT('Ctrl Pts',(99.080269424997,-6.09341640305894,4.59845779007474));
#36699=CARTESIAN_POINT('Ctrl Pts',(99.2787810294392,-7.16438111875819,-2.63630341719029));
#36700=CARTESIAN_POINT('Ctrl Pts',(99.4442073664741,-2.59408309049471,-6.63034295525578));
#36701=CARTESIAN_POINT('Ctrl Pts',(99.5765484361025,1.84532892465688,-6.46086690012156));
#36702=CARTESIAN_POINT('Ctrl Pts',(99.6758042383233,4.72226520925161,-4.80712676074899));
#36703=CARTESIAN_POINT('Ctrl Pts',(99.7750600405444,6.42697864563129,-1.96009832147819));
#36704=CARTESIAN_POINT('Ctrl Pts',(99.9074011101725,6.67548963887232,2.47559141742086));
#36705=CARTESIAN_POINT('Ctrl Pts',(100.072827447207,2.7634763067088,7.11629476796499));
#36706=CARTESIAN_POINT('Ctrl Pts',(100.27133905165,-4.48921039950884,6.1743442969362));
#36707=CARTESIAN_POINT('Ctrl Pts',(100.469850656092,-7.62224162748416,-0.420678119724112));
#36708=CARTESIAN_POINT('Ctrl Pts',(100.668362260534,-3.77057368086733,-6.6378631079179));
#36709=CARTESIAN_POINT('Ctrl Pts',(100.833788597569,2.29818426330452,-6.73862477636194));
#36710=CARTESIAN_POINT('Ctrl Pts',(100.966129667197,5.57963155419069,-3.74376169924608));
#36711=CARTESIAN_POINT('Ctrl Pts',(101.065385469418,6.70963774617368,-0.623712847021004));
#36712=CARTESIAN_POINT('Ctrl Pts',(101.164641271639,6.1740893111309,2.65116222050649));
#36713=CARTESIAN_POINT('Ctrl Pts',(101.296982341267,3.50088847425021,6.19955600632511));
#36714=CARTESIAN_POINT('Ctrl Pts',(101.462408678302,-2.48245865335913,7.21913094192572));
#36715=CARTESIAN_POINT('Ctrl Pts',(101.660920282745,-7.41409985309775,1.81842263417024));
#36716=CARTESIAN_POINT('Ctrl Pts',(101.859431887186,-5.55036334083896,-5.24108808291169));
#36717=CARTESIAN_POINT('Ctrl Pts',(102.057943491629,1.40443127803811,-7.50373409094269));
#36718=CARTESIAN_POINT('Ctrl Pts',(102.223369828664,6.10480246684229,-3.66361865176161));
#36719=CARTESIAN_POINT('Ctrl Pts',(102.355710898292,6.67814803189086,0.741875195308663));
#36720=CARTESIAN_POINT('Ctrl Pts',(102.454966700513,5.52741564527365,3.85433946154237));
#36721=CARTESIAN_POINT('Ctrl Pts',(102.554222502734,3.00459536781169,6.01002883661822));
#36722=CARTESIAN_POINT('Ctrl Pts',(102.686563572362,-1.32751245652532,6.99488566471813));
#36723=CARTESIAN_POINT('Ctrl Pts',(102.851989909397,-6.55569429135308,3.91169079563038));
#36724=CARTESIAN_POINT('Ctrl Pts',(103.050501513839,-6.83661078378366,-3.39651151907381));
#36725=CARTESIAN_POINT('Ctrl Pts',(103.249013118281,-0.856525039568993,
-7.58563790098237));
#36726=CARTESIAN_POINT('Ctrl Pts',(103.447524722723,5.91599090405775,-4.82488384786082));
#36727=CARTESIAN_POINT('Ctrl Pts',(103.612951059759,7.02754677198468,1.14206004755057));
#36728=CARTESIAN_POINT('Ctrl Pts',(103.745292129387,4.62194543336102,4.87705447504003));
#36729=CARTESIAN_POINT('Ctrl Pts',(103.844547931608,1.73407389036543,6.51162377157935));
#36730=CARTESIAN_POINT('Ctrl Pts',(103.943803733829,-1.58425230619208,6.52979207728556));
#36731=CARTESIAN_POINT('Ctrl Pts',(104.076144803457,-5.5288040674127,4.48587119382367));
#36732=CARTESIAN_POINT('Ctrl Pts',(104.241571140492,-7.53205730232312,-1.24360979221905));
#36733=CARTESIAN_POINT('Ctrl Pts',(104.440082744934,-3.02954573728368,-7.00695298559832));
#36734=CARTESIAN_POINT('Ctrl Pts',(104.638594349376,4.24193080980006,-6.34677559873763));
#36735=CARTESIAN_POINT('Ctrl Pts',(104.837105953818,7.63287013777217,0.133214029254973));
#36736=CARTESIAN_POINT('Ctrl Pts',(105.002532290853,4.63051802752086,5.40823609188528));
#36737=CARTESIAN_POINT('Ctrl Pts',(105.134873360481,0.382362148644849,6.70834100647539));
#36738=CARTESIAN_POINT('Ctrl Pts',(105.234129162702,-2.87843448765591,6.092854128331));
#36739=CARTESIAN_POINT('Ctrl Pts',(105.333384964924,-5.42470822093489,3.96491872848158));
#36740=CARTESIAN_POINT('Ctrl Pts',(105.465726034552,-7.11832013585827,-0.142243222249852));
#36741=CARTESIAN_POINT('Ctrl Pts',(105.631152371587,-4.95031937521908,-5.81143629238669));
#36742=CARTESIAN_POINT('Ctrl Pts',(105.829663976029,2.20865947171768,-7.30734963681115));
#36743=CARTESIAN_POINT('Ctrl Pts',(106.028175580471,7.33652268058591,-2.10973295029129));
#36744=CARTESIAN_POINT('Ctrl Pts',(106.226687184913,5.74402508331175,5.02838291200097));
#36745=CARTESIAN_POINT('Ctrl Pts',(106.392113521948,0.0460588288224911,
7.11959125045635));
#36746=CARTESIAN_POINT('Ctrl Pts',(106.524454591576,-4.03784666285289,5.37064683348793));
#36747=CARTESIAN_POINT('Ctrl Pts',(106.623710393797,-6.1311871946683,2.7958519411076));
#36748=CARTESIAN_POINT('Ctrl Pts',(106.722966196018,-6.70256218452041,-0.47295414784101));
#36749=CARTESIAN_POINT('Ctrl Pts',(106.855307265646,-5.34518384502274,-4.70317460525356));
#36750=CARTESIAN_POINT('Ctrl Pts',(107.020733602681,-0.0300757036994695,
-7.63394923387465));
#36751=CARTESIAN_POINT('Ctrl Pts',(107.219245207124,6.40350140800699,-4.15583616799732));
#36752=CARTESIAN_POINT('Ctrl Pts',(107.417756811565,6.96539247494741,3.12400954067283));
#36753=CARTESIAN_POINT('Ctrl Pts',(107.616268416008,1.1417167072316,7.54802637153462));
#36754=CARTESIAN_POINT('Ctrl Pts',(107.781694753043,-4.5601256002143,5.46794866870985));
#36755=CARTESIAN_POINT('Ctrl Pts',(107.914035822671,-6.55064542222453,1.49553103310081));
#36756=CARTESIAN_POINT('Ctrl Pts',(108.013291624892,-6.48750220584516,-1.82111132353179));
#36757=CARTESIAN_POINT('Ctrl Pts',(108.112547427113,-4.81434798793785,-4.68885257359087));
#36758=CARTESIAN_POINT('Ctrl Pts',(108.244888496741,-1.04661762809148,-7.03922361376705));
#36759=CARTESIAN_POINT('Ctrl Pts',(108.410314833777,4.90359337122379,-5.85665907486141));
#36760=CARTESIAN_POINT('Ctrl Pts',(108.608826438218,7.57453469313228,0.969844410039962));
#36761=CARTESIAN_POINT('Ctrl Pts',(108.774252775254,4.0147429951218,5.87799298002767));
#36762=CARTESIAN_POINT('Ctrl Pts',(108.906593844881,-0.353800513992823,
6.71099960051513));
#36763=CARTESIAN_POINT('Ctrl Pts',(109.005849647103,-3.5176048912445,5.74308483611783));
#36764=CARTESIAN_POINT('Ctrl Pts',(109.105105449324,-5.8393379223708,3.34881119764833));
#36765=CARTESIAN_POINT('Ctrl Pts',(109.171275984138,-6.43144388944538,1.2184826508284));
#36766=CARTESIAN_POINT('Ctrl Pts',(109.204361251545,-6.45554076211909,0.144895927237655));
#36767=CARTESIAN_POINT('Ctrl Pts',(30.9296387484553,0.703787020950697,-6.6579895365958));
#36768=CARTESIAN_POINT('Ctrl Pts',(30.9627240158623,1.81104192579756,-6.5409464522485));
#36769=CARTESIAN_POINT('Ctrl Pts',(31.0288945506763,3.9614630703719,-5.74628867867225));
#36770=CARTESIAN_POINT('Ctrl Pts',(31.1281503528974,6.23616430535044,-3.14177596404463));
#36771=CARTESIAN_POINT('Ctrl Pts',(31.2274061551185,6.96475406549829,0.21041611353608));
#36772=CARTESIAN_POINT('Ctrl Pts',(31.3597472247465,5.72907466288608,4.65287937038327));
#36773=CARTESIAN_POINT('Ctrl Pts',(31.5251735617817,0.352018242983719,7.90990755251631));
#36774=CARTESIAN_POINT('Ctrl Pts',(31.7236851662237,-6.47247608523396,4.56415182305037));
#36775=CARTESIAN_POINT('Ctrl Pts',(31.8891115032589,-7.18370815896518,-1.68562073726553));
#36776=CARTESIAN_POINT('Ctrl Pts',(32.0214525728869,-4.43172273725023,-5.37703885971554));
#36777=CARTESIAN_POINT('Ctrl Pts',(32.120708375108,-1.32491932170987,-6.85975389770393));
#36778=CARTESIAN_POINT('Ctrl Pts',(32.219964177329,2.10754325246999,-6.64033724856899));
#36779=CARTESIAN_POINT('Ctrl Pts',(32.3523052469572,6.04134746661423,-4.24261341996023));
#36780=CARTESIAN_POINT('Ctrl Pts',(32.5177315839921,7.70128519312101,1.82755503533256));
#36781=CARTESIAN_POINT('Ctrl Pts',(32.7162431884343,2.6301704824596,7.46537716506742));
#36782=CARTESIAN_POINT('Ctrl Pts',(32.9147547928764,-4.84377258193836,6.25996585329837));
#36783=CARTESIAN_POINT('Ctrl Pts',(33.1132663973185,-7.8854783960754,-0.686285559843319));
#36784=CARTESIAN_POINT('Ctrl Pts',(33.2786927343536,-4.40096077659904,-5.92677383246242));
#36785=CARTESIAN_POINT('Ctrl Pts',(33.4110338039817,0.0865720556418617,
-6.96626254547699));
#36786=CARTESIAN_POINT('Ctrl Pts',(33.5102896062028,3.41514643505138,-6.09531225030999));
#36787=CARTESIAN_POINT('Ctrl Pts',(33.6095454084238,5.89598045223297,-3.71130068472704));
#36788=CARTESIAN_POINT('Ctrl Pts',(33.7418864780519,7.35262722554128,0.65865425285292));
#36789=CARTESIAN_POINT('Ctrl Pts',(33.9073128150869,4.70276240256489,6.36680332881671));
#36790=CARTESIAN_POINT('Ctrl Pts',(34.1058244195291,-2.8096405407784,7.39965803111618));
#36791=CARTESIAN_POINT('Ctrl Pts',(34.3043360239712,-7.74015409929537,1.65500165199733));
#36792=CARTESIAN_POINT('Ctrl Pts',(34.5028476284133,-5.58000359828515,-5.61388574230308));
#36793=CARTESIAN_POINT('Ctrl Pts',(34.6682739654484,0.463975112574999,-7.36747544056416));
#36794=CARTESIAN_POINT('Ctrl Pts',(34.8006150350764,4.56249195730454,-5.26497779023408));
#36795=CARTESIAN_POINT('Ctrl Pts',(34.8998708372975,6.542717437068,-2.45130946226545));
#36796=CARTESIAN_POINT('Ctrl Pts',(34.9991266395185,6.89882340027391,0.970855166879508));
#36797=CARTESIAN_POINT('Ctrl Pts',(35.1314677091467,5.19083011233475,5.24883321944595));
#36798=CARTESIAN_POINT('Ctrl Pts',(35.2968940461817,-0.517467800843383,
7.89837825706199));
#36799=CARTESIAN_POINT('Ctrl Pts',(35.4954056506239,-6.92211770973079,3.83839870777912));
#36800=CARTESIAN_POINT('Ctrl Pts',(35.693917255066,-6.98017203345505,-3.73178464450976));
#36801=CARTESIAN_POINT('Ctrl Pts',(35.8924288595081,-0.638542187557634,
-7.88951303279094));
#36802=CARTESIAN_POINT('Ctrl Pts',(36.0578551965432,5.10971968290926,-5.32782621094353));
#36803=CARTESIAN_POINT('Ctrl Pts',(36.1901962661712,6.88312226592188,-1.07654633493236));
#36804=CARTESIAN_POINT('Ctrl Pts',(36.2894520683923,6.57954296507732,2.35067730093337));
#36805=CARTESIAN_POINT('Ctrl Pts',(36.3887078706133,4.64270287690269,5.19438486587639));
#36806=CARTESIAN_POINT('Ctrl Pts',(36.5210489402414,0.576913437500505,7.35949307078124));
#36807=CARTESIAN_POINT('Ctrl Pts',(36.6864752772765,-5.49324859747658,5.69880442441749));
#36808=CARTESIAN_POINT('Ctrl Pts',(36.8849868817186,-7.76462620399256,-1.53609835388737));
#36809=CARTESIAN_POINT('Ctrl Pts',(37.0834984861608,-2.92279631807994,-7.35569710656138));
#36810=CARTESIAN_POINT('Ctrl Pts',(37.2820100906028,4.60456282021147,-6.43817934327911));
#36811=CARTESIAN_POINT('Ctrl Pts',(37.4474364276379,7.34166183769624,-0.771342228995147));
#36812=CARTESIAN_POINT('Ctrl Pts',(37.5797774972661,5.9522048168692,3.62043946998871));
#36813=CARTESIAN_POINT('Ctrl Pts',(37.679033299487,3.50822990006823,6.0422175044686));
#36814=CARTESIAN_POINT('Ctrl Pts',(37.7782891017082,0.19339596467639,6.96411675222807));
#36815=CARTESIAN_POINT('Ctrl Pts',(37.9106301713363,-4.30953385401096,5.99357033281832));
#36816=CARTESIAN_POINT('Ctrl Pts',(38.0760565083712,-7.8740500609415,0.807147854668614));
#36817=CARTESIAN_POINT('Ctrl Pts',(38.2745681128135,-4.93916952350055,-6.18495130608158));
#36818=CARTESIAN_POINT('Ctrl Pts',(38.4730797172554,2.51529172241946,-7.50482017050409));
#36819=CARTESIAN_POINT('Ctrl Pts',(38.6715913216977,7.67249859020869,-1.94548641854781));
#36820=CARTESIAN_POINT('Ctrl Pts',(38.8370176587327,6.10544477510872,4.1495194265607));
#36821=CARTESIAN_POINT('Ctrl Pts',(38.9693587283608,2.20949972980517,6.60715029962298));
#36822=CARTESIAN_POINT('Ctrl Pts',(39.0686145305819,-1.22035097886095,6.87944858919891));
#36823=CARTESIAN_POINT('Ctrl Pts',(39.1678703328029,-4.34727009921643,5.44403956839734));
#36824=CARTESIAN_POINT('Ctrl Pts',(39.300211402431,-7.16018190988124,1.79631912273862));
#36825=CARTESIAN_POINT('Ctrl Pts',(39.465637739466,-6.53519514424037,-4.46580076226038));
#36826=CARTESIAN_POINT('Ctrl Pts',(39.6641493439083,0.219522695062288,-7.91206850493787));
#36827=CARTESIAN_POINT('Ctrl Pts',(39.8626609483503,6.76517028611504,-4.10870895055163));
#36828=CARTESIAN_POINT('Ctrl Pts',(40.0611725527925,7.11598974632188,3.46624320435687));
#36829=CARTESIAN_POINT('Ctrl Pts',(40.2265988898275,1.98505039136329,7.11017175017984));
#36830=CARTESIAN_POINT('Ctrl Pts',(40.3589399594556,-2.57696043924608,6.47268097718231));
#36831=CARTESIAN_POINT('Ctrl Pts',(40.4581957616766,-5.37244500929141,4.46686736149371));
#36832=CARTESIAN_POINT('Ctrl Pts',(40.5574515638977,-6.83431054025086,1.35222911417895));
#36833=CARTESIAN_POINT('Ctrl Pts',(40.6897926335258,-6.62840083232579,-3.24950300497319));
#36834=CARTESIAN_POINT('Ctrl Pts',(40.8552189705609,-2.10915128084571,-7.62913054653119));
#36835=CARTESIAN_POINT('Ctrl Pts',(41.053730575003,5.27451364338199,-5.90156962733256));
#36836=CARTESIAN_POINT('Ctrl Pts',(41.2522421794451,7.81922095656082,1.22833296502099));
#36837=CARTESIAN_POINT('Ctrl Pts',(41.4507537838873,3.197927895255,7.24053928918684));
#36838=CARTESIAN_POINT('Ctrl Pts',(41.6161801209223,-3.07307048586679,6.71201945484378));
#36839=CARTESIAN_POINT('Ctrl Pts',(41.7485211905504,-6.14607918106869,3.28055404434237));
#36840=CARTESIAN_POINT('Ctrl Pts',(41.8477769927714,-6.98662663108923,-0.0558365542697342));
#36841=CARTESIAN_POINT('Ctrl Pts',(41.9470327949925,-6.09286162596302,-3.37836666818218));
#36842=CARTESIAN_POINT('Ctrl Pts',(42.0793738646206,-2.9654009721384,-6.76027842975032));
#36843=CARTESIAN_POINT('Ctrl Pts',(42.2448002016556,3.31324362906204,-7.18850253362882));
#36844=CARTESIAN_POINT('Ctrl Pts',(42.4433118060978,7.83785440228319,-1.10320288663825));
#36845=CARTESIAN_POINT('Ctrl Pts',(42.6418234105398,5.17951620332599,5.98511738731672));
#36846=CARTESIAN_POINT('Ctrl Pts',(42.840335014982,-2.23081687080563,7.59444587250693));
#36847=CARTESIAN_POINT('Ctrl Pts',(43.005761352017,-6.67949037682418,3.14314741608154));
#36848=CARTESIAN_POINT('Ctrl Pts',(43.1381024216452,-6.81182513990394,-1.46128792549235));
#36849=CARTESIAN_POINT('Ctrl Pts',(43.2373582238662,-5.3003656441942,-4.5521635999691));
#36850=CARTESIAN_POINT('Ctrl Pts',(43.3366140260873,-2.47317959847062,-6.51304128741142));
#36851=CARTESIAN_POINT('Ctrl Pts',(43.4689550957153,2.09843740956863,-7.07753684634914));
#36852=CARTESIAN_POINT('Ctrl Pts',(43.6343814327504,7.17048112842823,-3.35206688602163));
#36853=CARTESIAN_POINT('Ctrl Pts',(43.8328930371925,6.69863740392336,4.2163106113326));
#36854=CARTESIAN_POINT('Ctrl Pts',(44.0314046416347,0.0930375100320632,
7.91456646078634));
#36855=CARTESIAN_POINT('Ctrl Pts',(44.2299162460768,-6.60573645894203,4.36077950101958));
#36856=CARTESIAN_POINT('Ctrl Pts',(44.3953425831118,-7.13055707545171,-1.91052955146803));
#36857=CARTESIAN_POINT('Ctrl Pts',(44.52768365274,-4.25970371841246,-5.51282580616876));
#36858=CARTESIAN_POINT('Ctrl Pts',(44.626939454961,-1.11024213000924,-6.89807450059728));
#36859=CARTESIAN_POINT('Ctrl Pts',(44.726195257182,2.31481837844153,-6.57099231567397));
#36860=CARTESIAN_POINT('Ctrl Pts',(44.8585363268101,6.17098591650305,-4.05140718659923));
#36861=CARTESIAN_POINT('Ctrl Pts',(45.0239626638452,7.64042420221512,2.06786605748864));
#36862=CARTESIAN_POINT('Ctrl Pts',(45.2224742682873,2.39502226673733,7.54406300227598));
#36863=CARTESIAN_POINT('Ctrl Pts',(45.4209858727294,-5.03739157284622,6.10521943768569));
#36864=CARTESIAN_POINT('Ctrl Pts',(45.6194974771716,-7.86014378528482,-0.932894257757612));
#36865=CARTESIAN_POINT('Ctrl Pts',(45.7849238142066,-4.21318924362712,-6.06168324565806));
#36866=CARTESIAN_POINT('Ctrl Pts',(45.9172648838348,0.304677466624451,-6.96013618969833));
#36867=CARTESIAN_POINT('Ctrl Pts',(46.0165206860557,3.60435343990901,-5.98537431438118));
#36868=CARTESIAN_POINT('Ctrl Pts',(46.1157764882769,6.00930934388733,-3.52484401744044));
#36869=CARTESIAN_POINT('Ctrl Pts',(46.2481175579048,7.32839584055675,0.888584142001863));
#36870=CARTESIAN_POINT('Ctrl Pts',(46.4135438949401,4.50107442023831,6.51095085874442));
#36871=CARTESIAN_POINT('Ctrl Pts',(46.6120554993821,-3.03998774172088,7.30804301921271));
#36872=CARTESIAN_POINT('Ctrl Pts',(46.8105671038243,-7.78818558123646,1.41180154154107));
#36873=CARTESIAN_POINT('Ctrl Pts',(47.0090787082663,-5.40146397684792,-5.7858740850733));
#36874=CARTESIAN_POINT('Ctrl Pts',(47.1745050453014,0.694465178907303,-7.34933231583605));
#36875=CARTESIAN_POINT('Ctrl Pts',(47.3068461149295,4.72513075256893,-5.11951789809788));
#36876=CARTESIAN_POINT('Ctrl Pts',(47.4061019171506,6.61627298347009,-2.24521740845774));
#36877=CARTESIAN_POINT('Ctrl Pts',(47.5053577193716,6.86503681807585,1.18642050904397));
#36878=CARTESIAN_POINT('Ctrl Pts',(47.6376987889997,5.02391332886568,5.40881338533256));
#36879=CARTESIAN_POINT('Ctrl Pts',(47.8031251260348,-0.764557269425916,
7.87829957562393));
#36880=CARTESIAN_POINT('Ctrl Pts',(48.0016367304769,-7.03892486372586,3.61974515723125));
#36881=CARTESIAN_POINT('Ctrl Pts',(48.200148334919,-6.85988510040067,-3.94854335797116));
#36882=CARTESIAN_POINT('Ctrl Pts',(48.3986599393611,-0.391163364863194,
-7.90563996419626));
#36883=CARTESIAN_POINT('Ctrl Pts',(48.5640862763962,5.27405820819081,-5.16519867864946));
#36884=CARTESIAN_POINT('Ctrl Pts',(48.6964273460243,6.91345919617128,-0.860468523940247));
#36885=CARTESIAN_POINT('Ctrl Pts',(48.7956831482453,6.50270287109063,2.55556740731831));
#36886=CARTESIAN_POINT('Ctrl Pts',(48.8949389504664,4.47776001838488,5.33722674762568));
#36887=CARTESIAN_POINT('Ctrl Pts',(49.0272800200945,0.346162788340026,7.37395000642637));
#36888=CARTESIAN_POINT('Ctrl Pts',(49.1927063571296,-5.66901646168339,5.52398446582457));
#36889=CARTESIAN_POINT('Ctrl Pts',(49.3912179615717,-7.71271398995097,-1.77849969066399));
#36890=CARTESIAN_POINT('Ctrl Pts',(49.5897295660138,-2.69101398775909,-7.44361887512801));
#36891=CARTESIAN_POINT('Ctrl Pts',(49.7882411704559,4.80392059172006,-6.29082657287229));
#36892=CARTESIAN_POINT('Ctrl Pts',(49.9536675074909,7.36221619304494,-0.541054618475516));
#36893=CARTESIAN_POINT('Ctrl Pts',(50.0860085771191,5.83590891040666,3.80506127772645));
#36894=CARTESIAN_POINT('Ctrl Pts',(50.1852643793401,3.31729297670311,6.1491167422447));
#36895=CARTESIAN_POINT('Ctrl Pts',(50.2845201815612,-0.0247850984101731,
6.96675748370172));
#36896=CARTESIAN_POINT('Ctrl Pts',(50.4168612511893,-4.49511308086105,5.85567466339949));
#36897=CARTESIAN_POINT('Ctrl Pts',(50.5822875882243,-7.89546458114876,0.560170571642261));
#36898=CARTESIAN_POINT('Ctrl Pts',(50.7807991926664,-4.74306097661419,-6.33659141909883));
#36899=CARTESIAN_POINT('Ctrl Pts',(50.9793107971086,2.74907679851826,-7.42237125158298));
#36900=CARTESIAN_POINT('Ctrl Pts',(51.1778224015507,7.72965983491366,-1.70426255548574));
#36901=CARTESIAN_POINT('Ctrl Pts',(51.3432487385858,5.97250520035709,4.33868056037944));
#36902=CARTESIAN_POINT('Ctrl Pts',(51.4755898082138,2.00150851007487,6.67310181414272));
#36903=CARTESIAN_POINT('Ctrl Pts',(51.5748456104349,-1.43518721697726,6.8378583675931));
#36904=CARTESIAN_POINT('Ctrl Pts',(51.6741014126559,-4.51562187594898,5.30523168309059));
#36905=CARTESIAN_POINT('Ctrl Pts',(51.806442482284,-7.21292314512711,1.57121197672262));
#36906=CARTESIAN_POINT('Ctrl Pts',(51.9718688193191,-6.39214022313651,-4.66826470856881));
#36907=CARTESIAN_POINT('Ctrl Pts',(52.1703804237613,0.467187014732091,-7.90131346889507));
#36908=CARTESIAN_POINT('Ctrl Pts',(52.3688920282033,6.89051937021597,-3.89483774362364));
#36909=CARTESIAN_POINT('Ctrl Pts',(52.5674036326456,7.00395181794738,3.68738538172778));
#36910=CARTESIAN_POINT('Ctrl Pts',(52.7328299696805,1.76141678409493,7.16884776557682));
#36911=CARTESIAN_POINT('Ctrl Pts',(52.8651710393087,-2.77839310523777,6.38880707883594));
#36912=CARTESIAN_POINT('Ctrl Pts',(52.9644268415297,-5.5096931474724,4.29643466419932));
#36913=CARTESIAN_POINT('Ctrl Pts',(53.0636826437507,-6.87330461061831,1.13754466614294));
#36914=CARTESIAN_POINT('Ctrl Pts',(53.1960237133789,-6.52338941697225,-3.45548229453452));
#36915=CARTESIAN_POINT('Ctrl Pts',(53.3614500504139,-1.86920524799151,-7.69143834158405));
#36916=CARTESIAN_POINT('Ctrl Pts',(53.5599616548561,5.45673852248659,-5.73350005997104));
#36917=CARTESIAN_POINT('Ctrl Pts',(53.7584732592981,7.7769198556102,1.47259492050349));
#36918=CARTESIAN_POINT('Ctrl Pts',(53.9569848637403,2.96961687274043,7.33713347640913));
#36919=CARTESIAN_POINT('Ctrl Pts',(54.1224112007753,-3.28175488390779,6.6124921364985));
#36920=CARTESIAN_POINT('Ctrl Pts',(54.2547522704034,-6.24579764972934,3.08647628477079));
#36921=CARTESIAN_POINT('Ctrl Pts',(54.3540080726245,-6.98145143093807,-0.274600292226041));
#36922=CARTESIAN_POINT('Ctrl Pts',(54.4532638748455,-5.98407741332333,-3.5675119690298));
#36923=CARTESIAN_POINT('Ctrl Pts',(54.5856049444736,-2.7522437004127,-6.84982642019823));
#36924=CARTESIAN_POINT('Ctrl Pts',(54.7510312815086,3.53673163502875,-7.08122033009106));
#36925=CARTESIAN_POINT('Ctrl Pts',(54.9495428859509,7.86855784630405,-0.857213893870046));
#36926=CARTESIAN_POINT('Ctrl Pts',(55.1480544903928,4.98954771636879,6.14438213545968));
#36927=CARTESIAN_POINT('Ctrl Pts',(55.3465660948351,-2.46754816140723,7.52086152595857));
#36928=CARTESIAN_POINT('Ctrl Pts',(55.5119924318701,-6.77464424514777,2.93243290204456));
#36929=CARTESIAN_POINT('Ctrl Pts',(55.6443335014982,-6.76272297486308,-1.67388831857923));
#36930=CARTESIAN_POINT('Ctrl Pts',(55.7435893037193,-5.15521184077243,-4.71591563535623));
#36931=CARTESIAN_POINT('Ctrl Pts',(55.8428451059403,-2.26800614499064,-6.58729627875518));
#36932=CARTESIAN_POINT('Ctrl Pts',(55.9751861755684,2.31904625713534,-7.00835157726648));
#36933=CARTESIAN_POINT('Ctrl Pts',(56.1406125126034,7.27193664698836,-3.12587418551931));
#36934=CARTESIAN_POINT('Ctrl Pts',(56.3391241170457,6.56331528086214,4.42401523104052));
#36935=CARTESIAN_POINT('Ctrl Pts',(56.5376357214876,-0.154858332188795,
7.91359824210381));
#36936=CARTESIAN_POINT('Ctrl Pts',(56.7361473259299,-6.73905750491416,4.151777446705));
#36937=CARTESIAN_POINT('Ctrl Pts',(56.9015736629648,-7.06723026887618,-2.13289092547814));
#36938=CARTESIAN_POINT('Ctrl Pts',(57.033914732593,-4.08497650263706,-5.64351761853546));
#36939=CARTESIAN_POINT('Ctrl Pts',(57.133170534814,-0.893679552924759,-6.92945930500514));
#36940=CARTESIAN_POINT('Ctrl Pts',(57.2324263370351,2.51945830247594,-6.49527936272969));
#36941=CARTESIAN_POINT('Ctrl Pts',(57.3647674066631,6.2948319774138,-3.8561713848629));
#36942=CARTESIAN_POINT('Ctrl Pts',(57.5301937436983,7.5719202245241,2.30611711215016));
#36943=CARTESIAN_POINT('Ctrl Pts',(57.7287053481404,2.15759997642325,7.61536477013516));
#36944=CARTESIAN_POINT('Ctrl Pts',(57.9272169525825,-5.22611018704844,5.94447563316609));
#36945=CARTESIAN_POINT('Ctrl Pts',(58.1257285570246,-7.82707448421245,-1.17858264033489));
#36946=CARTESIAN_POINT('Ctrl Pts',(58.2911548940597,-4.02129698472421,-6.19064923363895));
#36947=CARTESIAN_POINT('Ctrl Pts',(58.4234959636878,0.522489592048809,-6.94718135390302));
#36948=CARTESIAN_POINT('Ctrl Pts',(58.5227517659088,3.79002186327833,-5.86956588504724));
#36949=CARTESIAN_POINT('Ctrl Pts',(58.6220075681298,6.11674500446027,-3.33492948774446));
#36950=CARTESIAN_POINT('Ctrl Pts',(58.754348637758,7.29697494134825,1.11764219616219));
#36951=CARTESIAN_POINT('Ctrl Pts',(58.919774974793,4.29497183500168,6.64871182696699));
#36952=CARTESIAN_POINT('Ctrl Pts',(59.1182865792352,-3.26735326224477,7.20925938638466));
#36953=CARTESIAN_POINT('Ctrl Pts',(59.3167981836772,-7.82857736944446,1.16721660847457));
#36954=CARTESIAN_POINT('Ctrl Pts',(59.5153097881194,-5.21762607811918,-5.95218700398761));
#36955=CARTESIAN_POINT('Ctrl Pts',(59.6807361251544,0.924274080489811,-7.32398011995129));
#36956=CARTESIAN_POINT('Ctrl Pts',(59.8130771947825,4.88313458074863,-4.96903620474978));
#36957=CARTESIAN_POINT('Ctrl Pts',(59.9123329970036,6.68333854791715,-2.03692298748928));
#36958=CARTESIAN_POINT('Ctrl Pts',(60.0115887992246,6.82451622133231,1.40082207385138));
#36959=CARTESIAN_POINT('Ctrl Pts',(60.1439298688527,4.85206852327865,5.56348797237094));
#36960=CARTESIAN_POINT('Ctrl Pts',(60.3093562058879,-1.01089677537493,7.85049296102132));
#36961=CARTESIAN_POINT('Ctrl Pts',(60.5078678103299,-7.14882743815909,3.39754094896599));
#36962=CARTESIAN_POINT('Ctrl Pts',(60.7063794147721,-6.73286921202922,-4.16142889092029));
#36963=CARTESIAN_POINT('Ctrl Pts',(60.9048910192141,-0.143400844275535,
-7.91401214425207));
#36964=CARTESIAN_POINT('Ctrl Pts',(61.0703173562493,5.4332233368635,-4.99750453177072));
#36965=CARTESIAN_POINT('Ctrl Pts',(61.2026584258773,6.9370146190261,-0.643546667488384));
#36966=CARTESIAN_POINT('Ctrl Pts',(61.3019142280984,6.41948418612984,2.75795072237821));
#36967=CARTESIAN_POINT('Ctrl Pts',(61.4011700303195,4.30842486332835,5.47483327005227));
#36968=CARTESIAN_POINT('Ctrl Pts',(61.5335110999474,0.11507258331191,7.3811737328068));
#36969=CARTESIAN_POINT('Ctrl Pts',(61.6989374369827,-5.83922350944862,5.34374595468485));
#36970=CARTESIAN_POINT('Ctrl Pts',(61.8974490414247,-7.65323626838815,-2.01915647256606));
#36971=CARTESIAN_POINT('Ctrl Pts',(62.0959606458669,-2.45659200470146,-7.52423909527826));
#36972=CARTESIAN_POINT('Ctrl Pts',(62.2944722503089,4.9985661312639,-6.13730304391836));
#36973=CARTESIAN_POINT('Ctrl Pts',(62.4598985873441,7.37554884899199,-0.310236280018402));
#36974=CARTESIAN_POINT('Ctrl Pts',(62.592239656972,5.71388848040567,3.98595064837794));
#36975=CARTESIAN_POINT('Ctrl Pts',(62.6914954591932,3.12310207490572,6.24998422660072));
#36976=CARTESIAN_POINT('Ctrl Pts',(62.7907512614142,-0.242941849452053,
6.96256442667514));
#36977=CARTESIAN_POINT('Ctrl Pts',(62.9230923310423,-4.6762829892943,5.71203508194268));
#36978=CARTESIAN_POINT('Ctrl Pts',(63.0885186680774,-7.90913433125535,0.31264380957621));
#36979=CARTESIAN_POINT('Ctrl Pts',(63.2870302725194,-4.54229989580018,-6.48201588219981));
#36980=CARTESIAN_POINT('Ctrl Pts',(63.4855418769616,2.98016526727059,-7.33264162633296));
#36981=CARTESIAN_POINT('Ctrl Pts',(63.6840534814037,7.77923894968028,-1.46136695777802));
#36982=CARTESIAN_POINT('Ctrl Pts',(63.8494798184388,5.83370711288252,4.52358582259813));
#36983=CARTESIAN_POINT('Ctrl Pts',(63.9818208880669,1.79155398304252,6.73250759105857));
#36984=CARTESIAN_POINT('Ctrl Pts',(64.0810766902879,-1.64861566015868,6.78956079640785));
#36985=CARTESIAN_POINT('Ctrl Pts',(64.180332492509,-4.6795442169047,5.16121982285677));
#36986=CARTESIAN_POINT('Ctrl Pts',(64.3126735621371,-7.25858912458045,1.34456360720884));
#36987=CARTESIAN_POINT('Ctrl Pts',(64.4780998991721,-6.24281516352822,-4.86614948964095));
#36988=CARTESIAN_POINT('Ctrl Pts',(64.6766115036143,0.714393064215512,-7.88280792549629));
#36989=CARTESIAN_POINT('Ctrl Pts',(64.8751231080564,7.00910944883397,-3.67714603663721));
#36990=CARTESIAN_POINT('Ctrl Pts',(65.0736347124984,6.88504361663661,3.90491055192439));
#36991=CARTESIAN_POINT('Ctrl Pts',(65.2390610495337,1.53605537881087,7.22049175932465));
#36992=CARTESIAN_POINT('Ctrl Pts',(65.3714021191617,-2.97710040711504,6.2986663115184));
#36993=CARTESIAN_POINT('Ctrl Pts',(65.4706579213827,-5.64153675165296,4.12178753487387));
#36994=CARTESIAN_POINT('Ctrl Pts',(65.5699137236038,-6.90555656170388,0.921744384878935));
#36995=CARTESIAN_POINT('Ctrl Pts',(65.7022547932318,-6.41197911895647,-3.65807205390767));
#36996=CARTESIAN_POINT('Ctrl Pts',(65.8676811302669,-1.62742568595715,-7.74620149858267));
#36997=CARTESIAN_POINT('Ctrl Pts',(66.0661927347091,5.63361081156164,-5.55980642350118));
#36998=CARTESIAN_POINT('Ctrl Pts',(66.2647043391511,7.72699026663113,1.71541238764292));
#36999=CARTESIAN_POINT('Ctrl Pts',(66.4632159435934,2.73839291224447,7.42653056757245));
#37000=CARTESIAN_POINT('Ctrl Pts',(66.6286422806283,-3.48722016361297,6.50647853454183));
#37001=CARTESIAN_POINT('Ctrl Pts',(66.7609833502565,-6.33938952892727,2.88937095647236));
#37002=CARTESIAN_POINT('Ctrl Pts',(66.8602391524775,-6.96942802968025,-0.493094667537342));
#37003=CARTESIAN_POINT('Ctrl Pts',(66.9594949546985,-5.86942333497652,-3.75315785451707));
#37004=CARTESIAN_POINT('Ctrl Pts',(67.0918360243268,-2.53638671842853,-6.93265530775572));
#37005=CARTESIAN_POINT('Ctrl Pts',(67.2572623613616,3.75675041938502,-6.96699208776573));
#37006=CARTESIAN_POINT('Ctrl Pts',(67.4557739658039,7.89154290138557,-0.610384001760516));
#37007=CARTESIAN_POINT('Ctrl Pts',(67.6542855702459,4.79468493537967,6.2976196889886));
#37008=CARTESIAN_POINT('Ctrl Pts',(67.8527971746882,-2.70185904364832,7.43990003111806));
#37009=CARTESIAN_POINT('Ctrl Pts',(68.0182235117231,-6.86315269475213,2.7188416279581));
#37010=CARTESIAN_POINT('Ctrl Pts',(68.1505645813512,-6.70698726885656,-1.88484635754777));
#37011=CARTESIAN_POINT('Ctrl Pts',(68.2498203835723,-5.00500098465436,-4.87504266827532));
#37012=CARTESIAN_POINT('Ctrl Pts',(68.3490761857934,-2.06060840545458,-6.6550880314067));
#37013=CARTESIAN_POINT('Ctrl Pts',(68.4814172554214,2.53738125462533,-6.93229532543533));
#37014=CARTESIAN_POINT('Ctrl Pts',(68.6468435924565,7.36625711755882,-2.89660791997047));
#37015=CARTESIAN_POINT('Ctrl Pts',(68.8453551968987,6.42155828060474,4.62736804226398));
#37016=CARTESIAN_POINT('Ctrl Pts',(69.0438668013406,-0.402608105905313,
7.90488998104792));
#37017=CARTESIAN_POINT('Ctrl Pts',(69.242378405783,-6.86575660957116,3.9386584492253));
#37018=CARTESIAN_POINT('Ctrl Pts',(69.4078047428178,-6.99699134364105,-2.35308206491398));
#37019=CARTESIAN_POINT('Ctrl Pts',(69.5401458124461,-3.9062140072152,-5.76878272593319));
#37020=CARTESIAN_POINT('Ctrl Pts',(69.6394016146671,-0.67630210031753,-6.95380861243962));
#37021=CARTESIAN_POINT('Ctrl Pts',(69.7386574168881,2.72174082037459,-6.41363491508409));
#37022=CARTESIAN_POINT('Ctrl Pts',(69.8709984865163,6.41225712779278,-3.65620280145809));
#37023=CARTESIAN_POINT('Ctrl Pts',(70.0364248235513,7.4964906511866,2.54016968052848));
#37024=CARTESIAN_POINT('Ctrl Pts',(70.2349364279935,1.91722753812611,7.68241290066031));
#37025=CARTESIAN_POINT('Ctrl Pts',(70.4334480324354,-5.40817629061345,5.77201989048123));
#37026=CARTESIAN_POINT('Ctrl Pts',(70.6319596368777,-7.78926927884629,-1.41183502746632));
#37027=CARTESIAN_POINT('Ctrl Pts',(70.8304712413197,-3.02695043533247,-7.31525976480649));
#37028=CARTESIAN_POINT('Ctrl Pts',(70.9958975783549,3.23651895324008,-6.63681545056612));
#37029=CARTESIAN_POINT('Ctrl Pts',(71.1282386479829,6.21430277804793,-3.13408715922093));
#37030=CARTESIAN_POINT('Ctrl Pts',(71.260579717611,7.25906612343537,1.33970346626809));
#37031=CARTESIAN_POINT('Ctrl Pts',(71.4260060546461,4.08917549587174,6.78386515788701));
#37032=CARTESIAN_POINT('Ctrl Pts',(71.6245176590882,-3.50191772613163,7.10041261509974));
#37033=CARTESIAN_POINT('Ctrl Pts',(71.7899439961233,-7.11586513205948,1.95521631953288));
#37034=CARTESIAN_POINT('Ctrl Pts',(71.9222850657513,-6.4629128098114,-2.60461226368976));
#37035=CARTESIAN_POINT('Ctrl Pts',(72.0215408679724,-4.44333502316774,-5.39127437082873));
#37036=CARTESIAN_POINT('Ctrl Pts',(72.1207966701935,-1.3234918693767,-6.84003759421039));
#37037=CARTESIAN_POINT('Ctrl Pts',(72.2531377398215,3.27785032304679,-6.61450544205606));
#37038=CARTESIAN_POINT('Ctrl Pts',(72.4185640768567,7.63789641404816,-2.07674216600752));
#37039=CARTESIAN_POINT('Ctrl Pts',(72.6170756812987,5.87917379908106,5.29954484007954));
#37040=CARTESIAN_POINT('Ctrl Pts',(72.815587285741,-1.26157197373669,7.81392751410292));
#37041=CARTESIAN_POINT('Ctrl Pts',(73.0140988901829,-7.25403793956794,3.16714455742375));
#37042=CARTESIAN_POINT('Ctrl Pts',(73.1795252272182,-6.6989147707515,-3.10155658511558));
#37043=CARTESIAN_POINT('Ctrl Pts',(73.3118662968461,-3.25441148556226,-6.15995869185653));
#37044=CARTESIAN_POINT('Ctrl Pts',(73.4111220990672,0.0855123818222237,
-6.98632677128281));
#37045=CARTESIAN_POINT('Ctrl Pts',(73.5103779012882,3.40421955141891,-6.07845533473538));
#37046=CARTESIAN_POINT('Ctrl Pts',(73.6427189709164,6.77281349086935,-2.93665698018454));
#37047=CARTESIAN_POINT('Ctrl Pts',(73.8081453079514,7.17436363933803,3.34375023752143));
#37048=CARTESIAN_POINT('Ctrl Pts',(74.0066569123935,1.06989784145846,7.84247000558746));
#37049=CARTESIAN_POINT('Ctrl Pts',(74.2051685168357,-6.00706560616107,5.15404498146463));
#37050=CARTESIAN_POINT('Ctrl Pts',(74.4036801212777,-7.58490102008606,-2.26305761715745));
#37051=CARTESIAN_POINT('Ctrl Pts',(74.5691064583128,-3.11474484508245,-6.69278205299726));
#37052=CARTESIAN_POINT('Ctrl Pts',(74.7014475279409,1.4902110483153,-6.8055561970632));
#37053=CARTESIAN_POINT('Ctrl Pts',(74.8007033301619,4.57463825090347,-5.28098043453118));
#37054=CARTESIAN_POINT('Ctrl Pts',(74.8999591323831,6.52348847355142,-2.44549017964904));
#37055=CARTESIAN_POINT('Ctrl Pts',(75.0323002020111,7.06855892447008,2.12848353322983));
#37056=CARTESIAN_POINT('Ctrl Pts',(75.1977265390462,3.3215767601887,7.18465586037287));
#37057=CARTESIAN_POINT('Ctrl Pts',(75.3962381434883,-4.24472807719733,6.68066626805726));
#37058=CARTESIAN_POINT('Ctrl Pts',(75.5947497479305,-7.91489027044559,0.0594159499921341));
#37059=CARTESIAN_POINT('Ctrl Pts',(75.7932613523725,-4.33267928530105,-6.6242012521571));
#37060=CARTESIAN_POINT('Ctrl Pts',(75.9586876894076,1.94080259747868,-7.1223768961395));
#37061=CARTESIAN_POINT('Ctrl Pts',(76.0910287590358,5.53087109503579,-4.23624704999356));
#37062=CARTESIAN_POINT('Ctrl Pts',(76.1902845612566,6.90272852036613,-1.08092940410934));
#37063=CARTESIAN_POINT('Ctrl Pts',(76.289540363478,6.56109978442663,2.34271077106102));
#37064=CARTESIAN_POINT('Ctrl Pts',(76.4218814331058,4.02515656315956,6.18814043273438));
#37065=CARTESIAN_POINT('Ctrl Pts',(76.587307770141,-2.10030357655869,7.63157106419049));
#37066=CARTESIAN_POINT('Ctrl Pts',(76.7858193745831,-7.55416888152773,2.36295381882188));
#37067=CARTESIAN_POINT('Ctrl Pts',(76.9843309790252,-6.08376574105329,-5.06328081864295));
#37068=CARTESIAN_POINT('Ctrl Pts',(77.1828425834674,0.966275376086498,-7.8561099737133));
#37069=CARTESIAN_POINT('Ctrl Pts',(77.3482689205024,6.07952599095048,-4.18740147330903));
#37070=CARTESIAN_POINT('Ctrl Pts',(77.4806099901305,6.95877913506417,0.334241061524722));
#37071=CARTESIAN_POINT('Ctrl Pts',(77.5798657923515,5.97000918027016,3.6297465187709));
#37072=CARTESIAN_POINT('Ctrl Pts',(77.6791215945727,3.49928493975354,6.02422850232547));
#37073=CARTESIAN_POINT('Ctrl Pts',(77.8114626642005,-0.919706818894118,
7.32455505410309));
#37074=CARTESIAN_POINT('Ctrl Pts',(77.9768890012359,-6.53001247368982,4.4733755839371));
#37075=CARTESIAN_POINT('Ctrl Pts',(78.1754006056778,-7.29506335116228,-3.07100454949284));
#37076=CARTESIAN_POINT('Ctrl Pts',(78.37391221012,-1.37870494315477,-7.79411258067252));
#37077=CARTESIAN_POINT('Ctrl Pts',(78.5724238145621,5.80876705622893,-5.37683711004694));
#37078=CARTESIAN_POINT('Ctrl Pts',(78.7378501515972,7.34631594906046,0.725678544458096));
#37079=CARTESIAN_POINT('Ctrl Pts',(78.8701912212252,5.09939956490671,4.74683560019161));
#37080=CARTESIAN_POINT('Ctrl Pts',(78.9694470234464,2.21709152222903,6.62575086953153));
#37081=CARTESIAN_POINT('Ctrl Pts',(79.0687028256673,-1.2155721704975,6.85993501690279));
#37082=CARTESIAN_POINT('Ctrl Pts',(79.2010438952956,-5.43010594047177,5.00089160536001));
#37083=CARTESIAN_POINT('Ctrl Pts',(79.3664702323305,-7.87498068815616,-0.798017031570015));
#37084=CARTESIAN_POINT('Ctrl Pts',(79.5649818367727,-3.58981146310726,-7.05423786810604));
#37085=CARTESIAN_POINT('Ctrl Pts',(79.7634934412146,3.9776482136295,-6.8430499727159));
#37086=CARTESIAN_POINT('Ctrl Pts',(79.9620050456571,7.90723027905429,-0.357577034378644));
#37087=CARTESIAN_POINT('Ctrl Pts',(80.1274313826919,5.14274811428306,5.29595215295085));
#37088=CARTESIAN_POINT('Ctrl Pts',(80.2597724523201,0.831092698151305,6.91705205017979));
#37089=CARTESIAN_POINT('Ctrl Pts',(80.3590282545412,-2.5831675372795,6.49178826498396));
#37090=CARTESIAN_POINT('Ctrl Pts',(80.4582840567621,-5.35619991408986,4.45504731940314));
#37091=CARTESIAN_POINT('Ctrl Pts',(80.5906251263903,-7.37535395809592,0.314835458781826));
#37092=CARTESIAN_POINT('Ctrl Pts',(80.7560514634253,-5.49985289947136,-5.69243094869711));
#37093=CARTESIAN_POINT('Ctrl Pts',(80.9545630678674,1.81124690432845,-7.70508941492813));
#37094=CARTESIAN_POINT('Ctrl Pts',(81.1530746723097,7.45498302009343,-2.65936955134027));
#37095=CARTESIAN_POINT('Ctrl Pts',(81.3515862767515,6.27036297575581,4.83060039475208));
#37096=CARTESIAN_POINT('Ctrl Pts',(81.5170126137868,0.509775375194911,7.36444814226785));
#37097=CARTESIAN_POINT('Ctrl Pts',(81.6493536834148,-3.82981762340274,5.81969252704047));
#37098=CARTESIAN_POINT('Ctrl Pts',(81.7486094856359,-6.16315297181846,3.29114187615832));
#37099=CARTESIAN_POINT('Ctrl Pts',(81.8478652878569,-6.96658933945347,-0.0543793456253106));
#37100=CARTESIAN_POINT('Ctrl Pts',(81.980206357485,-5.83652679283063,-4.51994716450058));
#37101=CARTESIAN_POINT('Ctrl Pts',(82.1456326945201,-0.526625940840279,
-7.8977729227892));
#37102=CARTESIAN_POINT('Ctrl Pts',(82.3441442989623,6.35668255517161,-4.71610062798219));
#37103=CARTESIAN_POINT('Ctrl Pts',(82.5426559034043,7.41062632852998,2.78058189222602));
#37104=CARTESIAN_POINT('Ctrl Pts',(82.7411675078465,1.67141193306518,7.73682972356996));
#37105=CARTESIAN_POINT('Ctrl Pts',(82.9065938448815,-4.36401234628641,5.9540207939481));
#37106=CARTESIAN_POINT('Ctrl Pts',(83.0389349145097,-6.68154392307749,1.97314341643064));
#37107=CARTESIAN_POINT('Ctrl Pts',(83.1381907167306,-6.83170006191115,-1.46422118107929));
#37108=CARTESIAN_POINT('Ctrl Pts',(83.2374465189518,-5.28600165851457,-4.5381175176496));
#37109=CARTESIAN_POINT('Ctrl Pts',(83.3697875885797,-1.54055762886207,-7.2195325032485));
#37110=CARTESIAN_POINT('Ctrl Pts',(83.5352139256149,4.69537611137566,-6.37225197196651));
#37111=CARTESIAN_POINT('Ctrl Pts',(83.733725530057,7.89925758918072,0.500747221907372));
#37112=CARTESIAN_POINT('Ctrl Pts',(83.9322371344991,3.86553198727663,6.90700229447031));
#37113=CARTESIAN_POINT('Ctrl Pts',(84.1307487389412,-3.71710458261341,6.98822477768299));
#37114=CARTESIAN_POINT('Ctrl Pts',(84.2961750759764,-7.17626550279582,1.73094795031224));
#37115=CARTESIAN_POINT('Ctrl Pts',(84.4285161456044,-6.3769469468741,-2.8055074005553));
#37116=CARTESIAN_POINT('Ctrl Pts',(84.5277719478254,-4.27299097177398,-5.52789449593384));
#37117=CARTESIAN_POINT('Ctrl Pts',(84.6270277500466,-1.1083369152707,-6.87807483385178));
#37118=CARTESIAN_POINT('Ctrl Pts',(84.7593688196745,3.48316218043484,-6.50865182646114));
#37119=CARTESIAN_POINT('Ctrl Pts',(84.9247951567098,7.69930924419873,-1.83651550053466));
#37120=CARTESIAN_POINT('Ctrl Pts',(85.1233067611518,5.71026835033156,5.48104493757155));
#37121=CARTESIAN_POINT('Ctrl Pts',(85.3218183655939,-1.5056176378391,7.770594170918));
#37122=CARTESIAN_POINT('Ctrl Pts',(85.5203299700361,-7.34968207461022,2.9384222677589));
#37123=CARTESIAN_POINT('Ctrl Pts',(85.685756307071,-6.59849172823567,-3.30981484160565));
#37124=CARTESIAN_POINT('Ctrl Pts',(85.8180973766992,-3.05991657066862,-6.25885250811717));
#37125=CARTESIAN_POINT('Ctrl Pts',(85.9173531789202,0.304254704681881,-6.98022195046236));
#37126=CARTESIAN_POINT('Ctrl Pts',(86.0166089811413,3.5928998711205,-5.9688687918164));
#37127=CARTESIAN_POINT('Ctrl Pts',(86.1489500507693,6.86145602376702,-2.72312111504753));
#37128=CARTESIAN_POINT('Ctrl Pts',(86.3143763878044,7.06613256296911,3.56678042834934));
#37129=CARTESIAN_POINT('Ctrl Pts',(86.5128879922466,0.823780881558363,7.87212825731745));
#37130=CARTESIAN_POINT('Ctrl Pts',(86.7113995966886,-6.16552207028737,4.96340164013314));
#37131=CARTESIAN_POINT('Ctrl Pts',(86.9099112011308,-7.51031163519052,-2.4994741774684));
#37132=CARTESIAN_POINT('Ctrl Pts',(87.0753375381659,-2.90362806138492,-6.78703996263797));
#37133=CARTESIAN_POINT('Ctrl Pts',(87.2076786077939,1.70260095722469,-6.75555135560928));
#37134=CARTESIAN_POINT('Ctrl Pts',(87.3069344100151,4.73777219237801,-5.1351323309305));
#37135=CARTESIAN_POINT('Ctrl Pts',(87.4061902122361,6.59687123178447,-2.2400031448799));
#37136=CARTESIAN_POINT('Ctrl Pts',(87.5385312818641,6.99843714004682,2.34879649397724));
#37137=CARTESIAN_POINT('Ctrl Pts',(87.7039576188994,3.09495512387445,7.28514960743508));
#37138=CARTESIAN_POINT('Ctrl Pts',(87.9024692233413,-4.45185598151977,6.54446304598655));
#37139=CARTESIAN_POINT('Ctrl Pts',(88.1009808277835,-7.91286900967269,-0.188473542542395));
#37140=CARTESIAN_POINT('Ctrl Pts',(88.2994924322255,-4.12311277525013,-6.75663326399157));
#37141=CARTESIAN_POINT('Ctrl Pts',(88.4649187692607,2.16289295594546,-7.05810607985089));
#37142=CARTESIAN_POINT('Ctrl Pts',(88.5972598388886,5.66081949484133,-4.06096623781112));
#37143=CARTESIAN_POINT('Ctrl Pts',(88.6965156411099,6.93319309360078,-0.864235459746917));
#37144=CARTESIAN_POINT('Ctrl Pts',(88.7957714433308,6.48451821344733,2.54702722350721));
#37145=CARTESIAN_POINT('Ctrl Pts',(88.9281125129589,3.82939643050207,6.31115602337365));
#37146=CARTESIAN_POINT('Ctrl Pts',(89.093538849994,-2.33826147978246,7.56205562487302));
#37147=CARTESIAN_POINT('Ctrl Pts',(89.2920504544362,-7.62446144690003,2.12523078398847));
#37148=CARTESIAN_POINT('Ctrl Pts',(89.4905620588781,-5.92222171872122,-5.25131489769799));
#37149=CARTESIAN_POINT('Ctrl Pts',(89.6890736633205,1.21182106502083,-7.82199729786965));
#37150=CARTESIAN_POINT('Ctrl Pts',(89.8545000003553,6.20767566568141,-3.99496310408662));
#37151=CARTESIAN_POINT('Ctrl Pts',(89.9868410699837,6.94489916009337,0.551996190160592));
#37152=CARTESIAN_POINT('Ctrl Pts',(90.0860968722044,5.85341308476034,3.81492131795592));
#37153=CARTESIAN_POINT('Ctrl Pts',(90.1853526744257,3.30891574175122,6.13085644521284));
#37154=CARTESIAN_POINT('Ctrl Pts',(90.3176937440536,-1.14862933179586,7.29216141013383));
#37155=CARTESIAN_POINT('Ctrl Pts',(90.4831200810889,-6.66689668448537,4.26668965591664));
#37156=CARTESIAN_POINT('Ctrl Pts',(90.6816316855308,-7.19531477116699,-3.29794839018185));
#37157=CARTESIAN_POINT('Ctrl Pts',(90.8801432899731,-1.13395063439024,-7.83346501870296));
#37158=CARTESIAN_POINT('Ctrl Pts',(91.0786548944152,5.97429753948523,-5.1922943802532));
#37159=CARTESIAN_POINT('Ctrl Pts',(91.2440812314501,7.31998776409361,0.955377677584506));
#37160=CARTESIAN_POINT('Ctrl Pts',(91.3764223010784,4.94824803617576,4.90419876333531));
#37161=CARTESIAN_POINT('Ctrl Pts',(91.4756781032993,2.00851408913216,6.691931003589));
#37162=CARTESIAN_POINT('Ctrl Pts',(91.5749339055204,-1.42979967118216,6.81850401760568));
#37163=CARTESIAN_POINT('Ctrl Pts',(91.7072749751485,-5.58404914297759,4.82839129960669));
#37164=CARTESIAN_POINT('Ctrl Pts',(91.8727013121836,-7.84612788535665,-1.04423619365413));
#37165=CARTESIAN_POINT('Ctrl Pts',(92.0712129166257,-3.36714239853421,-7.1631955375008));
#37166=CARTESIAN_POINT('Ctrl Pts',(92.2697245210679,4.18999226804572,-6.71513090223818));
#37167=CARTESIAN_POINT('Ctrl Pts',(92.4682361255099,7.91454989958454,-0.109781184610879));
#37168=CARTESIAN_POINT('Ctrl Pts',(92.633662462545,4.97437935417045,5.45440348838535));
#37169=CARTESIAN_POINT('Ctrl Pts',(92.7660035321731,0.614072736527218,6.93968578626373));
#37170=CARTESIAN_POINT('Ctrl Pts',(92.8652593343941,-2.78519551710407,6.40771061569896));
#37171=CARTESIAN_POINT('Ctrl Pts',(92.9645151366152,-5.49308586686432,4.28512914590364));
#37172=CARTESIAN_POINT('Ctrl Pts',(93.0968562062433,-7.38159595855551,0.0837166527253544));
#37173=CARTESIAN_POINT('Ctrl Pts',(93.2622825432784,-5.31889298270758,-5.86187081570485));
#37174=CARTESIAN_POINT('Ctrl Pts',(93.4607941477204,2.05164885620794,-7.64458993087906));
#37175=CARTESIAN_POINT('Ctrl Pts',(93.6593057521627,7.53460669885321,-2.42460721232809));
#37176=CARTESIAN_POINT('Ctrl Pts',(93.8578173566046,6.11601398653092,5.02459201707624));
#37177=CARTESIAN_POINT('Ctrl Pts',(94.0232436936398,0.278902482799911,7.37680017205256));
#37178=CARTESIAN_POINT('Ctrl Pts',(94.1555847632679,-4.01018702469117,5.69690478811222));
#37179=CARTESIAN_POINT('Ctrl Pts',(94.2548405654889,-6.26319463191549,3.09652424595433));
#37180=CARTESIAN_POINT('Ctrl Pts',(94.3540963677101,-6.96146960024302,-0.27251631640912));
#37181=CARTESIAN_POINT('Ctrl Pts',(94.486437437338,-5.69211890579575,-4.70050526386146));
#37182=CARTESIAN_POINT('Ctrl Pts',(94.6518637743733,-0.279043343629097,
-7.91039106706398));
#37183=CARTESIAN_POINT('Ctrl Pts',(94.8503753788152,6.50125288217034,-4.51472360201029));
#37184=CARTESIAN_POINT('Ctrl Pts',(95.0488869832574,7.31991585950621,3.01128710856776));
#37185=CARTESIAN_POINT('Ctrl Pts',(95.2473985876994,1.42830791706925,7.78537658148567));
#37186=CARTESIAN_POINT('Ctrl Pts',(95.4128249247347,-4.5483263321779,5.81443848959844));
#37187=CARTESIAN_POINT('Ctrl Pts',(95.5451659943625,-6.74005728665945,1.76293843067934));
#37188=CARTESIAN_POINT('Ctrl Pts',(95.6444217965838,-6.78249629211747,-1.67744253268196));
#37189=CARTESIAN_POINT('Ctrl Pts',(95.7436775988047,-5.14129476294861,-4.70142662372754));
#37190=CARTESIAN_POINT('Ctrl Pts',(95.8760186684329,-1.3137173172897,-7.26423527864844));
#37191=CARTESIAN_POINT('Ctrl Pts',(96.0414450054678,4.89262478090952,-6.22208765405457));
#37192=CARTESIAN_POINT('Ctrl Pts',(96.2399566099102,7.87970209262807,0.747872430237851));
#37193=CARTESIAN_POINT('Ctrl Pts',(96.4384682143521,3.64733847914141,7.02466655856714));
#37194=CARTESIAN_POINT('Ctrl Pts',(96.6369798187943,-3.93412267350125,6.8683936121448));
#37195=CARTESIAN_POINT('Ctrl Pts',(96.8024061558295,-7.22695170552315,1.50536919702228));
#37196=CARTESIAN_POINT('Ctrl Pts',(96.9347472254574,-6.28596289321945,-3.00382999566979));
#37197=CARTESIAN_POINT('Ctrl Pts',(97.0340030276785,-4.0977853525626,-5.65899501743564));
#37198=CARTESIAN_POINT('Ctrl Pts',(97.1332588298995,-0.89240157623222,-6.90940978409554));
#37199=CARTESIAN_POINT('Ctrl Pts',(97.2655998995276,3.68527684596027,-6.39638194153036));
#37200=CARTESIAN_POINT('Ctrl Pts',(97.4310262365628,7.75304483854773,-1.59450548853764));
#37201=CARTESIAN_POINT('Ctrl Pts',(97.6295378410048,5.53582493536608,5.65717778803673));
#37202=CARTESIAN_POINT('Ctrl Pts',(97.8280494454469,-1.74822081517287,7.71963355489581));
#37203=CARTESIAN_POINT('Ctrl Pts',(98.0265610498892,-7.43809613088684,2.70682063853417));
#37204=CARTESIAN_POINT('Ctrl Pts',(98.191987386924,-6.49160627445521,-3.51482792619504));
#37205=CARTESIAN_POINT('Ctrl Pts',(98.3243284565523,-2.86241544827032,-6.35160624876261));
#37206=CARTESIAN_POINT('Ctrl Pts',(98.4235842587731,0.522696037167918,-6.96727050255458));
#37207=CARTESIAN_POINT('Ctrl Pts',(98.5228400609945,3.77805702993185,-5.85342713428637));
#37208=CARTESIAN_POINT('Ctrl Pts',(98.6551811306222,6.94336722695929,-2.50691422368103));
#37209=CARTESIAN_POINT('Ctrl Pts',(98.8206074676577,6.95097069356383,3.78631198380759));
#37210=CARTESIAN_POINT('Ctrl Pts',(99.0191190720994,0.576855623380361,7.89406459501387));
#37211=CARTESIAN_POINT('Ctrl Pts',(99.2176306765419,-6.31793055827079,4.76788964861238));
#37212=CARTESIAN_POINT('Ctrl Pts',(99.4161422809836,-7.42835536047989,-2.73343898046748));
#37213=CARTESIAN_POINT('Ctrl Pts',(99.581568618019,-2.68966303039799,-6.87464036559134));
#37214=CARTESIAN_POINT('Ctrl Pts',(99.713909687647,1.91332074356496,-6.69891990324268));
#37215=CARTESIAN_POINT('Ctrl Pts',(99.8131654898681,4.89625879741496,-4.98424710380356));
#37216=CARTESIAN_POINT('Ctrl Pts',(99.9124212920891,6.6637830236258,-2.03231886077308));
#37217=CARTESIAN_POINT('Ctrl Pts',(100.044762361717,6.92145049527186,2.5668054883079));
#37218=CARTESIAN_POINT('Ctrl Pts',(100.210188698752,2.86529760159607,7.37849725051084));
#37219=CARTESIAN_POINT('Ctrl Pts',(100.408700303194,-4.65461699799906,6.40184026998606));
#37220=CARTESIAN_POINT('Ctrl Pts',(100.607211907637,-7.90308590705035,-0.436178158851584));
#37221=CARTESIAN_POINT('Ctrl Pts',(100.805723512079,-3.90950184671483,-6.88243760102782));
#37222=CARTESIAN_POINT('Ctrl Pts',(100.971149849114,2.38286170273553,-6.9869118699854));
#37223=CARTESIAN_POINT('Ctrl Pts',(101.103490918742,5.7852151187988,-3.88170196782793));
#37224=CARTESIAN_POINT('Ctrl Pts',(101.202746720963,6.95685680207187,-0.6466937749077));
#37225=CARTESIAN_POINT('Ctrl Pts',(101.302002523184,6.40157588913561,2.74884526182444));
#37226=CARTESIAN_POINT('Ctrl Pts',(101.434343592812,3.6298799900591,6.42798091402542));
#37227=CARTESIAN_POINT('Ctrl Pts',(101.599769929847,-2.57392575006508,7.48512246089938));
#37228=CARTESIAN_POINT('Ctrl Pts',(101.798281534289,-7.68727507288713,1.88542308096755));
#37229=CARTESIAN_POINT('Ctrl Pts',(101.996793138731,-5.75486850742494,-5.43419788954419));
#37230=CARTESIAN_POINT('Ctrl Pts',(102.195304743174,1.45617806195801,-7.78021191699693));
#37231=CARTESIAN_POINT('Ctrl Pts',(102.360731080208,6.3297361457371,-3.79860602045742));
#37232=CARTESIAN_POINT('Ctrl Pts',(102.493072149837,6.92420683775317,0.769209858120306));
#37233=CARTESIAN_POINT('Ctrl Pts',(102.592327952058,5.73107529562657,3.99635400820522));
#37234=CARTESIAN_POINT('Ctrl Pts',(102.691583754279,3.11530078266195,6.2314705464568));
#37235=CARTESIAN_POINT('Ctrl Pts',(102.823924823907,-1.37642513834393,7.25261478446579));
#37236=CARTESIAN_POINT('Ctrl Pts',(102.989351160942,-6.79724124437457,4.05581847316578));
#37237=CARTESIAN_POINT('Ctrl Pts',(103.187862765384,-7.08850820767564,-3.52165722780795));
#37238=CARTESIAN_POINT('Ctrl Pts',(103.386374369826,-0.888084017809581,
-7.86513350286279));
#37239=CARTESIAN_POINT('Ctrl Pts',(103.584885974268,6.13396775188958,-5.00265845728224));
#37240=CARTESIAN_POINT('Ctrl Pts',(103.750312311303,7.28647930217096,1.18413966755644));
#37241=CARTESIAN_POINT('Ctrl Pts',(103.882653380931,4.792242702703,5.05675133029455));
#37242=CARTESIAN_POINT('Ctrl Pts',(103.981909183152,1.79796647685818,6.75154693018687));
#37243=CARTESIAN_POINT('Ctrl Pts',(104.081164985374,-1.64262466163945,6.77038465375933));
#37244=CARTESIAN_POINT('Ctrl Pts',(104.213506055001,-5.73251487468722,4.65115475805918));
#37245=CARTESIAN_POINT('Ctrl Pts',(104.378932392037,-7.80957870745604,-1.28943104969529));
#37246=CARTESIAN_POINT('Ctrl Pts',(104.577443996479,-3.14117045761931,-7.26512673019593));
#37247=CARTESIAN_POINT('Ctrl Pts',(104.775955600921,4.39822630139848,-6.58062486614574));
#37248=CARTESIAN_POINT('Ctrl Pts',(104.974467205363,7.91410602868588,0.138122348868092));
#37249=CARTESIAN_POINT('Ctrl Pts',(105.139893542398,4.80113115722892,5.60750452802011));
#37250=CARTESIAN_POINT('Ctrl Pts',(105.272234612026,0.396450421808572,6.95551228352529));
#37251=CARTESIAN_POINT('Ctrl Pts',(105.371490414247,-2.98449145875099,6.31734756632467));
#37252=CARTESIAN_POINT('Ctrl Pts',(105.470746216468,-5.62458357868699,4.11100760866382));
#37253=CARTESIAN_POINT('Ctrl Pts',(105.603087286096,-7.38059724382454,-0.147484225780056));
#37254=CARTESIAN_POINT('Ctrl Pts',(105.768513623131,-5.13271570250706,-6.02556078732482));
#37255=CARTESIAN_POINT('Ctrl Pts',(105.967025227573,2.29003833747114,-7.57659160585189));
#37256=CARTESIAN_POINT('Ctrl Pts',(106.165536832016,7.60683954109075,-2.18746683219334));
#37257=CARTESIAN_POINT('Ctrl Pts',(106.364048436458,5.95566578760469,5.2136555188432));
#37258=CARTESIAN_POINT('Ctrl Pts',(106.529474773493,0.0477558832100018,
7.38191519310475));
#37259=CARTESIAN_POINT('Ctrl Pts',(106.661815843121,-4.1866225994409,5.56853027965365));
#37260=CARTESIAN_POINT('Ctrl Pts',(106.761071645342,-6.35709302850648,2.89886612808133));
#37261=CARTESIAN_POINT('Ctrl Pts',(106.860327447563,-6.94952053876253,-0.490380316337293));
#37262=CARTESIAN_POINT('Ctrl Pts',(106.992668517191,-5.54212909806882,-4.87646479313282));
#37263=CARTESIAN_POINT('Ctrl Pts',(107.158094854226,-0.0311838539981387,
-7.91522488447879));
#37264=CARTESIAN_POINT('Ctrl Pts',(107.356606458668,6.63944075859768,-4.30895947104066));
#37265=CARTESIAN_POINT('Ctrl Pts',(107.55511806311,7.22203490733478,3.23911481438212));
#37266=CARTESIAN_POINT('Ctrl Pts',(107.753629667553,1.18378367673741,7.82613616286123));
#37267=CARTESIAN_POINT('Ctrl Pts',(107.919056004588,-4.72814509520211,5.66941723656927));
#37268=CARTESIAN_POINT('Ctrl Pts',(108.051397074216,-6.79200634781696,1.55063442080293));
#37269=CARTESIAN_POINT('Ctrl Pts',(108.150652876437,-6.72653659654391,-1.88821083607211));
#37270=CARTESIAN_POINT('Ctrl Pts',(108.249908678658,-4.99173439974838,-4.86161506097717));
#37271=CARTESIAN_POINT('Ctrl Pts',(108.382249748286,-1.08518063725679,-7.29858638145808));
#37272=CARTESIAN_POINT('Ctrl Pts',(108.547676085321,5.08426806181123,-6.07244981975362));
#37273=CARTESIAN_POINT('Ctrl Pts',(108.746187689763,7.85362119325993,1.00557868191725));
#37274=CARTESIAN_POINT('Ctrl Pts',(108.911614026798,4.16266766862485,6.094569780456));
#37275=CARTESIAN_POINT('Ctrl Pts',(109.043955096426,-0.366836423285678,
6.95826883443441));
#37276=CARTESIAN_POINT('Ctrl Pts',(109.143210898647,-3.64721232954971,5.9546908966592));
#37277=CARTESIAN_POINT('Ctrl Pts',(109.242466700868,-6.05449046306688,3.4721993705992));
#37278=CARTESIAN_POINT('Ctrl Pts',(109.308637235682,-6.66841279098075,1.26337808959281));
#37279=CARTESIAN_POINT('Ctrl Pts',(109.341722503089,-6.69339752173825,0.15023467065256));
#37280=CARTESIAN_POINT('Ctrl Pts',(31.067,0.728796816009639,-6.89458803707475));
#37281=CARTESIAN_POINT('Ctrl Pts',(31.100085267407,1.87539916180617,-6.77338570644206));
#37282=CARTESIAN_POINT('Ctrl Pts',(31.166255802221,4.10223773170205,-5.95048895222621));
#37283=CARTESIAN_POINT('Ctrl Pts',(31.2655116044422,6.457772812735,-3.25342220167339));
#37284=CARTESIAN_POINT('Ctrl Pts',(31.3647674066631,7.21225375876819,0.217893466371651));
#37285=CARTESIAN_POINT('Ctrl Pts',(31.4971084762913,5.93266321869853,4.81822422049041));
#37286=CARTESIAN_POINT('Ctrl Pts',(31.6625348133263,0.364527573010722,8.19099424626465));
#37287=CARTESIAN_POINT('Ctrl Pts',(31.8610464177684,-6.70248217457009,4.72634364857896));
#37288=CARTESIAN_POINT('Ctrl Pts',(32.0264727548035,-7.43898861096156,-1.74552100244657));
#37289=CARTESIAN_POINT('Ctrl Pts',(32.1588138244316,-4.58920855911997,-5.56811746148175));
#37290=CARTESIAN_POINT('Ctrl Pts',(32.2580696266526,-1.37200169140237,-7.10352230210452));
#37291=CARTESIAN_POINT('Ctrl Pts',(32.3573254288737,2.18243696783098,-6.87630845685192));
#37292=CARTESIAN_POINT('Ctrl Pts',(32.4896664985018,6.25603295742458,-4.39337904789581));
#37293=CARTESIAN_POINT('Ctrl Pts',(32.6550928355369,7.97495827693072,1.89249908165876));
#37294=CARTESIAN_POINT('Ctrl Pts',(32.853604439979,2.72363629353246,7.73066701466195));
#37295=CARTESIAN_POINT('Ctrl Pts',(33.0521160444211,-5.01590101849566,6.48242017314943));
#37296=CARTESIAN_POINT('Ctrl Pts',(33.2506276488632,-8.16569697464416,-0.710673422495908));
#37297=CARTESIAN_POINT('Ctrl Pts',(33.4160539858983,-4.55735344058351,-6.13738783143792));
#37298=CARTESIAN_POINT('Ctrl Pts',(33.5483950555264,0.0896484826078498,
-7.21381584413317));
#37299=CARTESIAN_POINT('Ctrl Pts',(33.6476508577474,3.53650717330565,-6.31191543516737));
#37300=CARTESIAN_POINT('Ctrl Pts',(33.7469066599685,6.10550017679619,-3.84318556859557));
#37301=CARTESIAN_POINT('Ctrl Pts',(33.8792477295966,7.61391039016358,0.682060208615401));
#37302=CARTESIAN_POINT('Ctrl Pts',(34.0446740666317,4.86987989748413,6.59305422815555));
#37303=CARTESIAN_POINT('Ctrl Pts',(34.2431856710737,-2.9094840048122,7.66261248374723));
#37304=CARTESIAN_POINT('Ctrl Pts',(34.4416972755159,-8.01520842963098,1.71381383651624));
#37305=CARTESIAN_POINT('Ctrl Pts',(34.640208879958,-5.77829476061933,-5.81338094144534));
#37306=CARTESIAN_POINT('Ctrl Pts',(34.8056352169931,0.480462945019444,-7.62928625176653));
#37307=CARTESIAN_POINT('Ctrl Pts',(34.9379762866211,4.72462479779841,-5.45207418673285));
#37308=CARTESIAN_POINT('Ctrl Pts',(35.0372320888422,6.77521962502725,-2.53841926317347));
#37309=CARTESIAN_POINT('Ctrl Pts',(35.1364878910633,7.14398017959929,1.00535550296516));
#37310=CARTESIAN_POINT('Ctrl Pts',(35.2688289606914,5.3752915948991,5.43535590203058));
#37311=CARTESIAN_POINT('Ctrl Pts',(35.4342552977264,-0.535856550938932,
8.17905524544786));
#37312=CARTESIAN_POINT('Ctrl Pts',(35.6327669021686,-7.16810227628201,3.97480015051313));
#37313=CARTESIAN_POINT('Ctrl Pts',(35.8312785066107,-7.22821962006094,-3.86439744694054));
#37314=CARTESIAN_POINT('Ctrl Pts',(36.0297901110528,-0.66123344041058,-8.16987498632177));
#37315=CARTESIAN_POINT('Ctrl Pts',(36.1952164480879,5.29129882300858,-5.51715599066038));
#37316=CARTESIAN_POINT('Ctrl Pts',(36.327557517716,7.12772108930233,-1.11480251529127));
#37317=CARTESIAN_POINT('Ctrl Pts',(36.426813319937,6.81335378601919,2.434211034571));
#37318=CARTESIAN_POINT('Ctrl Pts',(36.5260691221581,4.80768609485547,5.37897267026131));
#37319=CARTESIAN_POINT('Ctrl Pts',(36.6584101917861,0.597414649385422,7.62102022027007));
#37320=CARTESIAN_POINT('Ctrl Pts',(36.8238365288213,-5.68845683170082,5.90131729619776));
#37321=CARTESIAN_POINT('Ctrl Pts',(37.0223481332633,-8.04055017571803,-1.59068518751364));
#37322=CARTESIAN_POINT('Ctrl Pts',(37.2208597377055,-3.02666088894786,-7.61708936256067));
#37323=CARTESIAN_POINT('Ctrl Pts',(37.4193713421476,4.76819069205422,-6.66696666264346));
#37324=CARTESIAN_POINT('Ctrl Pts',(37.5847976791826,7.60255533599256,-0.798752667796797));
#37325=CARTESIAN_POINT('Ctrl Pts',(37.7171387488107,6.16372253201031,3.74909550721544));
#37326=CARTESIAN_POINT('Ctrl Pts',(37.8163945510318,3.63289845491171,6.25693391296819));
#37327=CARTESIAN_POINT('Ctrl Pts',(37.9156503532529,0.200268489030504,7.21159379791598));
#37328=CARTESIAN_POINT('Ctrl Pts',(38.0479914228809,-4.46267756834381,6.20655801407927));
#37329=CARTESIAN_POINT('Ctrl Pts',(38.213417759916,-8.15386252187664,0.835830683175351));
#37330=CARTESIAN_POINT('Ctrl Pts',(38.4119293643581,-5.1146879884136,-6.4047399069065));
#37331=CARTESIAN_POINT('Ctrl Pts',(38.6104409688002,2.60467519869591,-7.77151166783153));
#37332=CARTESIAN_POINT('Ctrl Pts',(38.8089525732423,7.94514871250055,-2.01462127777205));
#37333=CARTESIAN_POINT('Ctrl Pts',(38.9743789102775,6.32240802964781,4.29697686377015));
#37334=CARTESIAN_POINT('Ctrl Pts',(39.1067199799055,2.2880165733667,6.84194217556962));
#37335=CARTESIAN_POINT('Ctrl Pts',(39.2059757821266,-1.26371740502772,7.12391686470159));
#37336=CARTESIAN_POINT('Ctrl Pts',(39.3052315843476,-4.50175480980351,5.6374991092017));
#37337=CARTESIAN_POINT('Ctrl Pts',(39.4375726539757,-7.41462633243902,1.86015316880977));
#37338=CARTESIAN_POINT('Ctrl Pts',(39.6029989910108,-6.76743001979327,-4.62449758177058));
#37339=CARTESIAN_POINT('Ctrl Pts',(39.8015105954529,0.22732365963109,-8.19323199035126));
#37340=CARTESIAN_POINT('Ctrl Pts',(40.000022199895,7.00557756467603,-4.25471614555553));
#37341=CARTESIAN_POINT('Ctrl Pts',(40.1985338043371,7.36886375493194,3.58941971881967));
#37342=CARTESIAN_POINT('Ctrl Pts',(40.3639601413722,2.05559119702074,7.3628390103181));
#37343=CARTESIAN_POINT('Ctrl Pts',(40.4963012110003,-2.66853537675076,6.70269434756417));
#37344=CARTESIAN_POINT('Ctrl Pts',(40.5955570132213,-5.56336036386177,4.62560208370343));
#37345=CARTESIAN_POINT('Ctrl Pts',(40.6948128154424,-7.07717478879668,1.40028196541262));
#37346=CARTESIAN_POINT('Ctrl Pts',(40.8271538850705,-6.86394786779064,-3.36497743371087));
#37347=CARTESIAN_POINT('Ctrl Pts',(40.9925802221056,-2.18410213914716,-7.90023954082243));
#37348=CARTESIAN_POINT('Ctrl Pts',(41.1910918265477,5.46194890622252,-6.11128796897657));
#37349=CARTESIAN_POINT('Ctrl Pts',(41.3896034309898,8.09708500892483,1.27198303926893));
#37350=CARTESIAN_POINT('Ctrl Pts',(41.5881150354319,3.31156954946564,7.49783929380012));
#37351=CARTESIAN_POINT('Ctrl Pts',(41.753541372467,-3.18227520372151,6.95053796399318));
#37352=CARTESIAN_POINT('Ctrl Pts',(41.8858824420951,-6.36448642098304,3.39713190367425));
#37353=CARTESIAN_POINT('Ctrl Pts',(41.9851382443162,-7.23490358845545,-0.0578207636081432));
#37354=CARTESIAN_POINT('Ctrl Pts',(42.0843940465372,-6.30937772536576,-3.49842039962285));
#37355=CARTESIAN_POINT('Ctrl Pts',(42.2167351161653,-3.07077954317236,-7.00051187116809));
#37356=CARTESIAN_POINT('Ctrl Pts',(42.3821614532003,3.43098314638184,-7.44395335865592));
#37357=CARTESIAN_POINT('Ctrl Pts',(42.5806730576425,8.11638061329028,-1.14240633495646));
#37358=CARTESIAN_POINT('Ctrl Pts',(42.7791846620846,5.3635756345066,6.19780468447261));
#37359=CARTESIAN_POINT('Ctrl Pts',(42.9776962665267,-2.31009124088029,7.86432231126175));
#37360=CARTESIAN_POINT('Ctrl Pts',(43.1431226035618,-6.91685293175678,3.25484238966784));
#37361=CARTESIAN_POINT('Ctrl Pts',(43.2754636731899,-7.05389034664051,-1.51321629366424));
#37362=CARTESIAN_POINT('Ctrl Pts',(43.3747194754109,-5.48871958445089,-4.71392941167078));
#37363=CARTESIAN_POINT('Ctrl Pts',(43.473975277632,-2.56106657714424,-6.74448890289501));
#37364=CARTESIAN_POINT('Ctrl Pts',(43.6063163472601,2.17300753944422,-7.32904439164134));
#37365=CARTESIAN_POINT('Ctrl Pts',(43.7717426842951,7.42529154430146,-3.47118602767502));
#37366=CARTESIAN_POINT('Ctrl Pts',(43.9702542887373,6.93668036814076,4.36614154193306));
#37367=CARTESIAN_POINT('Ctrl Pts',(44.1687658931793,0.0963436935637944,
8.19581871362791));
#37368=CARTESIAN_POINT('Ctrl Pts',(44.3672774976216,-6.84047809260716,4.51574428208274));
#37369=CARTESIAN_POINT('Ctrl Pts',(44.5327038346565,-7.38394874907302,-1.9784221824965));
#37370=CARTESIAN_POINT('Ctrl Pts',(44.6650449042847,-4.41107666766695,-5.70872973662297));
#37371=CARTESIAN_POINT('Ctrl Pts',(44.7643007065056,-1.14969572507477,-7.14320466700307));
#37372=CARTESIAN_POINT('Ctrl Pts',(44.8635565087267,2.39707782841684,-6.80449928050194));
#37373=CARTESIAN_POINT('Ctrl Pts',(44.9958975783549,6.3902782428573,-4.19537810453311));
#37374=CARTESIAN_POINT('Ctrl Pts',(45.1613239153898,7.91193452816724,2.14134980295047));
#37375=CARTESIAN_POINT('Ctrl Pts',(45.3598355198321,2.4801318443069,7.81214903395972));
#37376=CARTESIAN_POINT('Ctrl Pts',(45.5583471242741,-5.21640045922418,6.32217468462786));
#37377=CARTESIAN_POINT('Ctrl Pts',(45.7568587287163,-8.1394620724232,-0.966045613925907));
#37378=CARTESIAN_POINT('Ctrl Pts',(45.9222850657513,-4.362909253218,-6.27709138927544));
#37379=CARTESIAN_POINT('Ctrl Pts',(46.0546261353795,0.315504493512712,-7.20747178200597));
#37380=CARTESIAN_POINT('Ctrl Pts',(46.1538819376004,3.73243784352554,-6.19807074170408));
#37381=CARTESIAN_POINT('Ctrl Pts',(46.2531377398216,6.22285632708154,-3.65010297201878));
#37382=CARTESIAN_POINT('Ctrl Pts',(46.3854788094495,7.58881791801145,0.920160892670061));
#37383=CARTESIAN_POINT('Ctrl Pts',(46.5509051464848,4.66102472543446,6.74232418869707));
#37384=CARTESIAN_POINT('Ctrl Pts',(46.7494167509267,-3.14801683026386,7.56774183824466));
#37385=CARTESIAN_POINT('Ctrl Pts',(46.947928355369,-8.06494675964391,1.46197136020253));
#37386=CARTESIAN_POINT('Ctrl Pts',(47.146439959811,-5.59341055025238,-5.99148106672523));
#37387=CARTESIAN_POINT('Ctrl Pts',(47.3118662968461,0.719143712729369,-7.61049839245583));
#37388=CARTESIAN_POINT('Ctrl Pts',(47.4442073664742,4.89304312979347,-5.30144522784307));
#37389=CARTESIAN_POINT('Ctrl Pts',(47.5434631686953,6.85138904336245,-2.32500351643662));
#37390=CARTESIAN_POINT('Ctrl Pts',(47.6427189709163,7.10899295648094,1.22858118109606));
#37391=CARTESIAN_POINT('Ctrl Pts',(47.7750600405444,5.20244325199208,5.60102112752069));
#37392=CARTESIAN_POINT('Ctrl Pts',(47.9404863775795,-0.791726597716949,
8.15826304743041));
#37393=CARTESIAN_POINT('Ctrl Pts',(48.1389979820216,-7.28906029253489,3.74837652134022));
#37394=CARTESIAN_POINT('Ctrl Pts',(48.3375095864638,-7.10365816722376,-4.08885890404384));
#37395=CARTESIAN_POINT('Ctrl Pts',(48.5360211909057,-0.405063757024925,
-8.18657500480791));
#37396=CARTESIAN_POINT('Ctrl Pts',(48.701447527941,5.46147728667374,-5.34874932187685));
#37397=CARTESIAN_POINT('Ctrl Pts',(48.833788597569,7.15913607354485,-0.891046157226271));
#37398=CARTESIAN_POINT('Ctrl Pts',(48.93304439979,6.73378310032549,2.64638212144819));
#37399=CARTESIAN_POINT('Ctrl Pts',(49.0323002020111,4.63688182235142,5.52689058507458));
#37400=CARTESIAN_POINT('Ctrl Pts',(49.1646412716391,0.358464038768738,7.63599089798048));
#37401=CARTESIAN_POINT('Ctrl Pts',(49.3300676086743,-5.87047078759569,5.72028493071691));
#37402=CARTESIAN_POINT('Ctrl Pts',(49.5285792131163,-7.9867932078012,-1.84170050490409));
#37403=CARTESIAN_POINT('Ctrl Pts',(49.7270908175585,-2.78664193532054,-7.70813552152894));
#37404=CARTESIAN_POINT('Ctrl Pts',(49.9256024220006,4.97463284684977,-6.51437756010842));
#37405=CARTESIAN_POINT('Ctrl Pts',(50.0910287590356,7.62384011148192,-0.560281550374918));
#37406=CARTESIAN_POINT('Ctrl Pts',(50.2233698286638,6.04329393099642,3.94027804062365));
#37407=CARTESIAN_POINT('Ctrl Pts',(50.3226256308848,3.43517639175237,6.36763192501709));
#37408=CARTESIAN_POINT('Ctrl Pts',(50.4218814331059,-0.0256658623535902,
7.21432837049636));
#37409=CARTESIAN_POINT('Ctrl Pts',(50.554222502734,-4.65485154373645,6.06376208033474));
#37410=CARTESIAN_POINT('Ctrl Pts',(50.719648839769,-8.17603802906677,0.580076808582549));
#37411=CARTESIAN_POINT('Ctrl Pts',(50.9181604442112,-4.9116105227764,-6.56176870717763));
#37412=CARTESIAN_POINT('Ctrl Pts',(51.1166720486532,2.84676806773059,-7.68613284184527));
#37413=CARTESIAN_POINT('Ctrl Pts',(51.3151836530954,8.00434124077968,-1.76482527683466));
#37414=CARTESIAN_POINT('Ctrl Pts',(51.4806099901304,6.18474431048777,4.49286003287664));
#37415=CARTESIAN_POINT('Ctrl Pts',(51.6129510597586,2.07263417189446,6.91023734493501));
#37416=CARTESIAN_POINT('Ctrl Pts',(51.7122068619796,-1.48618806964884,7.08084869182948));
#37417=CARTESIAN_POINT('Ctrl Pts',(51.8114626642006,-4.67608913993433,5.4937585430402));
#37418=CARTESIAN_POINT('Ctrl Pts',(51.9438037338288,-7.46924178168058,1.62704660902152));
#37419=CARTESIAN_POINT('Ctrl Pts',(52.1092300708638,-6.61929149505301,-4.83415629247963));
#37420=CARTESIAN_POINT('Ctrl Pts',(52.307741675306,0.483788985420524,-8.18209476304991));
#37421=CARTESIAN_POINT('Ctrl Pts',(52.506253279748,7.13538105729948,-4.03324480549778));
#37422=CARTESIAN_POINT('Ctrl Pts',(52.7047648841902,7.25284444363329,3.81842041072731));
#37423=CARTESIAN_POINT('Ctrl Pts',(52.8701912212252,1.82401053969385,7.42360013822247));
#37424=CARTESIAN_POINT('Ctrl Pts',(53.0025322908534,-2.87712615953718,6.61583990404437));
#37425=CARTESIAN_POINT('Ctrl Pts',(53.1017880930744,-5.70548575568047,4.44911288536006));
#37426=CARTESIAN_POINT('Ctrl Pts',(53.2010438952954,-7.11755455352814,1.17796848488831));
#37427=CARTESIAN_POINT('Ctrl Pts',(53.3333849649235,-6.75520476387417,-3.57827640900797));
#37428=CARTESIAN_POINT('Ctrl Pts',(53.4988113019586,-1.93562937742725,-7.96476150740508));
#37429=CARTESIAN_POINT('Ctrl Pts',(53.6973229064007,5.65064933367531,-5.93724587681677));
#37430=CARTESIAN_POINT('Ctrl Pts',(53.8958345108428,8.05328069487987,1.52492509436311));
#37431=CARTESIAN_POINT('Ctrl Pts',(54.094346115285,3.07514526013486,7.59786605473347));
#37432=CARTESIAN_POINT('Ctrl Pts',(54.25977245232,-3.39837541630809,6.84747384010805));
#37433=CARTESIAN_POINT('Ctrl Pts',(54.3921135219481,-6.46774848790643,3.19615739146608));
#37434=CARTESIAN_POINT('Ctrl Pts',(54.4913693241692,-7.22954448224845,-0.284358495812285));
#37435=CARTESIAN_POINT('Ctrl Pts',(54.5906251263902,-6.19672775393435,-3.69428717311731));
#37436=CARTESIAN_POINT('Ctrl Pts',(54.7229661960184,-2.85004750873798,-7.09324204148341));
#37437=CARTESIAN_POINT('Ctrl Pts',(54.8883925330533,3.66241302831517,-7.33285877176346));
#37438=CARTESIAN_POINT('Ctrl Pts',(55.0869041374955,8.1481751357478,-0.887675870531769));
#37439=CARTESIAN_POINT('Ctrl Pts',(55.2854157419376,5.16685642213818,6.36272906911433));
#37440=CARTESIAN_POINT('Ctrl Pts',(55.4839273463797,-2.55523502117791,7.7881230693375));
#37441=CARTESIAN_POINT('Ctrl Pts',(55.6493536834148,-7.01538819057916,3.03663991882703));
#37442=CARTESIAN_POINT('Ctrl Pts',(55.7816947530428,-7.0030432857035,-1.73337166020505));
#37443=CARTESIAN_POINT('Ctrl Pts',(55.880950555264,-5.33840759145258,-4.88350054392042));
#37444=CARTESIAN_POINT('Ctrl Pts',(55.980206357485,-2.34860207414178,-6.82138262166666));
#37445=CARTESIAN_POINT('Ctrl Pts',(56.1125474271131,2.40145594912496,-7.25740055292139));
#37446=CARTESIAN_POINT('Ctrl Pts',(56.2779737641482,7.53035238897762,-3.23695533710616));
#37447=CARTESIAN_POINT('Ctrl Pts',(56.4764853685902,6.79654943436846,4.58122715875659));
#37448=CARTESIAN_POINT('Ctrl Pts',(56.6749969730324,-0.160361382168487,
8.19481608829948));
#37449=CARTESIAN_POINT('Ctrl Pts',(56.8735085774745,-6.97853683895954,4.29931512498043));
#37450=CARTESIAN_POINT('Ctrl Pts',(57.0389349145096,-7.31837155934601,-2.20868539644884));
#37451=CARTESIAN_POINT('Ctrl Pts',(57.1712759841377,-4.23014034071495,-5.84406581685175));
#37452=CARTESIAN_POINT('Ctrl Pts',(57.2705317863588,-0.925437374256124,
-7.17570476268915));
#37453=CARTESIAN_POINT('Ctrl Pts',(57.3697875885798,2.60898984245657,-6.72609578996594));
#37454=CARTESIAN_POINT('Ctrl Pts',(57.5021286582079,6.51852530081687,-3.99320439794175));
#37455=CARTESIAN_POINT('Ctrl Pts',(57.667554995243,7.84099619122865,2.38806735368569));
#37456=CARTESIAN_POINT('Ctrl Pts',(57.8660665996851,2.2342725089119,7.88598458341533));
#37457=CARTESIAN_POINT('Ctrl Pts',(58.0645782041272,-5.41182538332481,6.15571868382113));
#37458=CARTESIAN_POINT('Ctrl Pts',(58.2630898085693,-8.10521761975249,-1.2204647856676));
#37459=CARTESIAN_POINT('Ctrl Pts',(58.4285161456044,-4.16419790569076,-6.41064031617526));
#37460=CARTESIAN_POINT('Ctrl Pts',(58.5608572152325,0.54105679665563,-7.19405658280721));
#37461=CARTESIAN_POINT('Ctrl Pts',(58.6601130174535,3.92470418512737,-6.07814694081951));
#37462=CARTESIAN_POINT('Ctrl Pts',(58.7593688196745,6.33410982426262,-3.4534396343383));
#37463=CARTESIAN_POINT('Ctrl Pts',(58.8917098893027,7.55628044485889,1.15735876018381));
#37464=CARTESIAN_POINT('Ctrl Pts',(59.0571362263377,4.44759807302352,6.88498063449988));
#37465=CARTESIAN_POINT('Ctrl Pts',(59.2556478307798,-3.383462018219,7.4654478275059));
#37466=CARTESIAN_POINT('Ctrl Pts',(59.454159435222,-8.10677391155581,1.20869485018397));
#37467=CARTESIAN_POINT('Ctrl Pts',(59.6526710396641,-5.40303978286539,-6.16370408612994));
#37468=CARTESIAN_POINT('Ctrl Pts',(59.8180973766991,0.957119109800075,-7.58424528023631));
#37469=CARTESIAN_POINT('Ctrl Pts',(59.9504384463273,5.05666178638522,-5.14561601287451));
#37470=CARTESIAN_POINT('Ctrl Pts',(60.0496942485483,6.92083785156421,-2.10930713915861));
#37471=CARTESIAN_POINT('Ctrl Pts',(60.1489500507693,7.06703241868983,1.45060172584553));
#37472=CARTESIAN_POINT('Ctrl Pts',(60.2812911203974,5.02449176463669,5.76119223496576));
#37473=CARTESIAN_POINT('Ctrl Pts',(60.4467174574326,-1.04682003116853,8.12946829620154));
#37474=CARTESIAN_POINT('Ctrl Pts',(60.6452290618746,-7.4028683678955,3.51827605817898));
#37475=CARTESIAN_POINT('Ctrl Pts',(60.8437406663167,-6.97212863872708,-4.30930954318493));
#37476=CARTESIAN_POINT('Ctrl Pts',(61.0422522707589,-0.148496740647099,
-8.19524469888595));
#37477=CARTESIAN_POINT('Ctrl Pts',(61.2076786077939,5.62629851176496,-5.1750959911525));
#37478=CARTESIAN_POINT('Ctrl Pts',(61.340019677422,7.1835285625583,-0.666415759678704));
#37479=CARTESIAN_POINT('Ctrl Pts',(61.4392754796431,6.64760715387227,2.85595733559444));
#37480=CARTESIAN_POINT('Ctrl Pts',(61.5385312818641,4.46152916853726,5.66938709669134));
#37481=CARTESIAN_POINT('Ctrl Pts',(61.6708723514923,0.119161805817699,7.64347132690151));
#37482=CARTESIAN_POINT('Ctrl Pts',(61.8362986885272,-6.04672631772197,5.53364145885595));
#37483=CARTESIAN_POINT('Ctrl Pts',(62.0348102929695,-7.92520188427845,-2.09090927286969));
#37484=CARTESIAN_POINT('Ctrl Pts',(62.2333218974115,-2.5438895261837,-7.79162066405417));
#37485=CARTESIAN_POINT('Ctrl Pts',(62.4318335018536,5.17619531567503,-6.35539841477975));
#37486=CARTESIAN_POINT('Ctrl Pts',(62.5972598388888,7.63764655705976,-0.321260845052877));
#37487=CARTESIAN_POINT('Ctrl Pts',(62.7296009085168,5.91693737961713,4.12759550095798));
#37488=CARTESIAN_POINT('Ctrl Pts',(62.8288567107379,3.23408471669311,6.47208383908938));
#37489=CARTESIAN_POINT('Ctrl Pts',(62.9281125129589,-0.251575037739509,
7.20998630887921));
#37490=CARTESIAN_POINT('Ctrl Pts',(63.060453582587,-4.84245951105093,5.91501811873503));
#37491=CARTESIAN_POINT('Ctrl Pts',(63.2258799196221,-8.19019354779154,0.323753928647688));
#37492=CARTESIAN_POINT('Ctrl Pts',(63.4243915240641,-4.70371519063712,-6.71236097802501));
#37493=CARTESIAN_POINT('Ctrl Pts',(63.6229031285063,3.0860685027055,-7.59321458214847));
#37494=CARTESIAN_POINT('Ctrl Pts',(63.8214147329484,8.05568220034109,-1.51329813444295));
#37495=CARTESIAN_POINT('Ctrl Pts',(63.9868410699835,6.04101389033449,4.68433609361207));
#37496=CARTESIAN_POINT('Ctrl Pts',(64.1191821396116,1.85521869497751,6.9717541671838));
#37497=CARTESIAN_POINT('Ctrl Pts',(64.2184379418327,-1.70720091189527,7.0308348168176));
#37498=CARTESIAN_POINT('Ctrl Pts',(64.3176937440536,-4.84583662973596,5.34462907335459));
#37499=CARTESIAN_POINT('Ctrl Pts',(64.4500348136819,-7.51653054864387,1.39234405677461));
#37500=CARTESIAN_POINT('Ctrl Pts',(64.6154611507168,-6.46466001599287,-5.0390731126098));
#37501=CARTESIAN_POINT('Ctrl Pts',(64.813972755159,0.739779755921552,-8.16293160614863));
#37502=CARTESIAN_POINT('Ctrl Pts',(65.012484359601,7.25818535623405,-3.80781719998572));
#37503=CARTESIAN_POINT('Ctrl Pts',(65.2109959640432,7.12971071718912,4.04367556139354));
#37504=CARTESIAN_POINT('Ctrl Pts',(65.3764223010783,1.59064068527316,7.47707935436174));
#37505=CARTESIAN_POINT('Ctrl Pts',(65.5087633707064,-3.08289472959458,6.52249589192415));
#37506=CARTESIAN_POINT('Ctrl Pts',(65.6080191729274,-5.84201455782888,4.26825949081232));
#37507=CARTESIAN_POINT('Ctrl Pts',(65.7072749751485,-7.15095261084027,0.95449951885552));
#37508=CARTESIAN_POINT('Ctrl Pts',(65.8396160447767,-6.63983538642403,-3.7880654036783));
#37509=CARTESIAN_POINT('Ctrl Pts',(66.0050423818115,-1.6852579301835,-8.02147072946674));
#37510=CARTESIAN_POINT('Ctrl Pts',(66.2035539862539,5.83380696131112,-5.75737985847315));
#37511=CARTESIAN_POINT('Ctrl Pts',(66.4020655906958,8.00157680664466,1.77637132973648));
#37512=CARTESIAN_POINT('Ctrl Pts',(66.600577195138,2.83570451857797,7.69043996340305));
#37513=CARTESIAN_POINT('Ctrl Pts',(66.7660035321731,-3.61114211588056,6.73769293585757));
#37514=CARTESIAN_POINT('Ctrl Pts',(66.8983446018012,-6.56466625071433,2.99204772276496));
#37515=CARTESIAN_POINT('Ctrl Pts',(66.9976004040222,-7.2170938170707,-0.510617293293015));
#37516=CARTESIAN_POINT('Ctrl Pts',(67.0968562062432,-6.07799932508554,-3.88653017593029));
#37517=CARTESIAN_POINT('Ctrl Pts',(67.2291972758714,-2.62651982706667,-7.17901433868201));
#37518=CARTESIAN_POINT('Ctrl Pts',(67.3946236129064,3.89025040628289,-7.21457131145677));
#37519=CARTESIAN_POINT('Ctrl Pts',(67.5931352173485,8.17197698838295,-0.632074624543493));
#37520=CARTESIAN_POINT('Ctrl Pts',(67.7916468217907,4.96506899196963,6.52141207658738));
#37521=CARTESIAN_POINT('Ctrl Pts',(67.9901584262327,-2.79787238141651,7.70428452457515));
#37522=CARTESIAN_POINT('Ctrl Pts',(68.1555847632679,-7.10704187889876,2.81545845931199));
#37523=CARTESIAN_POINT('Ctrl Pts',(68.2879258328959,-6.94532695410545,-1.95182630988612));
#37524=CARTESIAN_POINT('Ctrl Pts',(68.3871816351171,-5.18285883819335,-5.04828231948625));
#37525=CARTESIAN_POINT('Ctrl Pts',(68.486437437338,-2.13383424279239,-6.89158342391702));
#37526=CARTESIAN_POINT('Ctrl Pts',(68.6187785069662,2.62754970512971,-7.17864156401975));
#37527=CARTESIAN_POINT('Ctrl Pts',(68.7842048440012,7.62802463440124,-2.99954185919825));
#37528=CARTESIAN_POINT('Ctrl Pts',(68.9827164484433,6.64975495342578,4.7918063211089));
#37529=CARTESIAN_POINT('Ctrl Pts',(69.1812280528854,-0.416915198702002,
8.18579837023763));
#37530=CARTESIAN_POINT('Ctrl Pts',(69.3797396573275,-7.10973832650691,4.07862272490673));
#37531=CARTESIAN_POINT('Ctrl Pts',(69.5451659943627,-7.24563662171936,-2.43670125431101));
#37532=CARTESIAN_POINT('Ctrl Pts',(69.6775070639907,-4.04502533630726,-5.97378234857353));
#37533=CARTESIAN_POINT('Ctrl Pts',(69.7767628662118,-0.7003351904756,-7.20091934778666));
#37534=CARTESIAN_POINT('Ctrl Pts',(69.8760186684328,2.81846067751086,-6.64155002296871));
#37535=CARTESIAN_POINT('Ctrl Pts',(70.008359738061,6.64012327459028,-3.78612972542153));
#37536=CARTESIAN_POINT('Ctrl Pts',(70.1737860750959,7.76288615048499,2.63043722061295));
#37537=CARTESIAN_POINT('Ctrl Pts',(70.3722976795382,1.98535818899343,7.95541533816283));
#37538=CARTESIAN_POINT('Ctrl Pts',(70.5708092839802,-5.60036139298603,5.97713454909029));
#37539=CARTESIAN_POINT('Ctrl Pts',(70.7693208884224,-8.06606896756193,-1.46200603608502));
#37540=CARTESIAN_POINT('Ctrl Pts',(70.9678324928645,-3.13451622979428,-7.5752150383098));
#37541=CARTESIAN_POINT('Ctrl Pts',(71.1332588298995,3.35153198035595,-6.87266150813771));
#37542=CARTESIAN_POINT('Ctrl Pts',(71.2655998995277,6.4351344135931,-3.24546016726863));
#37543=CARTESIAN_POINT('Ctrl Pts',(71.3979409691556,7.51702449814323,1.38731120573129));
#37544=CARTESIAN_POINT('Ctrl Pts',(71.5633673061908,4.23448854948942,7.02493677792881));
#37545=CARTESIAN_POINT('Ctrl Pts',(71.7618789106328,-3.62636197138777,7.35273307434348));
#37546=CARTESIAN_POINT('Ctrl Pts',(71.9273052476681,-7.36873471237381,2.0246969407879));
#37547=CARTESIAN_POINT('Ctrl Pts',(72.0596463172959,-6.69257905832717,-2.69716983719333));
#37548=CARTESIAN_POINT('Ctrl Pts',(72.1589021195172,-4.60123349955128,-5.58285884611192));
#37549=CARTESIAN_POINT('Ctrl Pts',(72.2581579217382,-1.37052351308357,-7.08310535950425));
#37550=CARTESIAN_POINT('Ctrl Pts',(72.3904989913663,3.39433210286424,-6.84955869054765));
#37551=CARTESIAN_POINT('Ctrl Pts',(72.5559253284013,7.90931691245014,-2.15054133310692));
#37552=CARTESIAN_POINT('Ctrl Pts',(72.7544369328434,6.08809628195235,5.48786961221882));
#37553=CARTESIAN_POINT('Ctrl Pts',(72.9529485372855,-1.30640323031847,8.09160345854923));
#37554=CARTESIAN_POINT('Ctrl Pts',(73.1514601417277,-7.51181763259486,3.27969229408906));
#37555=CARTESIAN_POINT('Ctrl Pts',(73.3168864787628,-6.93696759148421,-3.21177358578175));
#37556=CARTESIAN_POINT('Ctrl Pts',(73.4492275483909,-3.37006034220166,-6.37885915445045));
#37557=CARTESIAN_POINT('Ctrl Pts',(73.5484833506119,0.0885511521900275,
-7.23459307282265));
#37558=CARTESIAN_POINT('Ctrl Pts',(73.647739152833,3.52519199163394,-6.29445949177426));
#37559=CARTESIAN_POINT('Ctrl Pts',(73.780080222461,7.01349237856603,-3.04101410392474));
#37560=CARTESIAN_POINT('Ctrl Pts',(73.9455065594961,7.42931202422622,3.46257383852393));
#37561=CARTESIAN_POINT('Ctrl Pts',(74.1440181639383,1.10791776076921,8.12116023680133));
#37562=CARTESIAN_POINT('Ctrl Pts',(74.3425297683803,-6.22053285582939,5.33719926660008));
#37563=CARTESIAN_POINT('Ctrl Pts',(74.5410413728225,-7.85443827270103,-2.34347769528696));
#37564=CARTESIAN_POINT('Ctrl Pts',(74.7064677098574,-3.22543050411949,-6.9306169413023));
#37565=CARTESIAN_POINT('Ctrl Pts',(74.8388087794857,1.54316722938047,-7.04739863047344));
#37566=CARTESIAN_POINT('Ctrl Pts',(74.9380645817065,4.73720272242289,-5.46864550144068));
#37567=CARTESIAN_POINT('Ctrl Pts',(75.0373203839278,6.75530734053086,-2.53239318636892));
#37568=CARTESIAN_POINT('Ctrl Pts',(75.1696614535558,7.31974743008187,2.20412138298759));
#37569=CARTESIAN_POINT('Ctrl Pts',(75.3350877905909,3.43961240388645,7.43996998991286));
#37570=CARTESIAN_POINT('Ctrl Pts',(75.533599395033,-4.39556885165141,6.91807060949306));
#37571=CARTESIAN_POINT('Ctrl Pts',(75.7321109994751,-8.19615403019618,0.0615273568355724));
#37572=CARTESIAN_POINT('Ctrl Pts',(75.9306226039173,-4.48664549632056,-6.85959905122507));
#37573=CARTESIAN_POINT('Ctrl Pts',(76.0960489409522,2.0097710123082,-7.37547787868233));
#37574=CARTESIAN_POINT('Ctrl Pts',(76.2283900105805,5.72741628337472,-4.38678644242978));
#37575=CARTESIAN_POINT('Ctrl Pts',(76.3276458128014,7.14802407214726,-1.11934134133585));
#37576=CARTESIAN_POINT('Ctrl Pts',(76.4269016150226,6.79425520799035,2.42596140587257));
#37577=CARTESIAN_POINT('Ctrl Pts',(76.5592426846505,4.16819463821222,6.40804236245229));
#37578=CARTESIAN_POINT('Ctrl Pts',(76.7246690216857,-2.17494002259612,7.90276678478469));
#37579=CARTESIAN_POINT('Ctrl Pts',(76.9231806261278,-7.82261403601631,2.44692381113861));
#37580=CARTESIAN_POINT('Ctrl Pts',(77.1216922305699,-6.29995860883805,-5.24320970597619));
#37581=CARTESIAN_POINT('Ctrl Pts',(77.320203835012,1.00061296459978,-8.13528491521204));
#37582=CARTESIAN_POINT('Ctrl Pts',(77.4856301720472,6.2955681948585,-4.33620508798002));
#37583=CARTESIAN_POINT('Ctrl Pts',(77.6179712416751,7.20606650304075,0.346118661139733));
#37584=CARTESIAN_POINT('Ctrl Pts',(77.7172270438963,6.18215959176197,3.75873329154079));
#37585=CARTESIAN_POINT('Ctrl Pts',(77.8164828461173,3.62363562623967,6.23830565314694));
#37586=CARTESIAN_POINT('Ctrl Pts',(77.9488239157453,-0.95238954586989,7.58484064526405));
#37587=CARTESIAN_POINT('Ctrl Pts',(78.1142502527805,-6.76206317771884,4.63234158251969));
#37588=CARTESIAN_POINT('Ctrl Pts',(78.3127618572225,-7.55430092435108,-3.1801358521754));
#37589=CARTESIAN_POINT('Ctrl Pts',(78.5112734616647,-1.4276986401798,-8.071084381096));
#37590=CARTESIAN_POINT('Ctrl Pts',(78.7097850661068,6.01518756313756,-5.56790854243103));
#37591=CARTESIAN_POINT('Ctrl Pts',(78.8752114031419,7.60737483598701,0.751466277302418));
#37592=CARTESIAN_POINT('Ctrl Pts',(79.00755247277,5.28061196900669,4.9155192814821));
#37593=CARTESIAN_POINT('Ctrl Pts',(79.106808274991,2.29587814793631,6.86120373584534));
#37594=CARTESIAN_POINT('Ctrl Pts',(79.2060640772122,-1.25876877679799,7.10370985756017));
#37595=CARTESIAN_POINT('Ctrl Pts',(79.33840514684,-5.62307033548875,5.17860342788263));
#37596=CARTESIAN_POINT('Ctrl Pts',(79.5038314838753,-8.1548262198857,-0.826375386894838));
#37597=CARTESIAN_POINT('Ctrl Pts',(79.7023430883173,-3.71737910263321,-7.30491746026261));
#37598=CARTESIAN_POINT('Ctrl Pts',(79.9008546927595,4.11899803065852,-7.08622478597556));
#37599=CARTESIAN_POINT('Ctrl Pts',(80.0993662972016,8.18822183313877,-0.370283901770539));
#37600=CARTESIAN_POINT('Ctrl Pts',(80.2647926342367,5.32550095363364,5.48414925526085));
#37601=CARTESIAN_POINT('Ctrl Pts',(80.3971337038647,0.860626431278914,7.16285660331288));
#37602=CARTESIAN_POINT('Ctrl Pts',(80.496389506086,-2.67496305039171,6.72248063247407));
#37603=CARTESIAN_POINT('Ctrl Pts',(80.5956453083067,-5.54653798250745,4.61336200426993));
#37604=CARTESIAN_POINT('Ctrl Pts',(80.7279863779351,-7.63744474051541,0.326023460360154));
#37605=CARTESIAN_POINT('Ctrl Pts',(80.8934127149699,-5.69529582435376,-5.89471733246808));
#37606=CARTESIAN_POINT('Ctrl Pts',(81.0919243194123,1.87561142445985,-7.97889768566929));
#37607=CARTESIAN_POINT('Ctrl Pts',(81.2904359238541,7.71990350306442,-2.75387298133316));
#37608=CARTESIAN_POINT('Ctrl Pts',(81.4889475282964,6.49318676803834,5.00226074410088));
#37609=CARTESIAN_POINT('Ctrl Pts',(81.6543738653314,0.527890767039223,7.62615137531419));
#37610=CARTESIAN_POINT('Ctrl Pts',(81.7867149349596,-3.96591412848519,6.02650128178202));
#37611=CARTESIAN_POINT('Ctrl Pts',(81.8859707371805,-6.38216694643353,3.4080959849747));
#37612=CARTESIAN_POINT('Ctrl Pts',(81.9852265394017,-7.21415425106946,-0.0563117715569949));
#37613=CARTESIAN_POINT('Ctrl Pts',(82.1175676090296,-6.04393377050729,-4.68056813205964));
#37614=CARTESIAN_POINT('Ctrl Pts',(82.2829939460648,-0.5453401348518,-8.17842839999966));
#37615=CARTESIAN_POINT('Ctrl Pts',(82.4815055505069,6.58257380241805,-4.88369211044909));
#37616=CARTESIAN_POINT('Ctrl Pts',(82.6800171549491,7.67397055088154,2.87939272732047));
#37617=CARTESIAN_POINT('Ctrl Pts',(82.8785287593911,1.73080727378638,8.01176591879775));
#37618=CARTESIAN_POINT('Ctrl Pts',(83.0439550964263,-4.51909200982883,6.16560304170094));
#37619=CARTESIAN_POINT('Ctrl Pts',(83.1762961660543,-6.91897945288657,2.04326109549728));
#37620=CARTESIAN_POINT('Ctrl Pts',(83.2755519682754,-7.07447154442634,-1.5162537855029));
#37621=CARTESIAN_POINT('Ctrl Pts',(83.3748077704965,-5.47384515977853,-4.69938418738115));
#37622=CARTESIAN_POINT('Ctrl Pts',(83.5071488401244,-1.59530292740683,-7.47608601013512));
#37623=CARTESIAN_POINT('Ctrl Pts',(83.6725751771596,4.86223112684713,-6.59869649443888));
#37624=CARTESIAN_POINT('Ctrl Pts',(83.8710867816016,8.17996582553711,0.518541789046997));
#37625=CARTESIAN_POINT('Ctrl Pts',(84.0695983860439,4.00289763898197,7.1524497192064));
#37626=CARTESIAN_POINT('Ctrl Pts',(84.2681099904858,-3.84919571395828,7.2365585268307));
#37627=CARTESIAN_POINT('Ctrl Pts',(84.433536327521,-7.43128147235665,1.79245896459043));
#37628=CARTESIAN_POINT('Ctrl Pts',(84.5658773971491,-6.60355831010481,-2.90520398920369));
#37629=CARTESIAN_POINT('Ctrl Pts',(84.6651331993701,-4.42483609723173,-5.72433390776467));
#37630=CARTESIAN_POINT('Ctrl Pts',(84.7643890015913,-1.14772280657254,-7.12249429154648));
#37631=CARTESIAN_POINT('Ctrl Pts',(84.8967300712191,3.60693992809988,-6.73994345793868));
#37632=CARTESIAN_POINT('Ctrl Pts',(85.0621564082546,7.97291211063296,-1.90177796619987));
#37633=CARTESIAN_POINT('Ctrl Pts',(85.2606680126964,5.91318860450045,5.67581950219958));
#37634=CARTESIAN_POINT('Ctrl Pts',(85.4591796171386,-1.5591213078961,8.04673022048133));
#37635=CARTESIAN_POINT('Ctrl Pts',(85.6576912215807,-7.6108605802676,3.04284212280718));
#37636=CARTESIAN_POINT('Ctrl Pts',(85.8231175586158,-6.83297591294963,-3.42743251343945));
#37637=CARTESIAN_POINT('Ctrl Pts',(85.9554586282438,-3.16865385062834,-6.4812672641033));
#37638=CARTESIAN_POINT('Ctrl Pts',(86.054714430465,0.315066708290052,-7.22827131092052));
#37639=CARTESIAN_POINT('Ctrl Pts',(86.153970232686,3.72057726039948,-6.18097867843254));
#37640=CARTESIAN_POINT('Ctrl Pts',(86.286311302314,7.10528491496656,-2.81989002237311));
#37641=CARTESIAN_POINT('Ctrl Pts',(86.4517376393491,7.31723484533139,3.69352963638701));
#37642=CARTESIAN_POINT('Ctrl Pts',(86.6502492437914,0.853054781769095,8.1518724249858));
#37643=CARTESIAN_POINT('Ctrl Pts',(86.8487608482333,-6.38462023325127,5.13978121821364));
#37644=CARTESIAN_POINT('Ctrl Pts',(87.0472724526756,-7.77719827735906,-2.58829556102961));
#37645=CARTESIAN_POINT('Ctrl Pts',(87.2126987897105,-3.00681146855234,-7.02822440262923));
#37646=CARTESIAN_POINT('Ctrl Pts',(87.3450398593387,1.76310463197224,-6.99561681558938));
#37647=CARTESIAN_POINT('Ctrl Pts',(87.4442956615597,4.90613379615755,-5.31761453559306));
#37648=CARTESIAN_POINT('Ctrl Pts',(87.5435514637808,6.83129783049185,-2.31960395864394));
#37649=CARTESIAN_POINT('Ctrl Pts',(87.6758925334088,7.24713379598624,2.43226339120684));
#37650=CARTESIAN_POINT('Ctrl Pts',(87.8413188704439,3.20493753483079,7.54403488555254));
#37651=CARTESIAN_POINT('Ctrl Pts',(88.0398304748861,-4.61005725891556,6.77702726595246));
#37652=CARTESIAN_POINT('Ctrl Pts',(88.238342079328,-8.1940609418445,-0.195171143567751));
#37653=CARTESIAN_POINT('Ctrl Pts',(88.4368536837704,-4.26963182496724,-6.99673717069805));
#37654=CARTESIAN_POINT('Ctrl Pts',(88.6022800208052,2.23975357990136,-7.30892313288694));
#37655=CARTESIAN_POINT('Ctrl Pts',(88.7346210904336,5.86198253311296,-4.2052768464535));
#37656=CARTESIAN_POINT('Ctrl Pts',(88.8338768926543,7.1795712352997,-0.894946954968044));
#37657=CARTESIAN_POINT('Ctrl Pts',(88.9331326948758,6.71495223218478,2.63753845342878));
#37658=CARTESIAN_POINT('Ctrl Pts',(89.0654737645034,3.96547796806157,6.53542943852582));
#37659=CARTESIAN_POINT('Ctrl Pts',(89.2309001015389,-2.421354004456,7.8307810428913));
#37660=CARTESIAN_POINT('Ctrl Pts',(89.4294117059807,-7.89540451993751,2.2007530439587));
#37661=CARTESIAN_POINT('Ctrl Pts',(89.627923310423,-6.13267395365651,-5.43792576926969));
#37662=CARTESIAN_POINT('Ctrl Pts',(89.8264349148651,1.25488437193329,-8.09996001037527));
#37663=CARTESIAN_POINT('Ctrl Pts',(89.9918612519001,6.42827179997809,-4.13692822354185));
#37664=CARTESIAN_POINT('Ctrl Pts',(90.1242023215283,7.19169328889517,0.571611942054712));
#37665=CARTESIAN_POINT('Ctrl Pts',(90.2234581237492,6.06142013417448,3.95048846751564));
#37666=CARTESIAN_POINT('Ctrl Pts',(90.3227139259704,3.42650146314732,6.34872272956444));
#37667=CARTESIAN_POINT('Ctrl Pts',(90.4550549955983,-1.18944705552714,7.55129585986596));
#37668=CARTESIAN_POINT('Ctrl Pts',(90.6204813326335,-6.90381170961845,4.41831085763963));
#37669=CARTESIAN_POINT('Ctrl Pts',(90.8189929370757,-7.45100767605583,-3.4151443754694));
#37670=CARTESIAN_POINT('Ctrl Pts',(91.0175045415177,-1.17424673552373,-8.11183524845364));
#37671=CARTESIAN_POINT('Ctrl Pts',(91.2160161459598,6.18660034222907,-5.37680789708281));
#37672=CARTESIAN_POINT('Ctrl Pts',(91.381442482995,7.58011105191034,0.989328005182139));
#37673=CARTESIAN_POINT('Ctrl Pts',(91.513783552623,5.12408911536659,5.0784745063474));
#37674=CARTESIAN_POINT('Ctrl Pts',(91.6130393548441,2.07988870140306,6.92973564897867));
#37675=CARTESIAN_POINT('Ctrl Pts',(91.7122951570651,-1.48060907187722,7.06080656512513));
#37676=CARTESIAN_POINT('Ctrl Pts',(91.8446362266932,-5.78248406790028,4.99997314648891));
#37677=CARTESIAN_POINT('Ctrl Pts',(92.0100625637283,-8.12494810308719,-1.08134419993861));
#37678=CARTESIAN_POINT('Ctrl Pts',(92.2085741681704,-3.48679726401757,-7.41774705241314));
#37679=CARTESIAN_POINT('Ctrl Pts',(92.4070857726126,4.33888794927058,-6.95375997986828));
#37680=CARTESIAN_POINT('Ctrl Pts',(92.6055973770546,8.19580156390679,-0.113682371825931));
#37681=CARTESIAN_POINT('Ctrl Pts',(92.7710237140897,5.15114903660088,5.64823132173759));
#37682=CARTESIAN_POINT('Ctrl Pts',(92.9033647837178,0.635894442291002,7.18629465246884));
#37683=CARTESIAN_POINT('Ctrl Pts',(93.0026205859388,-2.88417030209986,6.63541519751662));
#37684=CARTESIAN_POINT('Ctrl Pts',(93.10187638816,-5.68828831828898,4.43740561385328));
#37685=CARTESIAN_POINT('Ctrl Pts',(93.2342174577878,-7.64390855687611,0.0866916100138159));
#37686=CARTESIAN_POINT('Ctrl Pts',(93.3996437948232,-5.50790531097854,-6.07017841928023));
#37687=CARTESIAN_POINT('Ctrl Pts',(93.5981553992651,2.12455630675614,-7.9162482902803));
#37688=CARTESIAN_POINT('Ctrl Pts',(93.7966670037073,7.80235669107675,-2.51076812134315));
#37689=CARTESIAN_POINT('Ctrl Pts',(93.9951786081494,6.33335282885967,5.20314605808604));
#37690=CARTESIAN_POINT('Ctrl Pts',(94.1606049451845,0.288813569149044,7.63894234717125));
#37691=CARTESIAN_POINT('Ctrl Pts',(94.2929460148125,-4.15269314181078,5.89935015436421));
#37692=CARTESIAN_POINT('Ctrl Pts',(94.3922018170336,-6.48576368973312,3.20656241727638));
#37693=CARTESIAN_POINT('Ctrl Pts',(94.4914576192548,-7.20885257666468,-0.282200463773047));
#37694=CARTESIAN_POINT('Ctrl Pts',(94.6237986888826,-5.89439420080124,-4.86754254903762));
#37695=CARTESIAN_POINT('Ctrl Pts',(94.789225025918,-0.28895943561254,-8.19149494299867));
#37696=CARTESIAN_POINT('Ctrl Pts',(94.9877366303599,6.73228158455901,-4.67515894490773));
#37697=CARTESIAN_POINT('Ctrl Pts',(95.1862482348021,7.58003659211948,3.11829629061651));
#37698=CARTESIAN_POINT('Ctrl Pts',(95.3847598392441,1.47906430674842,8.06203793920023));
#37699=CARTESIAN_POINT('Ctrl Pts',(95.5501861762794,-4.70995578262514,6.02106053671999));
#37700=CARTESIAN_POINT('Ctrl Pts',(95.6825272459072,-6.97957214897654,1.82558625955343));
#37701=CARTESIAN_POINT('Ctrl Pts',(95.7817830481286,-7.0235192681072,-1.73705217695852));
#37702=CARTESIAN_POINT('Ctrl Pts',(95.8810388503493,-5.32399595596597,-4.8684966503734));
#37703=CARTESIAN_POINT('Ctrl Pts',(96.0133799199777,-1.36040161224302,-7.52237734459912));
#37704=CARTESIAN_POINT('Ctrl Pts',(96.1788062570125,5.06648923056177,-6.44319593316877));
#37705=CARTESIAN_POINT('Ctrl Pts',(96.3773178614548,8.15971540431764,0.774448845621636));
#37706=CARTESIAN_POINT('Ctrl Pts',(96.5758294658966,3.7769504003016,7.27429530384934));
#37707=CARTESIAN_POINT('Ctrl Pts',(96.7743410703392,-4.0739257657314,7.11246903767678));
#37708=CARTESIAN_POINT('Ctrl Pts',(96.9397674073737,-7.48376886138719,1.55886403847908));
#37709=CARTESIAN_POINT('Ctrl Pts',(97.0721084770024,-6.50934104460086,-3.11057418154813));
#37710=CARTESIAN_POINT('Ctrl Pts',(97.1713642792229,-4.24340436628601,-5.8600932210277));
#37711=CARTESIAN_POINT('Ctrl Pts',(97.2706200814444,-0.924113983348465,
-7.1549427614495));
#37712=CARTESIAN_POINT('Ctrl Pts',(97.4029611510721,3.81623694597436,-6.62368394726916));
#37713=CARTESIAN_POINT('Ctrl Pts',(97.5683874881075,8.02855725455025,-1.65116787971719));
#37714=CARTESIAN_POINT('Ctrl Pts',(97.7668990925495,5.73254616351181,5.85821141451459));
#37715=CARTESIAN_POINT('Ctrl Pts',(97.9654106969915,-1.81034563845534,7.99395866659747));
#37716=CARTESIAN_POINT('Ctrl Pts',(98.1639223014339,-7.70241652089553,2.80301029167512));
#37717=CARTESIAN_POINT('Ctrl Pts',(98.3293486384687,-6.72229217472482,-3.63973094867799));
#37718=CARTESIAN_POINT('Ctrl Pts',(98.461689708097,-2.96413432287727,-6.57731710424392));
#37719=CARTESIAN_POINT('Ctrl Pts',(98.5609455103179,0.541270578014203,-7.21485962000136));
#37720=CARTESIAN_POINT('Ctrl Pts',(98.6602013125391,3.91231416913188,-6.06143468296485));
#37721=CARTESIAN_POINT('Ctrl Pts',(98.792542382167,7.19010691694292,-2.59599999692997));
#37722=CARTESIAN_POINT('Ctrl Pts',(98.9579687192023,7.19798058054701,3.9208624712771));
#37723=CARTESIAN_POINT('Ctrl Pts',(99.1564803236443,0.597354780781096,8.17458829298583));
#37724=CARTESIAN_POINT('Ctrl Pts',(99.3549919280863,-6.54244471348264,4.93732150715004));
#37725=CARTESIAN_POINT('Ctrl Pts',(99.5535035325286,-7.69232960220158,-2.83057454374467));
#37726=CARTESIAN_POINT('Ctrl Pts',(99.7189298695635,-2.78524297030128,-7.1189377759269));
#37727=CARTESIAN_POINT('Ctrl Pts',(99.8512709391918,1.98131256247304,-6.9369729063638));
#37728=CARTESIAN_POINT('Ctrl Pts',(99.9505267414127,5.07025238557831,-5.16136744685812));
#37729=CARTESIAN_POINT('Ctrl Pts',(100.049782543634,6.90058740162031,-2.10453940006798));
#37730=CARTESIAN_POINT('Ctrl Pts',(100.182123613262,7.16741135167138,2.65801955919494));
#37731=CARTESIAN_POINT('Ctrl Pts',(100.347549950297,2.96711889648337,7.64069973305668));
#37732=CARTESIAN_POINT('Ctrl Pts',(100.546061554739,-4.8200235964893,6.62933624303592));
#37733=CARTESIAN_POINT('Ctrl Pts',(100.744573159181,-8.18393018661653,-0.451678197979063));
#37734=CARTESIAN_POINT('Ctrl Pts',(100.943084763623,-4.04843001256235,-7.12701209413773));
#37735=CARTESIAN_POINT('Ctrl Pts',(101.108511100658,2.46753914216655,-7.23519896360887));
#37736=CARTESIAN_POINT('Ctrl Pts',(101.240852170286,5.9907986834069,-4.01964223640978));
#37737=CARTESIAN_POINT('Ctrl Pts',(101.340107972508,7.20407585797007,-0.669674702794391));
#37738=CARTESIAN_POINT('Ctrl Pts',(101.439363774729,6.6290624671403,2.84652830314237));
#37739=CARTESIAN_POINT('Ctrl Pts',(101.571704844357,3.75887150586802,6.65640582172574));
#37740=CARTESIAN_POINT('Ctrl Pts',(101.737131181392,-2.66539284677105,7.75111397987301));
#37741=CARTESIAN_POINT('Ctrl Pts',(101.935642785834,-7.96045029267649,1.95242352776489));
#37742=CARTESIAN_POINT('Ctrl Pts',(102.134154390276,-5.95937367401093,-5.62730769617671));
#37743=CARTESIAN_POINT('Ctrl Pts',(102.332665994718,1.50792484587792,-8.05668974305115));
#37744=CARTESIAN_POINT('Ctrl Pts',(102.498092331753,6.55466982463192,-3.93359338915324));
#37745=CARTESIAN_POINT('Ctrl Pts',(102.630433401381,7.17026564361548,0.796544520931952));
#37746=CARTESIAN_POINT('Ctrl Pts',(102.729689203602,5.93473494597949,4.13836855486806));
#37747=CARTESIAN_POINT('Ctrl Pts',(102.828945005823,3.22600619751222,6.45291225629539));
#37748=CARTESIAN_POINT('Ctrl Pts',(102.961286075451,-1.42533782016256,7.51034390421344));
#37749=CARTESIAN_POINT('Ctrl Pts',(103.126712412487,-7.03878819739605,4.19994615070119));
#37750=CARTESIAN_POINT('Ctrl Pts',(103.325224016929,-7.34040563156762,-3.64680293654208));
#37751=CARTESIAN_POINT('Ctrl Pts',(103.523735621371,-0.919642996050166,
-8.14462910474322));
#37752=CARTESIAN_POINT('Ctrl Pts',(103.722247225813,6.35194459972139,-5.18043306670365));
#37753=CARTESIAN_POINT('Ctrl Pts',(103.887673562848,7.54541183235724,1.22621928756231));
#37754=CARTESIAN_POINT('Ctrl Pts',(104.020014632476,4.96253997204499,5.23644818554906));
#37755=CARTESIAN_POINT('Ctrl Pts',(104.119270434697,1.86185906335093,6.9914700887944));
#37756=CARTESIAN_POINT('Ctrl Pts',(104.218526236918,-1.70099701708682,7.0109772302331));
#37757=CARTESIAN_POINT('Ctrl Pts',(104.350867306546,-5.93622568196176,4.81643832229469));
#37758=CARTESIAN_POINT('Ctrl Pts',(104.516293643581,-8.08710011258896,-1.33525230717154));
#37759=CARTESIAN_POINT('Ctrl Pts',(104.714805248023,-3.25279517795495,-7.52330047479355));
#37760=CARTESIAN_POINT('Ctrl Pts',(104.913316852466,4.5545217929969,-6.81447413355386));
#37761=CARTESIAN_POINT('Ctrl Pts',(105.111828456908,8.19534191959957,0.143030668481208));
#37762=CARTESIAN_POINT('Ctrl Pts',(105.277254793943,4.97174428693698,5.80677296415496));
#37763=CARTESIAN_POINT('Ctrl Pts',(105.409595863571,0.410538694972291,7.20268356057518));
#37764=CARTESIAN_POINT('Ctrl Pts',(105.508851665792,-3.09054842984606,6.54184100431835));
#37765=CARTESIAN_POINT('Ctrl Pts',(105.608107468013,-5.82445893643908,4.25709648884606));
#37766=CARTESIAN_POINT('Ctrl Pts',(105.740448537641,-7.64287435179083,-0.152725229310253));
#37767=CARTESIAN_POINT('Ctrl Pts',(105.905874874676,-5.31511202979502,-6.23968528226296));
#37768=CARTESIAN_POINT('Ctrl Pts',(106.104386479118,2.37141720322459,-7.84583357489262));
#37769=CARTESIAN_POINT('Ctrl Pts',(106.30289808356,7.8771564015956,-2.26520071409541));
#37770=CARTESIAN_POINT('Ctrl Pts',(106.501409688003,6.16730649189762,5.39892812568543));
#37771=CARTESIAN_POINT('Ctrl Pts',(106.666836025037,0.0494529375975138,
7.64423913575313));
#37772=CARTESIAN_POINT('Ctrl Pts',(106.799177094666,-4.33539853602892,5.76641372581939));
#37773=CARTESIAN_POINT('Ctrl Pts',(106.898432896887,-6.58299886234465,3.00188031505507));
#37774=CARTESIAN_POINT('Ctrl Pts',(106.997688699108,-7.19647889300465,-0.507806484833575));
#37775=CARTESIAN_POINT('Ctrl Pts',(107.130029768736,-5.73907435111488,-5.04975498101209));
#37776=CARTESIAN_POINT('Ctrl Pts',(107.295456105771,-0.0322920042968116,
-8.19650053508292));
#37777=CARTESIAN_POINT('Ctrl Pts',(107.493967710213,6.87538010918837,-4.46208277408401));
#37778=CARTESIAN_POINT('Ctrl Pts',(107.692479314655,7.47867733972214,3.35422008809143));
#37779=CARTESIAN_POINT('Ctrl Pts',(107.890990919097,1.22585064624322,8.10424595418784));
#37780=CARTESIAN_POINT('Ctrl Pts',(108.056417256132,-4.89616459018992,5.8708858044287));
#37781=CARTESIAN_POINT('Ctrl Pts',(108.18875832576,-7.03336727340939,1.60573780850504));
#37782=CARTESIAN_POINT('Ctrl Pts',(108.288014127981,-6.96557098724266,-1.95531034861243));
#37783=CARTESIAN_POINT('Ctrl Pts',(108.387269930203,-5.16912081155891,-5.03437754836346));
#37784=CARTESIAN_POINT('Ctrl Pts',(108.51961099983,-1.12374364642211,-7.55794914914912));
#37785=CARTESIAN_POINT('Ctrl Pts',(108.685037336866,5.26494275239868,-6.28824056464582));
#37786=CARTESIAN_POINT('Ctrl Pts',(108.883548941308,8.13270769338756,1.04131295379453));
#37787=CARTESIAN_POINT('Ctrl Pts',(109.048975278343,4.31059234212791,6.31114658088431));
#37788=CARTESIAN_POINT('Ctrl Pts',(109.181316347971,-0.379872332578537,
7.2055380683537));
#37789=CARTESIAN_POINT('Ctrl Pts',(109.280572150192,-3.77681976785492,6.16629695720056));
#37790=CARTESIAN_POINT('Ctrl Pts',(109.379827952413,-6.26964300376297,3.59558754355007));
#37791=CARTESIAN_POINT('Ctrl Pts',(109.445998487227,-6.90538169251611,1.30827352835722));
#37792=CARTESIAN_POINT('Ctrl Pts',(109.479083754634,-6.93125428135741,0.155573414067464));
#37793=CARTESIAN_POINT('Ctrl Pts',(108.233548336394,-6.93028901950621,-0.00380765172104063));
#37794=CARTESIAN_POINT('Ctrl Pts',(108.251703600256,-6.93170393511236,-0.636222120076916));
#37795=CARTESIAN_POINT('Ctrl Pts',(108.269858864119,-6.84796028214185,-1.26769555840962));
#37796=CARTESIAN_POINT('Ctrl Pts',(108.288014127981,-6.67746200565648,-1.87498018905138));
#37797=CARTESIAN_POINT('Ctrl Pts',(108.321099395389,-6.36675426201473,-2.98166608186278));
#37798=CARTESIAN_POINT('Ctrl Pts',(108.354184662796,-5.76793753678676,-4.00802181511322));
#37799=CARTESIAN_POINT('Ctrl Pts',(108.387269930203,-4.96285702853069,-4.83664613183659));
#37800=CARTESIAN_POINT('Ctrl Pts',(108.420355197609,-4.15777652027462,-5.66527044855996));
#37801=CARTESIAN_POINT('Ctrl Pts',(108.453440465016,-3.14643222899067,-6.29616334875622));
#37802=CARTESIAN_POINT('Ctrl Pts',(108.486525732423,-2.04629027487981,-6.63211137658697));
#37803=CARTESIAN_POINT('Ctrl Pts',(108.552696267238,0.153993633341921,-7.30400743224846));
#37804=CARTESIAN_POINT('Ctrl Pts',(108.618866802052,2.70946819287044,-6.79612399844709));
#37805=CARTESIAN_POINT('Ctrl Pts',(108.685037336866,4.46516629613274,-5.32059002847302));
#37806=CARTESIAN_POINT('Ctrl Pts',(108.75120787168,6.22086439939495,-3.84505605849902));
#37807=CARTESIAN_POINT('Ctrl Pts',(108.817378406494,7.17678604639124,-1.40187155235226));
#37808=CARTESIAN_POINT('Ctrl Pts',(108.883548941308,6.89032379963751,0.873687426138972));
#37809=CARTESIAN_POINT('Ctrl Pts',(108.944699294205,6.6255946791913,2.97660581669859));
#37810=CARTESIAN_POINT('Ctrl Pts',(109.005849647103,5.29984338919197,4.93636845490143));
#37811=CARTESIAN_POINT('Ctrl Pts',(109.067,3.46405146923455,6.01146880811242));
#37812=CARTESIAN_POINT('',(31.067,5.11685509991379,3.5431531688378));
#37813=CARTESIAN_POINT('Ctrl Pts',(31.067,5.11685509991369,3.54315316883794));
#37814=CARTESIAN_POINT('Ctrl Pts',(31.067,5.2144007801441,3.41955272739614));
#37815=CARTESIAN_POINT('Ctrl Pts',(31.067,5.30690073322865,3.29228367909392));
#37816=CARTESIAN_POINT('Ctrl Pts',(31.067,5.39405337529976,3.16152164966802));
#37817=CARTESIAN_POINT('Ctrl Pts',(31.067,5.48890910442734,3.01920206705255));
#37818=CARTESIAN_POINT('Ctrl Pts',(31.067,5.57743177629917,2.87274515576473));
#37819=CARTESIAN_POINT('Ctrl Pts',(31.067,5.65961398733303,2.72265475190711));
#37820=CARTESIAN_POINT('Ctrl Pts',(31.067,5.71255046712117,2.62597619422109));
#37821=CARTESIAN_POINT('Ctrl Pts',(31.067,5.76285543012115,2.52778927668005));
#37822=CARTESIAN_POINT('Ctrl Pts',(31.067,5.81051785955815,2.42822180627828));
#37823=CARTESIAN_POINT('Ctrl Pts',(31.067,5.83809201900622,2.37061900807582));
#37824=CARTESIAN_POINT('Ctrl Pts',(31.067,5.86478159584491,2.31255405227071));
#37825=CARTESIAN_POINT('Ctrl Pts',(31.067,5.89058332834668,2.25405104435855));
#37826=CARTESIAN_POINT('Ctrl Pts',(31.067,5.9043177737656,2.22290947783945));
#37827=CARTESIAN_POINT('Ctrl Pts',(31.067,5.91780063355126,2.19164378162859));
#37828=CARTESIAN_POINT('Ctrl Pts',(31.067,5.93103131770442,2.160257546248));
#37829=CARTESIAN_POINT('Ctrl Pts',(31.067,5.94079597664893,2.13709352233995));
#37830=CARTESIAN_POINT('Ctrl Pts',(31.067,5.9504217117342,2.11386746706017));
#37831=CARTESIAN_POINT('Ctrl Pts',(31.067,5.95990532759805,2.0905886622763));
#37832=CARTESIAN_POINT('Ctrl Pts',(31.067,6.0261120429078,1.92807541593616));
#37833=CARTESIAN_POINT('Ctrl Pts',(31.067,6.08544315296794,1.76288224841305));
#37834=CARTESIAN_POINT('Ctrl Pts',(31.067,6.13789139515789,1.5955367961925));
#37835=CARTESIAN_POINT('Ctrl Pts',(31.067,6.19084866070303,1.42656721435372));
#37836=CARTESIAN_POINT('Ctrl Pts',(31.067,6.23678906352892,1.25540265586484));
#37837=CARTESIAN_POINT('Ctrl Pts',(31.067,6.27565901721259,1.08255884663743));
#37838=CARTESIAN_POINT('Ctrl Pts',(31.067,6.30838202285779,0.937048795580633));
#37839=CARTESIAN_POINT('Ctrl Pts',(31.067,6.33609328241928,0.790347903538514));
#37840=CARTESIAN_POINT('Ctrl Pts',(31.067,6.35873389224681,0.642754751803561));
#37841=CARTESIAN_POINT('Ctrl Pts',(31.067,6.36263630840976,0.61731507039662));
#37842=CARTESIAN_POINT('Ctrl Pts',(31.067,6.36638801856405,0.591848868190301));
#37843=CARTESIAN_POINT('Ctrl Pts',(31.067,6.36998864411347,0.566357661020381));
#37844=CARTESIAN_POINT('Ctrl Pts',(31.067,6.37338728944288,0.542296405274669));
#37845=CARTESIAN_POINT('Ctrl Pts',(31.067,6.37665015407961,0.518221047747062));
#37846=CARTESIAN_POINT('Ctrl Pts',(31.067,6.3797766793027,0.494137097499145));
#37847=CARTESIAN_POINT('Ctrl Pts',(31.067,6.39255495331688,0.395704718531514));
#37848=CARTESIAN_POINT('Ctrl Pts',(31.067,6.40305930999864,0.297106734753472));
#37849=CARTESIAN_POINT('Ctrl Pts',(31.067,6.41128905366097,0.198434233054838));
#37850=CARTESIAN_POINT('Ctrl Pts',(31.067,6.4260970453098,0.020890236415967));
#37851=CARTESIAN_POINT('Ctrl Pts',(31.067,6.433543840758,-0.15689427514383));
#37852=CARTESIAN_POINT('Ctrl Pts',(31.067,6.43375826100571,-0.334500592678881));
#37853=CARTESIAN_POINT('Ctrl Pts',(31.067,6.43397455628222,-0.513660014283607));
#37854=CARTESIAN_POINT('Ctrl Pts',(31.067,6.42683148569265,-0.692638769818387));
#37855=CARTESIAN_POINT('Ctrl Pts',(31.067,6.41240941578984,-0.871018380375883));
#37856=CARTESIAN_POINT('Ctrl Pts',(31.067,6.39782718168609,-1.0513789845066));
#37857=CARTESIAN_POINT('Ctrl Pts',(31.067,6.3758034632196,-1.23112777607217));
#37858=CARTESIAN_POINT('Ctrl Pts',(31.067,6.3463674681003,-1.40983329057961));
#37859=CARTESIAN_POINT('Ctrl Pts',(31.067,6.32429047176082,-1.54386242646019));
#37860=CARTESIAN_POINT('Ctrl Pts',(31.067,6.29804296076356,-1.67730481305471));
#37861=CARTESIAN_POINT('Ctrl Pts',(31.067,6.26761729626672,-1.80997509468729));
#37862=CARTESIAN_POINT('Ctrl Pts',(31.067,6.25927860899389,-1.8463357135013));
#37863=CARTESIAN_POINT('Ctrl Pts',(31.067,6.2506259889135,-1.88263831055097));
#37864=CARTESIAN_POINT('Ctrl Pts',(31.067,6.24165905425322,-1.91887900190174));
#37865=CARTESIAN_POINT('Ctrl Pts',(31.067,6.23650670208748,-1.93970270717483));
#37866=CARTESIAN_POINT('Ctrl Pts',(31.067,6.23125127551909,-1.96050299780219));
#37867=CARTESIAN_POINT('Ctrl Pts',(31.067,6.22589545585126,-1.98126916880994));
#37868=CARTESIAN_POINT('Ctrl Pts',(31.067,6.18033062290449,-2.1579381329641));
#37869=CARTESIAN_POINT('Ctrl Pts',(31.067,6.12745232170895,-2.33234672874841));
#37870=CARTESIAN_POINT('Ctrl Pts',(31.067,6.0673660129305,-2.50406902324849));
#37871=CARTESIAN_POINT('Ctrl Pts',(31.067,6.01225975549519,-2.66155869369896));
#37872=CARTESIAN_POINT('Ctrl Pts',(31.067,5.95109019025875,-2.81678940633195));
#37873=CARTESIAN_POINT('Ctrl Pts',(31.067,5.88390014609054,-2.96943153794234));
#37874=CARTESIAN_POINT('Ctrl Pts',(31.067,5.8114028299027,-3.1341307134815));
#37875=CARTESIAN_POINT('Ctrl Pts',(31.067,5.73189706641349,-3.29581698197365));
#37876=CARTESIAN_POINT('Ctrl Pts',(31.067,5.64574085447704,-3.45414022141883));
#37877=CARTESIAN_POINT('Ctrl Pts',(31.067,5.55896582325022,-3.61360062175447));
#37878=CARTESIAN_POINT('Ctrl Pts',(31.067,5.46544409047891,-3.7696501491991));
#37879=CARTESIAN_POINT('Ctrl Pts',(31.067,5.36549302718914,-3.92190981252245));
#37880=CARTESIAN_POINT('Ctrl Pts',(31.067,5.31398434674346,-4.00037515430829));
#37881=CARTESIAN_POINT('Ctrl Pts',(31.067,5.2607674524701,-4.07783360169406));
#37882=CARTESIAN_POINT('Ctrl Pts',(31.067,5.20588132288495,-4.15423023945157));
#37883=CARTESIAN_POINT('Ctrl Pts',(31.067,5.18904408415586,-4.177666186525));
#37884=CARTESIAN_POINT('Ctrl Pts',(31.067,5.17204974051512,-4.20100219435326));
#37885=CARTESIAN_POINT('Ctrl Pts',(31.067,5.15489936485222,-4.22423663144381));
#37886=CARTESIAN_POINT('Ctrl Pts',(31.067,5.14306101915661,-4.24027460657202));
#37887=CARTESIAN_POINT('Ctrl Pts',(31.067,5.13114984623005,-4.25626208650461));
#37888=CARTESIAN_POINT('Ctrl Pts',(31.067,5.11917153389746,-4.27219166789797));
#37889=CARTESIAN_POINT('Ctrl Pts',(31.067,5.00871211991934,-4.41908817358017));
#37890=CARTESIAN_POINT('Ctrl Pts',(31.067,4.89242109857996,-4.56123408705379));
#37891=CARTESIAN_POINT('Ctrl Pts',(31.067,4.77069968034181,-4.69828929887201));
#37892=CARTESIAN_POINT('Ctrl Pts',(31.067,4.64794056813919,-4.83651292762261));
#37893=CARTESIAN_POINT('Ctrl Pts',(31.067,4.51965767575762,-4.96955932709291));
#37894=CARTESIAN_POINT('Ctrl Pts',(31.067,4.3862135670772,-5.09705898614707));
#37895=CARTESIAN_POINT('Ctrl Pts',(31.067,4.25283777375098,-5.22449337304755));
#37896=CARTESIAN_POINT('Ctrl Pts',(31.067,4.11430557895959,-5.34638732154593));
#37897=CARTESIAN_POINT('Ctrl Pts',(31.067,3.97093688259113,-5.46234190382446));
#37898=CARTESIAN_POINT('Ctrl Pts',(31.067,3.92787994422503,-5.49716574911913));
#37899=CARTESIAN_POINT('Ctrl Pts',(31.067,3.88438652067304,-5.53145365890501));
#37900=CARTESIAN_POINT('Ctrl Pts',(31.067,3.84046463239738,-5.56519416757222));
#37901=CARTESIAN_POINT('Ctrl Pts',(31.067,3.72753604226176,-5.65194517541443));
#37902=CARTESIAN_POINT('Ctrl Pts',(31.067,3.61177574729217,-5.73507858328812));
#37903=CARTESIAN_POINT('Ctrl Pts',(31.067,3.49336789459867,-5.81452363421184));
#37904=CARTESIAN_POINT('Ctrl Pts',(31.067,3.44156445904527,-5.84928084399096));
#37905=CARTESIAN_POINT('Ctrl Pts',(31.067,3.38925412896203,-5.88333188073878));
#37906=CARTESIAN_POINT('Ctrl Pts',(31.067,3.33645174789616,-5.91666986399315));
#37907=CARTESIAN_POINT('Ctrl Pts',(31.067,3.30762568726353,-5.93486985246452));
#37908=CARTESIAN_POINT('Ctrl Pts',(31.067,3.27865297384291,-5.95285731744087));
#37909=CARTESIAN_POINT('Ctrl Pts',(31.067,3.24953598484261,-5.97063106297212));
#37910=CARTESIAN_POINT('Ctrl Pts',(31.067,3.22673123260147,-5.98455165974926));
#37911=CARTESIAN_POINT('Ctrl Pts',(31.067,3.20383615363947,-5.99834216605967));
#37912=CARTESIAN_POINT('Ctrl Pts',(31.067,3.18087127062506,-6.01199068150968));
#37913=CARTESIAN_POINT('Ctrl Pts',(31.067,3.02218322859531,-6.10630233953186));
#37914=CARTESIAN_POINT('Ctrl Pts',(31.067,2.85996735085955,-6.19395958629189));
#37915=CARTESIAN_POINT('Ctrl Pts',(31.067,2.69468188090138,-6.27489113780825));
#37916=CARTESIAN_POINT('Ctrl Pts',(31.067,2.52658802341311,-6.35719780814254));
#37917=CARTESIAN_POINT('Ctrl Pts',(31.067,2.35531886065546,-6.4325486765892));
#37918=CARTESIAN_POINT('Ctrl Pts',(31.067,2.18131982375181,-6.50082927234875));
#37919=CARTESIAN_POINT('Ctrl Pts',(31.067,2.0069903506746,-6.56923953766966));
#37920=CARTESIAN_POINT('Ctrl Pts',(31.067,1.82992000150959,-6.63055296436482));
#37921=CARTESIAN_POINT('Ctrl Pts',(31.067,1.65052909766165,-6.68460995303681));
#37922=CARTESIAN_POINT('Ctrl Pts',(31.067,1.472830493977,-6.73815699026314));
#37923=CARTESIAN_POINT('Ctrl Pts',(31.067,1.29285426780137,-6.78458408156556));
#37924=CARTESIAN_POINT('Ctrl Pts',(31.067,1.11099136235469,-6.82368859152074));
#37925=CARTESIAN_POINT('Ctrl Pts',(31.067,0.984463770055063,-6.85089479654938));
#37926=CARTESIAN_POINT('Ctrl Pts',(31.067,0.857022575344876,-6.87455559284932));
#37927=CARTESIAN_POINT('Ctrl Pts',(31.067,0.728796816010263,-6.89458803707468));
#37928=CARTESIAN_POINT('Ctrl Pts',(31.067,5.1168550999138,3.5431531688378));
#37929=CARTESIAN_POINT('Ctrl Pts',(31.1281503528974,4.01942676905249,5.1044661434557));
#37930=CARTESIAN_POINT('Ctrl Pts',(31.2554712406089,0.166680189710837,7.26913646933564));
#37931=CARTESIAN_POINT('Ctrl Pts',(31.4236261011954,-5.20334138794374,4.63644610479065));
#37932=CARTESIAN_POINT('Ctrl Pts',(31.5306306088845,-6.20309813924992,1.27936691419838));
#37933=CARTESIAN_POINT('Ctrl Pts',(31.5714645817597,-6.20816386984268,-0.000295703980951051));
#37934=CARTESIAN_POINT('Origin',(31.067,-1.12618006296016E-15,0.));
#37935=CARTESIAN_POINT('',(31.067,-1.68325362372072,5.98713018070687));
#37936=CARTESIAN_POINT('Ctrl Pts',(31.067,-4.95966987665984,-4.85170944379069));
#37937=CARTESIAN_POINT('Ctrl Pts',(31.067,-5.07635566737652,-4.72174660294797));
#37938=CARTESIAN_POINT('Ctrl Pts',(31.067,-5.18774208410829,-4.5873676703608));
#37939=CARTESIAN_POINT('Ctrl Pts',(31.067,-5.2934659950304,-4.44869245219079));
#37940=CARTESIAN_POINT('Ctrl Pts',(31.067,-5.40677951528188,-4.30006214703625));
#37941=CARTESIAN_POINT('Ctrl Pts',(31.067,-5.51358913810325,-4.14649635317199));
#37942=CARTESIAN_POINT('Ctrl Pts',(31.067,-5.61378552910678,-3.98851757493328));
#37943=CARTESIAN_POINT('Ctrl Pts',(31.067,-5.67722095415703,-3.88849949198516));
#37944=CARTESIAN_POINT('Ctrl Pts',(31.067,-5.73800468699189,-3.78671197565764));
#37945=CARTESIAN_POINT('Ctrl Pts',(31.067,-5.79609912672184,-3.68328336482282));
#37946=CARTESIAN_POINT('Ctrl Pts',(31.067,-5.8261073502107,-3.62985813370775));
#37947=CARTESIAN_POINT('Ctrl Pts',(31.067,-5.85539790107394,-3.57599498956757));
#37948=CARTESIAN_POINT('Ctrl Pts',(31.067,-5.88396477006812,-3.52171140149403));
#37949=CARTESIAN_POINT('Ctrl Pts',(31.067,-5.90334141911564,-3.48489133432616));
#37950=CARTESIAN_POINT('Ctrl Pts',(31.067,-5.9223851058769,-3.44787782708014));
#37951=CARTESIAN_POINT('Ctrl Pts',(31.067,-5.94109380441469,-3.41067630557261));
#37952=CARTESIAN_POINT('Ctrl Pts',(31.067,-5.95476449124947,-3.38349267495931));
#37953=CARTESIAN_POINT('Ctrl Pts',(31.067,-5.9682569544298,-3.35620718712805));
#37954=CARTESIAN_POINT('Ctrl Pts',(31.067,-5.98156221116727,-3.32883915699247));
#37955=CARTESIAN_POINT('Ctrl Pts',(31.067,-6.0632846669316,-3.16074148881201));
#37956=CARTESIAN_POINT('Ctrl Pts',(31.067,-6.13802128983771,-2.98938944330838));
#37957=CARTESIAN_POINT('Ctrl Pts',(31.067,-6.20566688241296,-2.81530388884709));
#37958=CARTESIAN_POINT('Ctrl Pts',(31.067,-6.27332997004571,-2.64117331095313));
#37959=CARTESIAN_POINT('Ctrl Pts',(31.067,-6.33389852210686,-2.46430702539236));
#37960=CARTESIAN_POINT('Ctrl Pts',(31.067,-6.3872172336922,-2.28521174662972));
#37961=CARTESIAN_POINT('Ctrl Pts',(31.067,-6.43351747954507,-2.12969119500265));
#37962=CARTESIAN_POINT('Ctrl Pts',(31.067,-6.47435018799297,-1.97248931528049));
#37963=CARTESIAN_POINT('Ctrl Pts',(31.067,-6.50958159881369,-1.81393587356536));
#37964=CARTESIAN_POINT('Ctrl Pts',(31.067,-6.5162987831482,-1.78370623841702));
#37965=CARTESIAN_POINT('Ctrl Pts',(31.067,-6.52281226624634,-1.75342747784606));
#37966=CARTESIAN_POINT('Ctrl Pts',(31.067,-6.5291209938122,-1.72310188852852));
#37967=CARTESIAN_POINT('Ctrl Pts',(31.067,-6.53378997379954,-1.70065844519546));
#37968=CARTESIAN_POINT('Ctrl Pts',(31.067,-6.53834599767253,-1.67819309129953));
#37969=CARTESIAN_POINT('Ctrl Pts',(31.067,-6.54278721332838,-1.65571492114972));
#37970=CARTESIAN_POINT('Ctrl Pts',(31.067,-6.56381992769274,-1.54926277632505));
#37971=CARTESIAN_POINT('Ctrl Pts',(31.067,-6.58228961498628,-1.44246888520439));
#37972=CARTESIAN_POINT('Ctrl Pts',(31.067,-6.59817669086173,-1.33543377907857));
#37973=CARTESIAN_POINT('Ctrl Pts',(31.067,-6.62523147934088,-1.15315906856664));
#37974=CARTESIAN_POINT('Ctrl Pts',(31.067,-6.64479957064315,-0.970184910999771));
#37975=CARTESIAN_POINT('Ctrl Pts',(31.067,-6.6569284968028,-0.786934728926997));
#37976=CARTESIAN_POINT('Ctrl Pts',(31.067,-6.66907982591669,-0.603346071263836));
#37977=CARTESIAN_POINT('Ctrl Pts',(31.067,-6.67376443191619,-0.419479680282065));
#37978=CARTESIAN_POINT('Ctrl Pts',(31.067,-6.67097793043684,-0.235762076334595));
#37979=CARTESIAN_POINT('Ctrl Pts',(31.067,-6.66818244407636,-0.0514520876912934));
#37980=CARTESIAN_POINT('Ctrl Pts',(31.067,-6.65786756519682,0.132708849422281));
#37981=CARTESIAN_POINT('Ctrl Pts',(31.067,-6.63997697058196,0.316278910548742));
#37982=CARTESIAN_POINT('Ctrl Pts',(31.067,-6.62655902462081,0.453956456393588));
#37983=CARTESIAN_POINT('Ctrl Pts',(31.067,-6.60887867008592,0.591301469579883));
#37984=CARTESIAN_POINT('Ctrl Pts',(31.067,-6.58689321254617,0.728119878393478));
#37985=CARTESIAN_POINT('Ctrl Pts',(31.067,-6.57965626197951,0.773156378516489));
#37986=CARTESIAN_POINT('Ctrl Pts',(31.067,-6.5719527115053,0.818135753944776));
#37987=CARTESIAN_POINT('Ctrl Pts',(31.067,-6.5637806567902,0.863050874087544));
#37988=CARTESIAN_POINT('Ctrl Pts',(31.067,-6.55946815526574,0.886753177956007));
#37989=CARTESIAN_POINT('Ctrl Pts',(31.067,-6.55502649277326,0.910430215125999));
#37990=CARTESIAN_POINT('Ctrl Pts',(31.067,-6.55045718629041,0.934073267148448));
#37991=CARTESIAN_POINT('Ctrl Pts',(31.067,-6.51616820861596,1.11149539586711));
#37992=CARTESIAN_POINT('Ctrl Pts',(31.067,-6.47467065207115,1.28714095330058));
#37993=CARTESIAN_POINT('Ctrl Pts',(31.067,-6.42598064130125,1.46061043020915));
#37994=CARTESIAN_POINT('Ctrl Pts',(31.067,-6.38139733331752,1.61944882421442));
#37995=CARTESIAN_POINT('Ctrl Pts',(31.067,-6.33078305800691,1.77646305987751));
#37996=CARTESIAN_POINT('Ctrl Pts',(31.067,-6.27411319884471,1.93133634328533));
#37997=CARTESIAN_POINT('Ctrl Pts',(31.067,-6.21205804932745,2.1009271081149));
#37998=CARTESIAN_POINT('Ctrl Pts',(31.067,-6.14274198333447,2.26795156050715));
#37999=CARTESIAN_POINT('Ctrl Pts',(31.067,-6.06645428682219,2.43198635086053));
#38000=CARTESIAN_POINT('Ctrl Pts',(31.067,-5.99042918402894,2.59545650880764));
#38001=CARTESIAN_POINT('Ctrl Pts',(31.067,-5.90747986319118,2.75595816053323));
#38002=CARTESIAN_POINT('Ctrl Pts',(31.067,-5.81785241493192,2.91304016625822));
#38003=CARTESIAN_POINT('Ctrl Pts',(31.067,-5.77330574632114,2.99111312481782));
#38004=CARTESIAN_POINT('Ctrl Pts',(31.067,-5.72710880713813,3.0683407746618));
#38005=CARTESIAN_POINT('Ctrl Pts',(31.067,-5.67928867316067,3.14466404153542));
#38006=CARTESIAN_POINT('Ctrl Pts',(31.067,-5.66592045077483,3.16600037667119));
#38007=CARTESIAN_POINT('Ctrl Pts',(31.067,-5.6524253652407,3.18726601863544));
#38008=CARTESIAN_POINT('Ctrl Pts',(31.067,-5.63880398215889,3.20845963827975));
#38009=CARTESIAN_POINT('Ctrl Pts',(31.067,-5.62723633649404,3.22645783133611));
#38010=CARTESIAN_POINT('Ctrl Pts',(31.067,-5.61557834605993,3.24440285810145));
#38011=CARTESIAN_POINT('Ctrl Pts',(31.067,-5.6038372074752,3.2622837478132));
#38012=CARTESIAN_POINT('Ctrl Pts',(31.067,-5.50559617042605,3.41189761498358));
#38013=CARTESIAN_POINT('Ctrl Pts',(31.067,-5.40141185916998,3.55721997451032));
#38014=CARTESIAN_POINT('Ctrl Pts',(31.067,-5.29159672322233,3.69786677176514));
#38015=CARTESIAN_POINT('Ctrl Pts',(31.067,-5.18185629256696,3.83841788949447));
#38016=CARTESIAN_POINT('Ctrl Pts',(31.067,-5.06649219437619,3.97430040459667));
#38017=CARTESIAN_POINT('Ctrl Pts',(31.067,-4.9457752208923,4.10509926031028));
#38018=CARTESIAN_POINT('Ctrl Pts',(31.067,-4.82662308589716,4.23420258740186));
#38019=CARTESIAN_POINT('Ctrl Pts',(31.067,-4.70225542548044,4.35835368787749));
#38020=CARTESIAN_POINT('Ctrl Pts',(31.067,-4.57290041499668,4.47711448579565));
#38021=CARTESIAN_POINT('Ctrl Pts',(31.067,-4.5364413095177,4.51058758004899));
#38022=CARTESIAN_POINT('Ctrl Pts',(31.067,-4.49958583096963,4.54363219780854));
#38023=CARTESIAN_POINT('Ctrl Pts',(31.067,-4.46233870438039,4.5762378790869));
#38024=CARTESIAN_POINT('Ctrl Pts',(31.067,-4.36358707308753,4.6626838552064));
#38025=CARTESIAN_POINT('Ctrl Pts',(31.067,-4.26208285674386,4.7460454941142));
#38026=CARTESIAN_POINT('Ctrl Pts',(31.067,-4.15797763636354,4.82622587042557));
#38027=CARTESIAN_POINT('Ctrl Pts',(31.067,-4.11243160244716,4.86130478506179));
#38028=CARTESIAN_POINT('Ctrl Pts',(31.067,-4.06638765091281,4.89577460051552));
#38029=CARTESIAN_POINT('Ctrl Pts',(31.067,-4.01985820004502,4.92962631219268));
#38030=CARTESIAN_POINT('Ctrl Pts',(31.067,-3.99192547401397,4.94994829257984));
#38031=CARTESIAN_POINT('Ctrl Pts',(31.067,-3.96381777685901,4.97004750497133));
#38032=CARTESIAN_POINT('Ctrl Pts',(31.067,-3.93553777385799,4.9899219041749));
#38033=CARTESIAN_POINT('Ctrl Pts',(31.067,-3.91343652477951,5.0054540470487));
#38034=CARTESIAN_POINT('Ctrl Pts',(31.067,-3.89122738800398,5.02085061138));
#38035=CARTESIAN_POINT('Ctrl Pts',(31.067,-3.86893240489384,5.03609662377786));
#38036=CARTESIAN_POINT('Ctrl Pts',(31.067,-3.72457833794962,5.13481048614953));
#38037=CARTESIAN_POINT('Ctrl Pts',(31.067,-3.5764575554336,5.22733828199603));
#38038=CARTESIAN_POINT('Ctrl Pts',(31.067,-3.4249789067786,5.31353849959259));
#38039=CARTESIAN_POINT('Ctrl Pts',(31.067,-3.27256982914678,5.40026818573783));
#38040=CARTESIAN_POINT('Ctrl Pts',(31.067,-3.11676086341988,5.48059262935479));
#38041=CARTESIAN_POINT('Ctrl Pts',(31.067,-2.95794275057018,5.55432203962601));
#38042=CARTESIAN_POINT('Ctrl Pts',(31.067,-2.79994827293749,5.62766908709402));
#38043=CARTESIAN_POINT('Ctrl Pts',(31.067,-2.63897511619471,5.69448954961524));
#38044=CARTESIAN_POINT('Ctrl Pts',(31.067,-2.47539248397361,5.75454770723132));
#38045=CARTESIAN_POINT('Ctrl Pts',(31.067,-2.31473325949493,5.81353255724385));
#38046=CARTESIAN_POINT('Ctrl Pts',(31.067,-2.1515563817662,5.86599474730277));
#38047=CARTESIAN_POINT('Ctrl Pts',(31.067,-1.98620606863935,5.91166147165176));
#38048=CARTESIAN_POINT('Ctrl Pts',(31.067,-1.88599462349867,5.93933803515691));
#38049=CARTESIAN_POINT('Ctrl Pts',(31.067,-1.78498480160803,5.96451763689186));
#38050=CARTESIAN_POINT('Ctrl Pts',(31.067,-1.68325362372016,5.98713018070703));
#38051=CARTESIAN_POINT('Origin',(31.067,0.,0.));
#38052=CARTESIAN_POINT('Origin',(28.1999754182402,0.,0.));
#38053=CARTESIAN_POINT('Ctrl Pts',(31.067,-1.68325362372015,5.98713018070703));
#38054=CARTESIAN_POINT('Ctrl Pts',(31.100085267407,-2.67894146944392,5.70719720383451));
#38055=CARTESIAN_POINT('Ctrl Pts',(31.166255802221,-4.52416925940906,4.64399692160856));
#38056=CARTESIAN_POINT('Ctrl Pts',(31.2522476083012,-5.97677244814931,2.2702138283845));
#38057=CARTESIAN_POINT('Ctrl Pts',(31.3051541469743,-6.21736961784573,0.620749375332392));
#38058=CARTESIAN_POINT('Ctrl Pts',(31.3249754182403,-6.21654608244749,0.00207115560223001));
#38059=CARTESIAN_POINT('Ctrl Pts',(30.6549162453659,-1.87643162330758,6.67424103273558));
#38060=CARTESIAN_POINT('Ctrl Pts',(30.6880015127729,-2.98638922822823,6.36218164797731));
#38061=CARTESIAN_POINT('Ctrl Pts',(30.754172047587,-5.04338392498871,5.17696356594593));
#38062=CARTESIAN_POINT('Ctrl Pts',(30.853427849808,-6.91246875169278,2.12258368035554));
#38063=CARTESIAN_POINT('Ctrl Pts',(30.952683652029,-7.07320345546478,-1.42613979719881));
#38064=CARTESIAN_POINT('Ctrl Pts',(31.0850247216572,-5.03913679692803,-5.74620551731878));
#38065=CARTESIAN_POINT('Ctrl Pts',(31.2504510586922,1.01637773032965,-8.13586156489377));
#38066=CARTESIAN_POINT('Ctrl Pts',(31.4489626631344,7.40108795243844,-3.53348110298655));
#38067=CARTESIAN_POINT('Ctrl Pts',(31.6143890001694,7.04014314253548,2.9701480866463));
#38068=CARTESIAN_POINT('Ctrl Pts',(31.7467300697975,3.58881749933384,6.25980480689558));
#38069=CARTESIAN_POINT('Ctrl Pts',(31.8459858720186,0.159432186662248,7.23304908842483));
#38070=CARTESIAN_POINT('Ctrl Pts',(31.9452416742397,-3.30635190225879,6.4120734720337));
#38071=CARTESIAN_POINT('Ctrl Pts',(32.0775827438677,-6.90505735872034,3.28023028088796));
#38072=CARTESIAN_POINT('Ctrl Pts',(32.2430090809028,-7.54381322647391,-3.20505761210972));
#38073=CARTESIAN_POINT('Ctrl Pts',(32.4415206853449,-1.38653337747383,-8.07830009000535));
#38074=CARTESIAN_POINT('Ctrl Pts',(32.640032289787,6.03340921861916,-5.54788315750085));
#38075=CARTESIAN_POINT('Ctrl Pts',(32.8385438942292,7.93033714683168,2.07205611235235));
#38076=CARTESIAN_POINT('Ctrl Pts',(33.0039702312642,3.46180249906012,6.81563813838305));
#38077=CARTESIAN_POINT('Ctrl Pts',(33.1363113008923,-1.29997896114567,7.09628287091765));
#38078=CARTESIAN_POINT('Ctrl Pts',(33.2355671031133,-4.54639362325622,5.62827366693923));
#38079=CARTESIAN_POINT('Ctrl Pts',(33.3348229053344,-6.66425465276717,2.76313547380338));
#38080=CARTESIAN_POINT('Ctrl Pts',(33.4671639749625,-7.39119473715877,-1.95117347127662));
#38081=CARTESIAN_POINT('Ctrl Pts',(33.6325903119975,-3.693357430702,-7.31732226708638));
#38082=CARTESIAN_POINT('Ctrl Pts',(33.8311019164397,4.15513537654513,-7.06509570019544));
#38083=CARTESIAN_POINT('Ctrl Pts',(34.0296135208818,8.18919366122636,-0.343265517627367));
#38084=CARTESIAN_POINT('Ctrl Pts',(34.2281251253239,4.71981863488245,6.70129840887398));
#38085=CARTESIAN_POINT('Ctrl Pts',(34.393551462359,-1.75502246952579,7.44021165588655));
#38086=CARTESIAN_POINT('Ctrl Pts',(34.525892531987,-5.57321788935264,4.58109536851286));
#38087=CARTESIAN_POINT('Ctrl Pts',(34.6251483342082,-7.10531700255993,1.36442061554992));
#38088=CARTESIAN_POINT('Ctrl Pts',(34.7244041364292,-6.87364072807772,-2.19094856972063));
#38089=CARTESIAN_POINT('Ctrl Pts',(34.8567452060573,-4.38603192732624,-6.26095659180019));
#38090=CARTESIAN_POINT('Ctrl Pts',(35.0221715430924,1.90196620680996,-7.97286720693537));
#38091=CARTESIAN_POINT('Ctrl Pts',(35.2206831475345,7.73386740697045,-2.71440995635487));
#38092=CARTESIAN_POINT('Ctrl Pts',(35.4191947519766,6.47649012537996,5.02352487399142));
#38093=CARTESIAN_POINT('Ctrl Pts',(35.6177063564187,-0.720339615174119,
8.16487585904735));
#38094=CARTESIAN_POINT('Ctrl Pts',(35.7831326934538,-6.14277290065803,4.55007632360081));
#38095=CARTESIAN_POINT('Ctrl Pts',(35.9154737630819,-7.21370596289137,-0.0981776753163467));
#38096=CARTESIAN_POINT('Ctrl Pts',(36.0147295653029,-6.30772612813385,-3.54397577118503));
#38097=CARTESIAN_POINT('Ctrl Pts',(36.113985367524,-3.83595946031657,-6.11004153773871));
#38098=CARTESIAN_POINT('Ctrl Pts',(36.246326437152,0.691068351408432,-7.61309910580096));
#38099=CARTESIAN_POINT('Ctrl Pts',(36.4117527741872,6.59881128900457,-4.86207533144359));
#38100=CARTESIAN_POINT('Ctrl Pts',(36.6102643786292,7.65916482667057,2.91854769567105));
#38101=CARTESIAN_POINT('Ctrl Pts',(36.8087759830714,1.70432940577044,8.01723067963919));
#38102=CARTESIAN_POINT('Ctrl Pts',(37.0072875875134,-5.82021344348282,5.77141251591789));
#38103=CARTESIAN_POINT('Ctrl Pts',(37.1727139245487,-7.62871246207274,-0.489489154279525));
#38104=CARTESIAN_POINT('Ctrl Pts',(37.3050549941766,-5.44648042441822,-4.73107213644686));
#38105=CARTESIAN_POINT('Ctrl Pts',(37.4043107963977,-2.53040138538347,-6.77821820272855));
#38106=CARTESIAN_POINT('Ctrl Pts',(37.5035665986188,1.01380720327794,-7.14278569806071));
#38107=CARTESIAN_POINT('Ctrl Pts',(37.6359076682468,5.44171187513046,-5.36885698535498));
#38108=CARTESIAN_POINT('Ctrl Pts',(37.8013340052819,8.17841552233659,0.545533225941051));
#38109=CARTESIAN_POINT('Ctrl Pts',(37.999845609724,3.96631642533182,7.17280004657078));
#38110=CARTESIAN_POINT('Ctrl Pts',(38.1983572141662,-3.87294681277729,7.22364239697269));
#38111=CARTESIAN_POINT('Ctrl Pts',(38.3968688186083,-8.17065160671188,0.65156678731938));
#38112=CARTESIAN_POINT('Ctrl Pts',(38.5622951556433,-5.51089172685842,-5.29782274486176));
#38113=CARTESIAN_POINT('Ctrl Pts',(38.6946362252715,-1.10636856916135,-7.12903507937862));
#38114=CARTESIAN_POINT('Ctrl Pts',(38.7938920274925,2.44227055290094,-6.81046897954778));
#38115=CARTESIAN_POINT('Ctrl Pts',(38.8931478297135,5.38465712099301,-4.80131859630022));
#38116=CARTESIAN_POINT('Ctrl Pts',(39.0254888993417,7.62172171751438,-0.588397418332726));
#38117=CARTESIAN_POINT('Ctrl Pts',(39.1909152363767,5.89458286590277,5.69543499599519));
#38118=CARTESIAN_POINT('Ctrl Pts',(39.3894268408188,-1.60019725410325,8.03866252817617));
#38119=CARTESIAN_POINT('Ctrl Pts',(39.5879384452609,-7.62066502615036,3.01764660839399));
#38120=CARTESIAN_POINT('Ctrl Pts',(39.786450049703,-6.66132050968186,-4.77607537879091));
#38121=CARTESIAN_POINT('Ctrl Pts',(39.9518763867381,-0.789757142543198,
-7.60349505930879));
#38122=CARTESIAN_POINT('Ctrl Pts',(40.0842174563662,3.75638549375725,-6.15928247413035));
#38123=CARTESIAN_POINT('Ctrl Pts',(40.1834732585872,6.26122779876381,-3.62549301846479));
#38124=CARTESIAN_POINT('Ctrl Pts',(40.2827290608083,7.21182569809585,-0.191735948959446));
#38125=CARTESIAN_POINT('Ctrl Pts',(40.4150701304364,6.20127365133498,4.47001773625));
#38126=CARTESIAN_POINT('Ctrl Pts',(40.5804964674715,0.826182852666716,8.1548457281889));
#38127=CARTESIAN_POINT('Ctrl Pts',(40.7790080719136,-6.41078686909009,5.1071066381118));
#38128=CARTESIAN_POINT('Ctrl Pts',(40.9775196763557,-7.76842450593914,-2.61386824256068));
#38129=CARTESIAN_POINT('Ctrl Pts',(41.1760312807978,-2.00521956202275,-7.94752675142916));
#38130=CARTESIAN_POINT('Ctrl Pts',(41.3414576178329,4.30445421564323,-6.31731963466804));
#38131=CARTESIAN_POINT('Ctrl Pts',(41.473798687461,6.84464445440369,-2.27991992548857));
#38132=CARTESIAN_POINT('Ctrl Pts',(41.573054489682,7.12241671079052,1.27214518542566));
#38133=CARTESIAN_POINT('Ctrl Pts',(41.6723102919031,5.63216891050179,4.5084216681025));
#38134=CARTESIAN_POINT('Ctrl Pts',(41.8046513615311,1.8513792489286,7.41682198369137));
#38135=CARTESIAN_POINT('Ctrl Pts',(41.9700776985663,-4.6325012323385,6.76195380707258));
#38136=CARTESIAN_POINT('Ctrl Pts',(42.1685893030084,-8.19295729764973,-0.237017326015257));
#38137=CARTESIAN_POINT('Ctrl Pts',(42.3671009074505,-4.24642451586804,-7.01060663031227));
#38138=CARTESIAN_POINT('Ctrl Pts',(42.5656125118925,3.59813568041071,-7.36461177401473));
#38139=CARTESIAN_POINT('Ctrl Pts',(42.7310388489278,7.36526593039372,-2.04687841253758));
#38140=CARTESIAN_POINT('Ctrl Pts',(42.8633799185557,6.69953237756773,2.67646380430612));
#38141=CARTESIAN_POINT('Ctrl Pts',(42.9626357207769,4.61901655424491,5.56882925277487));
#38142=CARTESIAN_POINT('Ctrl Pts',(43.0618915229978,1.39190762332577,7.07882657945274));
#38143=CARTESIAN_POINT('Ctrl Pts',(43.194232592626,-3.37309616097341,6.85996178924909));
#38144=CARTESIAN_POINT('Ctrl Pts',(43.359658929661,-7.90281813252849,2.17475343907767));
#38145=CARTESIAN_POINT('Ctrl Pts',(43.5581705341032,-6.10482138465689,-5.46917565592653));
#38146=CARTESIAN_POINT('Ctrl Pts',(43.7566821385453,1.28156221813536,-8.09557439438308));
#38147=CARTESIAN_POINT('Ctrl Pts',(43.9551937429874,7.50175213064336,-3.30269616025889));
#38148=CARTESIAN_POINT('Ctrl Pts',(44.1206200800225,6.94676798905697,3.19049650796619));
#38149=CARTESIAN_POINT('Ctrl Pts',(44.2529611496505,3.38959938145578,6.368501284217));
#38150=CARTESIAN_POINT('Ctrl Pts',(44.3522169518717,-0.0663807020241724,
7.23483011392448));
#38151=CARTESIAN_POINT('Ctrl Pts',(44.4514727540926,-3.50588289361426,6.30523415188539));
#38152=CARTESIAN_POINT('Ctrl Pts',(44.5838138237208,-7.00414016531606,3.06249473562607));
#38153=CARTESIAN_POINT('Ctrl Pts',(44.7492401607558,-7.43988877947175,-3.43978806115894));
#38154=CARTESIAN_POINT('Ctrl Pts',(44.947751765198,-1.13280263660267,-8.11772657093409));
#38155=CARTESIAN_POINT('Ctrl Pts',(45.1462633696401,6.20414626300639,-5.35623894548842));
#38156=CARTESIAN_POINT('Ctrl Pts',(45.3447749740821,7.86158362152895,2.31939429987847));
#38157=CARTESIAN_POINT('Ctrl Pts',(45.5102013111174,3.24665643439725,6.92069905848522));
#38158=CARTESIAN_POINT('Ctrl Pts',(45.6425423807453,-1.52156104753122,7.05209504703919));
#38159=CARTESIAN_POINT('Ctrl Pts',(45.7417981829665,-4.72042009291361,5.48313845542561));
#38160=CARTESIAN_POINT('Ctrl Pts',(45.8410539851874,-6.74751430915288,2.55308504002825));
#38161=CARTESIAN_POINT('Ctrl Pts',(45.9733950548156,-7.32646826719433,-2.18167738011961));
#38162=CARTESIAN_POINT('Ctrl Pts',(46.1388213918505,-3.46239836164604,-7.42939328221839));
#38163=CARTESIAN_POINT('Ctrl Pts',(46.3373329962928,4.37434562194319,-6.93150971100306));
#38164=CARTESIAN_POINT('Ctrl Pts',(46.5358446007348,8.19592696626587,-0.0866467401548151));
#38165=CARTESIAN_POINT('Ctrl Pts',(46.734356205177,4.50764780719777,6.8458161093376));
#38166=CARTESIAN_POINT('Ctrl Pts',(46.899782542212,-1.98715711947764,7.381602809935));
#38167=CARTESIAN_POINT('Ctrl Pts',(47.0321236118402,-5.71394470796255,4.40431929453189));
#38168=CARTESIAN_POINT('Ctrl Pts',(47.1313794140611,-7.14455993023938,1.14124343510381));
#38169=CARTESIAN_POINT('Ctrl Pts',(47.2306352162823,-6.80165841434973,-2.40512689651597));
#38170=CARTESIAN_POINT('Ctrl Pts',(47.3629762859103,-4.18781450800034,-6.39523753333001));
#38171=CARTESIAN_POINT('Ctrl Pts',(47.5284026229455,2.15070931246681,-7.90939545160498));
#38172=CARTESIAN_POINT('Ctrl Pts',(47.7269142273875,7.81507793497872,-2.47088716135563));
#38173=CARTESIAN_POINT('Ctrl Pts',(47.9254258318296,6.31599847344063,5.2238768914896));
#38174=CARTESIAN_POINT('Ctrl Pts',(48.1239374362717,-0.975675145363378,
8.13831339819997));
#38175=CARTESIAN_POINT('Ctrl Pts',(48.2893637733068,-6.28224897351141,4.35547945649454));
#38176=CARTESIAN_POINT('Ctrl Pts',(48.4217048429349,-7.20709344807375,-0.324031795618007));
#38177=CARTESIAN_POINT('Ctrl Pts',(48.5209606451559,-6.19365036830372,-3.7397684808235));
#38178=CARTESIAN_POINT('Ctrl Pts',(48.620216447377,-3.64273784243868,-6.22717059225972));
#38179=CARTESIAN_POINT('Ctrl Pts',(48.752557517005,0.929138961386053,-7.58772391772166));
#38180=CARTESIAN_POINT('Ctrl Pts',(48.9179838540402,6.74783416273851,-4.65304427969263));
#38181=CARTESIAN_POINT('Ctrl Pts',(49.1164954584823,7.56401196412085,3.15696840348137));
#38182=CARTESIAN_POINT('Ctrl Pts',(49.3150070629244,1.4524282921612,8.06667084676652));
#38183=CARTESIAN_POINT('Ctrl Pts',(49.5135186673665,-5.99809471893604,5.58631781223311));
#38184=CARTESIAN_POINT('Ctrl Pts',(49.6789450044016,-7.60964221054302,-0.728147573403291));
#38185=CARTESIAN_POINT('Ctrl Pts',(49.8112860740297,-5.29565231143276,-4.89931211194549));
#38186=CARTESIAN_POINT('Ctrl Pts',(49.9105418762507,-2.31689566560535,-6.85413507669997));
#38187=CARTESIAN_POINT('Ctrl Pts',(50.0097976784718,1.23699132885906,-7.10753438445193));
#38188=CARTESIAN_POINT('Ctrl Pts',(50.1421387480998,5.60717247991814,-5.19581276044276));
#38189=CARTESIAN_POINT('Ctrl Pts',(50.307565085135,8.15732060565719,0.801378495544836));
#38190=CARTESIAN_POINT('Ctrl Pts',(50.5060766895771,3.73974984335584,7.29349008383935));
#38191=CARTESIAN_POINT('Ctrl Pts',(50.7045882940192,-4.09726073797571,7.09881546027125));
#38192=CARTESIAN_POINT('Ctrl Pts',(50.9030998984613,-8.18704852617428,0.395377524233446));
#38193=CARTESIAN_POINT('Ctrl Pts',(51.0685262354963,-5.34228382927205,-5.46780183882237));
#38194=CARTESIAN_POINT('Ctrl Pts',(51.2008673051245,-0.882575199040403,
-7.1601853042975));
#38195=CARTESIAN_POINT('Ctrl Pts',(51.3001231073455,2.65434734717859,-6.7306473192016));
#38196=CARTESIAN_POINT('Ctrl Pts',(51.3993789095665,5.5323728451407,-4.63033943423036));
#38197=CARTESIAN_POINT('Ctrl Pts',(51.5317199791947,7.63640967023901,-0.349429262385304));
#38198=CARTESIAN_POINT('Ctrl Pts',(51.6971463162297,5.7133352772524,5.87723463597501));
#38199=CARTESIAN_POINT('Ctrl Pts',(51.8956579206719,-1.85114879322649,7.98460860902268));
#38200=CARTESIAN_POINT('Ctrl Pts',(52.0941695251139,-7.71142714287807,2.77752010146219));
#38201=CARTESIAN_POINT('Ctrl Pts',(52.2926811295562,-6.50848726183514,-4.98233685323774));
#38202=CARTESIAN_POINT('Ctrl Pts',(52.4581074665911,-0.551261008942458,
-7.6244976727094));
#38203=CARTESIAN_POINT('Ctrl Pts',(52.5904485362193,3.94742540820808,-6.03862775972094));
#38204=CARTESIAN_POINT('Ctrl Pts',(52.6897043384403,6.37169179839973,-3.42764012130142));
#38205=CARTESIAN_POINT('Ctrl Pts',(52.7889601406614,7.21429295444991,0.0342014796987391));
#38206=CARTESIAN_POINT('Ctrl Pts',(52.9213012102894,6.05825044682572,4.66202262807325));
#38207=CARTESIAN_POINT('Ctrl Pts',(53.0867275473245,0.570402920122291,8.17671862456552));
#38208=CARTESIAN_POINT('Ctrl Pts',(53.2852391517666,-6.56757528827362,4.90384352592947));
#38209=CARTESIAN_POINT('Ctrl Pts',(53.4837507562088,-7.68275930744305,-2.85585992615889));
#38210=CARTESIAN_POINT('Ctrl Pts',(53.6822623606508,-1.75535370226148,-8.00642369204619));
#38211=CARTESIAN_POINT('Ctrl Pts',(53.847688697686,4.50017437076574,-6.17942425261726));
#38212=CARTESIAN_POINT('Ctrl Pts',(53.980029767314,6.91268474619889,-2.06445687131224));
#38213=CARTESIAN_POINT('Ctrl Pts',(54.0792855695351,7.07908535181276,1.49456473820969));
#38214=CARTESIAN_POINT('Ctrl Pts',(54.1785413717561,5.48822218121968,4.68258580950818));
#38215=CARTESIAN_POINT('Ctrl Pts',(54.3108824413843,1.61820823400769,7.47116159459295));
#38216=CARTESIAN_POINT('Ctrl Pts',(54.4763087784192,-4.84198452615164,6.61356732823588));
#38217=CARTESIAN_POINT('Ctrl Pts',(54.6748203828615,-8.18151664109748,-0.49346929528404));
#38218=CARTESIAN_POINT('Ctrl Pts',(54.8733319873035,-4.02479975377234,-7.14014799818442));
#38219=CARTESIAN_POINT('Ctrl Pts',(55.0718435917456,3.82699894374387,-7.24832160166644));
#38220=CARTESIAN_POINT('Ctrl Pts',(55.2372699287808,7.42575302102872,-1.81522602774813));
#38221=CARTESIAN_POINT('Ctrl Pts',(55.3696109984087,6.61243120057668,2.88495167922774));
#38222=CARTESIAN_POINT('Ctrl Pts',(55.46886680063,4.44235932371993,5.7107457318557));
#38223=CARTESIAN_POINT('Ctrl Pts',(55.5681226028508,1.16954652307012,7.11894328564385));
#38224=CARTESIAN_POINT('Ctrl Pts',(55.7004636724791,-3.58626632753348,6.75096639668209));
#38225=CARTESIAN_POINT('Ctrl Pts',(55.8658900095141,-7.96704607330977,1.92620451208082));
#38226=CARTESIAN_POINT('Ctrl Pts',(56.0644016139562,-5.93055615333192,-5.65767003333709));
#38227=CARTESIAN_POINT('Ctrl Pts',(56.2629132183984,1.53445226909902,-8.05147084251073));
#38228=CARTESIAN_POINT('Ctrl Pts',(56.4614248228403,7.60149909607939,-3.06615368970725));
#38229=CARTESIAN_POINT('Ctrl Pts',(56.6268511598756,6.84344825826143,3.40647462894263));
#38230=CARTESIAN_POINT('Ctrl Pts',(56.7591922295035,3.18850283536113,6.47152549579565));
#38231=CARTESIAN_POINT('Ctrl Pts',(56.8584480317247,-0.292911935040842,
7.22920298326586));
#38232=CARTESIAN_POINT('Ctrl Pts',(56.9577038339457,-3.70161624816119,6.19235251945399));
#38233=CARTESIAN_POINT('Ctrl Pts',(57.0900449035739,-7.09660911153827,2.84165314195156));
#38234=CARTESIAN_POINT('Ctrl Pts',(57.2554712406088,-7.32852045398567,-3.67108633950697));
#38235=CARTESIAN_POINT('Ctrl Pts',(57.453982845051,-0.878034732768776,-8.14921968669363));
#38236=CARTESIAN_POINT('Ctrl Pts',(57.652494449493,6.36883778380394,-5.15932474046112));
#38237=CARTESIAN_POINT('Ctrl Pts',(57.8510060539352,7.78509439098304,2.56444775343258));
#38238=CARTESIAN_POINT('Ctrl Pts',(58.0164323909703,3.02833753425322,7.01897608200542));
#38239=CARTESIAN_POINT('Ctrl Pts',(58.1487734605984,-1.74165610026088,7.00098754478702));
#38240=CARTESIAN_POINT('Ctrl Pts',(58.2480292628194,-4.88981326478571,5.33262593948569));
#38241=CARTESIAN_POINT('Ctrl Pts',(58.3472850650406,-6.82415659664868,2.34052970890252));
#38242=CARTESIAN_POINT('Ctrl Pts',(58.4796261346684,-7.25455418979818,-2.41004086446941));
#38243=CARTESIAN_POINT('Ctrl Pts',(58.6450524717038,-3.22804353224311,-7.53417692323086));
#38244=CARTESIAN_POINT('Ctrl Pts',(58.8435640761456,4.5892652922565,-6.79112439668372));
#38245=CARTESIAN_POINT('Ctrl Pts',(59.042075680588,8.19462062093288,0.170056969646981));
#38246=CARTESIAN_POINT('Ctrl Pts',(59.2405872850298,4.29105545732191,6.98361869082136));
#38247=CARTESIAN_POINT('Ctrl Pts',(59.4060136220652,-2.21734258458696,7.31575323009928));
#38248=CARTESIAN_POINT('Ctrl Pts',(59.5383546916931,-5.84906661858366,4.22322297128738));
#38249=CARTESIAN_POINT('Ctrl Pts',(59.6376104939143,-7.17679467182627,0.916946788748299));
#38250=CARTESIAN_POINT('Ctrl Pts',(59.7368662961352,-6.72300425491146,-2.61694599911454));
#38251=CARTESIAN_POINT('Ctrl Pts',(59.8692073657634,-3.98548920736035,-6.52324529963));
#38252=CARTESIAN_POINT('Ctrl Pts',(60.0346337027983,2.39734275979888,-7.83816526035532));
#38253=CARTESIAN_POINT('Ctrl Pts',(60.2331453072407,7.88862254419044,-2.22494063948536));
#38254=CARTESIAN_POINT('Ctrl Pts',(60.4316569116826,6.14931137206838,5.41910473632808));
#38255=CARTESIAN_POINT('Ctrl Pts',(60.6301685161249,-1.23005362269408,8.10376795335961));
#38256=CARTESIAN_POINT('Ctrl Pts',(60.7955948531598,-6.41556270153213,4.1566102395872));
#38257=CARTESIAN_POINT('Ctrl Pts',(60.9279359227879,-7.19341139597279,-0.549568068693677));
#38258=CARTESIAN_POINT('Ctrl Pts',(61.027191725009,-6.07349917136267,-3.93189279996371));
#38259=CARTESIAN_POINT('Ctrl Pts',(61.1264475272301,-3.44594301279078,-6.33819132927032));
#38260=CARTESIAN_POINT('Ctrl Pts',(61.2587885968582,1.16629816615583,-7.55490582659723));
#38261=CARTESIAN_POINT('Ctrl Pts',(61.4242149338931,6.89023799286911,-4.43944899263683));
#38262=CARTESIAN_POINT('Ctrl Pts',(61.6227265383354,7.4614394579179,3.39229239744583));
#38263=CARTESIAN_POINT('Ctrl Pts',(61.8212381427774,1.19910247160641,8.10819830520507));
#38264=CARTESIAN_POINT('Ctrl Pts',(62.0197497472196,-6.17009238055327,5.39574341236128));
#38265=CARTESIAN_POINT('Ctrl Pts',(62.1851760842547,-7.58310755601865,-0.966091742530031));
#38266=CARTESIAN_POINT('Ctrl Pts',(62.3175171538827,-5.13962962005787,-5.06274628462288));
#38267=CARTESIAN_POINT('Ctrl Pts',(62.4167729561038,-2.10111727091473,-6.9233286350435));
#38268=CARTESIAN_POINT('Ctrl Pts',(62.5160287583248,1.45896207258534,-7.06531119233941));
#38269=CARTESIAN_POINT('Ctrl Pts',(62.648369827953,5.76713293188694,-5.01767189113402));
#38270=CARTESIAN_POINT('Ctrl Pts',(62.813796164988,8.12822406069122,1.05643768192989));
#38271=CARTESIAN_POINT('Ctrl Pts',(63.0123077694301,3.5095148891804,7.40702583609401));
#38272=CARTESIAN_POINT('Ctrl Pts',(63.2108193738722,-4.31755560360744,6.96702519757902));
#38273=CARTESIAN_POINT('Ctrl Pts',(63.4093309783143,-8.19541465682279,0.138800429881101));
#38274=CARTESIAN_POINT('Ctrl Pts',(63.5747573153495,-5.16843561179771,-5.6324174905481));
#38275=CARTESIAN_POINT('Ctrl Pts',(63.7070983849775,-0.657916098734519,
-7.18431200469918));
#38276=CARTESIAN_POINT('Ctrl Pts',(63.8063541871985,2.86382045553496,-6.64422347407206));
#38277=CARTESIAN_POINT('Ctrl Pts',(63.9056099894197,5.67466178846288,-4.45481830834851));
#38278=CARTESIAN_POINT('Ctrl Pts',(64.0379510590476,7.64360696339799,-0.110118346455386));
#38279=CARTESIAN_POINT('Ctrl Pts',(64.2033773960828,5.52648339923105,6.0532692154428));
#38280=CARTESIAN_POINT('Ctrl Pts',(64.4018890005249,-2.10028451496734,7.92272247716148));
#38281=CARTESIAN_POINT('Ctrl Pts',(64.600400604967,-7.79462501436703,2.53466908675698));
#38282=CARTESIAN_POINT('Ctrl Pts',(64.7989122094091,-6.34926974906822,-5.18371108475186));
#38283=CARTESIAN_POINT('Ctrl Pts',(64.9643385464442,-0.312224135817155,
-7.63802131118276));
#38284=CARTESIAN_POINT('Ctrl Pts',(65.0966796160723,4.13459323863624,-5.9120496720641));
#38285=CARTESIAN_POINT('Ctrl Pts',(65.1959354182933,6.47590571766751,-3.22642500465688));
#38286=CARTESIAN_POINT('Ctrl Pts',(65.2951912205144,7.20968361135704,0.260105359630372));
#38287=CARTESIAN_POINT('Ctrl Pts',(65.4275322901425,5.90928462087591,4.8494544776534));
#38288=CARTESIAN_POINT('Ctrl Pts',(65.5929586271776,0.314063471532927,8.19057086476803));
#38289=CARTESIAN_POINT('Ctrl Pts',(65.7914702316197,-6.71792148235531,4.69577016617119));
#38290=CARTESIAN_POINT('Ctrl Pts',(65.9899818360618,-7.58955798424059,-3.09505025768462));
#38291=CARTESIAN_POINT('Ctrl Pts',(66.1884934405039,-1.50376599212421,-8.05746702061639));
#38292=CARTESIAN_POINT('Ctrl Pts',(66.353919777539,4.69148024327508,-6.03546738918793));
#38293=CARTESIAN_POINT('Ctrl Pts',(66.486260847167,6.97394428949912,-1.84696876138537));
#38294=CARTESIAN_POINT('Ctrl Pts',(66.5855166493881,7.02881002188407,1.71551824848117));
#38295=CARTESIAN_POINT('Ctrl Pts',(66.6847724516092,5.33889197633087,4.85215674409092));
#38296=CARTESIAN_POINT('Ctrl Pts',(66.8171135212373,1.38344990231137,7.51817262669399));
#38297=CARTESIAN_POINT('Ctrl Pts',(66.9825398582723,-5.04671826279436,6.45869353721455));
#38298=CARTESIAN_POINT('Ctrl Pts',(67.1810514627146,-8.16205060168547,-0.749437259000661));
#38299=CARTESIAN_POINT('Ctrl Pts',(67.3795630671564,-3.79922704754698,-7.26268541304556));
#38300=CARTESIAN_POINT('Ctrl Pts',(67.5780746715988,4.05210832491136,-7.12492161511161));
#38301=CARTESIAN_POINT('Ctrl Pts',(67.7435010086337,7.47895595825633,-1.58179277372035));
#38302=CARTESIAN_POINT('Ctrl Pts',(67.8758420782618,6.5188439801296,3.09060926131331));
#38303=CARTESIAN_POINT('Ctrl Pts',(67.9750978804829,4.26134412521868,5.8470613439865));
#38304=CARTESIAN_POINT('Ctrl Pts',(68.074353682704,0.946038930223685,7.15207529371878));
#38305=CARTESIAN_POINT('Ctrl Pts',(68.206694752332,-3.7959202569988,6.6353524066251));
#38306=CARTESIAN_POINT('Ctrl Pts',(68.3721210893672,-8.02345580532069,1.67575897078913));
#38307=CARTESIAN_POINT('Ctrl Pts',(68.5706326938091,-5.75047892022695,-5.8406027897517));
#38308=CARTESIAN_POINT('Ctrl Pts',(68.7691442982514,1.78584702629977,-7.99949146132116));
#38309=CARTESIAN_POINT('Ctrl Pts',(68.9676559026935,7.69377017617253,-2.82656025581714));
#38310=CARTESIAN_POINT('Ctrl Pts',(69.1330822397285,6.73344991610245,3.61903513164787));
#38311=CARTESIAN_POINT('Ctrl Pts',(69.2654233093567,2.98423080922018,6.56830815330687));
#38312=CARTESIAN_POINT('Ctrl Pts',(69.3646791115776,-0.51905136839031,7.21625210960086));
#38313=CARTESIAN_POINT('Ctrl Pts',(69.4639349137988,-3.89391146946297,6.07382587552981));
#38314=CARTESIAN_POINT('Ctrl Pts',(69.5962759834268,-7.18170028038283,2.6170969569783));
#38315=CARTESIAN_POINT('Ctrl Pts',(69.7617023204619,-7.21081252221904,-3.89689416412441));
#38316=CARTESIAN_POINT('Ctrl Pts',(69.960213924904,-0.620995053939498,-8.17585747700275));
#38317=CARTESIAN_POINT('Ctrl Pts',(70.1587255293462,6.52470125732709,-4.9516117227233));
#38318=CARTESIAN_POINT('Ctrl Pts',(70.3572371337882,7.70593355233525,2.79598253320879));
#38319=CARTESIAN_POINT('Ctrl Pts',(70.5557487382304,1.81768565186861,7.99406615824949));
#38320=CARTESIAN_POINT('Ctrl Pts',(70.7211750752654,-4.45822679105659,6.2121217551084));
#38321=CARTESIAN_POINT('Ctrl Pts',(70.8535161448936,-6.88881467085553,2.11853700674387));
#38322=CARTESIAN_POINT('Ctrl Pts',(70.9858572145215,-7.17723399063616,-2.63013344355206));
#38323=CARTESIAN_POINT('Ctrl Pts',(71.1512835515568,-2.99445485884597,-7.63635188476723));
#38324=CARTESIAN_POINT('Ctrl Pts',(71.3497951559987,4.80978360231764,-6.63921429906795));
#38325=CARTESIAN_POINT('Ctrl Pts',(71.515221493034,7.60411813277866,-0.758311536326274));
#38326=CARTESIAN_POINT('Ctrl Pts',(71.6475625626619,6.14450154704762,3.78291426296633));
#38327=CARTESIAN_POINT('Ctrl Pts',(71.7468183648831,3.59819571462861,6.27635644400727));
#38328=CARTESIAN_POINT('Ctrl Pts',(71.8460741671041,0.161404155566158,7.21267391002245));
#38329=CARTESIAN_POINT('Ctrl Pts',(71.9784152367322,-4.49653865790636,6.18215858561921));
#38330=CARTESIAN_POINT('Ctrl Pts',(72.1438415737672,-8.15815741081568,0.791574195716444));
#38331=CARTESIAN_POINT('Ctrl Pts',(72.3423531782093,-5.07989086167079,-6.43244417407182));
#38332=CARTESIAN_POINT('Ctrl Pts',(72.5408647826515,2.64687881754866,-7.75723974463881));
#38333=CARTESIAN_POINT('Ctrl Pts',(72.7393763870936,7.95595254297234,-1.97144739296824));
#38334=CARTESIAN_POINT('Ctrl Pts',(72.9048027241286,6.29898760469208,4.33125433189542));
#38335=CARTESIAN_POINT('Ctrl Pts',(73.0371437937569,2.25081894201211,6.85426618338362));
#38336=CARTESIAN_POINT('Ctrl Pts',(73.1363995959777,-1.30238688003595,7.11694925165258));
#38337=CARTESIAN_POINT('Ctrl Pts',(73.235655398199,-4.53230734834526,5.61296614737723));
#38338=CARTESIAN_POINT('Ctrl Pts',(73.3679964678268,-7.4246188108322,1.81985648838285));
#38339=CARTESIAN_POINT('Ctrl Pts',(73.5334228048621,-6.74221461261432,-4.66118406180153));
#38340=CARTESIAN_POINT('Ctrl Pts',(73.731934409304,0.27181873891023,-8.19187645961583));
#38341=CARTESIAN_POINT('Ctrl Pts',(73.9304460137463,7.02858186584606,-4.21660550406958));
#38342=CARTESIAN_POINT('Ctrl Pts',(74.1289576181883,7.34926068645952,3.62938777901172));
#38343=CARTESIAN_POINT('Ctrl Pts',(74.2943839552235,2.01557258935635,7.3738945111119));
#38344=CARTESIAN_POINT('Ctrl Pts',(74.4267250248515,-2.70489894858274,6.68810243885279));
#38345=CARTESIAN_POINT('Ctrl Pts',(74.5259808270726,-5.5884003905664,4.59531874068335));
#38346=CARTESIAN_POINT('Ctrl Pts',(74.6252366292936,-7.08467546628861,1.36182453082842));
#38347=CARTESIAN_POINT('Ctrl Pts',(74.7575776989218,-6.84557113769722,-3.40220653545019));
#38348=CARTESIAN_POINT('Ctrl Pts',(74.9230040359568,-2.14116300119577,-7.91198508227128));
#38349=CARTESIAN_POINT('Ctrl Pts',(75.1215156403989,5.49505931408899,-6.08153349264663));
#38350=CARTESIAN_POINT('Ctrl Pts',(75.3200272448411,8.0900573333749,1.31594028931691));
#38351=CARTESIAN_POINT('Ctrl Pts',(75.5185388492831,3.27079925713886,7.51571414921572));
#38352=CARTESIAN_POINT('Ctrl Pts',(75.6839651863183,-3.21997727761606,6.93315222625922));
#38353=CARTESIAN_POINT('Ctrl Pts',(75.8163062559462,-6.38284268877731,3.36251569288139));
#38354=CARTESIAN_POINT('Ctrl Pts',(75.9155620581674,-7.23448285468373,-0.097113334340778));
#38355=CARTESIAN_POINT('Ctrl Pts',(76.0148178603884,-6.29028443025259,-3.53263561107129));
#38356=CARTESIAN_POINT('Ctrl Pts',(76.1471589300166,-3.03271383316493,-7.01708630894154));
#38357=CARTESIAN_POINT('Ctrl Pts',(76.3125852670515,3.47136133651406,-7.42520958814913));
#38358=CARTESIAN_POINT('Ctrl Pts',(76.5110968714938,8.12246542232142,-1.09830868028507));
#38359=CARTESIAN_POINT('Ctrl Pts',(76.7096084759357,5.32983568543061,6.22684334636948));
#38360=CARTESIAN_POINT('Ctrl Pts',(76.908120080378,-2.35276902473004,7.85166000746804));
#38361=CARTESIAN_POINT('Ctrl Pts',(77.073546417413,-6.93442826554184,3.21722832437996));
#38362=CARTESIAN_POINT('Ctrl Pts',(77.2058874870412,-7.0455678962576,-1.5515043000454));
#38363=CARTESIAN_POINT('Ctrl Pts',(77.3051432892621,-5.46303685210097,-4.74366962672763));
#38364=CARTESIAN_POINT('Ctrl Pts',(77.4043990914832,-2.52439886881471,-6.75829881885711));
#38365=CARTESIAN_POINT('Ctrl Pts',(77.5367401611113,2.21278020170318,-7.31713449651446));
#38366=CARTESIAN_POINT('Ctrl Pts',(77.7021664981463,7.44403436148341,-3.43080739501002));
#38367=CARTESIAN_POINT('Ctrl Pts',(77.9006781025885,6.91286514831034,4.40375089386527));
#38368=CARTESIAN_POINT('Ctrl Pts',(78.0991897070305,0.0518300311409729,
8.19622108912486));
#38369=CARTESIAN_POINT('Ctrl Pts',(78.2977013114727,-6.86490262637786,4.47852641914182));
#38370=CARTESIAN_POINT('Ctrl Pts',(78.4631276485078,-7.37309485507158,-2.01849590518484));
#38371=CARTESIAN_POINT('Ctrl Pts',(78.5954687181359,-4.38000697731177,-5.73260250257588));
#38372=CARTESIAN_POINT('Ctrl Pts',(78.694724520357,-1.11088337052448,-7.14934341824773));
#38373=CARTESIAN_POINT('Ctrl Pts',(78.793980322578,2.43399833347421,-6.79138017537552));
#38374=CARTESIAN_POINT('Ctrl Pts',(78.9263213922061,6.4129694783647,-4.16061004309389));
#38375=CARTESIAN_POINT('Ctrl Pts',(79.091747729241,7.90018797235732,2.18428866178938));
#38376=CARTESIAN_POINT('Ctrl Pts',(79.2902593336834,2.43766676976039,7.82550363960998));
#38377=CARTESIAN_POINT('Ctrl Pts',(79.4887709381253,-5.25065983451864,6.2937506938324));
#38378=CARTESIAN_POINT('Ctrl Pts',(79.6872825425675,-8.13409534553851,-1.01023752963825));
#38379=CARTESIAN_POINT('Ctrl Pts',(79.8527088796026,-4.3287534491085,-6.30069417111822));
#38380=CARTESIAN_POINT('Ctrl Pts',(79.9850499492307,0.354644279160853,-7.20565194892855));
#38381=CARTESIAN_POINT('Ctrl Pts',(80.0843057514517,3.76604508515065,-6.17770811802905));
#38382=CARTESIAN_POINT('Ctrl Pts',(80.1835615536727,6.24258859266155,-3.61625223630912));
#38383=CARTESIAN_POINT('Ctrl Pts',(80.3159026233008,7.583708516415,0.961362886316208));
#38384=CARTESIAN_POINT('Ctrl Pts',(80.4813289603358,4.62433780266202,6.76753920147287));
#38385=CARTESIAN_POINT('Ctrl Pts',(80.6798405647781,-3.18907150028927,7.55053305800232));
#38386=CARTESIAN_POINT('Ctrl Pts',(80.8783521692201,-8.07276791414114,1.41814833439819));
#38387=CARTESIAN_POINT('Ctrl Pts',(81.0768637736623,-5.56078777391149,-6.02177102604519));
#38388=CARTESIAN_POINT('Ctrl Pts',(81.2422901106974,0.760466419715527,-7.60648041380617));
#38389=CARTESIAN_POINT('Ctrl Pts',(81.3746311803254,4.92176359902424,-5.27479247451109));
#38390=CARTESIAN_POINT('Ctrl Pts',(81.4738869825466,6.86391530262252,-2.28775870523392));
#38391=CARTESIAN_POINT('Ctrl Pts',(81.5731427847675,7.10221557276389,1.26717265273106));
#38392=CARTESIAN_POINT('Ctrl Pts',(81.7054838543957,5.17194686549097,5.62919346635642));
#38393=CARTESIAN_POINT('Ctrl Pts',(81.8709101914307,-0.836023194187075,
8.15384278579016));
#38394=CARTESIAN_POINT('Ctrl Pts',(82.0694217958728,-7.30931056586058,3.70873368493102));
#38395=CARTESIAN_POINT('Ctrl Pts',(82.267933400315,-7.08134643210635,-4.12737921718344));
#38396=CARTESIAN_POINT('Ctrl Pts',(82.466445004757,-0.360595744877148,-8.18865420355369));
#38397=CARTESIAN_POINT('Ctrl Pts',(82.6318713417921,5.49044628522498,-5.31900865295313));
#38398=CARTESIAN_POINT('Ctrl Pts',(82.7642124114202,7.16386984035125,-0.852151092438711));
#38399=CARTESIAN_POINT('Ctrl Pts',(82.8634682136414,6.71931104372443,2.68291488359821));
#38400=CARTESIAN_POINT('Ctrl Pts',(82.9627240158622,4.60679638678563,5.55199240134011));
#38401=CARTESIAN_POINT('Ctrl Pts',(83.0950650854905,0.316986986568839,7.6378251296738));
#38402=CARTESIAN_POINT('Ctrl Pts',(83.2604914225255,-5.90145159800573,5.68831750107152));
#38403=CARTESIAN_POINT('Ctrl Pts',(83.4590030269676,-7.97667297070005,-1.88505034745662));
#38404=CARTESIAN_POINT('Ctrl Pts',(83.6575146314097,-2.74473724711928,-7.72315634557654));
#38405=CARTESIAN_POINT('Ctrl Pts',(83.8560262358518,5.00993965925736,-6.48726379664039));
#38406=CARTESIAN_POINT('Ctrl Pts',(84.021452572887,7.62677061175643,-0.518867513705835));
#38407=CARTESIAN_POINT('Ctrl Pts',(84.1537936425149,6.02180479091357,3.97304160989659));
#38408=CARTESIAN_POINT('Ctrl Pts',(84.2530494447361,3.40054253636251,6.38619476944906));
#38409=CARTESIAN_POINT('Ctrl Pts',(84.3523052469571,-0.0648471614422156,
7.2140825764259));
#38410=CARTESIAN_POINT('Ctrl Pts',(84.4846463165851,-4.68771573852409,6.03839172428596));
#38411=CARTESIAN_POINT('Ctrl Pts',(84.6500726536203,-8.17906789511689,0.53566344253681));
#38412=CARTESIAN_POINT('Ctrl Pts',(84.8485842580624,-4.87590051758694,-6.58834733727196));
#38413=CARTESIAN_POINT('Ctrl Pts',(85.0470958625044,2.88847017309471,-7.67055842511386));
#38414=CARTESIAN_POINT('Ctrl Pts',(85.2456074669467,8.01380811645443,-1.7213269385129));
#38415=CARTESIAN_POINT('Ctrl Pts',(85.4110338039818,6.16025196085469,4.52638368235799));
#38416=CARTESIAN_POINT('Ctrl Pts',(85.5433748736097,2.03507347224601,6.92139209526522));
#38417=CARTESIAN_POINT('Ctrl Pts',(85.6426306758309,-1.52462288789535,7.07267263661027));
#38418=CARTESIAN_POINT('Ctrl Pts',(85.7418864780518,-4.70585728012308,5.46828125035202));
#38419=CARTESIAN_POINT('Ctrl Pts',(85.8742275476801,-7.47796826070822,1.58645647686012));
#38420=CARTESIAN_POINT('Ctrl Pts',(86.039653884715,-6.59293912528612,-4.87003497388596));
#38421=CARTESIAN_POINT('Ctrl Pts',(86.2381654891572,0.528219555732677,-8.17934658728218));
#38422=CARTESIAN_POINT('Ctrl Pts',(86.4366770935992,7.15718074288302,-3.9944324137038));
#38423=CARTESIAN_POINT('Ctrl Pts',(86.6351886980415,7.23199928445137,3.85775495674566));
#38424=CARTESIAN_POINT('Ctrl Pts',(86.8006150350765,1.78366538655549,7.43339701952848));
#38425=CARTESIAN_POINT('Ctrl Pts',(86.9329561047045,-2.9130149582689,6.60011639493883));
#38426=CARTESIAN_POINT('Ctrl Pts',(87.0322119069257,-5.72956514765639,4.41806025238579));
#38427=CARTESIAN_POINT('Ctrl Pts',(87.1314677091467,-7.12384723501912,1.13929502147146));
#38428=CARTESIAN_POINT('Ctrl Pts',(87.2638087787747,-6.73567118817512,-3.61491177014297));
#38429=CARTESIAN_POINT('Ctrl Pts',(87.4292351158099,-1.89234348115796,-7.97515661952291));
#38430=CARTESIAN_POINT('Ctrl Pts',(87.6277467202519,5.68281172087316,-5.90646911775986));
#38431=CARTESIAN_POINT('Ctrl Pts',(87.8262583246941,8.04487991343423,1.56864070850067));
#38432=CARTESIAN_POINT('Ctrl Pts',(88.0247699291362,3.03383520051197,7.61445539304916));
#38433=CARTESIAN_POINT('Ctrl Pts',(88.1901962661713,-3.43551455250795,6.8289159623353));
#38434=CARTESIAN_POINT('Ctrl Pts',(88.3225373357993,-6.48501172170561,3.160983319029));
#38435=CARTESIAN_POINT('Ctrl Pts',(88.4217931380204,-7.22789348039601,-0.323618619671762));
#38436=CARTESIAN_POINT('Ctrl Pts',(88.5210489402415,-6.17657234984887,-3.72788768351753));
#38437=CARTESIAN_POINT('Ctrl Pts',(88.6533900098695,-2.81148142816453,-7.108616295751));
#38438=CARTESIAN_POINT('Ctrl Pts',(88.8188163469046,3.702184440345,-7.31285972286276));
#38439=CARTESIAN_POINT('Ctrl Pts',(89.0173279513468,8.15287601138966,-0.843409293789282));
#38440=CARTESIAN_POINT('Ctrl Pts',(89.2158395557888,5.13222365494829,6.39069689858097));
#38441=CARTESIAN_POINT('Ctrl Pts',(89.414351160231,-2.59749534447238,7.77413049106106));
#38442=CARTESIAN_POINT('Ctrl Pts',(89.5797774972659,-7.03177699352893,2.99849391768735));
#38443=CARTESIAN_POINT('Ctrl Pts',(89.7121185668942,-6.99352590129428,-1.77138026458615));
#38444=CARTESIAN_POINT('Ctrl Pts',(89.811374369115,-5.31180611963898,-4.91242189986933));
#38445=CARTESIAN_POINT('Ctrl Pts',(89.9106301713363,-2.31151988251846,-6.83403748940264));
#38446=CARTESIAN_POINT('Ctrl Pts',(90.0429712409643,2.44083613787073,-7.24425099021252));
#38447=CARTESIAN_POINT('Ctrl Pts',(90.2083975779994,7.54782152835416,-3.19600956392727));
#38448=CARTESIAN_POINT('Ctrl Pts',(90.4069091824415,6.77156813158818,4.61807227457544));
#38449=CARTESIAN_POINT('Ctrl Pts',(90.6054207868836,-0.204865813229847,
8.19382428982425));
#38450=CARTESIAN_POINT('Ctrl Pts',(90.8039323913256,-7.0017838900133,4.26135064435577));
#38451=CARTESIAN_POINT('Ctrl Pts',(90.969358728361,-7.30626805192062,-2.24839956738446));
#38452=CARTESIAN_POINT('Ctrl Pts',(91.1016997979887,-4.19833829625926,-5.86695390505177));
#38453=CARTESIAN_POINT('Ctrl Pts',(91.2009556002101,-0.886451816183042,
-7.18062506697956));
#38454=CARTESIAN_POINT('Ctrl Pts',(91.300211402431,2.64548140559999,-6.71182692763033));
#38455=CARTESIAN_POINT('Ctrl Pts',(91.4325524720591,6.54011662097128,-3.95774279675006));
#38456=CARTESIAN_POINT('Ctrl Pts',(91.5979788090942,7.82791073605462,2.43061730121419));
#38457=CARTESIAN_POINT('Ctrl Pts',(91.7964904135364,2.19141005279209,7.89800281555184));
#38458=CARTESIAN_POINT('Ctrl Pts',(91.9950020179783,-5.4451778386233,6.12623577735211));
#38459=CARTESIAN_POINT('Ctrl Pts',(92.1935136224206,-8.09846962411599,-1.26446696432582));
#38460=CARTESIAN_POINT('Ctrl Pts',(92.3589399594556,-4.12931971582869,-6.43316190885945));
#38461=CARTESIAN_POINT('Ctrl Pts',(92.4912810290837,0.580120396574044,-7.19101195238317));
#38462=CARTESIAN_POINT('Ctrl Pts',(92.5905368313047,3.95765727397703,-6.05674186974201));
#38463=CARTESIAN_POINT('Ctrl Pts',(92.6897926335259,6.35277235243675,-3.41898757119045));
#38464=CARTESIAN_POINT('Ctrl Pts',(92.8221337031538,7.54988327981452,1.19838054152583));
#38465=CARTESIAN_POINT('Ctrl Pts',(92.987560040189,4.41013951775851,6.9090344036273));
#38466=CARTESIAN_POINT('Ctrl Pts',(93.1860716446311,-3.42395764764996,7.44696183158223));
#38467=CARTESIAN_POINT('Ctrl Pts',(93.3845832490732,-8.11321888126058,1.16464839273495));
#38468=CARTESIAN_POINT('Ctrl Pts',(93.5830948535153,-5.36948445522538,-6.19295758436106));
#38469=CARTESIAN_POINT('Ctrl Pts',(93.7485211905504,0.998295723954193,-7.57893522261972));
#38470=CARTESIAN_POINT('Ctrl Pts',(93.8808622601784,5.08453351976072,-5.11807692988962));
#38471=CARTESIAN_POINT('Ctrl Pts',(93.9801180623996,6.93219161979444,-2.07168832631786));
#38472=CARTESIAN_POINT('Ctrl Pts',(94.0793738646205,7.05904983992973,1.48896203149283));
#38473=CARTESIAN_POINT('Ctrl Pts',(94.2117149342488,4.99312809870757,5.78839574070638));
#38474=CARTESIAN_POINT('Ctrl Pts',(94.3771412712837,-1.09095647846726,8.12366302345754));
#38475=CARTESIAN_POINT('Ctrl Pts',(94.5756528757259,-7.42186726605041,3.47801851333087));
#38476=CARTESIAN_POINT('Ctrl Pts',(94.7741644801679,-6.94862155587487,-4.34711225610455));
#38477=CARTESIAN_POINT('Ctrl Pts',(94.9726760846102,-0.103985426572741,
-8.19593033082037));
#38478=CARTESIAN_POINT('Ctrl Pts',(95.1381024216451,5.65432195232088,-5.14446272419511));
#38479=CARTESIAN_POINT('Ctrl Pts',(95.2704434912733,7.18704198136562,-0.627391530009471));
#38480=CARTESIAN_POINT('Ctrl Pts',(95.3696992934942,6.63199814606807,2.89201897737531));
#38481=CARTESIAN_POINT('Ctrl Pts',(95.4689550957155,4.43067240756226,5.69353445503804));
#38482=CARTESIAN_POINT('Ctrl Pts',(95.6012961653433,0.0776476560697105,
7.64400577594225));
#38483=CARTESIAN_POINT('Ctrl Pts',(95.7667225023786,-6.07669085085267,5.50071952200477));
#38484=CARTESIAN_POINT('Ctrl Pts',(95.9652341068207,-7.91372907993021,-2.13392093185527));
#38485=CARTESIAN_POINT('Ctrl Pts',(96.1637457112627,-2.50153500276373,-7.805321846272));
#38486=CARTESIAN_POINT('Ctrl Pts',(96.3622573157049,5.21063572505351,-6.32719229179871));
#38487=CARTESIAN_POINT('Ctrl Pts',(96.52768365274,7.63927871038486,-0.279775349507908));
#38488=CARTESIAN_POINT('Ctrl Pts',(96.6600247223681,5.89443276483208,4.1596700535876));
#38489=CARTESIAN_POINT('Ctrl Pts',(96.759280524589,3.1988865391963,6.48955299572309));
#38490=CARTESIAN_POINT('Ctrl Pts',(96.8585363268103,-0.290729422875887,
7.20851364544127));
#38491=CARTESIAN_POINT('Ctrl Pts',(96.9908773964381,-4.87451309683684,5.88863104039446));
#38492=CARTESIAN_POINT('Ctrl Pts',(97.1563037334734,-8.19183109205004,0.279267463058967));
#38493=CARTESIAN_POINT('Ctrl Pts',(97.3548153379154,-4.66719037118441,-6.73780828853616));
#38494=CARTESIAN_POINT('Ctrl Pts',(97.5533269423575,3.12726243117806,-7.57634187325818));
#38495=CARTESIAN_POINT('Ctrl Pts',(97.7518385467997,8.06378225188477,-1.46952466831598));
#38496=CARTESIAN_POINT('Ctrl Pts',(97.9172648838347,6.01548373649835,4.71707630604539));
#38497=CARTESIAN_POINT('Ctrl Pts',(98.0496059534629,1.81732709838692,6.98172720688136));
#38498=CARTESIAN_POINT('Ctrl Pts',(98.1488617556837,-1.74536084060413,7.02145915825447));
#38499=CARTESIAN_POINT('Ctrl Pts',(98.2481175579051,-4.87479233060809,5.31823206594859));
#38500=CARTESIAN_POINT('Ctrl Pts',(98.3804586275328,-7.52398163919293,1.35150055649951));
#38501=CARTESIAN_POINT('Ctrl Pts',(98.5458849645683,-6.43719700480271,-5.07410895408839));
#38502=CARTESIAN_POINT('Ctrl Pts',(98.7443965690101,0.784102473898442,-8.1587934037068));
#38503=CARTESIAN_POINT('Ctrl Pts',(98.9429081734525,7.27875891268348,-3.76834117152016));
#38504=CARTESIAN_POINT('Ctrl Pts',(99.1414197778943,7.10764399270585,4.08233803469939));
#38505=CARTESIAN_POINT('Ctrl Pts',(99.3068461149296,1.55000852346872,7.4856079938977));
#38506=CARTESIAN_POINT('Ctrl Pts',(99.4391871845575,-3.11827353367708,6.50565621155993));
#38507=CARTESIAN_POINT('Ctrl Pts',(99.5384429867787,-5.86510970487799,4.23646802474608));
#38508=CARTESIAN_POINT('Ctrl Pts',(99.6376987889998,-7.15603111934792,0.915647963337127));
#38509=CARTESIAN_POINT('Ctrl Pts',(99.7700398586277,-6.61916412903343,-3.82407108904214));
#38510=CARTESIAN_POINT('Ctrl Pts',(99.935466195663,-1.64166773351012,-8.03050521507537));
#38511=CARTESIAN_POINT('Ctrl Pts',(100.133977800105,5.86498977835619,-5.72561100614777));
#38512=CARTESIAN_POINT('Ctrl Pts',(100.332489404547,7.9918111603258,1.81980242653843));
#38513=CARTESIAN_POINT('Ctrl Pts',(100.531001008989,2.7938952127985,7.70572751247425));
#38514=CARTESIAN_POINT('Ctrl Pts',(100.696427346024,-3.64768188364758,6.71798112060759));
#38515=CARTESIAN_POINT('Ctrl Pts',(100.828768415652,-6.58081951726305,2.95635029302163));
#38516=CARTESIAN_POINT('Ctrl Pts',(100.928024217873,-7.21421416567094,-0.549806463023575));
#38517=CARTESIAN_POINT('Ctrl Pts',(101.027280020094,-6.05680158445754,-3.91948301952586));
#38518=CARTESIAN_POINT('Ctrl Pts',(101.159621089723,-2.58749120224389,-7.19317334279116));
#38519=CARTESIAN_POINT('Ctrl Pts',(101.325047426758,3.92937602039146,-7.19333657261869));
#38520=CARTESIAN_POINT('Ctrl Pts',(101.5235590312,8.17528933193856,-0.587682595483952));
#38521=CARTESIAN_POINT('Ctrl Pts',(101.722070635642,4.92957735549824,6.54828172806438));
#38522=CARTESIAN_POINT('Ctrl Pts',(101.920582240084,-2.83967374520597,7.68897522283621));
#38523=CARTESIAN_POINT('Ctrl Pts',(102.086008577119,-7.12222815448253,2.77681824695588));
#38524=CARTESIAN_POINT('Ctrl Pts',(102.218349646747,-6.93462386032044,-1.98951865779466));
#38525=CARTESIAN_POINT('Ctrl Pts',(102.317605448968,-5.15536496329487,-5.07635551061814));
#38526=CARTESIAN_POINT('Ctrl Pts',(102.416861251189,-2.09637349448938,-6.90307255832048));
#38527=CARTESIAN_POINT('Ctrl Pts',(102.549202320817,2.66649782420712,-7.16426149820347));
#38528=CARTESIAN_POINT('Ctrl Pts',(102.714628657852,7.64420493298944,-2.9580767229826));
#38529=CARTESIAN_POINT('Ctrl Pts',(102.913140262295,6.62362879029324,4.82786372449762));
#38530=CARTESIAN_POINT('Ctrl Pts',(103.111651866737,-0.461360701899278,
8.18339005527401));
#38531=CARTESIAN_POINT('Ctrl Pts',(103.310163471179,-7.13179700726309,4.03999485194223));
#38532=CARTESIAN_POINT('Ctrl Pts',(103.475589808214,-7.23227442967135,-2.47609774342373));
#38533=CARTESIAN_POINT('Ctrl Pts',(103.607930877842,-4.01255140726822,-5.99555033154707));
#38534=CARTESIAN_POINT('Ctrl Pts',(103.707186680063,-0.661150729031283,
-7.20486314150311));
#38535=CARTESIAN_POINT('Ctrl Pts',(103.806442482284,2.85436948853256,-6.6256899563683));
#38536=CARTESIAN_POINT('Ctrl Pts',(103.938783551912,6.66084847297623,-3.75099334572874));
#38537=CARTESIAN_POINT('Ctrl Pts',(104.104209888947,7.74795499416537,2.67456171423117));
#38538=CARTESIAN_POINT('Ctrl Pts',(104.302721493389,1.9430037514535,7.96275473222629));
#38539=CARTESIAN_POINT('Ctrl Pts',(104.501233097831,-5.63435459263867,5.95271155055995));
#38540=CARTESIAN_POINT('Ctrl Pts',(104.699744702274,-8.0549000022414,-1.51745606366842));
#38541=CARTESIAN_POINT('Ctrl Pts',(104.865171039309,-3.9258354757219,-6.55931927333122));
#38542=CARTESIAN_POINT('Ctrl Pts',(104.997512108937,0.805027465655755,-7.16931818748407));
#38543=CARTESIAN_POINT('Ctrl Pts',(105.096767911158,4.14538734270979,-5.92983449194886));
#38544=CARTESIAN_POINT('Ctrl Pts',(105.196023713379,6.45672458925401,-3.21836915162517));
#38545=CARTESIAN_POINT('Ctrl Pts',(105.328364783007,7.50865226061103,1.43422264037047));
#38546=CARTESIAN_POINT('Ctrl Pts',(105.493791120042,4.19161526203335,7.0437525372525));
#38547=CARTESIAN_POINT('Ctrl Pts',(105.692302724484,-3.65548518083639,7.33608561355083));
#38548=CARTESIAN_POINT('Ctrl Pts',(105.890814328926,-8.14571149277621,0.910006333379135));
#38549=CARTESIAN_POINT('Ctrl Pts',(106.089325933368,-5.17291411014704,-6.35806998076943));
#38550=CARTESIAN_POINT('Ctrl Pts',(106.254752270403,1.23514574214642,-7.54395470249355));
#38551=CARTESIAN_POINT('Ctrl Pts',(106.387093340031,5.24231601294789,-4.95634245627861));
#38552=CARTESIAN_POINT('Ctrl Pts',(106.486349142253,6.99366792025834,-1.8535826036882));
#38553=CARTESIAN_POINT('Ctrl Pts',(106.585604944474,7.00896003570272,1.70928496788058));
#38554=CARTESIAN_POINT('Ctrl Pts',(106.717946014102,4.80941096796698,5.94193284353501));
#38555=CARTESIAN_POINT('Ctrl Pts',(106.883372351137,-1.34481853620912,8.08548866178312));
#38556=CARTESIAN_POINT('Ctrl Pts',(107.081883955579,-7.52714557143349,3.24393493693221));
#38557=CARTESIAN_POINT('Ctrl Pts',(107.280395560021,-6.80907733581119,-4.56266073535736));
#38558=CARTESIAN_POINT('Ctrl Pts',(107.478907164463,0.152720294781448,-8.19500999416272));
#38559=CARTESIAN_POINT('Ctrl Pts',(107.644333501498,5.81266281373758,-4.96514640636761));
#38560=CARTESIAN_POINT('Ctrl Pts',(107.776674571126,7.2031480419312,-0.401630923051306));
#38561=CARTESIAN_POINT('Ctrl Pts',(107.875930373347,6.53821527098569,3.09744391522371));
#38562=CARTESIAN_POINT('Ctrl Pts',(107.975186175568,4.25013664469689,5.83104671267199));
#38563=CARTESIAN_POINT('Ctrl Pts',(108.107527245197,-0.161622961106447,
7.63932412864128));
#38564=CARTESIAN_POINT('Ctrl Pts',(108.272953582232,-6.24629954731418,5.3146339055588));
#38565=CARTESIAN_POINT('Ctrl Pts',(108.471465186674,-7.84228358717403,-2.39245798963491));
#38566=CARTESIAN_POINT('Ctrl Pts',(108.636891523709,-3.18936293666094,-6.9454835370673));
#38567=CARTESIAN_POINT('Ctrl Pts',(108.769232593337,1.58468972940029,-7.03937783508502));
#38568=CARTESIAN_POINT('Ctrl Pts',(108.868488395558,4.75883494996184,-5.44436182139488));
#38569=CARTESIAN_POINT('Ctrl Pts',(108.967744197779,6.7844801612218,-2.49148592609996));
#38570=CARTESIAN_POINT('Ctrl Pts',(109.033914732593,7.02701963797669,-0.129888228207554));
#38571=CARTESIAN_POINT('Ctrl Pts',(109.067,6.85892174064777,1.01078264511681));
#38572=CARTESIAN_POINT('Ctrl Pts',(30.7922774969106,-1.81203895677844,6.4452040820594));
#38573=CARTESIAN_POINT('Ctrl Pts',(30.8253627643176,-2.88390664196679,6.14385349992971));
#38574=CARTESIAN_POINT('Ctrl Pts',(30.8915332991317,-4.8703123697955,4.99930801783347));
#38575=CARTESIAN_POINT('Ctrl Pts',(30.9907891013527,-6.67525664671072,2.04974392354754));
#38576=CARTESIAN_POINT('Ctrl Pts',(31.0900449035737,-6.83047548939251,-1.37719959429219));
#38577=CARTESIAN_POINT('Ctrl Pts',(31.2223859732019,-4.8662109885332,-5.54901554722458));
#38578=CARTESIAN_POINT('Ctrl Pts',(31.3878123102369,0.981499149386936,-7.85666683476529));
#38579=CARTESIAN_POINT('Ctrl Pts',(31.5863239146791,7.14710812042464,-3.4122242090372));
#38580=CARTESIAN_POINT('Ctrl Pts',(31.7517502517141,6.79854969246659,2.86822284039177));
#38581=CARTESIAN_POINT('Ctrl Pts',(31.8840913213422,3.46566165096873,6.04498987921042));
#38582=CARTESIAN_POINT('Ctrl Pts',(31.9833471235633,0.153961023470463,6.98483577110846));
#38583=CARTESIAN_POINT('Ctrl Pts',(32.0826029257843,-3.19288929971824,6.19203320852766));
#38584=CARTESIAN_POINT('Ctrl Pts',(32.2149439954124,-6.66809958720304,3.16766408236977));
#38585=CARTESIAN_POINT('Ctrl Pts',(32.3803703324475,-7.28493555493229,-3.09507108051456));
#38586=CARTESIAN_POINT('Ctrl Pts',(32.5788819368896,-1.33895233039623,-7.80108067131974));
#38587=CARTESIAN_POINT('Ctrl Pts',(32.7773935413317,5.82636340729205,-5.35749892731368));
#38588=CARTESIAN_POINT('Ctrl Pts',(32.9759051457738,7.65819530642828,2.00095028754364));
#38589=CARTESIAN_POINT('Ctrl Pts',(33.1413314828089,3.34300536777016,6.58174892634051));
#38590=CARTESIAN_POINT('Ctrl Pts',(33.273672552437,-1.25536816334185,6.85276289884607));
#38591=CARTESIAN_POINT('Ctrl Pts',(33.372928354658,-4.39037706243106,5.43513071151949));
#38592=CARTESIAN_POINT('Ctrl Pts',(33.4721841568791,-6.43556040023512,2.66831418699039));
#38593=CARTESIAN_POINT('Ctrl Pts',(33.6045252265073,-7.13755440619835,-1.88421592210945));
#38594=CARTESIAN_POINT('Ctrl Pts',(33.7699515635422,-3.56661413217037,-7.06621698471055));
#38595=CARTESIAN_POINT('Ctrl Pts',(33.9684631679844,4.01254545034611,-6.82264596434217));
#38596=CARTESIAN_POINT('Ctrl Pts',(34.1669747724265,7.90816875735116,-0.331485828065288));
#38597=CARTESIAN_POINT('Ctrl Pts',(34.3654863768686,4.55785072533662,6.47133294229691));
#38598=CARTESIAN_POINT('Ctrl Pts',(34.5309127139037,-1.69479614673967,7.18488923320334));
#38599=CARTESIAN_POINT('Ctrl Pts',(34.6632537835318,-5.38196425847962,4.42388796338411));
#38600=CARTESIAN_POINT('Ctrl Pts',(34.7625095857528,-6.86148701022481,1.31759840225387));
#38601=CARTESIAN_POINT('Ctrl Pts',(34.8617653879739,-6.63776106705247,-2.11576276551648));
#38602=CARTESIAN_POINT('Ctrl Pts',(34.9941064576019,-4.2355184272481,-6.0461021388265));
#38603=CARTESIAN_POINT('Ctrl Pts',(35.1595327946371,1.83669728137531,-7.6992658814414));
#38604=CARTESIAN_POINT('Ctrl Pts',(35.3580443990791,7.46846773094147,-2.62126076137705));
#38605=CARTESIAN_POINT('Ctrl Pts',(35.5565560035213,6.2542393043315,4.85113481298777));
#38606=CARTESIAN_POINT('Ctrl Pts',(35.7550676079634,-0.695620042101597,
7.88468545833603));
#38607=CARTESIAN_POINT('Ctrl Pts',(35.9204939449985,-5.93197410466557,4.39393338519193));
#38608=CARTESIAN_POINT('Ctrl Pts',(36.0528350146266,-6.96615643498071,-0.0948085558509277));
#38609=CARTESIAN_POINT('Ctrl Pts',(36.1520908168476,-6.09126670585619,-3.42235873639071));
#38610=CARTESIAN_POINT('Ctrl Pts',(36.2513466190687,-3.70432255158069,-5.90036596931892));
#38611=CARTESIAN_POINT('Ctrl Pts',(36.3836876886967,0.667353267230231,-7.35184378166206));
#38612=CARTESIAN_POINT('Ctrl Pts',(36.5491140257318,6.37236282717805,-4.69522566233383));
#38613=CARTESIAN_POINT('Ctrl Pts',(36.7476256301739,7.39632868574868,2.81839319700334));
#38614=CARTESIAN_POINT('Ctrl Pts',(36.9461372346161,1.64584269422835,7.74210695265263));
#38615=CARTESIAN_POINT('Ctrl Pts',(37.1446488390582,-5.62048377641761,5.57335752850344));
#38616=CARTESIAN_POINT('Ctrl Pts',(37.3100751760933,-7.36692134135521,-0.472691573440474));
#38617=CARTESIAN_POINT('Ctrl Pts',(37.4424162457214,-5.25957598656419,-4.56871804551017));
#38618=CARTESIAN_POINT('Ctrl Pts',(37.5416720479423,-2.44356673040902,-6.54561311391665));
#38619=CARTESIAN_POINT('Ctrl Pts',(37.6409278501635,0.979016833964809,-6.89766990922517));
#38620=CARTESIAN_POINT('Ctrl Pts',(37.7732689197915,5.25497107745377,-5.18461631641446));
#38621=CARTESIAN_POINT('Ctrl Pts',(37.9386952568267,7.8977604870432,0.526812405708338));
#38622=CARTESIAN_POINT('Ctrl Pts',(38.1372068612687,3.8302061148084,6.92665426873328));
#38623=CARTESIAN_POINT('Ctrl Pts',(38.3357184657109,-3.74004062557482,6.9757518848886));
#38624=CARTESIAN_POINT('Ctrl Pts',(38.534230070153,-7.89026300224576,0.629207260686155));
#38625=CARTESIAN_POINT('Ctrl Pts',(38.6996564071881,-5.3217769150866,-5.11601972624796));
#38626=CARTESIAN_POINT('Ctrl Pts',(38.8319974768161,-1.06840181276754,-6.88439116438718));
#38627=CARTESIAN_POINT('Ctrl Pts',(38.9312532790372,2.35846024436991,-6.57675715522205));
#38628=CARTESIAN_POINT('Ctrl Pts',(39.0305090812582,5.19987424584941,-4.63655388895342));
#38629=CARTESIAN_POINT('Ctrl Pts',(39.1628501508863,7.36017049505773,-0.568205646741278));
#38630=CARTESIAN_POINT('Ctrl Pts',(39.3282764879214,5.69230109656122,5.49998729522135));
#38631=CARTESIAN_POINT('Ctrl Pts',(39.5267880923636,-1.54528399913325,7.76280333400891));
#38632=CARTESIAN_POINT('Ctrl Pts',(39.7252996968056,-7.35915006569954,2.91409137656859));
#38633=CARTESIAN_POINT('Ctrl Pts',(39.9238113012478,-6.43272694682871,-4.6121769316725));
#38634=CARTESIAN_POINT('Ctrl Pts',(40.0892376382828,-0.762655399166796,
-7.34256931294684));
#38635=CARTESIAN_POINT('Ctrl Pts',(40.2215787079109,3.62747928931603,-5.94791712647381));
#38636=CARTESIAN_POINT('Ctrl Pts',(40.320834510132,6.04636403890181,-3.50107859267866));
#38637=CARTESIAN_POINT('Ctrl Pts',(40.420090312353,6.96434069439297,-0.185156231974706));
#38638=CARTESIAN_POINT('Ctrl Pts',(40.5524313819811,5.98846731119182,4.31662213265117));
#38639=CARTESIAN_POINT('Ctrl Pts',(40.7178577190162,0.797831104453527,7.87499952700156));
#38640=CARTESIAN_POINT('Ctrl Pts',(40.9163693234583,-6.19079075736279,4.93184833901336));
#38641=CARTESIAN_POINT('Ctrl Pts',(41.1148809279004,-7.50183894936851,-2.52416929270096));
#38642=CARTESIAN_POINT('Ctrl Pts',(41.3133925323426,-1.93640733728171,-7.67479502303675));
#38643=CARTESIAN_POINT('Ctrl Pts',(41.4788188693776,4.15674018148683,-6.10053099630842));
#38644=CARTESIAN_POINT('Ctrl Pts',(41.6111599390057,6.60975984556038,-2.20168093097857));
#38645=CARTESIAN_POINT('Ctrl Pts',(41.7104157412267,6.87799991540007,1.22848954688046));
#38646=CARTESIAN_POINT('Ctrl Pts',(41.8096715434478,5.43889228374724,4.35370817391472));
#38647=CARTESIAN_POINT('Ctrl Pts',(41.9420126130758,1.78784629355005,7.16230221394951));
#38648=CARTESIAN_POINT('Ctrl Pts',(42.107438950111,-4.47352975512394,6.52990685626748));
#38649=CARTESIAN_POINT('Ctrl Pts',(42.3059505545531,-7.91180323874318,-0.228883708223626));
#38650=CARTESIAN_POINT('Ctrl Pts',(42.5044621589952,-4.1007018610194,-6.77002677155041));
#38651=CARTESIAN_POINT('Ctrl Pts',(42.7029737634372,3.47466006418408,-7.11188367873607));
#38652=CARTESIAN_POINT('Ctrl Pts',(42.8684001004724,7.11251538672242,-1.97663659961656));
#38653=CARTESIAN_POINT('Ctrl Pts',(43.0007411701004,6.46962751509898,2.58461679049164));
#38654=CARTESIAN_POINT('Ctrl Pts',(43.0999969723216,4.46050782471037,5.37772622478455));
#38655=CARTESIAN_POINT('Ctrl Pts',(43.1992527745425,1.34414215065186,6.83590564714421));
#38656=CARTESIAN_POINT('Ctrl Pts',(43.3315938441707,-3.25734312549581,6.62455154226247));
#38657=CARTESIAN_POINT('Ctrl Pts',(43.4970201812057,-7.63162064985655,2.10012339594401));
#38658=CARTESIAN_POINT('Ctrl Pts',(43.6955317856479,-5.89532495390081,-5.28149239594187));
#38659=CARTESIAN_POINT('Ctrl Pts',(43.89404339009,1.23758341948163,-7.81776218110407));
#38660=CARTESIAN_POINT('Ctrl Pts',(44.092554994532,7.2443178509545,-3.18935901018531));
#38661=CARTESIAN_POINT('Ctrl Pts',(44.2579813315672,6.70837885245484,3.08100966328303));
#38662=CARTESIAN_POINT('Ctrl Pts',(44.3903224011952,3.27328001232696,6.14995626803296));
#38663=CARTESIAN_POINT('Ctrl Pts',(44.4895782034164,-0.0641027450996106,
6.98655567795094));
#38664=CARTESIAN_POINT('Ctrl Pts',(44.5888340056373,-3.38557307509794,6.08886024564441));
#38665=CARTESIAN_POINT('Ctrl Pts',(44.7211750752655,-6.76378221334741,2.95740047063501));
#38666=CARTESIAN_POINT('Ctrl Pts',(44.8866014123005,-7.18457743679441,-3.32174638950854));
#38667=CARTESIAN_POINT('Ctrl Pts',(45.0851130167426,-1.09392875411456,-7.83915417129927));
#38668=CARTESIAN_POINT('Ctrl Pts',(45.2836246211847,5.99124134473033,-5.17243128419034));
#38669=CARTESIAN_POINT('Ctrl Pts',(45.4821362256269,7.59180116516734,2.23980068088031));
#38670=CARTESIAN_POINT('Ctrl Pts',(45.647562562662,3.13524237458443,6.68320451773826));
#38671=CARTESIAN_POINT('Ctrl Pts',(45.7799036322901,-1.46934631616532,6.81009144879777));
#38672=CARTESIAN_POINT('Ctrl Pts',(45.8791594345111,-4.55843154340064,5.29497604028271));
#38673=CARTESIAN_POINT('Ctrl Pts',(45.9784152367321,-6.51596287215306,2.46547196020152));
#38674=CARTESIAN_POINT('Ctrl Pts',(46.1107563063602,-7.075049125615,-2.10680973119107));
#38675=CARTESIAN_POINT('Ctrl Pts',(46.2761826433953,-3.34358078240567,-7.17444210883576));
#38676=CARTESIAN_POINT('Ctrl Pts',(46.4746942478375,4.22423315559067,-6.69364418591888));
#38677=CARTESIAN_POINT('Ctrl Pts',(46.6732058522795,7.91467099856683,-0.0836733226452872));
#38678=CARTESIAN_POINT('Ctrl Pts',(46.8717174567217,4.35296086924962,6.61089129333479));
#38679=CARTESIAN_POINT('Ctrl Pts',(47.0371437937567,-1.91896473551536,7.12829164086005));
#38680=CARTESIAN_POINT('Ctrl Pts',(47.1694848633849,-5.51786181766442,4.25317823503533));
#38681=CARTESIAN_POINT('Ctrl Pts',(47.2687406656058,-6.89938325586998,1.10207989350079));
#38682=CARTESIAN_POINT('Ctrl Pts',(47.367996467827,-6.56824893825758,-2.32259123026316));
#38683=CARTESIAN_POINT('Ctrl Pts',(47.5003375374549,-4.04410314663289,-6.17577502121804));
#38684=CARTESIAN_POINT('Ctrl Pts',(47.6657638744901,2.07690438089424,-7.63797225801001));
#38685=CARTESIAN_POINT('Ctrl Pts',(47.8642754789321,7.54689139350594,-2.38609482944481));
#38686=CARTESIAN_POINT('Ctrl Pts',(48.0627870833744,6.09925517278121,5.04461143972248));
#38687=CARTESIAN_POINT('Ctrl Pts',(48.2612986878164,-0.942193336862589,
7.85903452960222));
#38688=CARTESIAN_POINT('Ctrl Pts',(48.4267250248516,-6.06666383937774,4.20601441192175));
#38689=CARTESIAN_POINT('Ctrl Pts',(48.5590660944796,-6.9597708388828,-0.312912141109297));
#38690=CARTESIAN_POINT('Ctrl Pts',(48.6583218967007,-5.9811056329619,-3.61143251499863));
#38691=CARTESIAN_POINT('Ctrl Pts',(48.7575776989217,-3.51773163372495,-6.01347555835291));
#38692=CARTESIAN_POINT('Ctrl Pts',(48.8899187685498,0.897254114340819,-7.32733938258665));
#38693=CARTESIAN_POINT('Ctrl Pts',(49.0553451055848,6.51627174946588,-4.49336783589115));
#38694=CARTESIAN_POINT('Ctrl Pts',(49.253856710027,7.30444114151449,3.04863212779555));
#38695=CARTESIAN_POINT('Ctrl Pts',(49.452368314469,1.40258595870646,7.78985050363078));
#38696=CARTESIAN_POINT('Ctrl Pts',(49.6508799189113,-5.79226077953301,5.39461463715364));
#38697=CARTESIAN_POINT('Ctrl Pts',(49.8163062559462,-7.3485055151358,-0.703160058113078));
#38698=CARTESIAN_POINT('Ctrl Pts',(49.9486473255744,-5.11392377461454,-4.73118460485842));
#38699=CARTESIAN_POINT('Ctrl Pts',(50.0479031277955,-2.23738779112476,-6.61892478240717));
#38700=CARTESIAN_POINT('Ctrl Pts',(50.1471589300164,1.19454204951979,-6.86362829921216));
#38701=CARTESIAN_POINT('Ctrl Pts',(50.2794999996447,5.41475364451525,-5.01751037293554));
#38702=CARTESIAN_POINT('Ctrl Pts',(50.4449263366795,7.8773894752044,0.773877947383871));
#38703=CARTESIAN_POINT('Ctrl Pts',(50.6434379411219,3.61141451710502,7.04320263985923));
#38704=CARTESIAN_POINT('Ctrl Pts',(50.8419495455637,-3.95665686991791,6.85520857846125));
#38705=CARTESIAN_POINT('Ctrl Pts',(51.0404611500061,-7.90609723594123,0.381809530199271));
#38706=CARTESIAN_POINT('Ctrl Pts',(51.205887487041,-5.15895505946872,-5.28016572350612));
#38707=CARTESIAN_POINT('Ctrl Pts',(51.3382285566692,-0.852288259845684,
-6.91447242094047));
#38708=CARTESIAN_POINT('Ctrl Pts',(51.4374843588902,2.56325929395234,-6.49967469916801));
#38709=CARTESIAN_POINT('Ctrl Pts',(51.5367401611113,5.34252087541995,-4.47144214247698));
#38710=CARTESIAN_POINT('Ctrl Pts',(51.6690812307394,7.37435440786423,-0.337438054345343));
#38711=CARTESIAN_POINT('Ctrl Pts',(51.8345075677744,5.51727330051624,5.67554819809671));
#38712=CARTESIAN_POINT('Ctrl Pts',(52.0330191722166,-1.78762374629298,7.71060435907371));
#38713=CARTESIAN_POINT('Ctrl Pts',(52.2315307766586,-7.44679753937642,2.682205183802));
#38714=CARTESIAN_POINT('Ctrl Pts',(52.4300423811009,-6.28513840933588,-4.81136022315926));
#38715=CARTESIAN_POINT('Ctrl Pts',(52.5954687181358,-0.532343630937353,
-7.36285118903727));
#38716=CARTESIAN_POINT('Ctrl Pts',(52.727809787764,3.81196337228751,-5.83140286604824));
#38717=CARTESIAN_POINT('Ctrl Pts',(52.8270655899849,6.15303729476447,-3.31001532508164));
#38718=CARTESIAN_POINT('Ctrl Pts',(52.9263213922061,6.96672328301192,0.0330278027845019));
#38719=CARTESIAN_POINT('Ctrl Pts',(53.0586624618341,5.85035217015766,4.50203807829726));
#38720=CARTESIAN_POINT('Ctrl Pts',(53.2240887988693,0.550828657694646,7.89612182095554));
#38721=CARTESIAN_POINT('Ctrl Pts',(53.4226004033113,-6.34219873834294,4.7355605163315));
#38722=CARTESIAN_POINT('Ctrl Pts',(53.6211120077535,-7.41911348525517,-2.75785665569876));
#38723=CARTESIAN_POINT('Ctrl Pts',(53.8196236121955,-1.69511601270984,-7.73167082362948));
#38724=CARTESIAN_POINT('Ctrl Pts',(53.9850499492307,4.34574389539973,-5.9673677085381));
#38725=CARTESIAN_POINT('Ctrl Pts',(54.1173910188587,6.67546522902976,-1.99361182626703));
#38726=CARTESIAN_POINT('Ctrl Pts',(54.2166468210798,6.83615553932873,1.44327642714178));
#38727=CARTESIAN_POINT('Ctrl Pts',(54.3159026233008,5.29988531012766,4.52189560221267));
#38728=CARTESIAN_POINT('Ctrl Pts',(54.448243692929,1.56267690427941,7.21477707667661));
#38729=CARTESIAN_POINT('Ctrl Pts',(54.6136700299639,-4.6758243042398,6.38661248999724));
#38730=CARTESIAN_POINT('Ctrl Pts',(54.8121816344062,-7.90075518609565,-0.476535129722538));
#38731=CARTESIAN_POINT('Ctrl Pts',(55.0106932388481,-3.8866824969691,-6.89512272611814));
#38732=CARTESIAN_POINT('Ctrl Pts',(55.2092048432904,3.69566952905561,-6.99958418432969));
#38733=CARTESIAN_POINT('Ctrl Pts',(55.3746311803254,7.17092676886464,-1.75293372632495));
#38734=CARTESIAN_POINT('Ctrl Pts',(55.5069722499535,6.3855153503238,2.78595008006179));
#38735=CARTESIAN_POINT('Ctrl Pts',(55.6062280521746,4.28991286151973,5.51477261939286));
#38736=CARTESIAN_POINT('Ctrl Pts',(55.7054838543956,1.12941171702959,6.87464568623383));
#38737=CARTESIAN_POINT('Ctrl Pts',(55.8378249240237,-3.46319802659206,6.51929649593543));
#38738=CARTESIAN_POINT('Ctrl Pts',(56.0032512610588,-7.69364450906023,1.86010381154267));
#38739=CARTESIAN_POINT('Ctrl Pts',(56.2017628655009,-5.72703990474126,-5.46351829593155));
#38740=CARTESIAN_POINT('Ctrl Pts',(56.400274469943,1.48179515543616,-7.77517211113707));
#38741=CARTESIAN_POINT('Ctrl Pts',(56.5987860743851,7.34064184429667,-2.96093386202206));
#38742=CARTESIAN_POINT('Ctrl Pts',(56.7642124114202,6.60860469874742,3.28957615947717));
#38743=CARTESIAN_POINT('Ctrl Pts',(56.8965534810483,3.07908440665131,6.24944504372459));
#38744=CARTESIAN_POINT('Ctrl Pts',(56.9958092832693,-0.282860206898158,
6.98112165102364));
#38745=CARTESIAN_POINT('Ctrl Pts',(57.0950650854904,-3.57458953547651,5.97985232181189));
#38746=CARTESIAN_POINT('Ctrl Pts',(57.2274061551185,-6.85307794401281,2.74413739936472));
#38747=CARTESIAN_POINT('Ctrl Pts',(57.3928324921536,-7.07703088842817,-3.54510730807145));
#38748=CARTESIAN_POINT('Ctrl Pts',(57.5913440965957,-0.847903606728639,
-7.86956655186127));
#38749=CARTESIAN_POINT('Ctrl Pts',(57.7898557010378,6.15028122011372,-4.98227449605031));
#38750=CARTESIAN_POINT('Ctrl Pts',(57.9883673054799,7.51793678140744,2.47644474444095));
#38751=CARTESIAN_POINT('Ctrl Pts',(58.153793642515,2.92441542669665,6.77810901250529));
#38752=CARTESIAN_POINT('Ctrl Pts',(58.2861347121431,-1.68188846520317,6.76073777989012));
#38753=CARTESIAN_POINT('Ctrl Pts',(58.3853905143641,-4.72201172539709,5.14962859517563));
#38754=CARTESIAN_POINT('Ctrl Pts',(58.4846463165852,-6.58997506047582,2.26021079550644));
#38755=CARTESIAN_POINT('Ctrl Pts',(58.6169873862132,-7.0056028915162,-2.32733656777153));
#38756=CARTESIAN_POINT('Ctrl Pts',(58.7824137232484,-3.11726820308623,-7.27562993640659));
#38757=CARTESIAN_POINT('Ctrl Pts',(58.9809253276904,4.4317775235007,-6.55807641177433));
#38758=CARTESIAN_POINT('Ctrl Pts',(59.1794369321326,7.91340948250359,0.164221200519121));
#38759=CARTESIAN_POINT('Ctrl Pts',(59.3779485365746,4.14380122237507,6.74396496513376));
#38760=CARTESIAN_POINT('Ctrl Pts',(59.5433748736098,-2.1412510287548,7.06470179166561));
#38761=CARTESIAN_POINT('Ctrl Pts',(59.6757159432378,-5.64834680998629,4.07829651348879));
#38762=CARTESIAN_POINT('Ctrl Pts',(59.7749717454589,-6.93051181221684,0.885480335050289));
#38763=CARTESIAN_POINT('Ctrl Pts',(59.87422754768,-6.49229391850386,-2.52714143125686));
#38764=CARTESIAN_POINT('Ctrl Pts',(60.006568617308,-3.84872095303324,-6.2993900021343));
#38765=CARTESIAN_POINT('Ctrl Pts',(60.1719949543432,2.31507421829155,-7.56918644144204));
#38766=CARTESIAN_POINT('Ctrl Pts',(60.3705065587852,7.61791220518773,-2.14858834459484));
#38767=CARTESIAN_POINT('Ctrl Pts',(60.5690181632275,5.93828819827106,5.23313973774365));
#38768=CARTESIAN_POINT('Ctrl Pts',(60.7675297676693,-1.18784242152082,7.82567456537414));
#38769=CARTESIAN_POINT('Ctrl Pts',(60.9329561047047,-6.19540269969449,4.01396970117181));
#38770=CARTESIAN_POINT('Ctrl Pts',(61.0652971743325,-6.94655830765724,-0.53070878656308));
#38771=CARTESIAN_POINT('Ctrl Pts',(61.1645529765538,-5.86507761102045,-3.79696378962774));
#38772=CARTESIAN_POINT('Ctrl Pts',(61.2638087787747,-3.32769012441271,-6.12068644628227));
#38773=CARTESIAN_POINT('Ctrl Pts',(61.3961498484029,1.12627483252932,-7.29564749524797));
#38774=CARTESIAN_POINT('Ctrl Pts',(61.5615761854378,6.65378877091549,-4.28710240296953));
#38775=CARTESIAN_POINT('Ctrl Pts',(61.7600877898801,7.20538857022683,3.27588061328884));
#38776=CARTESIAN_POINT('Ctrl Pts',(61.9585993943221,1.15795340727137,7.82995288281261));
#38777=CARTESIAN_POINT('Ctrl Pts',(62.1571109987642,-5.95835607416243,5.21058009390514));
#38778=CARTESIAN_POINT('Ctrl Pts',(62.3225373357994,-7.32288143850781,-0.932938803387027));
#38779=CARTESIAN_POINT('Ctrl Pts',(62.4548784054274,-4.96325524430359,-4.8890102799759));
#38780=CARTESIAN_POINT('Ctrl Pts',(62.5541342076486,-2.02901416729863,-6.68574385629147));
#38781=CARTESIAN_POINT('Ctrl Pts',(62.6533900098694,1.40889552230351,-6.82285406153834));
#38782=CARTESIAN_POINT('Ctrl Pts',(62.7857310794977,5.56922480504733,-4.84548268433111));
#38783=CARTESIAN_POINT('Ctrl Pts',(62.9511574165326,7.84929142338568,1.02018438150764));
#38784=CARTESIAN_POINT('Ctrl Pts',(63.1496690209748,3.38908043309366,7.152842236377));
#38785=CARTESIAN_POINT('Ctrl Pts',(63.348180625417,-4.16939197496766,6.72794090339327));
#38786=CARTESIAN_POINT('Ctrl Pts',(63.546692229859,-7.91417626981825,0.134037277478446));
#38787=CARTESIAN_POINT('Ctrl Pts',(63.7121185668942,-4.99107271368159,-5.43913233338277));
#38788=CARTESIAN_POINT('Ctrl Pts',(63.8444596365222,-0.635338685615254,
-6.93777117613269));
#38789=CARTESIAN_POINT('Ctrl Pts',(63.9437154387432,2.76554400714119,-6.41621662255914));
#38790=CARTESIAN_POINT('Ctrl Pts',(64.0429712409643,5.47992695258048,-4.30194429673351));
#38791=CARTESIAN_POINT('Ctrl Pts',(64.1753123105923,7.38130471472616,-0.106339464308261));
#38792=CARTESIAN_POINT('Ctrl Pts',(64.3407386476275,5.3368335349973,5.84554187746859));
#38793=CARTESIAN_POINT('Ctrl Pts',(64.5392502520696,-2.02820998866499,7.6508419459786));
#38794=CARTESIAN_POINT('Ctrl Pts',(64.7377618565118,-7.52714034664233,2.44768797897928));
#38795=CARTESIAN_POINT('Ctrl Pts',(64.9362734609538,-6.13138469289272,-5.00582398504777));
#38796=CARTESIAN_POINT('Ctrl Pts',(65.1016997979889,-0.301509679500262,
-7.37591074284501));
#38797=CARTESIAN_POINT('Ctrl Pts',(65.234040867617,3.99270824781552,-5.70916850213125));
#38798=CARTESIAN_POINT('Ctrl Pts',(65.333296669838,6.25367495147746,-3.11570521778876));
#38799=CARTESIAN_POINT('Ctrl Pts',(65.4325524720591,6.96227211668874,0.251179440093837));
#38800=CARTESIAN_POINT('Ctrl Pts',(65.5648935416872,5.70649833797061,4.68303791274987));
#38801=CARTESIAN_POINT('Ctrl Pts',(65.7303198787222,0.303285895553221,7.90949870001355));
#38802=CARTESIAN_POINT('Ctrl Pts',(65.9288314831644,-6.48738556918477,4.53462751719283));
#38803=CARTESIAN_POINT('Ctrl Pts',(66.1273430876064,-7.32911051026348,-2.98883879937283));
#38804=CARTESIAN_POINT('Ctrl Pts',(66.3258546920486,-1.45216192573285,-7.78096252107479));
#38805=CARTESIAN_POINT('Ctrl Pts',(66.4912810290837,4.53048480966573,-5.8283509485403));
#38806=CARTESIAN_POINT('Ctrl Pts',(66.6236220987118,6.73462255592388,-1.78358715873934));
#38807=CARTESIAN_POINT('Ctrl Pts',(66.7228779009328,6.78760548545835,1.65664757441715));
#38808=CARTESIAN_POINT('Ctrl Pts',(66.822133703154,5.15567960323104,4.68564744671614));
#38809=CARTESIAN_POINT('Ctrl Pts',(66.9544747727818,1.33597466947468,7.260174852171));
#38810=CARTESIAN_POINT('Ctrl Pts',(67.1199011098171,-4.87353228461882,6.23705343373919));
#38811=CARTESIAN_POINT('Ctrl Pts',(67.3184127142591,-7.88195715407007,-0.723719155071791));
#38812=CARTESIAN_POINT('Ctrl Pts',(67.5169243187013,-3.66885066862576,-7.01345507920435));
#38813=CARTESIAN_POINT('Ctrl Pts',(67.7154359231434,3.91305393206027,-6.88041886003763));
#38814=CARTESIAN_POINT('Ctrl Pts',(67.8808622601784,7.22230396464096,-1.52751109708982));
#38815=CARTESIAN_POINT('Ctrl Pts',(68.0132033298065,6.29513972075098,2.98455020269193));
#38816=CARTESIAN_POINT('Ctrl Pts',(68.1124591320276,4.11510948079485,5.64641034950249));
#38817=CARTESIAN_POINT('Ctrl Pts',(68.2117149342486,0.913574134491054,6.90664071797512));
#38818=CARTESIAN_POINT('Ctrl Pts',(68.3440560038768,-3.66565735573255,6.40764997957445));
#38819=CARTESIAN_POINT('Ctrl Pts',(68.5094823409118,-7.74811845347451,1.61825269811276));
#38820=CARTESIAN_POINT('Ctrl Pts',(68.7079939453539,-5.55314230167276,-5.64017343059075));
#38821=CARTESIAN_POINT('Ctrl Pts',(68.906505549796,1.72456291095644,-7.72497648317235));
#38822=CARTESIAN_POINT('Ctrl Pts',(69.1050171542383,7.42974649891666,-2.72956244906754));
#38823=CARTESIAN_POINT('Ctrl Pts',(69.2704434912731,6.50238112060189,3.494842318281));
#38824=CARTESIAN_POINT('Ctrl Pts',(69.4027845609014,2.88182229246086,6.34290645397399));
#38825=CARTESIAN_POINT('Ctrl Pts',(69.5020403631223,-0.501239314243825,
6.96861520670999));
#38826=CARTESIAN_POINT('Ctrl Pts',(69.6012961653434,-3.76028584749399,5.8653931038265));
#38827=CARTESIAN_POINT('Ctrl Pts',(69.7336372349715,-6.93524907719399,2.52728720876738));
#38828=CARTESIAN_POINT('Ctrl Pts',(69.8990635720067,-6.96336228722064,-3.76316618635394));
#38829=CARTESIAN_POINT('Ctrl Pts',(70.0975751764487,-0.599684643835917,
-7.89529022500933));
#38830=CARTESIAN_POINT('Ctrl Pts',(70.2960867808908,6.30079599638089,-4.78168947323583));
#38831=CARTESIAN_POINT('Ctrl Pts',(70.4945983853329,7.4414924699285,2.70003404851807));
#38832=CARTESIAN_POINT('Ctrl Pts',(70.6931099897751,1.75530894462229,7.71973735780468));
#38833=CARTESIAN_POINT('Ctrl Pts',(70.8585363268101,-4.30523581206144,5.99894314542976));
#38834=CARTESIAN_POINT('Ctrl Pts',(70.9908773964383,-6.65241429240827,2.04583611782808));
#38835=CARTESIAN_POINT('Ctrl Pts',(71.1232184660662,-6.93093605511931,-2.53987632804942));
#38836=CARTESIAN_POINT('Ctrl Pts',(71.2886448031015,-2.89169548793886,-7.37429860539061));
#38837=CARTESIAN_POINT('Ctrl Pts',(71.4871564075434,4.6447284051371,-6.411379345178));
#38838=CARTESIAN_POINT('Ctrl Pts',(71.6525827445787,7.34317100468254,-0.732288897783634));
#38839=CARTESIAN_POINT('Ctrl Pts',(71.7849238142065,5.93364342986877,3.65309768259248));
#38840=CARTESIAN_POINT('Ctrl Pts',(71.8841796164278,3.47471803823491,6.06097352117865));
#38841=CARTESIAN_POINT('Ctrl Pts',(71.9834354186487,0.155865321197622,6.96515979860947));
#38842=CARTESIAN_POINT('Ctrl Pts',(72.1157764882769,-4.34223294767585,5.97000820865479));
#38843=CARTESIAN_POINT('Ctrl Pts',(72.2812028253119,-7.87819756409372,0.764410097337301));
#38844=CARTESIAN_POINT('Ctrl Pts',(72.4797144297541,-4.90556651422554,-6.21170485827554));
#38845=CARTESIAN_POINT('Ctrl Pts',(72.6782260341962,2.55604705852035,-7.49103801052975));
#38846=CARTESIAN_POINT('Ctrl Pts',(72.8767376386383,7.68293167045214,-1.90379411267946));
#38847=CARTESIAN_POINT('Ctrl Pts',(73.0421639756733,6.08282805842319,4.18262061011101));
#38848=CARTESIAN_POINT('Ctrl Pts',(73.1745050453015,2.17357859296375,6.61905138996127));
#38849=CARTESIAN_POINT('Ctrl Pts',(73.2737608475224,-1.25769345075426,6.87272008061714));
#38850=CARTESIAN_POINT('Ctrl Pts',(73.3730166497437,-4.37677417992924,5.42034849327425));
#38851=CARTESIAN_POINT('Ctrl Pts',(73.5053577193714,-7.16983148085324,1.75740528550872));
#38852=CARTESIAN_POINT('Ctrl Pts',(73.670784056407,-6.51084504293545,-4.50122828872999));
#38853=CARTESIAN_POINT('Ctrl Pts',(73.8692956608486,0.262490856564827,-7.9107594913457));
#38854=CARTESIAN_POINT('Ctrl Pts',(74.0678072652911,6.78738515894909,-4.07190613494002));
#38855=CARTESIAN_POINT('Ctrl Pts',(74.266318869733,7.097059387601,3.50483969846582));
#38856=CARTESIAN_POINT('Ctrl Pts',(74.4317452067681,1.94640508439703,7.12084786428718));
#38857=CARTESIAN_POINT('Ctrl Pts',(74.5640862763962,-2.61207613861328,6.45858981248953));
#38858=CARTESIAN_POINT('Ctrl Pts',(74.6633420786172,-5.39662574857546,4.43762323844));
#38859=CARTESIAN_POINT('Ctrl Pts',(74.7625978808384,-6.84155382034101,1.31509140621307));
#38860=CARTESIAN_POINT('Ctrl Pts',(74.8949389504664,-6.61065472827709,-3.28545453224419));
#38861=CARTESIAN_POINT('Ctrl Pts',(75.0603652875015,-2.06768566612684,-7.64047302147642));
#38862=CARTESIAN_POINT('Ctrl Pts',(75.2588768919436,5.30648781615955,-5.87283622208682));
#38863=CARTESIAN_POINT('Ctrl Pts',(75.4573884963857,7.81243444661612,1.27078175373805));
#38864=CARTESIAN_POINT('Ctrl Pts',(75.6559001008279,3.15855669885345,7.25780074116703));
#38865=CARTESIAN_POINT('Ctrl Pts',(75.8213264378629,-3.10947875451868,6.69523033571205));
#38866=CARTESIAN_POINT('Ctrl Pts',(75.953667507491,-6.16380552501382,3.2471257426054));
#38867=CARTESIAN_POINT('Ctrl Pts',(76.0529233097121,-6.98622033545058,-0.0937807393895811));
#38868=CARTESIAN_POINT('Ctrl Pts',(76.1521791119331,-6.07442354693653,-3.41140773149026));
#38869=CARTESIAN_POINT('Ctrl Pts',(76.2845201815612,-2.92864154611183,-6.7762840899402));
#38870=CARTESIAN_POINT('Ctrl Pts',(76.4499465185962,3.35223617886508,-7.1704019847288));
#38871=CARTESIAN_POINT('Ctrl Pts',(76.6484581230384,7.84373040163857,-1.06061851150057));
#38872=CARTESIAN_POINT('Ctrl Pts',(76.8469697274805,5.14693409302365,6.01315954241379));
#38873=CARTESIAN_POINT('Ctrl Pts',(77.0454813319226,-2.27203010019493,7.58221809534107));
#38874=CARTESIAN_POINT('Ctrl Pts',(77.2109076689577,-6.69646258572395,3.10682413588426));
#38875=CARTESIAN_POINT('Ctrl Pts',(77.3432487385858,-6.80378828733636,-1.49826201944722));
#38876=CARTESIAN_POINT('Ctrl Pts',(77.4425045408069,-5.27556425470762,-4.58088323333947));
#38877=CARTESIAN_POINT('Ctrl Pts',(77.5417603430279,-2.43777019952231,-6.52637729465111));
#38878=CARTESIAN_POINT('Ctrl Pts',(77.674101412656,2.13684521112816,-7.06603565777769));
#38879=CARTESIAN_POINT('Ctrl Pts',(77.839527749691,7.18858075671824,-3.31307390887204));
#38880=CARTESIAN_POINT('Ctrl Pts',(78.0380393541333,6.67563944036266,4.25262933992035));
#38881=CARTESIAN_POINT('Ctrl Pts',(78.2365509585752,0.0500514030952952,
7.91495502814294));
#38882=CARTESIAN_POINT('Ctrl Pts',(78.4350625630174,-6.62932282688847,4.32483882687015));
#38883=CARTESIAN_POINT('Ctrl Pts',(78.6004889000525,-7.12007564968641,-1.94922808210056));
#38884=CARTESIAN_POINT('Ctrl Pts',(78.7328299696805,-4.2297002327542,-5.53587934106734));
#38885=CARTESIAN_POINT('Ctrl Pts',(78.8320857719017,-1.07276168170734,-6.90400259105531));
#38886=CARTESIAN_POINT('Ctrl Pts',(78.9313415741226,2.35047189900519,-6.55832341302287));
#38887=CARTESIAN_POINT('Ctrl Pts',(79.0636826437508,6.19289846700909,-4.01783224520675));
#38888=CARTESIAN_POINT('Ctrl Pts',(79.2291089807858,7.62908074771822,2.10933140267323));
#38889=CARTESIAN_POINT('Ctrl Pts',(79.427620585228,2.35401444720104,7.55695932388457));
#38890=CARTESIAN_POINT('Ctrl Pts',(79.62613218967,-5.07047528444934,6.07777086029618));
#38891=CARTESIAN_POINT('Ctrl Pts',(79.8246437941122,-7.85496122597134,-0.975569659222166));
#38892=CARTESIAN_POINT('Ctrl Pts',(79.9900701311471,-4.18020554900285,-6.08447606137072));
#38893=CARTESIAN_POINT('Ctrl Pts',(80.1224112007755,0.342474109717358,-6.95837880702041));
#38894=CARTESIAN_POINT('Ctrl Pts',(80.2216670029962,3.63680739682284,-5.96571046577456));
#38895=CARTESIAN_POINT('Ctrl Pts',(80.3209228052176,6.02836446611632,-3.4921549223199));
#38896=CARTESIAN_POINT('Ctrl Pts',(80.4532638748454,7.32346177601447,0.92837222522132));
#38897=CARTESIAN_POINT('Ctrl Pts',(80.6186902118807,4.46564646622055,6.53530057918074));
#38898=CARTESIAN_POINT('Ctrl Pts',(80.8172018163227,-3.07963355695854,7.29142478500135));
#38899=CARTESIAN_POINT('Ctrl Pts',(81.0157134207649,-7.79573834066554,1.36948237095418));
#38900=CARTESIAN_POINT('Ctrl Pts',(81.2142250252069,-5.36996070176256,-5.81512459737828));
#38901=CARTESIAN_POINT('Ctrl Pts',(81.3796513622421,0.734369833000959,-7.3454522203664));
#38902=CARTESIAN_POINT('Ctrl Pts',(81.5119924318701,4.75286563427561,-5.09377977540636));
#38903=CARTESIAN_POINT('Ctrl Pts',(81.6112482340912,6.62836938468186,-2.20925071081801));
#38904=CARTESIAN_POINT('Ctrl Pts',(81.7105040363122,6.85849201081093,1.22368765437101));
#38905=CARTESIAN_POINT('Ctrl Pts',(81.8428451059403,4.994463473249,5.43601894659032));
#38906=CARTESIAN_POINT('Ctrl Pts',(82.0082714429754,-0.807333759365405,
7.87403100212955));
#38907=CARTESIAN_POINT('Ctrl Pts',(82.2067830474175,-7.05848021745994,3.58146272634573));
#38908=CARTESIAN_POINT('Ctrl Pts',(82.4052946518597,-6.8383390271391,-3.98574178671712));
#38909=CARTESIAN_POINT('Ctrl Pts',(82.6038062563016,-0.348221341641362,
-7.90764781200667));
#38910=CARTESIAN_POINT('Ctrl Pts',(82.769232593337,5.3020330905482,-5.13647860698734));
#38911=CARTESIAN_POINT('Ctrl Pts',(82.9015736629648,6.91803051641495,-0.822908203731382));
#38912=CARTESIAN_POINT('Ctrl Pts',(83.0008294651861,6.48872744559679,2.59084649097491));
#38913=CARTESIAN_POINT('Ctrl Pts',(83.100085267407,4.44870701128368,5.36146715606584));
#38914=CARTESIAN_POINT('Ctrl Pts',(83.2324263370351,0.306109085628454,7.37572129360934));
#38915=CARTESIAN_POINT('Ctrl Pts',(83.3978526740702,-5.69893411744994,5.49311404819464));
#38916=CARTESIAN_POINT('Ctrl Pts',(83.5963642785123,-7.70294104450956,-1.82036191601753));
#38917=CARTESIAN_POINT('Ctrl Pts',(83.7948758829544,-2.65054732403995,-7.45812423626086));
#38918=CARTESIAN_POINT('Ctrl Pts',(83.9933874873965,4.83801579600438,-6.26464326032379));
#38919=CARTESIAN_POINT('Ctrl Pts',(84.1588138244316,7.36504612864948,-0.501061768818908));
#38920=CARTESIAN_POINT('Ctrl Pts',(84.2911548940597,5.81515720355302,3.83670051421568));
#38921=CARTESIAN_POINT('Ctrl Pts',(84.3904106962808,3.2838476358709,6.16704257382927));
#38922=CARTESIAN_POINT('Ctrl Pts',(84.4896664985018,-0.0626218303453555,
6.96652012443667));
#38923=CARTESIAN_POINT('Ctrl Pts',(84.6220075681298,-4.5268494897441,5.83117493053597));
#38924=CARTESIAN_POINT('Ctrl Pts',(84.7874339051651,-7.89839047263792,0.51728131925656));
#38925=CARTESIAN_POINT('Ctrl Pts',(84.985945509607,-4.70857641573474,-6.36225796220678));
#38926=CARTESIAN_POINT('Ctrl Pts',(85.1844571140492,2.78934783134507,-7.40733129515937));
#38927=CARTESIAN_POINT('Ctrl Pts',(85.3829687184914,7.73880184004112,-1.66225693022602));
#38928=CARTESIAN_POINT('Ctrl Pts',(85.5483950555264,5.94885334375496,4.3710537937438));
#38929=CARTESIAN_POINT('Ctrl Pts',(85.6807361251546,1.96523676419218,6.68387377188444));
#38930=CARTESIAN_POINT('Ctrl Pts',(85.7799919273754,-1.47230308472022,6.82996288641172));
#38931=CARTESIAN_POINT('Ctrl Pts',(85.8792477295967,-4.54436847615697,5.28062868328456));
#38932=CARTESIAN_POINT('Ctrl Pts',(86.0115887992246,-7.22135016146877,1.53201475801043));
#38933=CARTESIAN_POINT('Ctrl Pts',(86.1770151362597,-6.36669217588134,-4.70291215727867));
#38934=CARTESIAN_POINT('Ctrl Pts',(86.375526740702,0.510092880993074,-7.8986596010486));
#38935=CARTESIAN_POINT('Ctrl Pts',(86.5740383451439,6.91157096571897,-3.85735725935614));
#38936=CARTESIAN_POINT('Ctrl Pts',(86.7725499495862,6.98382199278953,3.72537010168621));
#38937=CARTESIAN_POINT('Ctrl Pts',(86.9379762866211,1.72245613756997,7.17830845167958));
#38938=CARTESIAN_POINT('Ctrl Pts',(87.0703173562493,-2.81305032408128,6.37362314637467));
#38939=CARTESIAN_POINT('Ctrl Pts',(87.1695731584703,-5.53294621770099,4.26644765057143));
#38940=CARTESIAN_POINT('Ctrl Pts',(87.2688289606914,-6.87938134896713,1.10019834270945));
#38941=CARTESIAN_POINT('Ctrl Pts',(87.4011700303194,-6.50452616627225,-3.49086045633253));
#38942=CARTESIAN_POINT('Ctrl Pts',(87.5665963673546,-1.82740477450515,-7.70147672927888));
#38943=CARTESIAN_POINT('Ctrl Pts',(87.7651079717965,5.48779720739767,-5.7037794532184));
#38944=CARTESIAN_POINT('Ctrl Pts',(87.9636195762388,7.76880736003202,1.51481036542182));
#38945=CARTESIAN_POINT('Ctrl Pts',(88.1621311806809,2.92972443199612,7.35315352580599));
#38946=CARTESIAN_POINT('Ctrl Pts',(88.327557517716,-3.31761953294659,6.59457110113453));
#38947=CARTESIAN_POINT('Ctrl Pts',(88.4598985873441,-6.26246846883917,3.05250926527866));
#38948=CARTESIAN_POINT('Ctrl Pts',(88.5591543895651,-6.97985708577932,-0.312513143937597));
#38949=CARTESIAN_POINT('Ctrl Pts',(88.6584101917861,-5.96461367324412,-3.59995942571118));
#38950=CARTESIAN_POINT('Ctrl Pts',(88.7907512614142,-2.71500107481349,-6.86467308304396));
#38951=CARTESIAN_POINT('Ctrl Pts',(88.9561775984493,3.5751382292627,-7.06190757962553));
#38952=CARTESIAN_POINT('Ctrl Pts',(89.1546892028915,7.87309740409461,-0.814466393484584));
#38953=CARTESIAN_POINT('Ctrl Pts',(89.3532008073335,4.95610342639328,6.17139020540508));
#38954=CARTESIAN_POINT('Ctrl Pts',(89.5517124117758,-2.50835825604882,7.5073491247457));
#38955=CARTESIAN_POINT('Ctrl Pts',(89.7171387488106,-6.79047064086134,2.89559594020068));
#38956=CARTESIAN_POINT('Ctrl Pts',(89.849479818439,-6.75353219428684,-1.71059259864776));
#38957=CARTESIAN_POINT('Ctrl Pts',(89.9487356206597,-5.1295232397943,-4.74384451004123));
#38958=CARTESIAN_POINT('Ctrl Pts',(90.0479914228811,-2.23219648638674,-6.59951687504316));
#38959=CARTESIAN_POINT('Ctrl Pts',(90.1803324925088,2.35707505352007,-6.99565326223221));
#38960=CARTESIAN_POINT('Ctrl Pts',(90.3457588295442,7.28880630570573,-3.08633353016368));
#38961=CARTESIAN_POINT('Ctrl Pts',(90.5442704339861,6.53919125029974,4.4595959494645));
#38962=CARTESIAN_POINT('Ctrl Pts',(90.7427820384283,-0.19783552455262,7.91264047873421));
#38963=CARTESIAN_POINT('Ctrl Pts',(90.9412936428704,-6.76150679729253,4.11511577621764));
#38964=CARTESIAN_POINT('Ctrl Pts',(91.1067199799056,-7.05554211211308,-2.17124224293496));
#38965=CARTESIAN_POINT('Ctrl Pts',(91.2390610495335,-4.05426579474709,-5.66562026642814));
#38966=CARTESIAN_POINT('Ctrl Pts',(91.3383168517547,-0.856031844848053,
-6.93421076140923));
#38967=CARTESIAN_POINT('Ctrl Pts',(91.4375726539757,2.55469760093386,-6.48150015857438));
#38968=CARTESIAN_POINT('Ctrl Pts',(91.5699137236037,6.31568235787109,-3.8219267036121));
#38969=CARTESIAN_POINT('Ctrl Pts',(91.735340060639,7.55928381707499,2.34720689212017));
#38970=CARTESIAN_POINT('Ctrl Pts',(91.933851665081,2.11620841207976,7.62697057796343));
#38971=CARTESIAN_POINT('Ctrl Pts',(92.1323632695231,-5.25831810102433,5.91600447843957));
#38972=CARTESIAN_POINT('Ctrl Pts',(92.3308748739652,-7.82055805653044,-1.22107481586712));
#38973=CARTESIAN_POINT('Ctrl Pts',(92.4963012110002,-3.98761569413683,-6.21239796287884));
#38974=CARTESIAN_POINT('Ctrl Pts',(92.6286422806284,0.560212663843672,-6.94424120470236));
#38975=CARTESIAN_POINT('Ctrl Pts',(92.7278980828494,3.82184411568555,-5.8488953622404));
#38976=CARTESIAN_POINT('Ctrl Pts',(92.8271538850705,6.13476709898446,-3.30165970067103));
#38977=CARTESIAN_POINT('Ctrl Pts',(92.9594949546986,7.29079730496156,1.15725625134272));
#38978=CARTESIAN_POINT('Ctrl Pts',(93.1249212917336,4.25879872825919,6.67194015363493));
#38979=CARTESIAN_POINT('Ctrl Pts',(93.3234328961758,-3.30645922123453,7.19140776613244));
#38980=CARTESIAN_POINT('Ctrl Pts',(93.5219445006179,-7.83480117000039,1.12468167364702));
#38981=CARTESIAN_POINT('Ctrl Pts',(93.7204561050599,-5.18522225368139,-5.98043662297633));
#38982=CARTESIAN_POINT('Ctrl Pts',(93.8858824420952,0.96403765515393,-7.31885228521195));
#38983=CARTESIAN_POINT('Ctrl Pts',(94.0182235117231,4.91004985228958,-4.94244216818445));
#38984=CARTESIAN_POINT('Ctrl Pts',(94.1174793139444,6.69430269395043,-2.00059512265878));
#38985=CARTESIAN_POINT('Ctrl Pts',(94.2167351161651,6.81680757716476,1.43786598601073));
#38986=CARTESIAN_POINT('Ctrl Pts',(94.3490761857935,4.82178115027497,5.58975794754651));
#38987=CARTESIAN_POINT('Ctrl Pts',(94.5145025228283,-1.05351861191065,7.84488690523109));
#38988=CARTESIAN_POINT('Ctrl Pts',(94.7130141272707,-7.16717435960562,3.35866490431669));
#38989=CARTESIAN_POINT('Ctrl Pts',(94.9115257317125,-6.71016881124756,-4.19793434501272));
#38990=CARTESIAN_POINT('Ctrl Pts',(95.1100373361551,-0.100417005100013,
-7.91467424766143));
#38991=CARTESIAN_POINT('Ctrl Pts',(95.2754636731895,5.46028510951729,-4.96792249296327));
#38992=CARTESIAN_POINT('Ctrl Pts',(95.4078047428182,6.9404074694083,-0.605861614891436));
#38993=CARTESIAN_POINT('Ctrl Pts',(95.5070605450388,6.40441082567987,2.7927748528931));
#38994=CARTESIAN_POINT('Ctrl Pts',(95.6063163472603,4.27862700004775,5.49815197428002));
#38995=CARTESIAN_POINT('Ctrl Pts',(95.7386574168879,0.0749830561122438,
7.38168984139835));
#38996=CARTESIAN_POINT('Ctrl Pts',(95.9040837539233,-5.86815976306963,5.31195378524688));
#38997=CARTESIAN_POINT('Ctrl Pts',(96.1025953583653,-7.64215717114619,-2.06069211964716));
#38998=CARTESIAN_POINT('Ctrl Pts',(96.3011069628075,-2.41569094255804,-7.53747010014103));
#38999=CARTESIAN_POINT('Ctrl Pts',(96.4996185672496,5.03182466448517,-6.11006485787073));
#39000=CARTESIAN_POINT('Ctrl Pts',(96.6650449042846,7.3771249924399,-0.270174423708261));
#39001=CARTESIAN_POINT('Ctrl Pts',(96.7973859739128,5.69215614644194,4.01692451290047));
#39002=CARTESIAN_POINT('Ctrl Pts',(96.8966417761337,3.08911177755644,6.26685390198305));
#39003=CARTESIAN_POINT('Ctrl Pts',(96.995897578355,-0.280752591029069,6.96114229997113));
#39004=CARTESIAN_POINT('Ctrl Pts',(97.1282386479826,-4.70723660648295,5.68655351719244));
#39005=CARTESIAN_POINT('Ctrl Pts',(97.2936649850182,-7.91071568063838,0.269683966171925));
#39006=CARTESIAN_POINT('Ctrl Pts',(97.4921765894599,-4.50702848227491,-6.50658992871379));
#39007=CARTESIAN_POINT('Ctrl Pts',(97.6906881939024,3.01994556208542,-7.31634793066305));
#39008=CARTESIAN_POINT('Ctrl Pts',(97.8891997983443,7.78706103537034,-1.41909564615117));
#39009=CARTESIAN_POINT('Ctrl Pts',(98.0546261353794,5.80905306594097,4.55520250377396));
#39010=CARTESIAN_POINT('Ctrl Pts',(98.1869672050076,1.75496269546036,6.742138390404));
#39011=CARTESIAN_POINT('Ctrl Pts',(98.2862230072284,-1.68546607162555,6.78050687813509));
#39012=CARTESIAN_POINT('Ctrl Pts',(98.3854788094498,-4.70750625791352,5.13572866977243));
#39013=CARTESIAN_POINT('Ctrl Pts',(98.5178198790775,-7.26578451938068,1.30512171510342));
#39014=CARTESIAN_POINT('Ctrl Pts',(98.6832462161129,-6.21629458823582,-4.89998302178471));
#39015=CARTESIAN_POINT('Ctrl Pts',(98.8817578205548,0.757194779261698,-7.87881173190068));
#39016=CARTESIAN_POINT('Ctrl Pts',(99.0802694249971,7.0289769917291,-3.63902468942159));
#39017=CARTESIAN_POINT('Ctrl Pts',(99.2787810294391,6.86373414608865,3.94224626238962));
#39018=CARTESIAN_POINT('Ctrl Pts',(99.4442073664742,1.49681757276813,7.22872772534415));
#39019=CARTESIAN_POINT('Ctrl Pts',(99.5765484361023,-3.01126513256809,6.28240451094936));
#39020=CARTESIAN_POINT('Ctrl Pts',(99.6758042383233,-5.66383935284861,4.09108704235948));
#39021=CARTESIAN_POINT('Ctrl Pts',(99.7750600405444,-6.91046079330171,0.884226080851057));
#39022=CARTESIAN_POINT('Ctrl Pts',(99.9074011101725,-6.39201722787976,-3.69284214823692));
#39023=CARTESIAN_POINT('Ctrl Pts',(100.072827447207,-1.58533135460785,-7.75492595178093));
#39024=CARTESIAN_POINT('Ctrl Pts',(100.27133905165,5.66372354179168,-5.52912776870199));
#39025=CARTESIAN_POINT('Ctrl Pts',(100.469850656092,7.71755974363839,1.75735307888005));
#39026=CARTESIAN_POINT('Ctrl Pts',(100.668362260534,2.69801835775111,7.44129350064531));
#39027=CARTESIAN_POINT('Ctrl Pts',(100.833788597569,-3.52250601247792,6.487443160858));
#39028=CARTESIAN_POINT('Ctrl Pts',(100.966129667197,-6.35498847103736,2.85489853949308));
#39029=CARTESIAN_POINT('Ctrl Pts',(101.065385469418,-6.96664719799234,-0.530939000021162));
#39030=CARTESIAN_POINT('Ctrl Pts',(101.164641271639,-5.84895302775269,-3.78497987008646));
#39031=CARTESIAN_POINT('Ctrl Pts',(101.296982341267,-2.49869742150455,-6.9463284236403));
#39032=CARTESIAN_POINT('Ctrl Pts',(101.462408678302,3.79453337725676,-6.94648605198287));
#39033=CARTESIAN_POINT('Ctrl Pts',(101.660920282744,7.89474157672574,-0.567515354149183));
#39034=CARTESIAN_POINT('Ctrl Pts',(101.859431887187,4.76041124955647,6.32356726662831));
#39035=CARTESIAN_POINT('Ctrl Pts',(102.057943491629,-2.74222592869338,7.42511609185407));
#39036=CARTESIAN_POINT('Ctrl Pts',(102.223369828664,-6.87781782969463,2.68152741452352));
#39037=CARTESIAN_POINT('Ctrl Pts',(102.355710898292,-6.69665146836396,-1.92124523397596));
#39038=CARTESIAN_POINT('Ctrl Pts',(102.454966700513,-4.97845060478972,-4.90215248423675));
#39039=CARTESIAN_POINT('Ctrl Pts',(102.554222502734,-2.02443318093161,-6.66618289831267));
#39040=CARTESIAN_POINT('Ctrl Pts',(102.686563572362,2.57499280848366,-6.91840873391956));
#39041=CARTESIAN_POINT('Ctrl Pts',(102.851989909397,7.38188216406195,-2.85656572432764));
#39042=CARTESIAN_POINT('Ctrl Pts',(103.050501513839,6.39632867735181,4.66218807983374));
#39043=CARTESIAN_POINT('Ctrl Pts',(103.249013118281,-0.445528392606267,
7.90256431115402));
#39044=CARTESIAN_POINT('Ctrl Pts',(103.447524722723,-6.88705831242505,3.90135615173695));
#39045=CARTESIAN_POINT('Ctrl Pts',(103.612951059759,-6.98408769597376,-2.39112660229325));
#39046=CARTESIAN_POINT('Ctrl Pts',(103.745292129387,-3.87485447150524,-5.78980370675049));
#39047=CARTESIAN_POINT('Ctrl Pts',(103.844547931608,-0.638462314547805,
-6.95761706874731));
#39048=CARTESIAN_POINT('Ctrl Pts',(103.943803733829,2.75641736475526,-6.39831911131053));
#39049=CARTESIAN_POINT('Ctrl Pts',(104.076144803457,6.4322711087958,-3.62227218122517));
#39050=CARTESIAN_POINT('Ctrl Pts',(104.241571140492,7.48207188069434,2.58277997359283));
#39051=CARTESIAN_POINT('Ctrl Pts',(104.440082744934,1.87632655891563,7.68950043201341));
#39052=CARTESIAN_POINT('Ctrl Pts',(104.638594349376,-5.44100296080544,5.74843500509099));
#39053=CARTESIAN_POINT('Ctrl Pts',(104.837105953818,-7.77848359392374,-1.46538220120157));
#39054=CARTESIAN_POINT('Ctrl Pts',(105.002532290853,-3.79111433187881,-6.33422604138052));
#39055=CARTESIAN_POINT('Ctrl Pts',(105.134873360482,0.777401697416134,-6.92329189505096));
#39056=CARTESIAN_POINT('Ctrl Pts',(105.234129162702,4.00313193543719,-5.72634300828974));
#39057=CARTESIAN_POINT('Ctrl Pts',(105.333384964924,6.23515205328682,-3.10792581387005));
#39058=CARTESIAN_POINT('Ctrl Pts',(105.465726034551,7.25098119224185,1.38500506214225));
#39059=CARTESIAN_POINT('Ctrl Pts',(105.631152371587,4.04777347188614,6.80203522519585));
#39060=CARTESIAN_POINT('Ctrl Pts',(105.829663976029,-3.53004152739988,7.08433643778901));
#39061=CARTESIAN_POINT('Ctrl Pts',(106.028175580471,-7.86617874706874,0.878778052190405));
#39062=CARTESIAN_POINT('Ctrl Pts',(106.226687184913,-4.99539752540193,-6.13988293097007));
#39063=CARTESIAN_POINT('Ctrl Pts',(106.392113521948,1.19275979698265,-7.28507217598246));
#39064=CARTESIAN_POINT('Ctrl Pts',(106.524454591576,5.06241779407946,-4.78625786431911));
#39065=CARTESIAN_POINT('Ctrl Pts',(106.623710393797,6.75366933964939,-1.78997403676776));
#39066=CARTESIAN_POINT('Ctrl Pts',(106.722966196018,6.76843668239335,1.65062819852489));
#39067=CARTESIAN_POINT('Ctrl Pts',(106.855307265646,4.64436855831348,5.73802618614398));
#39068=CARTESIAN_POINT('Ctrl Pts',(107.020733602682,-1.29866899872058,7.80802255608828));
#39069=CARTESIAN_POINT('Ctrl Pts',(107.219245207124,-7.26883987637063,3.13261426953325));
#39070=CARTESIAN_POINT('Ctrl Pts',(107.417756811566,-6.57541326790252,-4.40608594330653));
#39071=CARTESIAN_POINT('Ctrl Pts',(107.616268416008,0.147479460587251,-7.91378549378608));
#39072=CARTESIAN_POINT('Ctrl Pts',(107.781694753043,5.61319225826337,-4.79475969318229));
#39073=CARTESIAN_POINT('Ctrl Pts',(107.914035822671,6.95596082548192,-0.387848333920882));
#39074=CARTESIAN_POINT('Ctrl Pts',(108.013291624892,6.31384625566456,2.99115031483452));
#39075=CARTESIAN_POINT('Ctrl Pts',(108.112547427113,4.10428660238,5.63094528514316));
#39076=CARTESIAN_POINT('Ctrl Pts',(108.244888496741,-0.156076618085431,
7.37716885209829));
#39077=CARTESIAN_POINT('Ctrl Pts',(108.410314833777,-6.03194807359435,5.13225398584684));
#39078=CARTESIAN_POINT('Ctrl Pts',(108.608826438218,-7.57316344147741,-2.31035707660512));
#39079=CARTESIAN_POINT('Ctrl Pts',(108.774252775254,-3.07991499223872,-6.70713847843066));
#39080=CARTESIAN_POINT('Ctrl Pts',(108.906593844881,1.53030863923424,-6.79781064773029));
#39081=CARTESIAN_POINT('Ctrl Pts',(109.005849647103,4.59552813494485,-5.25753008669525));
#39082=CARTESIAN_POINT('Ctrl Pts',(109.105105449324,6.55166018357511,-2.40598671557301));
#39083=CARTESIAN_POINT('Ctrl Pts',(109.171275984138,6.78587654135638,-0.125430911852007));
#39084=CARTESIAN_POINT('Ctrl Pts',(109.204361251545,6.62354718454475,0.976096068216178));
#39085=CARTESIAN_POINT('Ctrl Pts',(30.9296387484553,-1.74764629024929,6.21616713138321));
#39086=CARTESIAN_POINT('Ctrl Pts',(30.9627240158623,-2.78142405570536,5.92552535188211));
#39087=CARTESIAN_POINT('Ctrl Pts',(31.0288945506764,-4.69724081460228,4.82165246972101));
#39088=CARTESIAN_POINT('Ctrl Pts',(31.1281503528974,-6.43804454172866,1.97690416673953));
#39089=CARTESIAN_POINT('Ctrl Pts',(31.2274061551185,-6.58774752332024,-1.32825939138557));
#39090=CARTESIAN_POINT('Ctrl Pts',(31.3597472247465,-4.69328518013838,-5.35182557713039));
#39091=CARTESIAN_POINT('Ctrl Pts',(31.5251735617817,0.946620568444218,-7.57747210463679));
#39092=CARTESIAN_POINT('Ctrl Pts',(31.7236851662237,6.89312828841085,-3.29096731508787));
#39093=CARTESIAN_POINT('Ctrl Pts',(31.8891115032589,6.55695624239769,2.76629759413725));
#39094=CARTESIAN_POINT('Ctrl Pts',(32.0214525728869,3.34250580260362,5.83017495152525));
#39095=CARTESIAN_POINT('Ctrl Pts',(32.120708375108,0.148489860278677,6.73662245379208));
#39096=CARTESIAN_POINT('Ctrl Pts',(32.219964177329,-3.07942669717768,5.97199294502161));
#39097=CARTESIAN_POINT('Ctrl Pts',(32.3523052469571,-6.43114181568573,3.05509788385159));
#39098=CARTESIAN_POINT('Ctrl Pts',(32.5177315839922,-7.02605788339069,-2.9850845489194));
#39099=CARTESIAN_POINT('Ctrl Pts',(32.7162431884343,-1.29137128331862,-7.52386125263412));
#39100=CARTESIAN_POINT('Ctrl Pts',(32.9147547928764,5.61931759596494,-5.16711469712653));
#39101=CARTESIAN_POINT('Ctrl Pts',(33.1132663973185,7.38605346602491,1.92984446273495));
#39102=CARTESIAN_POINT('Ctrl Pts',(33.2786927343536,3.22420823648018,6.34785971429795));
#39103=CARTESIAN_POINT('Ctrl Pts',(33.4110338039817,-1.21075736553802,6.60924292677451));
#39104=CARTESIAN_POINT('Ctrl Pts',(33.5102896062028,-4.2343605016059,5.24198775609974));
#39105=CARTESIAN_POINT('Ctrl Pts',(33.6095454084238,-6.20686614770307,2.57349290017741));
#39106=CARTESIAN_POINT('Ctrl Pts',(33.7418864780519,-6.88391407523792,-1.81725837294228));
#39107=CARTESIAN_POINT('Ctrl Pts',(33.907312815087,-3.43987083363875,-6.8151117023347));
#39108=CARTESIAN_POINT('Ctrl Pts',(34.1058244195291,3.8699555241471,-6.58019622848891));
#39109=CARTESIAN_POINT('Ctrl Pts',(34.3043360239712,7.62714385347594,-0.319706138503197));
#39110=CARTESIAN_POINT('Ctrl Pts',(34.5028476284133,4.39588281579082,6.24136747571982));
#39111=CARTESIAN_POINT('Ctrl Pts',(34.6682739654485,-1.63456982395356,6.92956681052015));
#39112=CARTESIAN_POINT('Ctrl Pts',(34.8006150350764,-5.19071062760659,4.26668055825536));
#39113=CARTESIAN_POINT('Ctrl Pts',(34.8998708372976,-6.61765701788971,1.27077618895782));
#39114=CARTESIAN_POINT('Ctrl Pts',(34.9991266395185,-6.40188140602722,-2.04057696131233));
#39115=CARTESIAN_POINT('Ctrl Pts',(35.1314677091467,-4.08500492716994,-5.8312476858528));
#39116=CARTESIAN_POINT('Ctrl Pts',(35.2968940461817,1.77142835594066,-7.42566455594743));
#39117=CARTESIAN_POINT('Ctrl Pts',(35.4954056506239,7.2030680549125,-2.52811156639923));
#39118=CARTESIAN_POINT('Ctrl Pts',(35.6939172550659,6.03198848328303,4.67874475198411));
#39119=CARTESIAN_POINT('Ctrl Pts',(35.8924288595082,-0.670900469029075,
7.60449505762471));
#39120=CARTESIAN_POINT('Ctrl Pts',(36.0578551965431,-5.72117530867311,4.23779044678305));
#39121=CARTESIAN_POINT('Ctrl Pts',(36.1901962661713,-6.71860690707006,-0.0914394363855131));
#39122=CARTESIAN_POINT('Ctrl Pts',(36.2894520683923,-5.8748072835785,-3.30074170159639));
#39123=CARTESIAN_POINT('Ctrl Pts',(36.3887078706134,-3.57268564284483,-5.69069040089914));
#39124=CARTESIAN_POINT('Ctrl Pts',(36.5210489402414,0.643638183052046,-7.09058845752315));
#39125=CARTESIAN_POINT('Ctrl Pts',(36.6864752772765,6.14591436535152,-4.52837599322407));
#39126=CARTESIAN_POINT('Ctrl Pts',(36.8849868817187,7.1334925448268,2.71823869833564));
#39127=CARTESIAN_POINT('Ctrl Pts',(37.0834984861608,1.58735598268625,7.46698322566606));
#39128=CARTESIAN_POINT('Ctrl Pts',(37.2820100906028,-5.4207541093524,5.37530254108901));
#39129=CARTESIAN_POINT('Ctrl Pts',(37.447436427638,-7.10513022063766,-0.455893992601426));
#39130=CARTESIAN_POINT('Ctrl Pts',(37.579777497266,-5.07267154871018,-4.40636395457348));
#39131=CARTESIAN_POINT('Ctrl Pts',(37.6790332994871,-2.35673207543457,-6.31300802510474));
#39132=CARTESIAN_POINT('Ctrl Pts',(37.7782891017082,0.944226464651675,-6.65255412038963));
#39133=CARTESIAN_POINT('Ctrl Pts',(37.9106301713362,5.06823027977708,-5.00037564747394));
#39134=CARTESIAN_POINT('Ctrl Pts',(38.0760565083713,7.61710545174979,0.508091585475629));
#39135=CARTESIAN_POINT('Ctrl Pts',(38.2745681128134,3.694095804285,6.68050849089578));
#39136=CARTESIAN_POINT('Ctrl Pts',(38.4730797172555,-3.60713443837236,6.72786137280452));
#39137=CARTESIAN_POINT('Ctrl Pts',(38.6715913216977,-7.60987439777963,0.606847734052926));
#39138=CARTESIAN_POINT('Ctrl Pts',(38.8370176587327,-5.13266210331478,-4.93421670763416));
#39139=CARTESIAN_POINT('Ctrl Pts',(38.9693587283608,-1.03043505637373,-6.63974724939573));
#39140=CARTESIAN_POINT('Ctrl Pts',(39.0686145305819,2.27464993583887,-6.34304533089632));
#39141=CARTESIAN_POINT('Ctrl Pts',(39.1678703328029,5.01509137070583,-4.47178918160662));
#39142=CARTESIAN_POINT('Ctrl Pts',(39.300211402431,7.09861927260105,-0.548013875149835));
#39143=CARTESIAN_POINT('Ctrl Pts',(39.4656377394661,5.49001932721968,5.30453959444752));
#39144=CARTESIAN_POINT('Ctrl Pts',(39.6641493439083,-1.49037074416326,7.48694413984165));
#39145=CARTESIAN_POINT('Ctrl Pts',(39.8626609483503,-7.09763510524872,2.81053614474318));
#39146=CARTESIAN_POINT('Ctrl Pts',(40.0611725527924,-6.20413338397556,-4.44827848455409));
#39147=CARTESIAN_POINT('Ctrl Pts',(40.2265988898275,-0.735553655790395,
-7.0816435665849));
#39148=CARTESIAN_POINT('Ctrl Pts',(40.3589399594556,3.49857308487482,-5.73655177881727));
#39149=CARTESIAN_POINT('Ctrl Pts',(40.4581957616766,5.83150027903981,-3.37666416689254));
#39150=CARTESIAN_POINT('Ctrl Pts',(40.5574515638978,6.71685569069011,-0.178576514989967));
#39151=CARTESIAN_POINT('Ctrl Pts',(40.6897926335258,5.77566097104865,4.16322652905234));
#39152=CARTESIAN_POINT('Ctrl Pts',(40.8552189705609,0.769479356240343,7.59515332581423));
#39153=CARTESIAN_POINT('Ctrl Pts',(41.053730575003,-5.9707946456355,4.75659003991491));
#39154=CARTESIAN_POINT('Ctrl Pts',(41.2522421794451,-7.23525339279788,-2.43447034284124));
#39155=CARTESIAN_POINT('Ctrl Pts',(41.4507537838872,-1.86759511254066,-7.40206329464434));
#39156=CARTESIAN_POINT('Ctrl Pts',(41.6161801209223,4.00902614733043,-5.88374235794879));
#39157=CARTESIAN_POINT('Ctrl Pts',(41.7485211905504,6.37487523671707,-2.12344193646858));
#39158=CARTESIAN_POINT('Ctrl Pts',(41.8477769927715,6.63358312000962,1.18483390833526));
#39159=CARTESIAN_POINT('Ctrl Pts',(41.9470327949925,5.24561565699268,4.19899467972695));
#39160=CARTESIAN_POINT('Ctrl Pts',(42.0793738646206,1.7243133381715,6.90778244420767));
#39161=CARTESIAN_POINT('Ctrl Pts',(42.2448002016556,-4.31455827790939,6.29785990546237));
#39162=CARTESIAN_POINT('Ctrl Pts',(42.4433118060978,-7.63064917983663,-0.220750090431982));
#39163=CARTESIAN_POINT('Ctrl Pts',(42.6418234105399,-3.95497920617077,-6.52944691278856));
#39164=CARTESIAN_POINT('Ctrl Pts',(42.840335014982,3.35118444795746,-6.8591555834574));
#39165=CARTESIAN_POINT('Ctrl Pts',(43.0057613520171,6.85976484305111,-1.90639478669554));
#39166=CARTESIAN_POINT('Ctrl Pts',(43.1381024216452,6.23972265263023,2.49276977667716));
#39167=CARTESIAN_POINT('Ctrl Pts',(43.2373582238662,4.30199909517582,5.18662319679422));
#39168=CARTESIAN_POINT('Ctrl Pts',(43.3366140260872,1.29637667797795,6.59298471483567));
#39169=CARTESIAN_POINT('Ctrl Pts',(43.4689550957154,-3.14159009001819,6.38914129527586));
#39170=CARTESIAN_POINT('Ctrl Pts',(43.6343814327504,-7.36042316718463,2.02549335281035));
#39171=CARTESIAN_POINT('Ctrl Pts',(43.8328930371926,-5.68582852314473,-5.09380913595719));
#39172=CARTESIAN_POINT('Ctrl Pts',(44.0314046416347,1.19360462082791,-7.53994996782506));
#39173=CARTESIAN_POINT('Ctrl Pts',(44.2299162460768,6.98688357126563,-3.07602186011172));
#39174=CARTESIAN_POINT('Ctrl Pts',(44.3953425831118,6.46998971585273,2.97152281859987));
#39175=CARTESIAN_POINT('Ctrl Pts',(44.52768365274,3.15696064319814,5.93141125184893));
#39176=CARTESIAN_POINT('Ctrl Pts',(44.626939454961,-0.0618247881750454,
6.7382812419774));
#39177=CARTESIAN_POINT('Ctrl Pts',(44.726195257182,-3.26526325658163,5.87248633940344));
#39178=CARTESIAN_POINT('Ctrl Pts',(44.8585363268102,-6.52342426137875,2.85230620564395));
#39179=CARTESIAN_POINT('Ctrl Pts',(45.0239626638452,-6.92926609411708,-3.20370471785814));
#39180=CARTESIAN_POINT('Ctrl Pts',(45.2224742682874,-1.05505487162644,-7.56058177166444));
#39181=CARTESIAN_POINT('Ctrl Pts',(45.4209858727294,5.77833642645426,-4.98862362289226));
#39182=CARTESIAN_POINT('Ctrl Pts',(45.6194974771717,7.32201870880574,2.16020706188214));
#39183=CARTESIAN_POINT('Ctrl Pts',(45.7849238142066,3.0238283147716,6.44570997699132));
#39184=CARTESIAN_POINT('Ctrl Pts',(45.9172648838347,-1.41713158479941,6.56808785055635));
#39185=CARTESIAN_POINT('Ctrl Pts',(46.0165206860558,-4.39644299388766,5.10681362513981));
#39186=CARTESIAN_POINT('Ctrl Pts',(46.1157764882768,-6.28441143515325,2.37785888037478));
#39187=CARTESIAN_POINT('Ctrl Pts',(46.248117557905,-6.82362998403564,-2.03194208226253));
#39188=CARTESIAN_POINT('Ctrl Pts',(46.41354389494,-3.22476320316531,-6.91949093545313));
#39189=CARTESIAN_POINT('Ctrl Pts',(46.6120554993822,4.07412068923817,-6.45577866083469));
#39190=CARTESIAN_POINT('Ctrl Pts',(46.8105671038242,7.63341503086778,-0.0806999051357613));
#39191=CARTESIAN_POINT('Ctrl Pts',(47.0090787082664,4.19827393130149,6.37596647733199));
#39192=CARTESIAN_POINT('Ctrl Pts',(47.1745050453014,-1.85077235155308,6.8749804717851));
#39193=CARTESIAN_POINT('Ctrl Pts',(47.3068461149295,-5.32177892736629,4.10203717553878));
#39194=CARTESIAN_POINT('Ctrl Pts',(47.4061019171506,-6.6542065815006,1.06291635189777));
#39195=CARTESIAN_POINT('Ctrl Pts',(47.5053577193716,-6.33483946216542,-2.24005556401035));
#39196=CARTESIAN_POINT('Ctrl Pts',(47.6376987889997,-3.90039178526545,-5.95631250910608));
#39197=CARTESIAN_POINT('Ctrl Pts',(47.8031251260348,2.00309944932168,-7.36654906441504));
#39198=CARTESIAN_POINT('Ctrl Pts',(48.0016367304768,7.27870485203315,-2.301302497534));
#39199=CARTESIAN_POINT('Ctrl Pts',(48.2001483349191,5.88251187212179,4.86534598795536));
#39200=CARTESIAN_POINT('Ctrl Pts',(48.3986599393611,-0.9087115283618,7.57975566100446));
#39201=CARTESIAN_POINT('Ctrl Pts',(48.5640862763962,-5.85107870524407,4.05654936734897));
#39202=CARTESIAN_POINT('Ctrl Pts',(48.6964273460243,-6.71244822969185,-0.301792486600593));
#39203=CARTESIAN_POINT('Ctrl Pts',(48.7956831482453,-5.76856089762008,-3.48309654917376));
#39204=CARTESIAN_POINT('Ctrl Pts',(48.8949389504664,-3.39272542501121,-5.79978052444612));
#39205=CARTESIAN_POINT('Ctrl Pts',(49.0272800200945,0.865369267295591,-7.06695484745162));
#39206=CARTESIAN_POINT('Ctrl Pts',(49.1927063571296,6.28470933619326,-4.33369139208969));
#39207=CARTESIAN_POINT('Ctrl Pts',(49.3912179615717,7.04487031890815,2.94029585210974));
#39208=CARTESIAN_POINT('Ctrl Pts',(49.5897295660138,1.3527436252517,7.51303016049503));
#39209=CARTESIAN_POINT('Ctrl Pts',(49.7882411704559,-5.58642684012997,5.20291146207417));
#39210=CARTESIAN_POINT('Ctrl Pts',(49.953667507491,-7.08736881972858,-0.678172542822872));
#39211=CARTESIAN_POINT('Ctrl Pts',(50.0860085771191,-4.93219523779632,-4.56305709777133));
#39212=CARTESIAN_POINT('Ctrl Pts',(50.1852643793401,-2.15787991664417,-6.38371448811436));
#39213=CARTESIAN_POINT('Ctrl Pts',(50.2845201815612,1.15209277018053,-6.61972221397241));
#39214=CARTESIAN_POINT('Ctrl Pts',(50.4168612511892,5.22233480911237,-4.83920798542831));
#39215=CARTESIAN_POINT('Ctrl Pts',(50.5822875882244,7.59745834475163,0.746377399222896));
#39216=CARTESIAN_POINT('Ctrl Pts',(50.7807991926665,3.48307919085419,6.79291519587912));
#39217=CARTESIAN_POINT('Ctrl Pts',(50.9793107971085,-3.8160530018601,6.61160169665124));
#39218=CARTESIAN_POINT('Ctrl Pts',(51.1778224015507,-7.62514594570818,0.368241536165105));
#39219=CARTESIAN_POINT('Ctrl Pts',(51.3432487385857,-4.97562628966537,-5.09252960818989));
#39220=CARTESIAN_POINT('Ctrl Pts',(51.4755898082139,-0.822001320650966,
-6.66875953758343));
#39221=CARTESIAN_POINT('Ctrl Pts',(51.5748456104349,2.47217124072609,-6.26870207913443));
#39222=CARTESIAN_POINT('Ctrl Pts',(51.674101412656,5.15266890569921,-4.31254485072359));
#39223=CARTESIAN_POINT('Ctrl Pts',(51.806442482284,7.11229914548942,-0.325446846305394));
#39224=CARTESIAN_POINT('Ctrl Pts',(51.9718688193191,5.32121132378008,5.47386176021844));
#39225=CARTESIAN_POINT('Ctrl Pts',(52.1703804237614,-1.72409869935947,7.43660010912471));
#39226=CARTESIAN_POINT('Ctrl Pts',(52.3688920282032,-7.18216793587477,2.58689026614183));
#39227=CARTESIAN_POINT('Ctrl Pts',(52.5674036326456,-6.06178955683664,-4.6403835930808));
#39228=CARTESIAN_POINT('Ctrl Pts',(52.7328299696805,-0.513426252932243,
-7.10120470536513));
#39229=CARTESIAN_POINT('Ctrl Pts',(52.8651710393087,3.67650133636693,-5.62417797237554));
#39230=CARTESIAN_POINT('Ctrl Pts',(52.9644268415297,5.93438279112921,-3.19239052886186));
#39231=CARTESIAN_POINT('Ctrl Pts',(53.0636826437508,6.71915361157393,0.0318541258702626));
#39232=CARTESIAN_POINT('Ctrl Pts',(53.1960237133788,5.64245389348959,4.34205352852127));
#39233=CARTESIAN_POINT('Ctrl Pts',(53.361450050414,0.531254395267008,7.61552501734556));
#39234=CARTESIAN_POINT('Ctrl Pts',(53.559961654856,-6.11682218841227,4.56727750673352));
#39235=CARTESIAN_POINT('Ctrl Pts',(53.7584732592982,-7.15546766306728,-2.65985338523861));
#39236=CARTESIAN_POINT('Ctrl Pts',(53.9569848637402,-1.63487832315821,-7.45691795521279));
#39237=CARTESIAN_POINT('Ctrl Pts',(54.1224112007754,4.19131342003372,-5.7553111644589));
#39238=CARTESIAN_POINT('Ctrl Pts',(54.2547522704034,6.43824571186064,-1.92276678122184));
#39239=CARTESIAN_POINT('Ctrl Pts',(54.3540080726245,6.59322572684469,1.39198811607388));
#39240=CARTESIAN_POINT('Ctrl Pts',(54.4532638748455,5.11154843903565,4.36120539491713));
#39241=CARTESIAN_POINT('Ctrl Pts',(54.5856049444738,1.50714557455112,6.95839255876029));
#39242=CARTESIAN_POINT('Ctrl Pts',(54.7510312815086,-4.50966408232794,6.15965765175859));
#39243=CARTESIAN_POINT('Ctrl Pts',(54.9495428859509,-7.61999373109382,-0.459600964161025));
#39244=CARTESIAN_POINT('Ctrl Pts',(55.1480544903929,-3.74856524016585,-6.65009745405187));
#39245=CARTESIAN_POINT('Ctrl Pts',(55.3465660948351,3.56434011436733,-6.75084676699293));
#39246=CARTESIAN_POINT('Ctrl Pts',(55.5119924318701,6.91610051670058,-1.69064142490175));
#39247=CARTESIAN_POINT('Ctrl Pts',(55.6443335014983,6.1585995000709,2.68694848089583));
#39248=CARTESIAN_POINT('Ctrl Pts',(55.7435893037193,4.13746639931955,5.31879950693002));
#39249=CARTESIAN_POINT('Ctrl Pts',(55.8428451059403,1.08927691098905,6.63034808682382));
#39250=CARTESIAN_POINT('Ctrl Pts',(55.9751861755685,-3.34012972565061,6.28762659518877));
#39251=CARTESIAN_POINT('Ctrl Pts',(56.1406125126035,-7.42024294481071,1.79400311100452));
#39252=CARTESIAN_POINT('Ctrl Pts',(56.3391241170456,-5.52352365615058,-5.26936655852601));
#39253=CARTESIAN_POINT('Ctrl Pts',(56.5376357214877,1.42913804177327,-7.49887337976339));
#39254=CARTESIAN_POINT('Ctrl Pts',(56.7361473259298,7.07978459251398,-2.85571403433688));
#39255=CARTESIAN_POINT('Ctrl Pts',(56.9015736629649,6.37376113923339,3.17267769001173));
#39256=CARTESIAN_POINT('Ctrl Pts',(57.0339147325929,2.96966597794152,6.02736459165353));
#39257=CARTESIAN_POINT('Ctrl Pts',(57.133170534814,-0.272808478755478,6.73304031878143));
#39258=CARTESIAN_POINT('Ctrl Pts',(57.2324263370351,-3.44756282279183,5.76735212416978));
#39259=CARTESIAN_POINT('Ctrl Pts',(57.3647674066631,-6.60954677648735,2.64662165677788));
#39260=CARTESIAN_POINT('Ctrl Pts',(57.5301937436982,-6.82554132287069,-3.41912827663594));
#39261=CARTESIAN_POINT('Ctrl Pts',(57.7287053481404,-0.817772480688494,
-7.58991341702892));
#39262=CARTESIAN_POINT('Ctrl Pts',(57.9272169525824,5.93172465642349,-4.80522425163951));
#39263=CARTESIAN_POINT('Ctrl Pts',(58.1257285570247,7.25077917183186,2.38844173544932));
#39264=CARTESIAN_POINT('Ctrl Pts',(58.2911548940596,2.82049331914008,6.53724194300516));
#39265=CARTESIAN_POINT('Ctrl Pts',(58.4234959636878,-1.62212083014546,6.52048801499322));
#39266=CARTESIAN_POINT('Ctrl Pts',(58.5227517659088,-4.55421018600847,4.96663125086556));
#39267=CARTESIAN_POINT('Ctrl Pts',(58.6220075681299,-6.35579352430296,2.17989188211036));
#39268=CARTESIAN_POINT('Ctrl Pts',(58.7543486377579,-6.75665159323421,-2.24463227107365));
#39269=CARTESIAN_POINT('Ctrl Pts',(58.9197749747931,-3.00649287392933,-7.01708294958232));
#39270=CARTESIAN_POINT('Ctrl Pts',(59.1182865792351,4.27428975474489,-6.32502842686495));
#39271=CARTESIAN_POINT('Ctrl Pts',(59.3167981836773,7.6321983440743,0.158385431391267));
#39272=CARTESIAN_POINT('Ctrl Pts',(59.5153097881193,3.99654698742823,6.50431123944617));
#39273=CARTESIAN_POINT('Ctrl Pts',(59.6807361251545,-2.06515947292264,6.81365035323193));
#39274=CARTESIAN_POINT('Ctrl Pts',(59.8130771947826,-5.44762700138892,3.9333700556902));
#39275=CARTESIAN_POINT('Ctrl Pts',(59.9123329970036,-6.68422895260743,0.854013881352277));
#39276=CARTESIAN_POINT('Ctrl Pts',(60.0115887992247,-6.26158358209626,-2.43733686339917));
#39277=CARTESIAN_POINT('Ctrl Pts',(60.1439298688528,-3.71195269870614,-6.07553470463859));
#39278=CARTESIAN_POINT('Ctrl Pts',(60.3093562058878,2.23280567678422,-7.30020762252876));
#39279=CARTESIAN_POINT('Ctrl Pts',(60.50786781033,7.34720186618502,-2.07223604970431));
#39280=CARTESIAN_POINT('Ctrl Pts',(60.706379414772,5.72726502447374,5.04717473915921));
#39281=CARTESIAN_POINT('Ctrl Pts',(60.9048910192142,-1.14563122034757,7.54758117738868));
#39282=CARTESIAN_POINT('Ctrl Pts',(61.0703173562493,-5.97524269785684,3.87132916275642));
#39283=CARTESIAN_POINT('Ctrl Pts',(61.2026584258773,-6.69970521934169,-0.511849504432479));
#39284=CARTESIAN_POINT('Ctrl Pts',(61.3019142280984,-5.65665605067822,-3.66203477929179));
#39285=CARTESIAN_POINT('Ctrl Pts',(61.4011700303195,-3.20943723603463,-5.90318156329419));
#39286=CARTESIAN_POINT('Ctrl Pts',(61.5335110999475,1.08625149890279,-7.03638916389873));
#39287=CARTESIAN_POINT('Ctrl Pts',(61.6989374369826,6.4173395489619,-4.1347558133022));
#39288=CARTESIAN_POINT('Ctrl Pts',(61.8974490414248,6.94933768253574,3.15946882913184));
#39289=CARTESIAN_POINT('Ctrl Pts',(62.0959606458668,1.11680434293635,7.55170746042015));
#39290=CARTESIAN_POINT('Ctrl Pts',(62.2944722503089,-5.74661976777159,5.025416775449));
#39291=CARTESIAN_POINT('Ctrl Pts',(62.4598985873441,-7.06265532099699,-0.899785864244022));
#39292=CARTESIAN_POINT('Ctrl Pts',(62.5922396569721,-4.78688086854931,-4.71527427532892));
#39293=CARTESIAN_POINT('Ctrl Pts',(62.6914954591932,-1.95691106368252,-6.44815907753943));
#39294=CARTESIAN_POINT('Ctrl Pts',(62.7907512614142,1.35882897202167,-6.58039693073728));
#39295=CARTESIAN_POINT('Ctrl Pts',(62.9230923310424,5.37131667820771,-4.67329347752821));
#39296=CARTESIAN_POINT('Ctrl Pts',(63.0885186680773,7.57035878608015,0.983931081085398));
#39297=CARTESIAN_POINT('Ctrl Pts',(63.2870302725196,3.26864597700691,6.89865863665999));
#39298=CARTESIAN_POINT('Ctrl Pts',(63.4855418769615,-4.02122834632787,6.48885660920751));
#39299=CARTESIAN_POINT('Ctrl Pts',(63.6840534814038,-7.63293788281372,0.129274125075791));
#39300=CARTESIAN_POINT('Ctrl Pts',(63.8494798184388,-4.81370981556546,-5.24584717621744));
#39301=CARTESIAN_POINT('Ctrl Pts',(63.9818208880669,-0.612761272495992,
-6.6912303475662));
#39302=CARTESIAN_POINT('Ctrl Pts',(64.0810766902879,2.66726755874743,-6.18820977104621));
#39303=CARTESIAN_POINT('Ctrl Pts',(64.180332492509,5.28519211669809,-4.14907028511851));
#39304=CARTESIAN_POINT('Ctrl Pts',(64.3126735621372,7.11900246605432,-0.102560582161132));
#39305=CARTESIAN_POINT('Ctrl Pts',(64.4780998991721,5.14718367076357,5.63781453949438));
#39306=CARTESIAN_POINT('Ctrl Pts',(64.6766115036143,-1.95613546236265,7.37896141479572));
#39307=CARTESIAN_POINT('Ctrl Pts',(64.8751231080564,-7.25965567891763,2.36070687120159));
#39308=CARTESIAN_POINT('Ctrl Pts',(65.0736347124985,-5.91349963671721,-4.82793688534368));
#39309=CARTESIAN_POINT('Ctrl Pts',(65.2390610495336,-0.290795223183368,
-7.11380017450725));
#39310=CARTESIAN_POINT('Ctrl Pts',(65.3714021191617,3.8508232569948,-5.50628733219841));
#39311=CARTESIAN_POINT('Ctrl Pts',(65.4706579213827,6.03144418528739,-3.00498543092064));
#39312=CARTESIAN_POINT('Ctrl Pts',(65.5699137236038,6.71486062202045,0.242253520557295));
#39313=CARTESIAN_POINT('Ctrl Pts',(65.7022547932319,5.50371205506531,4.51662134784635));
#39314=CARTESIAN_POINT('Ctrl Pts',(65.8676811302669,0.292508319573518,7.62842653525906));
#39315=CARTESIAN_POINT('Ctrl Pts',(66.0661927347091,-6.25684965601425,4.37348486821448));
#39316=CARTESIAN_POINT('Ctrl Pts',(66.2647043391512,-7.06866303628636,-2.88262734106105));
#39317=CARTESIAN_POINT('Ctrl Pts',(66.4632159435933,-1.40055785934149,-7.50445802153318));
#39318=CARTESIAN_POINT('Ctrl Pts',(66.6286422806284,4.36948937605636,-5.62123450789267));
#39319=CARTESIAN_POINT('Ctrl Pts',(66.7609833502565,6.49530082234867,-1.72020555609331));
#39320=CARTESIAN_POINT('Ctrl Pts',(66.8602391524775,6.54640094903262,1.59777690035313));
#39321=CARTESIAN_POINT('Ctrl Pts',(66.9594949546986,4.97246723013121,4.51913814934136));
#39322=CARTESIAN_POINT('Ctrl Pts',(67.0918360243266,1.28849943663799,7.00217707764802));
#39323=CARTESIAN_POINT('Ctrl Pts',(67.2572623613617,-4.70034630644326,6.01541333026384));
#39324=CARTESIAN_POINT('Ctrl Pts',(67.4557739658039,-7.60186370645468,-0.698001051142927));
#39325=CARTESIAN_POINT('Ctrl Pts',(67.654285570246,-3.53847428970454,-6.76422474536313));
#39326=CARTESIAN_POINT('Ctrl Pts',(67.852797174688,3.77399953920919,-6.63591610496366));
#39327=CARTESIAN_POINT('Ctrl Pts',(68.0182235117233,6.96565197102557,-1.47322942045928));
#39328=CARTESIAN_POINT('Ctrl Pts',(68.1505645813511,6.07143546137237,2.87849114407054));
#39329=CARTESIAN_POINT('Ctrl Pts',(68.2498203835724,3.96887483637101,5.44575935501849));
#39330=CARTESIAN_POINT('Ctrl Pts',(68.3490761857933,0.881109338758424,6.66120614223146));
#39331=CARTESIAN_POINT('Ctrl Pts',(68.4814172554215,-3.53539445446629,6.17994755252381));
#39332=CARTESIAN_POINT('Ctrl Pts',(68.6468435924565,-7.47278110162834,1.56074642543637));
#39333=CARTESIAN_POINT('Ctrl Pts',(68.8453551968986,-5.35580568311857,-5.43974407142979));
#39334=CARTESIAN_POINT('Ctrl Pts',(69.0438668013406,1.6632787956131,-7.45046150502356));
#39335=CARTESIAN_POINT('Ctrl Pts',(69.242378405783,7.16572282166079,-2.63256464231793));
#39336=CARTESIAN_POINT('Ctrl Pts',(69.4078047428178,6.27131232510135,3.37064950491412));
#39337=CARTESIAN_POINT('Ctrl Pts',(69.5401458124461,2.77941377570154,6.11750475464112));
#39338=CARTESIAN_POINT('Ctrl Pts',(69.639401614667,-0.483427260097334,6.72097830381911));
#39339=CARTESIAN_POINT('Ctrl Pts',(69.7386574168881,-3.62666022552501,5.6569603321232));
#39340=CARTESIAN_POINT('Ctrl Pts',(69.8709984865162,-6.68879787400515,2.43747746055645));
#39341=CARTESIAN_POINT('Ctrl Pts',(70.0364248235513,-6.71591205222224,-3.62943820858347));
#39342=CARTESIAN_POINT('Ctrl Pts',(70.2349364279934,-0.57837423373233,-7.61472297301591));
#39343=CARTESIAN_POINT('Ctrl Pts',(70.4334480324355,6.07689073543469,-4.61176722374836));
#39344=CARTESIAN_POINT('Ctrl Pts',(70.6319596368776,7.17705138752177,2.60408556382735));
#39345=CARTESIAN_POINT('Ctrl Pts',(70.8304712413198,1.69293223737595,7.44540855735987));
#39346=CARTESIAN_POINT('Ctrl Pts',(70.9958975783548,-4.15224483306629,5.78576453575111));
#39347=CARTESIAN_POINT('Ctrl Pts',(71.128238647983,-6.41601391396102,1.9731352289123));
#39348=CARTESIAN_POINT('Ctrl Pts',(71.2605797176109,-6.68463811960246,-2.44961921254678));
#39349=CARTESIAN_POINT('Ctrl Pts',(71.4260060546462,-2.78893611703176,-7.11224532601399));
#39350=CARTESIAN_POINT('Ctrl Pts',(71.6245176590881,4.47967320795655,-6.18354439128806));
#39351=CARTESIAN_POINT('Ctrl Pts',(71.7899439961234,7.08222387658641,-0.70626625924099));
#39352=CARTESIAN_POINT('Ctrl Pts',(71.9222850657513,5.72278531268991,3.52328110221862));
#39353=CARTESIAN_POINT('Ctrl Pts',(72.0215408679725,3.35124036184121,5.84559059835005));
#39354=CARTESIAN_POINT('Ctrl Pts',(72.1207966701934,0.150326486829087,6.71764568719649));
#39355=CARTESIAN_POINT('Ctrl Pts',(72.2531377398217,-4.18792723744534,5.75785783169036));
#39356=CARTESIAN_POINT('Ctrl Pts',(72.4185640768566,-7.59823771737176,0.737245998958156));
#39357=CARTESIAN_POINT('Ctrl Pts',(72.6170756812988,-4.73124216678028,-5.99096554247927));
#39358=CARTESIAN_POINT('Ctrl Pts',(72.8155872857409,2.46521529949203,-7.22483627642068));
#39359=CARTESIAN_POINT('Ctrl Pts',(73.014098890183,7.40991079793194,-1.83614083239068));
#39360=CARTESIAN_POINT('Ctrl Pts',(73.1795252272181,5.86666851215432,4.03398688832659));
#39361=CARTESIAN_POINT('Ctrl Pts',(73.3118662968462,2.09633824391537,6.38383659653893));
#39362=CARTESIAN_POINT('Ctrl Pts',(73.4111220990671,-1.21300002147258,6.62849090958169));
#39363=CARTESIAN_POINT('Ctrl Pts',(73.5103779012884,-4.22124101151322,5.22773083917127));
#39364=CARTESIAN_POINT('Ctrl Pts',(73.6427189709162,-6.91504415087427,1.6949540826346));
#39365=CARTESIAN_POINT('Ctrl Pts',(73.8081453079515,-6.27947547325658,-4.34127251565845));
#39366=CARTESIAN_POINT('Ctrl Pts',(74.0066569123935,0.253162974219424,-7.62964252307557));
#39367=CARTESIAN_POINT('Ctrl Pts',(74.2051685168357,6.54618845205212,-3.92720676581047));
#39368=CARTESIAN_POINT('Ctrl Pts',(74.4036801212777,6.84485808874247,3.38029161791993));
#39369=CARTESIAN_POINT('Ctrl Pts',(74.5691064583128,1.87723757943772,6.86780121746246));
#39370=CARTESIAN_POINT('Ctrl Pts',(74.7014475279409,-2.51925332864382,6.22907718612626));
#39371=CARTESIAN_POINT('Ctrl Pts',(74.8007033301619,-5.20485110658452,4.27992773619665));
#39372=CARTESIAN_POINT('Ctrl Pts',(74.8999591323831,-6.5984321743934,1.26835828159773));
#39373=CARTESIAN_POINT('Ctrl Pts',(75.0323002020111,-6.37573831885696,-3.16870252903819));
#39374=CARTESIAN_POINT('Ctrl Pts',(75.1977265390462,-1.99420833105789,-7.36896096068155));
#39375=CARTESIAN_POINT('Ctrl Pts',(75.3962381434883,5.11791631823011,-5.66413895152702));
#39376=CARTESIAN_POINT('Ctrl Pts',(75.5947497479304,7.53481155985735,1.22562321815919));
#39377=CARTESIAN_POINT('Ctrl Pts',(75.7932613523725,3.04631414056803,6.99988733311835));
#39378=CARTESIAN_POINT('Ctrl Pts',(75.9586876894077,-2.9989802314213,6.45730844516487));
#39379=CARTESIAN_POINT('Ctrl Pts',(76.0910287590357,-5.94476836125033,3.13173579232941));
#39380=CARTESIAN_POINT('Ctrl Pts',(76.1902845612568,-6.73795781621743,-0.0904481444383849));
#39381=CARTESIAN_POINT('Ctrl Pts',(76.2895403634778,-5.85856266362047,-3.29017985190923));
#39382=CARTESIAN_POINT('Ctrl Pts',(76.4218814331059,-2.82456925905874,-6.53548187093887));
#39383=CARTESIAN_POINT('Ctrl Pts',(76.587307770141,3.23311102121609,-6.91559438130846));
#39384=CARTESIAN_POINT('Ctrl Pts',(76.7858193745831,7.56499538095572,-1.02292834271609));
#39385=CARTESIAN_POINT('Ctrl Pts',(76.9843309790252,4.96403250061669,5.79947573845812));
#39386=CARTESIAN_POINT('Ctrl Pts',(77.1828425834674,-2.19129117565982,7.31277618321408));
#39387=CARTESIAN_POINT('Ctrl Pts',(77.3482689205024,-6.45849690590605,2.99641994738856));
#39388=CARTESIAN_POINT('Ctrl Pts',(77.4806099901305,-6.56200867841511,-1.44501973884905));
#39389=CARTESIAN_POINT('Ctrl Pts',(77.5798657923516,-5.08809165731427,-4.41809683995133));
#39390=CARTESIAN_POINT('Ctrl Pts',(77.6791215945725,-2.35114153022991,-6.2944557704451));
#39391=CARTESIAN_POINT('Ctrl Pts',(77.8114626642008,2.06091022055313,-6.81493681904093));
#39392=CARTESIAN_POINT('Ctrl Pts',(77.9768890012357,6.93312715195307,-3.19534042273405));
#39393=CARTESIAN_POINT('Ctrl Pts',(78.1754006056779,6.43841373241497,4.10150778597543));
#39394=CARTESIAN_POINT('Ctrl Pts',(78.3739122101199,0.0482727750496181,
7.63368896716102));
#39395=CARTESIAN_POINT('Ctrl Pts',(78.5724238145622,-6.39374302739908,4.17115123459849));
#39396=CARTESIAN_POINT('Ctrl Pts',(78.7378501515971,-6.86705644430124,-1.87996025901627));
#39397=CARTESIAN_POINT('Ctrl Pts',(78.8701912212254,-4.07939348819663,-5.33915617955881));
#39398=CARTESIAN_POINT('Ctrl Pts',(78.9694470234462,-1.0346399928902,-6.6586617638629));
#39399=CARTESIAN_POINT('Ctrl Pts',(79.0687028256675,2.26694546453617,-6.32526665067021));
#39400=CARTESIAN_POINT('Ctrl Pts',(79.2010438952954,5.97282745565348,-3.87505444731962));
#39401=CARTESIAN_POINT('Ctrl Pts',(79.3664702323306,7.35797352307912,2.03437414355709));
#39402=CARTESIAN_POINT('Ctrl Pts',(79.5649818367726,2.27036212464169,7.28841500815914));
#39403=CARTESIAN_POINT('Ctrl Pts',(79.7634934412148,-4.89029073438004,5.86179102675996));
#39404=CARTESIAN_POINT('Ctrl Pts',(79.9620050456568,-7.57582710640418,-0.940901788806087));
#39405=CARTESIAN_POINT('Ctrl Pts',(80.127431382692,-4.03165764889719,-5.86825795162323));
#39406=CARTESIAN_POINT('Ctrl Pts',(80.25977245232,0.330303940273858,-6.71110566511225));
#39407=CARTESIAN_POINT('Ctrl Pts',(80.3590282545411,3.50756970849505,-5.75371281352009));
#39408=CARTESIAN_POINT('Ctrl Pts',(80.4582840567622,5.81414033957109,-3.36805760833066));
#39409=CARTESIAN_POINT('Ctrl Pts',(80.5906251263901,7.06321503561394,0.895381564126428));
#39410=CARTESIAN_POINT('Ctrl Pts',(80.7560514634254,4.30695512977908,6.30306195688861));
#39411=CARTESIAN_POINT('Ctrl Pts',(80.9545630678673,-2.9701956136278,7.03231651200037));
#39412=CARTESIAN_POINT('Ctrl Pts',(81.1530746723096,-7.51870876718994,1.32081640751017));
#39413=CARTESIAN_POINT('Ctrl Pts',(81.3515862767517,-5.17913362961361,-5.60847816871138));
#39414=CARTESIAN_POINT('Ctrl Pts',(81.5170126137868,0.70827324628638,-7.08442402692663));
#39415=CARTESIAN_POINT('Ctrl Pts',(81.6493536834148,4.58396766952698,-4.91276707630163));
#39416=CARTESIAN_POINT('Ctrl Pts',(81.7486094856359,6.39282346674118,-2.13074271640208));
#39417=CARTESIAN_POINT('Ctrl Pts',(81.8478652878569,6.61476844885798,1.18020265601094));
#39418=CARTESIAN_POINT('Ctrl Pts',(81.980206357485,4.81698008100702,5.24284442682424));
#39419=CARTESIAN_POINT('Ctrl Pts',(82.1456326945201,-0.77864432454375,7.59421921846892));
#39420=CARTESIAN_POINT('Ctrl Pts',(82.3441442989622,-6.80764986905927,3.45419176776045));
#39421=CARTESIAN_POINT('Ctrl Pts',(82.5426559034044,-6.59533162217188,-3.84410435625081));
#39422=CARTESIAN_POINT('Ctrl Pts',(82.7411675078464,-0.33584693840556,-7.62664142045963));
#39423=CARTESIAN_POINT('Ctrl Pts',(82.9065938448816,5.11361989587141,-4.95394856102158));
#39424=CARTESIAN_POINT('Ctrl Pts',(83.0389349145096,6.67219119247864,-0.793665315024038));
#39425=CARTESIAN_POINT('Ctrl Pts',(83.1381907167307,6.25814384746915,2.4987780983516));
#39426=CARTESIAN_POINT('Ctrl Pts',(83.2374465189517,4.29061763578174,5.17094191079159));
#39427=CARTESIAN_POINT('Ctrl Pts',(83.3697875885797,0.295231184688071,7.11361745754488));
#39428=CARTESIAN_POINT('Ctrl Pts',(83.5352139256149,-5.49641663689415,5.29791059531774));
#39429=CARTESIAN_POINT('Ctrl Pts',(83.7337255300571,-7.42920911831907,-1.75567348457842));
#39430=CARTESIAN_POINT('Ctrl Pts',(83.9322371344991,-2.55635740096063,-7.19309212694518));
#39431=CARTESIAN_POINT('Ctrl Pts',(84.1307487389412,4.6660919327514,-6.04202272400717));
#39432=CARTESIAN_POINT('Ctrl Pts',(84.2961750759763,7.10332164554252,-0.483256023931992));
#39433=CARTESIAN_POINT('Ctrl Pts',(84.4285161456044,5.60850961619246,3.70035941853477));
#39434=CARTESIAN_POINT('Ctrl Pts',(84.5277719478254,3.16715273537929,5.94789037820946));
#39435=CARTESIAN_POINT('Ctrl Pts',(84.6270277500466,-0.0603964992484957,
6.71895767244744));
#39436=CARTESIAN_POINT('Ctrl Pts',(84.7593688196744,-4.3659832409641,5.62395813678596));
#39437=CARTESIAN_POINT('Ctrl Pts',(84.9247951567098,-7.61771305015897,0.498899195976315));
#39438=CARTESIAN_POINT('Ctrl Pts',(85.1233067611518,-4.54125231388254,-6.1361685871416));
#39439=CARTESIAN_POINT('Ctrl Pts',(85.3218183655939,2.69022548959542,-7.14410416520489));
#39440=CARTESIAN_POINT('Ctrl Pts',(85.5203299700359,7.46379556362782,-1.60318692193913));
#39441=CARTESIAN_POINT('Ctrl Pts',(85.6857563070712,5.73745472665523,4.2157239051296));
#39442=CARTESIAN_POINT('Ctrl Pts',(85.8180973766991,1.89540005613835,6.44635544850367));
#39443=CARTESIAN_POINT('Ctrl Pts',(85.9173531789203,-1.41998328154509,6.58725313621316));
#39444=CARTESIAN_POINT('Ctrl Pts',(86.0166089811413,-4.38287967219087,5.09297611621711));
#39445=CARTESIAN_POINT('Ctrl Pts',(86.1489500507694,-6.9647320622293,1.47757303916075));
#39446=CARTESIAN_POINT('Ctrl Pts',(86.3143763878045,-6.14044522647656,-4.53578934067139));
#39447=CARTESIAN_POINT('Ctrl Pts',(86.5128879922466,0.491966206253473,-7.61797261481501));
#39448=CARTESIAN_POINT('Ctrl Pts',(86.7113995966886,6.66596118855492,-3.72028210500849));
#39449=CARTESIAN_POINT('Ctrl Pts',(86.9099112011309,6.73564470112767,3.59298524662677));
#39450=CARTESIAN_POINT('Ctrl Pts',(87.0753375381658,1.66124688858446,6.92321988383066));
#39451=CARTESIAN_POINT('Ctrl Pts',(87.207678607794,-2.71308568989366,6.14712989781052));
#39452=CARTESIAN_POINT('Ctrl Pts',(87.306934410015,-5.33632728774559,4.11483504875706));
#39453=CARTESIAN_POINT('Ctrl Pts',(87.4061902122361,-6.63491546291512,1.06110166394744));
#39454=CARTESIAN_POINT('Ctrl Pts',(87.5385312818642,-6.27338114436937,-3.36680914252208));
#39455=CARTESIAN_POINT('Ctrl Pts',(87.7039576188991,-1.76246606785234,-7.42779683903485));
#39456=CARTESIAN_POINT('Ctrl Pts',(87.9024692233414,5.29278269392219,-5.50108978867694));
#39457=CARTESIAN_POINT('Ctrl Pts',(88.1009808277834,7.49273480662979,1.46098002234296));
#39458=CARTESIAN_POINT('Ctrl Pts',(88.2994924322256,2.82561366348029,7.09185165856283));
#39459=CARTESIAN_POINT('Ctrl Pts',(88.4649187692607,-3.19972451338524,6.36022623993376));
#39460=CARTESIAN_POINT('Ctrl Pts',(88.5972598388888,-6.03992521597272,2.94403521152833));
#39461=CARTESIAN_POINT('Ctrl Pts',(88.6965156411097,-6.73182069116263,-0.301407668203426));
#39462=CARTESIAN_POINT('Ctrl Pts',(88.7957714433308,-5.75265499663935,-3.47203116790483));
#39463=CARTESIAN_POINT('Ctrl Pts',(88.928112512959,-2.61852072146245,-6.6207298703369));
#39464=CARTESIAN_POINT('Ctrl Pts',(89.0935388499939,3.44809201818041,-6.81095543638831));
#39465=CARTESIAN_POINT('Ctrl Pts',(89.2920504544363,7.59331879679955,-0.785523493179886));
#39466=CARTESIAN_POINT('Ctrl Pts',(89.4905620588782,4.77998319783827,5.9520835122292));
#39467=CARTESIAN_POINT('Ctrl Pts',(89.6890736633205,-2.41922116762525,7.24056775843034));
#39468=CARTESIAN_POINT('Ctrl Pts',(89.8545000003553,-6.54916428819377,2.792697962714));
#39469=CARTESIAN_POINT('Ctrl Pts',(89.9868410699836,-6.5135384872794,-1.64980493270938));
#39470=CARTESIAN_POINT('Ctrl Pts',(90.0860968722044,-4.94724035994962,-4.57526712021312));
#39471=CARTESIAN_POINT('Ctrl Pts',(90.1853526744257,-2.15287309025503,-6.3649962606837));
#39472=CARTESIAN_POINT('Ctrl Pts',(90.3176937440536,2.27331396916941,-6.7470555342519));
#39473=CARTESIAN_POINT('Ctrl Pts',(90.4831200810889,7.0297910830573,-2.97665749640009));
#39474=CARTESIAN_POINT('Ctrl Pts',(90.6816316855308,6.3068143690113,4.30111962435357));
#39475=CARTESIAN_POINT('Ctrl Pts',(90.8801432899731,-0.190805235875399,
7.63145666764416));
#39476=CARTESIAN_POINT('Ctrl Pts',(91.078654894415,-6.52122970457174,3.96888090807952));
#39477=CARTESIAN_POINT('Ctrl Pts',(91.2440812314504,-6.80481617230556,-2.09408491848547));
#39478=CARTESIAN_POINT('Ctrl Pts',(91.3764223010781,-3.91019329323491,-5.46428662780449));
#39479=CARTESIAN_POINT('Ctrl Pts',(91.4756781032995,-0.825611873513067,
-6.68779645583891));
#39480=CARTESIAN_POINT('Ctrl Pts',(91.5749339055203,2.46391379626772,-6.25117338951843));
#39481=CARTESIAN_POINT('Ctrl Pts',(91.7072749751485,6.09124809477092,-3.68611061047414));
#39482=CARTESIAN_POINT('Ctrl Pts',(91.8727013121836,7.29065689809534,2.26379648302618));
#39483=CARTESIAN_POINT('Ctrl Pts',(92.0712129166257,2.04100677136742,7.35593834037501));
#39484=CARTESIAN_POINT('Ctrl Pts',(92.2697245210678,-5.07145836342535,5.70577317952703));
#39485=CARTESIAN_POINT('Ctrl Pts',(92.4682361255099,-7.54264648894489,-1.17768266740843));
#39486=CARTESIAN_POINT('Ctrl Pts',(92.633662462545,-3.84591167244496,-5.99163401689822));
#39487=CARTESIAN_POINT('Ctrl Pts',(92.7660035321731,0.5403049311133,-6.69747045702155));
#39488=CARTESIAN_POINT('Ctrl Pts',(92.8652593343941,3.68603095739406,-5.64104885473879));
#39489=CARTESIAN_POINT('Ctrl Pts',(92.9645151366152,5.9167618455322,-3.18433183015161));
#39490=CARTESIAN_POINT('Ctrl Pts',(93.0968562062433,7.03171133010858,1.11613196115961));
#39491=CARTESIAN_POINT('Ctrl Pts',(93.2622825432784,4.10745793875989,6.43484590364255));
#39492=CARTESIAN_POINT('Ctrl Pts',(93.4607941477204,-3.1889607948191,6.93585370068267));
#39493=CARTESIAN_POINT('Ctrl Pts',(93.6593057521627,-7.55638345874021,1.0847149545591));
#39494=CARTESIAN_POINT('Ctrl Pts',(93.8578173566046,-5.0009600521374,-5.76791566159161));
#39495=CARTESIAN_POINT('Ctrl Pts',(94.0232436936399,0.929779586353665,-7.05876934780418));
#39496=CARTESIAN_POINT('Ctrl Pts',(94.1555847632678,4.73556618481844,-4.76680740647929));
#39497=CARTESIAN_POINT('Ctrl Pts',(94.254840565489,6.45641376810642,-1.92950191899969));
#39498=CARTESIAN_POINT('Ctrl Pts',(94.35409636771,6.57456531439976,1.38676994052863));
#39499=CARTESIAN_POINT('Ctrl Pts',(94.4864374373379,4.65043420184241,5.39112015438664));
#39500=CARTESIAN_POINT('Ctrl Pts',(94.6518637743732,-1.01608074535405,7.56611078700463));
#39501=CARTESIAN_POINT('Ctrl Pts',(94.8503753788152,-6.91248145316082,3.23931129530254));
#39502=CARTESIAN_POINT('Ctrl Pts',(95.0488869832573,-6.47171606662027,-4.04875643392091));
#39503=CARTESIAN_POINT('Ctrl Pts',(95.2473985876995,-0.0968485836272764,
-7.63341816450247));
#39504=CARTESIAN_POINT('Ctrl Pts',(95.4128249247347,5.2662482667137,-4.79138226173144));
#39505=CARTESIAN_POINT('Ctrl Pts',(95.5451659943625,6.69377295745098,-0.5843316997734));
#39506=CARTESIAN_POINT('Ctrl Pts',(95.6444217965838,6.17682350529167,2.69353072841089));
#39507=CARTESIAN_POINT('Ctrl Pts',(95.7436775988047,4.12658159253324,5.302769493522));
#39508=CARTESIAN_POINT('Ctrl Pts',(95.8760186684327,0.0723184561547882,
7.11937390685444));
#39509=CARTESIAN_POINT('Ctrl Pts',(96.0414450054678,-5.65962867528661,5.12318804848898));
#39510=CARTESIAN_POINT('Ctrl Pts',(96.2399566099102,-7.37058526236216,-1.98746330743906));
#39511=CARTESIAN_POINT('Ctrl Pts',(96.438468214352,-2.32984688235236,-7.26961835401006));
#39512=CARTESIAN_POINT('Ctrl Pts',(96.6369798187944,4.85301360391685,-5.89293742394273));
#39513=CARTESIAN_POINT('Ctrl Pts',(96.8024061558294,7.11497127449493,-0.260573497908623));
#39514=CARTESIAN_POINT('Ctrl Pts',(96.9347472254574,5.4898795280518,3.87417897221335));
#39515=CARTESIAN_POINT('Ctrl Pts',(97.0340030276785,2.97933701591658,6.04415480824299));
#39516=CARTESIAN_POINT('Ctrl Pts',(97.1332588298996,-0.270775759182261,
6.71377095450099));
#39517=CARTESIAN_POINT('Ctrl Pts',(97.2655998995276,-4.53996011612904,5.48447599399042));
#39518=CARTESIAN_POINT('Ctrl Pts',(97.4310262365626,-7.62960026922674,0.26010046928489));
#39519=CARTESIAN_POINT('Ctrl Pts',(97.6295378410049,-4.34686659336538,-6.27537156889143));
#39520=CARTESIAN_POINT('Ctrl Pts',(97.8280494454467,2.91262869299278,-7.05635398806792));
#39521=CARTESIAN_POINT('Ctrl Pts',(98.0265610498892,7.51033981885591,-1.36866662398636));
#39522=CARTESIAN_POINT('Ctrl Pts',(98.1919873869241,5.60262239538359,4.39332870150253));
#39523=CARTESIAN_POINT('Ctrl Pts',(98.3243284565523,1.6925982925338,6.50254957392664));
#39524=CARTESIAN_POINT('Ctrl Pts',(98.4235842587731,-1.62557130264698,6.53955459801569));
#39525=CARTESIAN_POINT('Ctrl Pts',(98.5228400609944,-4.54022018521893,4.95322527359627));
#39526=CARTESIAN_POINT('Ctrl Pts',(98.6551811306222,-7.00758739956846,1.25874287370734));
#39527=CARTESIAN_POINT('Ctrl Pts',(98.8206074676577,-5.9953921716689,-4.72585708948102));
#39528=CARTESIAN_POINT('Ctrl Pts',(99.0191190720994,0.730287084624933,-7.59883006009458));
#39529=CARTESIAN_POINT('Ctrl Pts',(99.217630676542,6.77919507077474,-3.50970820732301));
#39530=CARTESIAN_POINT('Ctrl Pts',(99.4161422809837,6.61982429947142,3.80215449007985));
#39531=CARTESIAN_POINT('Ctrl Pts',(99.581568618019,1.44362662206756,6.9718474567906));
#39532=CARTESIAN_POINT('Ctrl Pts',(99.7139096876469,-2.90425673145911,6.0591528103388));
#39533=CARTESIAN_POINT('Ctrl Pts',(99.8131654898681,-5.46256900081922,3.94570605997287));
#39534=CARTESIAN_POINT('Ctrl Pts',(99.9124212920891,-6.6648904672555,0.85280419836499));
#39535=CARTESIAN_POINT('Ctrl Pts',(100.044762361717,-6.16487032672607,-3.5616132074317));
#39536=CARTESIAN_POINT('Ctrl Pts',(100.210188698752,-1.52899497570559,-7.4793466884865));
#39537=CARTESIAN_POINT('Ctrl Pts',(100.408700303195,5.46245730522718,-5.33264453125622));
#39538=CARTESIAN_POINT('Ctrl Pts',(100.607211907636,7.44330832695098,1.69490373122168));
#39539=CARTESIAN_POINT('Ctrl Pts',(100.805723512079,2.60214150270374,7.17685948881637));
#39540=CARTESIAN_POINT('Ctrl Pts',(100.971149849114,-3.39733014130829,6.25690520110843));
#39541=CARTESIAN_POINT('Ctrl Pts',(101.103490918742,-6.12915742481166,2.75344678596453));
#39542=CARTESIAN_POINT('Ctrl Pts',(101.202746720963,-6.71908023031374,-0.512071537018741));
#39543=CARTESIAN_POINT('Ctrl Pts',(101.302002523184,-5.64110447104782,-3.65047672064705));
#39544=CARTESIAN_POINT('Ctrl Pts',(101.434343592812,-2.40990364076523,-6.69948350448945));
#39545=CARTESIAN_POINT('Ctrl Pts',(101.599769929847,3.65969073412208,-6.69963553134705));
#39546=CARTESIAN_POINT('Ctrl Pts',(101.798281534289,7.6141938215129,-0.547348112814414));
#39547=CARTESIAN_POINT('Ctrl Pts',(101.996793138732,4.59124514361469,6.09885280519223));
#39548=CARTESIAN_POINT('Ctrl Pts',(102.195304743173,-2.6447781121808,7.16125696087193));
#39549=CARTESIAN_POINT('Ctrl Pts',(102.360731080209,-6.63340750490673,2.58623658209116));
#39550=CARTESIAN_POINT('Ctrl Pts',(102.493072149836,-6.45867907640749,-1.85297181015727));
#39551=CARTESIAN_POINT('Ctrl Pts',(102.592327952058,-4.80153624628457,-4.72794945785535));
#39552=CARTESIAN_POINT('Ctrl Pts',(102.691583754279,-1.95249286737386,-6.42929323830486));
#39553=CARTESIAN_POINT('Ctrl Pts',(102.823924823907,2.48348779276022,-6.67255596963564));
#39554=CARTESIAN_POINT('Ctrl Pts',(102.989351160942,7.11955939513445,-2.75505472567269));
#39555=CARTESIAN_POINT('Ctrl Pts',(103.187862765384,6.16902856441037,4.49651243516987));
#39556=CARTESIAN_POINT('Ctrl Pts',(103.386374369826,-0.429696083313257,
7.62173856703403));
#39557=CARTESIAN_POINT('Ctrl Pts',(103.584885974268,-6.642319617587,3.76271745153168));
#39558=CARTESIAN_POINT('Ctrl Pts',(103.750312311303,-6.73590096227615,-2.30615546116277));
#39559=CARTESIAN_POINT('Ctrl Pts',(103.882653380931,-3.73715753574226,-5.58405708195391));
#39560=CARTESIAN_POINT('Ctrl Pts',(103.981909183152,-0.615773900064327,
-6.71037099599149));
#39561=CARTESIAN_POINT('Ctrl Pts',(104.081164985373,2.65846524097796,-6.17094826625278));
#39562=CARTESIAN_POINT('Ctrl Pts',(104.213506055002,6.20369374461536,-3.49355101672159));
#39563=CARTESIAN_POINT('Ctrl Pts',(104.378932392037,7.21618876722331,2.49099823295448));
#39564=CARTESIAN_POINT('Ctrl Pts',(104.577443996479,1.80964936637775,7.41624613180053));
#39565=CARTESIAN_POINT('Ctrl Pts',(104.775955600921,-5.24765132897221,5.54415845962204));
#39566=CARTESIAN_POINT('Ctrl Pts',(104.974467205363,-7.50206718560608,-1.41330833873472));
#39567=CARTESIAN_POINT('Ctrl Pts',(105.139893542398,-3.65639318803571,-6.10913280942983));
#39568=CARTESIAN_POINT('Ctrl Pts',(105.272234612026,0.749775929176509,-6.67726560261785));
#39569=CARTESIAN_POINT('Ctrl Pts',(105.371490414247,3.8608765281646,-5.52285152463062));
#39570=CARTESIAN_POINT('Ctrl Pts',(105.470746216468,6.01357951731961,-2.99748247611494));
#39571=CARTESIAN_POINT('Ctrl Pts',(105.603087286096,6.99331012387269,1.33578748391403));
#39572=CARTESIAN_POINT('Ctrl Pts',(105.768513623132,3.9039316817389,6.56031791313918));
#39573=CARTESIAN_POINT('Ctrl Pts',(105.967025227573,-3.40459787396335,6.83258726202722));
#39574=CARTESIAN_POINT('Ctrl Pts',(106.165536832016,-7.58664600136129,0.847549771001657));
#39575=CARTESIAN_POINT('Ctrl Pts',(106.364048436458,-4.8178809406568,-5.92169588117069));
#39576=CARTESIAN_POINT('Ctrl Pts',(106.529474773493,1.15037385181886,-7.02618964947138));
#39577=CARTESIAN_POINT('Ctrl Pts',(106.661815843121,4.88251957521103,-4.6161732723596));
#39578=CARTESIAN_POINT('Ctrl Pts',(106.761071645342,6.51367075904044,-1.72636546984731));
#39579=CARTESIAN_POINT('Ctrl Pts',(106.860327447563,6.52791332908397,1.59197142916921));
#39580=CARTESIAN_POINT('Ctrl Pts',(106.992668517191,4.47932614866,5.53411952875296));
#39581=CARTESIAN_POINT('Ctrl Pts',(107.158094854226,-1.25251946123205,7.53055645039344));
#39582=CARTESIAN_POINT('Ctrl Pts',(107.356606458668,-7.01053418130777,3.0212936021343));
#39583=CARTESIAN_POINT('Ctrl Pts',(107.555118063111,-6.34174919999383,-4.2495111512557));
#39584=CARTESIAN_POINT('Ctrl Pts',(107.753629667552,0.142238626393045,-7.63256099340945));
#39585=CARTESIAN_POINT('Ctrl Pts',(107.919056004588,5.41372170278917,-4.62437297999697));
#39586=CARTESIAN_POINT('Ctrl Pts',(108.051397074216,6.70877360903263,-0.374065744790461));
#39587=CARTESIAN_POINT('Ctrl Pts',(108.150652876437,6.08947724034344,2.88485671444533));
#39588=CARTESIAN_POINT('Ctrl Pts',(108.249908678658,3.9584365600631,5.43084385761433));
#39589=CARTESIAN_POINT('Ctrl Pts',(108.382249748286,-0.150530275064401,
7.1150135755553));
#39590=CARTESIAN_POINT('Ctrl Pts',(108.547676085321,-5.81759659987454,4.94987406613489));
#39591=CARTESIAN_POINT('Ctrl Pts',(108.746187689763,-7.30404329578078,-2.22825616357533));
#39592=CARTESIAN_POINT('Ctrl Pts',(108.911614026798,-2.97046704781651,-6.46879341979401));
#39593=CARTESIAN_POINT('Ctrl Pts',(109.043955096426,1.4759275490682,-6.55624346037556));
#39594=CARTESIAN_POINT('Ctrl Pts',(109.143210898647,4.43222131992785,-5.07069835199561));
#39595=CARTESIAN_POINT('Ctrl Pts',(109.242466700868,6.31884020592842,-2.32048750504607));
#39596=CARTESIAN_POINT('Ctrl Pts',(109.308637235682,6.54473344473606,-0.120973595496458));
#39597=CARTESIAN_POINT('Ctrl Pts',(109.341722503089,6.38817262844173,0.941409491315552));
#39598=CARTESIAN_POINT('Ctrl Pts',(31.067,-1.68325362372015,5.98713018070703));
#39599=CARTESIAN_POINT('Ctrl Pts',(31.100085267407,-2.67894146944392,5.70719720383451));
#39600=CARTESIAN_POINT('Ctrl Pts',(31.166255802221,-4.52416925940906,4.64399692160856));
#39601=CARTESIAN_POINT('Ctrl Pts',(31.2655116044422,-6.20083243674659,1.90406440993152));
#39602=CARTESIAN_POINT('Ctrl Pts',(31.3647674066631,-6.34501955724797,-1.27931918847895));
#39603=CARTESIAN_POINT('Ctrl Pts',(31.4971084762913,-4.52035937174355,-5.15463560703619));
#39604=CARTESIAN_POINT('Ctrl Pts',(31.6625348133263,0.911741987501496,-7.29827737450832));
#39605=CARTESIAN_POINT('Ctrl Pts',(31.8610464177685,6.63914845639706,-3.16971042113852));
#39606=CARTESIAN_POINT('Ctrl Pts',(32.0264727548036,6.31536279232879,2.66437234788271));
#39607=CARTESIAN_POINT('Ctrl Pts',(32.1588138244316,3.21934995423852,5.61536002384009));
#39608=CARTESIAN_POINT('Ctrl Pts',(32.2580696266527,0.14301869708689,6.4884091364757));
#39609=CARTESIAN_POINT('Ctrl Pts',(32.3573254288737,-2.96596409463713,5.75195268151558));
#39610=CARTESIAN_POINT('Ctrl Pts',(32.4896664985018,-6.19418404416841,2.9425316853334));
#39611=CARTESIAN_POINT('Ctrl Pts',(32.6550928355369,-6.76718021184908,-2.87509801732424));
#39612=CARTESIAN_POINT('Ctrl Pts',(32.853604439979,-1.24379023624101,-7.2466418339485));
#39613=CARTESIAN_POINT('Ctrl Pts',(33.0521160444211,5.41227178463782,-4.97673046693937));
#39614=CARTESIAN_POINT('Ctrl Pts',(33.2506276488633,7.11391162562153,1.85873863792625));
#39615=CARTESIAN_POINT('Ctrl Pts',(33.4160539858983,3.10541110519021,6.11397050225541));
#39616=CARTESIAN_POINT('Ctrl Pts',(33.5483950555264,-1.16614656773419,6.36572295470293));
#39617=CARTESIAN_POINT('Ctrl Pts',(33.6476508577475,-4.07834394078075,5.04884480068));
#39618=CARTESIAN_POINT('Ctrl Pts',(33.7469066599685,-5.97817189517101,2.47867161336443));
#39619=CARTESIAN_POINT('Ctrl Pts',(33.8792477295966,-6.6302737442775,-1.75030082377511));
#39620=CARTESIAN_POINT('Ctrl Pts',(34.0446740666317,-3.31312753510712,-6.56400641995886));
#39621=CARTESIAN_POINT('Ctrl Pts',(34.2431856710738,3.72736559794809,-6.33774649263565));
#39622=CARTESIAN_POINT('Ctrl Pts',(34.4416972755159,7.34611894960073,-0.307926448941118));
#39623=CARTESIAN_POINT('Ctrl Pts',(34.640208879958,4.233914906245,6.01140200914276));
#39624=CARTESIAN_POINT('Ctrl Pts',(34.8056352169931,-1.57434350116745,6.67424438783693));
#39625=CARTESIAN_POINT('Ctrl Pts',(34.9379762866212,-4.99945699673356,4.10947315312662));
#39626=CARTESIAN_POINT('Ctrl Pts',(35.0372320888423,-6.37382702555459,1.22395397566176));
#39627=CARTESIAN_POINT('Ctrl Pts',(35.1364878910633,-6.16600174500198,-1.96539115710818));
#39628=CARTESIAN_POINT('Ctrl Pts',(35.2688289606914,-3.93449142709178,-5.61639323287909));
#39629=CARTESIAN_POINT('Ctrl Pts',(35.4342552977265,1.706159430506,-7.15206323045347));
#39630=CARTESIAN_POINT('Ctrl Pts',(35.6327669021685,6.93766837888352,-2.43496237142141));
#39631=CARTESIAN_POINT('Ctrl Pts',(35.8312785066107,5.80973766223456,4.50635469098045));
#39632=CARTESIAN_POINT('Ctrl Pts',(36.0297901110528,-0.646180895956555,
7.3243046569134));
#39633=CARTESIAN_POINT('Ctrl Pts',(36.1952164480879,-5.51037651268064,4.08164750837416));
#39634=CARTESIAN_POINT('Ctrl Pts',(36.3275575177159,-6.47105737915941,-0.0880703169200902));
#39635=CARTESIAN_POINT('Ctrl Pts',(36.426813319937,-5.65834786130082,-3.17912466680208));
#39636=CARTESIAN_POINT('Ctrl Pts',(36.526069122158,-3.44104873410895,-5.48101483247933));
#39637=CARTESIAN_POINT('Ctrl Pts',(36.6584101917862,0.619923098873849,-6.82933313338426));
#39638=CARTESIAN_POINT('Ctrl Pts',(36.8238365288212,5.919465903525,-4.36152632411429));
#39639=CARTESIAN_POINT('Ctrl Pts',(37.0223481332634,6.8706564039049,2.61808419966792));
#39640=CARTESIAN_POINT('Ctrl Pts',(37.2208597377055,1.52886927114417,7.19185949867951));
#39641=CARTESIAN_POINT('Ctrl Pts',(37.4193713421476,-5.22102444228719,5.17724755367456));
#39642=CARTESIAN_POINT('Ctrl Pts',(37.5847976791827,-6.84333909992013,-0.439096411762364));
#39643=CARTESIAN_POINT('Ctrl Pts',(37.7171387488107,-4.88576711085616,-4.2440098636368));
#39644=CARTESIAN_POINT('Ctrl Pts',(37.8163945510318,-2.26989742046013,-6.08040293629282));
#39645=CARTESIAN_POINT('Ctrl Pts',(37.9156503532528,0.909436095338548,-6.40743833155411));
#39646=CARTESIAN_POINT('Ctrl Pts',(38.0479914228809,4.88148948210039,-4.81613497853341));
#39647=CARTESIAN_POINT('Ctrl Pts',(38.213417759916,7.33645041645639,0.489370765242909));
#39648=CARTESIAN_POINT('Ctrl Pts',(38.4119293643581,3.55798549376158,6.43436271305828));
#39649=CARTESIAN_POINT('Ctrl Pts',(38.6104409688003,-3.4742282511699,6.47997086072042));
#39650=CARTESIAN_POINT('Ctrl Pts',(38.8089525732423,-7.32948579331351,0.584488207419706));
#39651=CARTESIAN_POINT('Ctrl Pts',(38.9743789102775,-4.94354729154295,-4.75241368902037));
#39652=CARTESIAN_POINT('Ctrl Pts',(39.1067199799055,-0.992468299979939,
-6.39510333440429));
#39653=CARTESIAN_POINT('Ctrl Pts',(39.2059757821266,2.19083962730784,-6.10933350657059));
#39654=CARTESIAN_POINT('Ctrl Pts',(39.3052315843476,4.83030849556222,-4.30702447425982));
#39655=CARTESIAN_POINT('Ctrl Pts',(39.4375726539757,6.83706805014439,-0.527822103558383));
#39656=CARTESIAN_POINT('Ctrl Pts',(39.6029989910108,5.28773755787813,5.10909189367368));
#39657=CARTESIAN_POINT('Ctrl Pts',(39.8015105954529,-1.43545748919326,7.2110849456744));
#39658=CARTESIAN_POINT('Ctrl Pts',(40.000022199895,-6.8361201447979,2.70698091291776));
#39659=CARTESIAN_POINT('Ctrl Pts',(40.1985338043371,-5.97553982112241,-4.28438003743567));
#39660=CARTESIAN_POINT('Ctrl Pts',(40.3639601413723,-0.708451912413997,
-6.82071782022295));
#39661=CARTESIAN_POINT('Ctrl Pts',(40.4963012110003,3.3696668804336,-5.52518643116073));
#39662=CARTESIAN_POINT('Ctrl Pts',(40.5955570132214,5.6166365191778,-3.25224974110642));
#39663=CARTESIAN_POINT('Ctrl Pts',(40.6948128154424,6.46937068698724,-0.17199679800523));
#39664=CARTESIAN_POINT('Ctrl Pts',(40.8271538850705,5.56285463090548,4.00983092545351));
#39665=CARTESIAN_POINT('Ctrl Pts',(40.9925802221055,0.741127608027151,7.3153071246269));
#39666=CARTESIAN_POINT('Ctrl Pts',(41.1910918265477,-5.75079853390819,4.58133174081647));
#39667=CARTESIAN_POINT('Ctrl Pts',(41.3896034309898,-6.96866783622726,-2.34477139298153));
#39668=CARTESIAN_POINT('Ctrl Pts',(41.5881150354319,-1.7987828877996,-7.12933156625193));
#39669=CARTESIAN_POINT('Ctrl Pts',(41.753541372467,3.86131211317401,-5.66695371958917));
#39670=CARTESIAN_POINT('Ctrl Pts',(41.8858824420951,6.13999062787377,-2.04520294195858));
#39671=CARTESIAN_POINT('Ctrl Pts',(41.9851382443162,6.38916632461915,1.14117826979005));
#39672=CARTESIAN_POINT('Ctrl Pts',(42.0843940465372,5.05233903023813,4.04428118553917));
#39673=CARTESIAN_POINT('Ctrl Pts',(42.2167351161653,1.66078038279294,6.65326267446582));
#39674=CARTESIAN_POINT('Ctrl Pts',(42.3821614532004,-4.15558680069482,6.06581295465727));
#39675=CARTESIAN_POINT('Ctrl Pts',(42.5806730576425,-7.34949512093008,-0.212616472640353));
#39676=CARTESIAN_POINT('Ctrl Pts',(42.7791846620846,-3.80925655132213,-6.2888670540267));
#39677=CARTESIAN_POINT('Ctrl Pts',(42.9776962665266,3.22770883173084,-6.60642748817874));
#39678=CARTESIAN_POINT('Ctrl Pts',(43.1431226035619,6.60701429937979,-1.83615297377451));
#39679=CARTESIAN_POINT('Ctrl Pts',(43.2754636731898,6.00981779016149,2.40092276286268));
#39680=CARTESIAN_POINT('Ctrl Pts',(43.3747194754109,4.14349036564128,4.9955201688039));
#39681=CARTESIAN_POINT('Ctrl Pts',(43.473975277632,1.24861120530404,6.35006378252714));
#39682=CARTESIAN_POINT('Ctrl Pts',(43.6063163472601,-3.02583705454058,6.15373104828925));
#39683=CARTESIAN_POINT('Ctrl Pts',(43.7717426842951,-7.08922568451271,1.95086330967669));
#39684=CARTESIAN_POINT('Ctrl Pts',(43.9702542887373,-5.47633209238865,-4.90612587597253));
#39685=CARTESIAN_POINT('Ctrl Pts',(44.1687658931793,1.14962582217418,-7.26213775454605));
#39686=CARTESIAN_POINT('Ctrl Pts',(44.3672774976215,6.72944929157678,-2.96268471003815));
#39687=CARTESIAN_POINT('Ctrl Pts',(44.5327038346566,6.2316005792506,2.86203597391672));
#39688=CARTESIAN_POINT('Ctrl Pts',(44.6650449042847,3.04064127406932,5.71286623566488));
#39689=CARTESIAN_POINT('Ctrl Pts',(44.7643007065057,-0.0595468312504839,
6.49000680600387));
#39690=CARTESIAN_POINT('Ctrl Pts',(44.8635565087267,-3.14495343806531,5.65611243316245));
#39691=CARTESIAN_POINT('Ctrl Pts',(44.9958975783549,-6.28306630941009,2.7472119406529));
#39692=CARTESIAN_POINT('Ctrl Pts',(45.1613239153899,-6.67395475143974,-3.08566304620775));
#39693=CARTESIAN_POINT('Ctrl Pts',(45.3598355198321,-1.01618098913832,-7.2820093720296));
#39694=CARTESIAN_POINT('Ctrl Pts',(45.5583471242741,5.56543150817819,-4.80481596159418));
#39695=CARTESIAN_POINT('Ctrl Pts',(45.7568587287163,7.05223625244414,2.08061344288397));
#39696=CARTESIAN_POINT('Ctrl Pts',(45.9222850657513,2.91241425495877,6.20821543624437));
#39697=CARTESIAN_POINT('Ctrl Pts',(46.0546261353794,-1.3649168534335,6.32608425231493));
#39698=CARTESIAN_POINT('Ctrl Pts',(46.1538819376005,-4.23445444437469,4.9186512099969));
#39699=CARTESIAN_POINT('Ctrl Pts',(46.2531377398215,-6.05285999815342,2.29024580054805));
#39700=CARTESIAN_POINT('Ctrl Pts',(46.3854788094496,-6.5722108424563,-1.957074433334));
#39701=CARTESIAN_POINT('Ctrl Pts',(46.5509051464847,-3.10594562392494,-6.66453976207049));
#39702=CARTESIAN_POINT('Ctrl Pts',(46.7494167509268,3.92400822288565,-6.21791313575052));
#39703=CARTESIAN_POINT('Ctrl Pts',(46.947928355369,7.35215906316875,-0.077726487626221));
#39704=CARTESIAN_POINT('Ctrl Pts',(47.146439959811,4.04358699335335,6.14104166132917));
#39705=CARTESIAN_POINT('Ctrl Pts',(47.3118662968462,-1.7825799675908,6.62166930271015));
#39706=CARTESIAN_POINT('Ctrl Pts',(47.4442073664742,-5.12569603706815,3.95089611604222));
#39707=CARTESIAN_POINT('Ctrl Pts',(47.5434631686953,-6.4090299071312,1.02375281029476));
#39708=CARTESIAN_POINT('Ctrl Pts',(47.6427189709163,-6.10142998607327,-2.15751989775753));
#39709=CARTESIAN_POINT('Ctrl Pts',(47.7750600405443,-3.756680423898,-5.73684999699412));
#39710=CARTESIAN_POINT('Ctrl Pts',(47.9404863775796,1.92929451774911,-7.09512587082007));
#39711=CARTESIAN_POINT('Ctrl Pts',(48.1389979820215,7.01051831056036,-2.21651016562319));
#39712=CARTESIAN_POINT('Ctrl Pts',(48.3375095864638,5.66576857146238,4.68608053618823));
#39713=CARTESIAN_POINT('Ctrl Pts',(48.5360211909057,-0.875229719861018,
7.30047679240671));
#39714=CARTESIAN_POINT('Ctrl Pts',(48.701447527941,-5.63549357111038,3.90708432277619));
#39715=CARTESIAN_POINT('Ctrl Pts',(48.833788597569,-6.46512562050092,-0.290672832091888));
#39716=CARTESIAN_POINT('Ctrl Pts',(48.93304439979,-5.55601616227824,-3.3547605833489));
#39717=CARTESIAN_POINT('Ctrl Pts',(49.0323002020111,-3.26771921629748,-5.58608549053932));
#39718=CARTESIAN_POINT('Ctrl Pts',(49.1646412716392,0.833484420250366,-6.80657031231661));
#39719=CARTESIAN_POINT('Ctrl Pts',(49.3300676086743,6.05314692292063,-4.17401494828823));
#39720=CARTESIAN_POINT('Ctrl Pts',(49.5285792131164,6.78529949630181,2.83195957642392));
#39721=CARTESIAN_POINT('Ctrl Pts',(49.7270908175584,1.30290129179695,7.23620981735928));
#39722=CARTESIAN_POINT('Ctrl Pts',(49.9256024220008,-5.38059290072692,5.0112082869947));
#39723=CARTESIAN_POINT('Ctrl Pts',(50.0910287590355,-6.82623212432137,-0.653185027532664));
#39724=CARTESIAN_POINT('Ctrl Pts',(50.2233698286639,-4.75046670097809,-4.39492959068425));
#39725=CARTESIAN_POINT('Ctrl Pts',(50.3226256308848,-2.07837204216358,-6.14850419382157));
#39726=CARTESIAN_POINT('Ctrl Pts',(50.4218814331059,1.10964349084127,-6.37581612873264));
#39727=CARTESIAN_POINT('Ctrl Pts',(50.554222502734,5.02991597370948,-4.66090559792109));
#39728=CARTESIAN_POINT('Ctrl Pts',(50.719648839769,7.31752721429885,0.718876851061941));
#39729=CARTESIAN_POINT('Ctrl Pts',(50.9181604442113,3.35474386460336,6.54262775189899));
#39730=CARTESIAN_POINT('Ctrl Pts',(51.1166720486532,-3.6754491338023,6.36799481484125));
#39731=CARTESIAN_POINT('Ctrl Pts',(51.3151836530955,-7.34419465547514,0.35467354213092));
#39732=CARTESIAN_POINT('Ctrl Pts',(51.4806099901304,-4.79229751986203,-4.90489349287364));
#39733=CARTESIAN_POINT('Ctrl Pts',(51.6129510597586,-0.791714381456252,
-6.42304665422641));
#39734=CARTESIAN_POINT('Ctrl Pts',(51.7122068619796,2.38108318749985,-6.03772945910084));
#39735=CARTESIAN_POINT('Ctrl Pts',(51.8114626642006,4.96281693597846,-4.15364755897021));
#39736=CARTESIAN_POINT('Ctrl Pts',(51.9438037338288,6.85024388311463,-0.313455638265433));
#39737=CARTESIAN_POINT('Ctrl Pts',(52.1092300708638,5.12514934704392,5.27217532234014));
#39738=CARTESIAN_POINT('Ctrl Pts',(52.307741675306,-1.66057365242597,7.16259585917574));
#39739=CARTESIAN_POINT('Ctrl Pts',(52.506253279748,-6.91753833237311,2.49157534848164));
#39740=CARTESIAN_POINT('Ctrl Pts',(52.7047648841903,-5.83844070433739,-4.46940696300231));
#39741=CARTESIAN_POINT('Ctrl Pts',(52.8701912212252,-0.494508874927136,
-6.83955822169301));
#39742=CARTESIAN_POINT('Ctrl Pts',(53.0025322908534,3.54103930044635,-5.41695307870284));
#39743=CARTESIAN_POINT('Ctrl Pts',(53.1017880930744,5.71572828749395,-3.07476573264209));
#39744=CARTESIAN_POINT('Ctrl Pts',(53.2010438952954,6.47158394013595,0.0306804489560287));
#39745=CARTESIAN_POINT('Ctrl Pts',(53.3333849649236,5.43455561682152,4.18206897874528));
#39746=CARTESIAN_POINT('Ctrl Pts',(53.4988113019586,0.511680132839369,7.33492821373557));
#39747=CARTESIAN_POINT('Ctrl Pts',(53.6973229064008,-5.89144563848159,4.39899449713555));
#39748=CARTESIAN_POINT('Ctrl Pts',(53.8958345108428,-6.8918218408794,-2.56185011477848));
#39749=CARTESIAN_POINT('Ctrl Pts',(54.094346115285,-1.57464063360658,-7.18216508679608));
#39750=CARTESIAN_POINT('Ctrl Pts',(54.2597724523201,4.03688294466771,-5.54325462037972));
#39751=CARTESIAN_POINT('Ctrl Pts',(54.3921135219481,6.20102619469151,-1.85192173617664));
#39752=CARTESIAN_POINT('Ctrl Pts',(54.4913693241692,6.35029591436066,1.34069980500598));
#39753=CARTESIAN_POINT('Ctrl Pts',(54.5906251263902,4.92321156794364,4.2005151876216));
#39754=CARTESIAN_POINT('Ctrl Pts',(54.7229661960184,1.45161424482283,6.70200804084397));
#39755=CARTESIAN_POINT('Ctrl Pts',(54.8883925330533,-4.34350386041609,5.93270281351995));
#39756=CARTESIAN_POINT('Ctrl Pts',(55.0869041374956,-7.339232276092,-0.442666798599518));
#39757=CARTESIAN_POINT('Ctrl Pts',(55.2854157419376,-3.61044798336259,-6.4050721819856));
#39758=CARTESIAN_POINT('Ctrl Pts',(55.4839273463797,3.43301069967906,-6.50210934965618));
#39759=CARTESIAN_POINT('Ctrl Pts',(55.6493536834148,6.66127426453652,-1.62834912347856));
#39760=CARTESIAN_POINT('Ctrl Pts',(55.7816947530429,5.93168364981801,2.58794688172988));
#39761=CARTESIAN_POINT('Ctrl Pts',(55.880950555264,3.98501993711935,5.12282639446718));
#39762=CARTESIAN_POINT('Ctrl Pts',(55.980206357485,1.04914210494851,6.38605048741379));
#39763=CARTESIAN_POINT('Ctrl Pts',(56.1125474271131,-3.21706142470918,6.05595669444211));
#39764=CARTESIAN_POINT('Ctrl Pts',(56.2779737641482,-7.14684138056117,1.72790241046636));
#39765=CARTESIAN_POINT('Ctrl Pts',(56.4764853685903,-5.32000740755992,-5.07521482112047));
#39766=CARTESIAN_POINT('Ctrl Pts',(56.6749969730323,1.3764809281104,-7.2225746483897));
#39767=CARTESIAN_POINT('Ctrl Pts',(56.8735085774746,6.81892734073127,-2.7504942066517));
#39768=CARTESIAN_POINT('Ctrl Pts',(57.0389349145096,6.13891757971937,3.05577922054628));
#39769=CARTESIAN_POINT('Ctrl Pts',(57.1712759841377,2.86024754923171,5.80528413958247));
#39770=CARTESIAN_POINT('Ctrl Pts',(57.2705317863587,-0.262756750612794,
6.48495898653921));
#39771=CARTESIAN_POINT('Ctrl Pts',(57.3697875885798,-3.32053611010715,5.55485192652768));
#39772=CARTESIAN_POINT('Ctrl Pts',(57.5021286582079,-6.36601560896188,2.54910591419103));
#39773=CARTESIAN_POINT('Ctrl Pts',(57.6675549952429,-6.57405175731321,-3.29314924520042));
#39774=CARTESIAN_POINT('Ctrl Pts',(57.8660665996852,-0.787641354648353,
-7.31026028219656));
#39775=CARTESIAN_POINT('Ctrl Pts',(58.0645782041271,5.71316809273326,-4.6281740072287));
#39776=CARTESIAN_POINT('Ctrl Pts',(58.2630898085693,6.98362156225626,2.30043872645768));
#39777=CARTESIAN_POINT('Ctrl Pts',(58.4285161456044,2.71657121158352,6.29637487350503));
#39778=CARTESIAN_POINT('Ctrl Pts',(58.5608572152325,-1.56235319508776,6.28023825009631));
#39779=CARTESIAN_POINT('Ctrl Pts',(58.6601130174535,-4.38640864661985,4.78363390655549));
#39780=CARTESIAN_POINT('Ctrl Pts',(58.7593688196746,-6.1216119881301,2.09957296871427));
#39781=CARTESIAN_POINT('Ctrl Pts',(58.8917098893027,-6.50770029495222,-2.16192797437576));
#39782=CARTESIAN_POINT('Ctrl Pts',(59.0571362263377,-2.89571754477245,-6.75853596275806));
#39783=CARTESIAN_POINT('Ctrl Pts',(59.2556478307799,4.11680198598908,-6.09198044195556));
#39784=CARTESIAN_POINT('Ctrl Pts',(59.4541594352219,7.35098720564501,0.15254966226341));
#39785=CARTESIAN_POINT('Ctrl Pts',(59.6526710396641,3.84929275248138,6.26465751375856));
#39786=CARTESIAN_POINT('Ctrl Pts',(59.8180973766992,-1.98906791709047,6.56259891479826));
#39787=CARTESIAN_POINT('Ctrl Pts',(59.9504384463272,-5.24690719279156,3.7884435978916));
#39788=CARTESIAN_POINT('Ctrl Pts',(60.0496942485483,-6.43794609299798,0.822547427654274));
#39789=CARTESIAN_POINT('Ctrl Pts',(60.1489500507694,-6.03087324568868,-2.34753229554149));
#39790=CARTESIAN_POINT('Ctrl Pts',(60.2812911203974,-3.57518444437901,-5.85167940714288));
#39791=CARTESIAN_POINT('Ctrl Pts',(60.4467174574326,2.15053713527687,-7.03122880361549));
#39792=CARTESIAN_POINT('Ctrl Pts',(60.6452290618746,7.07649152718233,-1.99588375481379));
#39793=CARTESIAN_POINT('Ctrl Pts',(60.8437406663167,5.5162418506764,4.86120974057477));
#39794=CARTESIAN_POINT('Ctrl Pts',(61.0422522707589,-1.1034200191743,7.26948778940321));
#39795=CARTESIAN_POINT('Ctrl Pts',(61.207678607794,-5.75508269601921,3.72868862434105));
#39796=CARTESIAN_POINT('Ctrl Pts',(61.340019677422,-6.45285213102613,-0.492990222301885));
#39797=CARTESIAN_POINT('Ctrl Pts',(61.4392754796431,-5.448234490336,-3.52710576895582));
#39798=CARTESIAN_POINT('Ctrl Pts',(61.5385312818642,-3.09118434765655,-5.68567668030614));
#39799=CARTESIAN_POINT('Ctrl Pts',(61.6708723514922,1.04622816527626,-6.77713083254947));
#39800=CARTESIAN_POINT('Ctrl Pts',(61.8362986885273,6.18089032700829,-3.98240922363489));
#39801=CARTESIAN_POINT('Ctrl Pts',(62.0348102929695,6.69328679484465,3.04305704497484));
#39802=CARTESIAN_POINT('Ctrl Pts',(62.2333218974115,1.07565527860131,7.27346203802769));
#39803=CARTESIAN_POINT('Ctrl Pts',(62.4318335018537,-5.53488346138075,4.84025345699285));
#39804=CARTESIAN_POINT('Ctrl Pts',(62.5972598388888,-6.80242920348616,-0.866632925101025));
#39805=CARTESIAN_POINT('Ctrl Pts',(62.7296009085167,-4.61050649279502,-4.54153827068194));
#39806=CARTESIAN_POINT('Ctrl Pts',(62.828856710738,-1.88480796006642,-6.2105742987874));
#39807=CARTESIAN_POINT('Ctrl Pts',(62.9281125129588,1.30876242173983,-6.33793979993621));
#39808=CARTESIAN_POINT('Ctrl Pts',(63.0604535825871,5.17340855136809,-4.50110427072531));
#39809=CARTESIAN_POINT('Ctrl Pts',(63.225879919622,7.29142614877463,0.947677780663159));
#39810=CARTESIAN_POINT('Ctrl Pts',(63.4243915240643,3.14821152092017,6.64447503694298));
#39811=CARTESIAN_POINT('Ctrl Pts',(63.6229031285063,-3.87306471768808,6.24977231502176));
#39812=CARTESIAN_POINT('Ctrl Pts',(63.8214147329484,-7.35169949580919,0.124510972673139));
#39813=CARTESIAN_POINT('Ctrl Pts',(63.9868410699835,-4.63634691744933,-5.05256201905211));
#39814=CARTESIAN_POINT('Ctrl Pts',(64.1191821396116,-0.590183859376729,
-6.44468951899971));
#39815=CARTESIAN_POINT('Ctrl Pts',(64.2184379418327,2.56899111035366,-5.9602029195333));
#39816=CARTESIAN_POINT('Ctrl Pts',(64.3176937440537,5.09045728081569,-3.99619627350351));
#39817=CARTESIAN_POINT('Ctrl Pts',(64.4500348136817,6.85670021738249,-0.098781700014005));
#39818=CARTESIAN_POINT('Ctrl Pts',(64.615461150717,4.95753380652983,5.43008720152017));
#39819=CARTESIAN_POINT('Ctrl Pts',(64.8139727551589,-1.8840609360603,7.10708088361284));
#39820=CARTESIAN_POINT('Ctrl Pts',(65.0124843596012,-6.99217101119294,2.27372576342389));
#39821=CARTESIAN_POINT('Ctrl Pts',(65.2109959640432,-5.6956145805417,-4.65004978563959));
#39822=CARTESIAN_POINT('Ctrl Pts',(65.3764223010783,-0.280080766866481,
-6.8516896061695));
#39823=CARTESIAN_POINT('Ctrl Pts',(65.5087633707064,3.70893826617409,-5.30340616226556));
#39824=CARTESIAN_POINT('Ctrl Pts',(65.6080191729274,5.80921341909733,-2.89426564405251));
#39825=CARTESIAN_POINT('Ctrl Pts',(65.7072749751485,6.46744912735215,0.233327601020761));
#39826=CARTESIAN_POINT('Ctrl Pts',(65.8396160447766,5.30092577216001,4.35020478294281));
#39827=CARTESIAN_POINT('Ctrl Pts',(66.0050423818117,0.281730743593815,7.34735437050459));
#39828=CARTESIAN_POINT('Ctrl Pts',(66.2035539862537,-6.02631374284371,4.21234221923613));
#39829=CARTESIAN_POINT('Ctrl Pts',(66.402065590696,-6.80821556230926,-2.77641588274926));
#39830=CARTESIAN_POINT('Ctrl Pts',(66.6005771951379,-1.34895379295012,-7.22795352199158));
#39831=CARTESIAN_POINT('Ctrl Pts',(66.7660035321732,4.20849394244699,-5.41411806724503));
#39832=CARTESIAN_POINT('Ctrl Pts',(66.8983446018011,6.25597908877345,-1.65682395344729));
#39833=CARTESIAN_POINT('Ctrl Pts',(66.9976004040223,6.30519641260689,1.53890622628911));
#39834=CARTESIAN_POINT('Ctrl Pts',(67.0968562062432,4.78925485703138,4.35262885196658));
#39835=CARTESIAN_POINT('Ctrl Pts',(67.2291972758714,1.24102420380131,6.74417930312503));
#39836=CARTESIAN_POINT('Ctrl Pts',(67.3946236129065,-4.52716032826772,5.79377322678848));
#39837=CARTESIAN_POINT('Ctrl Pts',(67.5931352173485,-7.32177025883928,-0.672282947214057));
#39838=CARTESIAN_POINT('Ctrl Pts',(67.7916468217906,-3.40809791078333,-6.51499441152191));
#39839=CARTESIAN_POINT('Ctrl Pts',(67.9901584262328,3.63494514635811,-6.39141334988969));
#39840=CARTESIAN_POINT('Ctrl Pts',(68.1555847632678,6.70899997741019,-1.41894774382875));
#39841=CARTESIAN_POINT('Ctrl Pts',(68.2879258328959,5.84773120199377,2.77243208544916));
#39842=CARTESIAN_POINT('Ctrl Pts',(68.387181635117,3.82264019194717,5.24510836053448));
#39843=CARTESIAN_POINT('Ctrl Pts',(68.486437437338,0.848644543025793,6.4157715664878));
#39844=CARTESIAN_POINT('Ctrl Pts',(68.6187785069662,-3.40513155320004,5.95224512547316));
#39845=CARTESIAN_POINT('Ctrl Pts',(68.7842048440012,-7.19744374978217,1.50324015275999));
#39846=CARTESIAN_POINT('Ctrl Pts',(68.9827164484433,-5.15846906456438,-5.23931471226884));
#39847=CARTESIAN_POINT('Ctrl Pts',(69.1812280528855,1.60199468026975,-7.17594652687476));
#39848=CARTESIAN_POINT('Ctrl Pts',(69.3797396573275,6.90169914440493,-2.53556683556833));
#39849=CARTESIAN_POINT('Ctrl Pts',(69.5451659943627,6.04024352960078,3.24645669154724));
#39850=CARTESIAN_POINT('Ctrl Pts',(69.6775070639907,2.67700525894223,5.89210305530824));
#39851=CARTESIAN_POINT('Ctrl Pts',(69.7767628662118,-0.46561520595085,6.47334140092824));
#39852=CARTESIAN_POINT('Ctrl Pts',(69.8760186684328,-3.49303460355603,5.44852756041988));
#39853=CARTESIAN_POINT('Ctrl Pts',(70.008359738061,-6.44234667081631,2.34766771234552));
#39854=CARTESIAN_POINT('Ctrl Pts',(70.1737860750959,-6.46846181722385,-3.49571023081299));
#39855=CARTESIAN_POINT('Ctrl Pts',(70.3722976795382,-0.557063823628739,
-7.3341557210225));
#39856=CARTESIAN_POINT('Ctrl Pts',(70.5708092839802,5.85298547448848,-4.44184497426088));
#39857=CARTESIAN_POINT('Ctrl Pts',(70.7693208884224,6.91261030511504,2.50813707913662));
#39858=CARTESIAN_POINT('Ctrl Pts',(70.9678324928645,1.6305555301296,7.17107975691506));
#39859=CARTESIAN_POINT('Ctrl Pts',(71.1332588298994,-3.99925385407112,5.57258592607248));
#39860=CARTESIAN_POINT('Ctrl Pts',(71.2655998995277,-6.17961353551377,1.90043433999651));
#39861=CARTESIAN_POINT('Ctrl Pts',(71.3979409691555,-6.4383401840856,-2.35936209704413));
#39862=CARTESIAN_POINT('Ctrl Pts',(71.563367306191,-2.68617674612466,-6.85019204663737));
#39863=CARTESIAN_POINT('Ctrl Pts',(71.7618789106327,4.31461801077602,-5.95570943739811));
#39864=CARTESIAN_POINT('Ctrl Pts',(71.9273052476681,6.82127674849029,-0.680243620698351));
#39865=CARTESIAN_POINT('Ctrl Pts',(72.059646317296,5.51192719551105,3.39346452184477));
#39866=CARTESIAN_POINT('Ctrl Pts',(72.1589021195172,3.22776268544752,5.63020767552143));
#39867=CARTESIAN_POINT('Ctrl Pts',(72.2581579217381,0.144787652460555,6.47013157578351));
#39868=CARTESIAN_POINT('Ctrl Pts',(72.3904989913663,-4.03362152721484,5.54570745472594));
#39869=CARTESIAN_POINT('Ctrl Pts',(72.5559253284013,-7.31827787064979,0.71008190057901));
#39870=CARTESIAN_POINT('Ctrl Pts',(72.7544369328434,-4.55691781933503,-5.77022622668299));
#39871=CARTESIAN_POINT('Ctrl Pts',(72.9529485372856,2.37438354046372,-6.95863454231163));
#39872=CARTESIAN_POINT('Ctrl Pts',(73.1514601417277,7.13688992541174,-1.76848755210188));
#39873=CARTESIAN_POINT('Ctrl Pts',(73.3168864787627,5.65050896588544,3.88535316654217));
#39874=CARTESIAN_POINT('Ctrl Pts',(73.4492275483909,2.01909789486699,6.14862180311659));
#39875=CARTESIAN_POINT('Ctrl Pts',(73.5484833506118,-1.16830659219089,6.38426173854624));
#39876=CARTESIAN_POINT('Ctrl Pts',(73.647739152833,-4.06570784309721,5.0351131850683));
#39877=CARTESIAN_POINT('Ctrl Pts',(73.780080222461,-6.6602568208953,1.63250287976047));
#39878=CARTESIAN_POINT('Ctrl Pts',(73.9455065594962,-6.04810590357771,-4.18131674258692));
#39879=CARTESIAN_POINT('Ctrl Pts',(74.1440181639382,0.243835091874022,-7.34852555480543));
#39880=CARTESIAN_POINT('Ctrl Pts',(74.3425297683804,6.30499174515516,-3.78250739668092));
#39881=CARTESIAN_POINT('Ctrl Pts',(74.5410413728224,6.59265678988395,3.25574353737405));
#39882=CARTESIAN_POINT('Ctrl Pts',(74.7064677098575,1.80807007447841,6.61475457063774));
#39883=CARTESIAN_POINT('Ctrl Pts',(74.8388087794856,-2.42643051867436,5.99956455976299));
#39884=CARTESIAN_POINT('Ctrl Pts',(74.9380645817067,-5.01307646459359,4.1222322339533));
#39885=CARTESIAN_POINT('Ctrl Pts',(75.0373203839277,-6.35531052844578,1.22162515698238));
#39886=CARTESIAN_POINT('Ctrl Pts',(75.1696614535559,-6.14082190943682,-3.05195052583219));
#39887=CARTESIAN_POINT('Ctrl Pts',(75.3350877905908,-1.92073099598895,-7.09744889988669));
#39888=CARTESIAN_POINT('Ctrl Pts',(75.533599395033,4.92934482030065,-5.45544168096722));
#39889=CARTESIAN_POINT('Ctrl Pts',(75.7321109994751,7.25718867309859,1.18046468258034));
#39890=CARTESIAN_POINT('Ctrl Pts',(75.9306226039172,2.93407158228261,6.74197392506965));
#39891=CARTESIAN_POINT('Ctrl Pts',(76.0960489409524,-2.88848170832391,6.21938655461771));
#39892=CARTESIAN_POINT('Ctrl Pts',(76.2283900105804,-5.72573119748685,3.01634584205342));
#39893=CARTESIAN_POINT('Ctrl Pts',(76.3276458128015,-6.48969529698426,-0.0871155494871867));
#39894=CARTESIAN_POINT('Ctrl Pts',(76.4269016150225,-5.64270178030442,-3.1689519723282));
#39895=CARTESIAN_POINT('Ctrl Pts',(76.5592426846506,-2.72049697200563,-6.29467965193754));
#39896=CARTESIAN_POINT('Ctrl Pts',(76.7246690216857,3.1139858635671,-6.66078677788813));
#39897=CARTESIAN_POINT('Ctrl Pts',(76.9231806261278,7.28626036027289,-0.985238173931595));
#39898=CARTESIAN_POINT('Ctrl Pts',(77.1216922305699,4.78113090820971,5.58579193450243));
#39899=CARTESIAN_POINT('Ctrl Pts',(77.3202038350121,-2.11055225112471,7.0433342710871));
#39900=CARTESIAN_POINT('Ctrl Pts',(77.4856301720471,-6.22053122608817,2.88601575889286));
#39901=CARTESIAN_POINT('Ctrl Pts',(77.6179712416752,-6.32022906949386,-1.39177745825087));
#39902=CARTESIAN_POINT('Ctrl Pts',(77.7172270438963,-4.90061905992092,-4.25531044656318));
#39903=CARTESIAN_POINT('Ctrl Pts',(77.8164828461173,-2.26451286093752,-6.0625342462391));
#39904=CARTESIAN_POINT('Ctrl Pts',(77.9488239157454,1.98497522997811,-6.56383798030416));
#39905=CARTESIAN_POINT('Ctrl Pts',(78.1142502527804,6.6776735471879,-3.07760693659607));
#39906=CARTESIAN_POINT('Ctrl Pts',(78.3127618572227,6.20118802446728,3.95038623203051));
#39907=CARTESIAN_POINT('Ctrl Pts',(78.5112734616646,0.0464941470039349,
7.3524229061791));
#39908=CARTESIAN_POINT('Ctrl Pts',(78.7097850661068,-6.15816322790969,4.01746364232682));
#39909=CARTESIAN_POINT('Ctrl Pts',(78.8752114031418,-6.61403723891607,-1.81069243593199));
#39910=CARTESIAN_POINT('Ctrl Pts',(79.0075524727701,-3.92908674363906,-5.14243301805027));
#39911=CARTESIAN_POINT('Ctrl Pts',(79.106808274991,-0.996518304073061,-6.41332093667049));
#39912=CARTESIAN_POINT('Ctrl Pts',(79.2060640772121,2.18341903006714,-6.09220988831756));
#39913=CARTESIAN_POINT('Ctrl Pts',(79.33840514684,5.75275644429788,-3.73227664943248));
#39914=CARTESIAN_POINT('Ctrl Pts',(79.5038314838753,7.08686629844,1.95941688444093));
#39915=CARTESIAN_POINT('Ctrl Pts',(79.7023430883174,2.18670980208234,7.01987069243372));
#39916=CARTESIAN_POINT('Ctrl Pts',(79.9008546927594,-4.71010618431074,5.64581119322374));
#39917=CARTESIAN_POINT('Ctrl Pts',(80.0993662972016,-7.29669298683701,-0.906233918390003));
#39918=CARTESIAN_POINT('Ctrl Pts',(80.2647926342366,-3.88310974879154,-5.65203984187573));
#39919=CARTESIAN_POINT('Ctrl Pts',(80.3971337038648,0.318133770830362,-6.46383252320411));
#39920=CARTESIAN_POINT('Ctrl Pts',(80.4963895060858,3.37833202016725,-5.5417151612656));
#39921=CARTESIAN_POINT('Ctrl Pts',(80.5956453083068,5.59991621302585,-3.24396029434143));
#39922=CARTESIAN_POINT('Ctrl Pts',(80.7279863779349,6.80296829521341,0.862390903031537));
#39923=CARTESIAN_POINT('Ctrl Pts',(80.89341271497,4.14826379333761,6.07082333459648));
#39924=CARTESIAN_POINT('Ctrl Pts',(81.0919243194122,-2.86075767029707,6.77320823899939));
#39925=CARTESIAN_POINT('Ctrl Pts',(81.2904359238541,-7.24167919371434,1.27215044406616));
#39926=CARTESIAN_POINT('Ctrl Pts',(81.4889475282965,-4.98830655746467,-5.40183174004447));
#39927=CARTESIAN_POINT('Ctrl Pts',(81.6543738653314,0.682176659571807,-6.82339583348686));
#39928=CARTESIAN_POINT('Ctrl Pts',(81.7867149349596,4.41506970477836,-4.73175437719689));
#39929=CARTESIAN_POINT('Ctrl Pts',(81.8859707371805,6.1572775488005,-2.05223472198617));
#39930=CARTESIAN_POINT('Ctrl Pts',(81.9852265394016,6.37104488690502,1.13671765765088));
#39931=CARTESIAN_POINT('Ctrl Pts',(82.1175676090297,4.63949668876505,5.04966990705815));
#39932=CARTESIAN_POINT('Ctrl Pts',(82.2829939460648,-0.749954889722087,
7.3144074348083));
#39933=CARTESIAN_POINT('Ctrl Pts',(82.4815055505069,-6.55681952065862,3.32692080917517));
#39934=CARTESIAN_POINT('Ctrl Pts',(82.680017154949,-6.35232421720465,-3.7024669257845));
#39935=CARTESIAN_POINT('Ctrl Pts',(82.8785287593912,-0.323472535169768,
-7.34563502891261));
#39936=CARTESIAN_POINT('Ctrl Pts',(83.0439550964262,4.92520670119462,-4.77141851505581));
#39937=CARTESIAN_POINT('Ctrl Pts',(83.1762961660544,6.42635186854234,-0.7644224263167));
#39938=CARTESIAN_POINT('Ctrl Pts',(83.2755519682753,6.02756024934152,2.40670970572829));
#39939=CARTESIAN_POINT('Ctrl Pts',(83.3748077704965,4.13252826027979,4.98041666551734));
#39940=CARTESIAN_POINT('Ctrl Pts',(83.5071488401245,0.284353283747686,6.85151362148041));
#39941=CARTESIAN_POINT('Ctrl Pts',(83.6725751771596,-5.29389915633836,5.10270714244087));
#39942=CARTESIAN_POINT('Ctrl Pts',(83.8710867816018,-7.15547719212857,-1.69098505313933));
#39943=CARTESIAN_POINT('Ctrl Pts',(84.0695983860438,-2.46216747788131,-6.92806001762949));
#39944=CARTESIAN_POINT('Ctrl Pts',(84.2681099904858,4.49416806949842,-5.81940218769057));
#39945=CARTESIAN_POINT('Ctrl Pts',(84.4335363275211,6.84159716243557,-0.465450279045067));
#39946=CARTESIAN_POINT('Ctrl Pts',(84.565877397149,5.4018620288319,3.56401832285386));
#39947=CARTESIAN_POINT('Ctrl Pts',(84.6651331993702,3.05045783488768,5.72873818258966));
#39948=CARTESIAN_POINT('Ctrl Pts',(84.7643890015912,-0.0581711681516334,
6.47139522045821));
#39949=CARTESIAN_POINT('Ctrl Pts',(84.8967300712192,-4.20511699218411,5.41674134303595));
#39950=CARTESIAN_POINT('Ctrl Pts',(85.0621564082545,-7.33703562768,0.480517072696063));
#39951=CARTESIAN_POINT('Ctrl Pts',(85.2606680126964,-4.37392821203035,-5.91007921207641));
#39952=CARTESIAN_POINT('Ctrl Pts',(85.4591796171386,2.59110314784578,-6.88087703525041));
#39953=CARTESIAN_POINT('Ctrl Pts',(85.6576912215807,7.18878928721451,-1.54411691365224));
#39954=CARTESIAN_POINT('Ctrl Pts',(85.8231175586158,5.52605610955549,4.0603940165154));
#39955=CARTESIAN_POINT('Ctrl Pts',(85.9554586282439,1.82556334808452,6.2088371251229));
#39956=CARTESIAN_POINT('Ctrl Pts',(86.0547144304649,-1.36766347836997,6.34454338601461));
#39957=CARTESIAN_POINT('Ctrl Pts',(86.1539702326861,-4.22139086822476,4.90532354914965));
#39958=CARTESIAN_POINT('Ctrl Pts',(86.286311302314,-6.70811396298986,1.42313132031107));
#39959=CARTESIAN_POINT('Ctrl Pts',(86.4517376393492,-5.91419827707177,-4.36866652406411));
#39960=CARTESIAN_POINT('Ctrl Pts',(86.6502492437913,0.473839531513867,-7.33728562858142));
#39961=CARTESIAN_POINT('Ctrl Pts',(86.8487608482334,6.42035141139087,-3.58320695066083));
#39962=CARTESIAN_POINT('Ctrl Pts',(87.0472724526755,6.48746740946582,3.46060039156732));
#39963=CARTESIAN_POINT('Ctrl Pts',(87.2126987897107,1.60003763959895,6.66813131598175));
#39964=CARTESIAN_POINT('Ctrl Pts',(87.3450398593386,-2.61312105570604,5.92063664924637));
#39965=CARTESIAN_POINT('Ctrl Pts',(87.4442956615597,-5.13970835779019,3.9632224469427));
#39966=CARTESIAN_POINT('Ctrl Pts',(87.5435514637809,-6.39044957686313,1.02200498518542));
#39967=CARTESIAN_POINT('Ctrl Pts',(87.6758925334087,-6.0422361224665,-3.24275782871163));
#39968=CARTESIAN_POINT('Ctrl Pts',(87.8413188704441,-1.69752736119953,-7.15411694879083));
#39969=CARTESIAN_POINT('Ctrl Pts',(88.0398304748858,5.0977681804467,-5.29840012413548));
#39970=CARTESIAN_POINT('Ctrl Pts',(88.2383420793283,7.21666225322758,1.40714967926411));
#39971=CARTESIAN_POINT('Ctrl Pts',(88.4368536837702,2.72150289496444,6.83054979131966));
#39972=CARTESIAN_POINT('Ctrl Pts',(88.6022800208054,-3.0818294938239,6.125881378733));
#39973=CARTESIAN_POINT('Ctrl Pts',(88.7346210904335,-5.81738196310627,2.835561157778));
#39974=CARTESIAN_POINT('Ctrl Pts',(88.8338768926545,-6.48378429654595,-0.290302192469259));
#39975=CARTESIAN_POINT('Ctrl Pts',(88.9331326948756,-5.54069632003458,-3.34410291009848));
#39976=CARTESIAN_POINT('Ctrl Pts',(89.0654737645036,-2.52204036811142,-6.37678665762986));
#39977=CARTESIAN_POINT('Ctrl Pts',(89.2309001015388,3.32104580709813,-6.56000329315107));
#39978=CARTESIAN_POINT('Ctrl Pts',(89.4294117059809,7.31354018950449,-0.7565805928752));
#39979=CARTESIAN_POINT('Ctrl Pts',(89.6279233104229,4.60386296928326,5.73277681905332));
#39980=CARTESIAN_POINT('Ctrl Pts',(89.8264349148652,-2.33008407920169,6.97378639211496));
#39981=CARTESIAN_POINT('Ctrl Pts',(89.9918612518999,-6.30785793552618,2.68979998522734));
#39982=CARTESIAN_POINT('Ctrl Pts',(90.1242023215284,-6.27354478027196,-1.589017266771));
#39983=CARTESIAN_POINT('Ctrl Pts',(90.2234581237491,-4.76495748010495,-4.406689730385));
#39984=CARTESIAN_POINT('Ctrl Pts',(90.3227139259705,-2.07354969412331,-6.13047564632424));
#39985=CARTESIAN_POINT('Ctrl Pts',(90.4550549955982,2.18955288481874,-6.49845780627156));
#39986=CARTESIAN_POINT('Ctrl Pts',(90.6204813326336,6.77077586040887,-2.86698146263652));
#39987=CARTESIAN_POINT('Ctrl Pts',(90.8189929370755,6.07443748772285,4.14264329924265));
#39988=CARTESIAN_POINT('Ctrl Pts',(91.0175045415178,-0.183774947198175,
7.35027285655411));
#39989=CARTESIAN_POINT('Ctrl Pts',(91.2160161459598,-6.28095261185096,3.82264603994139));
#39990=CARTESIAN_POINT('Ctrl Pts',(91.3814424829949,-6.55409023249801,-2.01692759403598));
#39991=CARTESIAN_POINT('Ctrl Pts',(91.513783552623,-3.76612079172275,-5.26295298918085));
#39992=CARTESIAN_POINT('Ctrl Pts',(91.613039354844,-0.795191902178077,-6.44138215026858));
#39993=CARTESIAN_POINT('Ctrl Pts',(91.7122951570653,2.37312999160159,-6.02084662046249));
#39994=CARTESIAN_POINT('Ctrl Pts',(91.844636226693,5.86681383167074,-3.55029451733617));
#39995=CARTESIAN_POINT('Ctrl Pts',(92.0100625637283,7.0220299791157,2.18038607393216));
#39996=CARTESIAN_POINT('Ctrl Pts',(92.2085741681705,1.9658051306551,7.08490610278661));
#39997=CARTESIAN_POINT('Ctrl Pts',(92.4070857726124,-4.88459862582638,5.49554188061449));
#39998=CARTESIAN_POINT('Ctrl Pts',(92.6055973770546,-7.26473492135933,-1.13429051894974));
#39999=CARTESIAN_POINT('Ctrl Pts',(92.7710237140898,-3.7042076507531,-5.7708700709176));
#40000=CARTESIAN_POINT('Ctrl Pts',(92.9033647837178,0.520397198382932,-6.45069970934075));
#40001=CARTESIAN_POINT('Ctrl Pts',(93.0026205859388,3.55021779910258,-5.43320234723718));
#40002=CARTESIAN_POINT('Ctrl Pts',(93.10187638816,5.69875659207993,-3.06700395963218));
#40003=CARTESIAN_POINT('Ctrl Pts',(93.2342174577878,6.77262535525563,1.0750076709765));
#40004=CARTESIAN_POINT('Ctrl Pts',(93.3996437948232,3.95611714926058,6.19775165365016));
#40005=CARTESIAN_POINT('Ctrl Pts',(93.5981553992651,-3.07146236840367,6.6802996352329));
#40006=CARTESIAN_POINT('Ctrl Pts',(93.7966670037075,-7.27796574748004,1.04474823547117));
#40007=CARTESIAN_POINT('Ctrl Pts',(93.9951786081492,-4.8166978505934,-5.55539470020689));
#40008=CARTESIAN_POINT('Ctrl Pts',(94.1606049451846,0.895521517553394,-6.7986864103964));
#40009=CARTESIAN_POINT('Ctrl Pts',(94.2929460148125,4.56108251734731,-4.59117264477413));
#40010=CARTESIAN_POINT('Ctrl Pts',(94.3922018170336,6.21852484226242,-1.85840871534061));
#40011=CARTESIAN_POINT('Ctrl Pts',(94.4914576192548,6.33232305163478,1.33567389504654));
#40012=CARTESIAN_POINT('Ctrl Pts',(94.6237986888826,4.47908725340983,5.19248236122677));
#40013=CARTESIAN_POINT('Ctrl Pts',(94.7892250259181,-0.978642878797454,
7.28733466877817));
#40014=CARTESIAN_POINT('Ctrl Pts',(94.9877366303597,-6.657788546716,3.11995768628837));
#40015=CARTESIAN_POINT('Ctrl Pts',(95.1862482348023,-6.23326332199298,-3.89957852282909));
#40016=CARTESIAN_POINT('Ctrl Pts',(95.384759839244,-0.0932801621545284,
-7.35216208134352));
#40017=CARTESIAN_POINT('Ctrl Pts',(95.5501861762794,5.07221142391009,-4.61484203049959));
#40018=CARTESIAN_POINT('Ctrl Pts',(95.6825272459072,6.44713844549368,-0.562801784655363));
#40019=CARTESIAN_POINT('Ctrl Pts',(95.7817830481286,5.94923618490345,2.59428660392868));
#40020=CARTESIAN_POINT('Ctrl Pts',(95.8810388503493,3.97453618501874,5.10738701276399));
#40021=CARTESIAN_POINT('Ctrl Pts',(96.0133799199776,0.069653856197323,6.85705797231051));
#40022=CARTESIAN_POINT('Ctrl Pts',(96.1788062570125,-5.45109758750357,4.93442231173111));
#40023=CARTESIAN_POINT('Ctrl Pts',(96.3773178614549,-7.09901335357813,-1.91423449523096));
#40024=CARTESIAN_POINT('Ctrl Pts',(96.5758294658966,-2.24400282214668,-7.00176660787908));
#40025=CARTESIAN_POINT('Ctrl Pts',(96.7743410703392,4.67420254334854,-5.67580999001474));
#40026=CARTESIAN_POINT('Ctrl Pts',(96.9397674073738,6.85281755654995,-0.250972572108975));
#40027=CARTESIAN_POINT('Ctrl Pts',(97.0721084770024,5.28760290966167,3.73143343152621));
#40028=CARTESIAN_POINT('Ctrl Pts',(97.171364279223,2.86956225427671,5.82145571450295));
#40029=CARTESIAN_POINT('Ctrl Pts',(97.2706200814443,-0.260798927335446,
6.46639960903085));
#40030=CARTESIAN_POINT('Ctrl Pts',(97.4029611510722,-4.37268362577514,5.28239847078841));
#40031=CARTESIAN_POINT('Ctrl Pts',(97.5683874881074,-7.34848485781509,0.250516972397847));
#40032=CARTESIAN_POINT('Ctrl Pts',(97.7668990925496,-4.18670470445587,-6.04415320906906));
#40033=CARTESIAN_POINT('Ctrl Pts',(97.9654106969916,2.80531182390014,-6.79636004547279));
#40034=CARTESIAN_POINT('Ctrl Pts',(98.1639223014338,7.23361860234148,-1.31823760182156));
#40035=CARTESIAN_POINT('Ctrl Pts',(98.3293486384688,5.39619172482621,4.2314548992311));
#40036=CARTESIAN_POINT('Ctrl Pts',(98.4616897080969,1.63023388960724,6.26296075744928));
#40037=CARTESIAN_POINT('Ctrl Pts',(98.5609455103179,-1.56567653366841,6.29860231789631));
#40038=CARTESIAN_POINT('Ctrl Pts',(98.6602013125392,-4.37293411252434,4.77072187742011));
#40039=CARTESIAN_POINT('Ctrl Pts',(98.7925423821669,-6.74939027975622,1.21236403231126));
#40040=CARTESIAN_POINT('Ctrl Pts',(98.9579687192024,-5.77448975510201,-4.55173115717733));
#40041=CARTESIAN_POINT('Ctrl Pts',(99.1564803236441,0.70337938998819,-7.31884838828847));
#40042=CARTESIAN_POINT('Ctrl Pts',(99.3549919280866,6.52941314982036,-3.38039172522444));
#40043=CARTESIAN_POINT('Ctrl Pts',(99.5535035325282,6.37591445285421,3.66206271777009));
#40044=CARTESIAN_POINT('Ctrl Pts',(99.7189298695639,1.39043567136697,6.71496718823704));
#40045=CARTESIAN_POINT('Ctrl Pts',(99.8512709391915,-2.79724833035012,5.83590110972824));
#40046=CARTESIAN_POINT('Ctrl Pts',(99.9505267414128,-5.26129864878984,3.80032507758626));
#40047=CARTESIAN_POINT('Ctrl Pts',(100.049782543634,-6.41932014120929,0.821382315878928));
#40048=CARTESIAN_POINT('Ctrl Pts',(100.182123613262,-5.9377234255724,-3.43038426662649));
#40049=CARTESIAN_POINT('Ctrl Pts',(100.347549950297,-1.47265859680333,-7.20376742519206));
#40050=CARTESIAN_POINT('Ctrl Pts',(100.546061554739,5.26119106866268,-5.13616129381046));
#40051=CARTESIAN_POINT('Ctrl Pts',(100.744573159181,7.16905691026357,1.63245438356331));
#40052=CARTESIAN_POINT('Ctrl Pts',(100.943084763623,2.50626464765636,6.91242547698743));
#40053=CARTESIAN_POINT('Ctrl Pts',(101.108511100658,-3.27215427013865,6.02636724135885));
#40054=CARTESIAN_POINT('Ctrl Pts',(101.240852170287,-5.90332637858596,2.65199503243598));
#40055=CARTESIAN_POINT('Ctrl Pts',(101.340107972507,-6.47151326263513,-0.493204074016322));
#40056=CARTESIAN_POINT('Ctrl Pts',(101.439363774729,-5.43325591434297,-3.51597357120765));
#40057=CARTESIAN_POINT('Ctrl Pts',(101.571704844356,-2.3211098600259,-6.45263858533859));
#40058=CARTESIAN_POINT('Ctrl Pts',(101.737131181392,3.52484809098738,-6.45278501071125));
#40059=CARTESIAN_POINT('Ctrl Pts',(101.935642785834,7.33364606630008,-0.527180871479639));
#40060=CARTESIAN_POINT('Ctrl Pts',(102.134154390276,4.42207903767292,5.87413834375616));
#40061=CARTESIAN_POINT('Ctrl Pts',(102.332665994718,-2.54733029566822,6.89739782988979));
#40062=CARTESIAN_POINT('Ctrl Pts',(102.498092331753,-6.38899718011882,2.4909457496588));
#40063=CARTESIAN_POINT('Ctrl Pts',(102.630433401381,-6.22070668445104,-1.78469838633858));
#40064=CARTESIAN_POINT('Ctrl Pts',(102.729689203602,-4.62462188777941,-4.55374643147395));
#40065=CARTESIAN_POINT('Ctrl Pts',(102.828945005823,-1.88055255381611,-6.19240357829704));
#40066=CARTESIAN_POINT('Ctrl Pts',(102.961286075451,2.39198277703677,-6.42670320535172));
#40067=CARTESIAN_POINT('Ctrl Pts',(103.126712412487,6.85723662620696,-2.65354372701774));
#40068=CARTESIAN_POINT('Ctrl Pts',(103.325224016929,5.94172845146893,4.33083679050598));
#40069=CARTESIAN_POINT('Ctrl Pts',(103.523735621371,-0.413863774020237,
7.34091282291405));
#40070=CARTESIAN_POINT('Ctrl Pts',(103.722247225813,-6.39758092274897,3.6240787513264));
#40071=CARTESIAN_POINT('Ctrl Pts',(103.887673562848,-6.48771422857854,-2.22118432003229));
#40072=CARTESIAN_POINT('Ctrl Pts',(104.020014632476,-3.59946059997928,-5.37831045715732));
#40073=CARTESIAN_POINT('Ctrl Pts',(104.119270434697,-0.593085485580851,
-6.46312492323568));
#40074=CARTESIAN_POINT('Ctrl Pts',(104.218526236918,2.56051311720067,-5.94357742119504));
#40075=CARTESIAN_POINT('Ctrl Pts',(104.350867306546,5.97511638043491,-3.364829852218));
#40076=CARTESIAN_POINT('Ctrl Pts',(104.516293643581,6.95030565375228,2.39921649231612));
#40077=CARTESIAN_POINT('Ctrl Pts',(104.714805248023,1.74297217383987,7.14299183158766));
#40078=CARTESIAN_POINT('Ctrl Pts',(104.913316852465,-5.05429969713898,5.33988191415307));
#40079=CARTESIAN_POINT('Ctrl Pts',(105.111828456908,-7.22565077728843,-1.36123447626787));
#40080=CARTESIAN_POINT('Ctrl Pts',(105.277254793943,-3.52167204419261,-5.88403957747914));
#40081=CARTESIAN_POINT('Ctrl Pts',(105.409595863571,0.722150160936881,-6.43123931018474));
#40082=CARTESIAN_POINT('Ctrl Pts',(105.508851665792,3.71862112089202,-5.3193600409715));
#40083=CARTESIAN_POINT('Ctrl Pts',(105.608107468013,5.79200698135239,-2.88703913835982));
#40084=CARTESIAN_POINT('Ctrl Pts',(105.740448537641,6.73563905550354,1.2865699056858));
#40085=CARTESIAN_POINT('Ctrl Pts',(105.905874874676,3.76008989159166,6.31860060108252));
#40086=CARTESIAN_POINT('Ctrl Pts',(106.104386479118,-3.27915422052681,6.58083808626542));
#40087=CARTESIAN_POINT('Ctrl Pts',(106.30289808356,-7.30711325565383,0.816321489812915));
#40088=CARTESIAN_POINT('Ctrl Pts',(106.501409688003,-4.64036435591168,-5.70350883137131));
#40089=CARTESIAN_POINT('Ctrl Pts',(106.666836025037,1.10798790665508,-6.76730712296029));
#40090=CARTESIAN_POINT('Ctrl Pts',(106.799177094666,4.70262135634261,-4.44608868040009));
#40091=CARTESIAN_POINT('Ctrl Pts',(106.898432896887,6.2736721784315,-1.66275690292686));
#40092=CARTESIAN_POINT('Ctrl Pts',(106.997688699108,6.28738997577458,1.53331465981352));
#40093=CARTESIAN_POINT('Ctrl Pts',(107.130029768736,4.31428373900651,5.33021287136194));
#40094=CARTESIAN_POINT('Ctrl Pts',(107.295456105771,-1.20636992374352,7.25309034469861));
#40095=CARTESIAN_POINT('Ctrl Pts',(107.493967710213,-6.7522284862449,2.90997293473533));
#40096=CARTESIAN_POINT('Ctrl Pts',(107.692479314655,-6.10808513208516,-4.09293635920486));
#40097=CARTESIAN_POINT('Ctrl Pts',(107.890990919097,0.136997792198854,-7.35133649303282));
#40098=CARTESIAN_POINT('Ctrl Pts',(108.056417256132,5.21425114731496,-4.45398626681165));
#40099=CARTESIAN_POINT('Ctrl Pts',(108.18875832576,6.46158639258335,-0.360283155660035));
#40100=CARTESIAN_POINT('Ctrl Pts',(108.288014127981,5.8651082250223,2.77856311405613));
#40101=CARTESIAN_POINT('Ctrl Pts',(108.387269930202,3.81258651774621,5.23074243008551));
#40102=CARTESIAN_POINT('Ctrl Pts',(108.519610999831,-0.144983932043383,
6.8528582990123));
#40103=CARTESIAN_POINT('Ctrl Pts',(108.685037336866,-5.60324512615471,4.76749414642294));
#40104=CARTESIAN_POINT('Ctrl Pts',(108.883548941308,-7.03492315008415,-2.14615525054554));
#40105=CARTESIAN_POINT('Ctrl Pts',(109.048975278343,-2.8610191033943,-6.23044836115737));
#40106=CARTESIAN_POINT('Ctrl Pts',(109.181316347971,1.42154645890215,-6.31467627302082));
#40107=CARTESIAN_POINT('Ctrl Pts',(109.280572150192,4.26891450491086,-4.88386661729597));
#40108=CARTESIAN_POINT('Ctrl Pts',(109.379827952413,6.08602022828173,-2.23498829451912));
#40109=CARTESIAN_POINT('Ctrl Pts',(109.445998487227,6.30359034811574,-0.116516279140912));
#40110=CARTESIAN_POINT('Ctrl Pts',(109.479083754634,6.15279807233871,0.906722914414925));
#40111=CARTESIAN_POINT('Ctrl Pts',(109.067,6.85892174064777,1.0107826451168));
#40112=CARTESIAN_POINT('Ctrl Pts',(109.033914732593,7.0270196379767,-0.129888228207594));
#40113=CARTESIAN_POINT('Ctrl Pts',(109.000829465186,6.90574989959926,-1.31068707715371));
#40114=CARTESIAN_POINT('Ctrl Pts',(108.967744197779,6.50750749520052,-2.39323248417603));
#40115=CARTESIAN_POINT('Ctrl Pts',(108.934658930372,6.10926509080182,-3.47577789119822));
#40116=CARTESIAN_POINT('Ctrl Pts',(108.901573662965,5.4340500203817,-4.46006985629672));
#40117=CARTESIAN_POINT('Ctrl Pts',(108.868488395558,4.56741828174481,-5.21805184112751));
#40118=CARTESIAN_POINT('Ctrl Pts',(108.835403128151,3.70078654310793,-5.9760338259583));
#40119=CARTESIAN_POINT('Ctrl Pts',(108.802317860744,2.64273813625421,-6.50770583052161));
#40120=CARTESIAN_POINT('Ctrl Pts',(108.769232593337,1.51695734956969,-6.76180504555109));
#40121=CARTESIAN_POINT('Ctrl Pts',(108.73614732593,0.391176562885175,-7.01590426058057));
#40122=CARTESIAN_POINT('Ctrl Pts',(108.703062058523,-0.802336603629954,
-6.99243068607618));
#40123=CARTESIAN_POINT('Ctrl Pts',(108.669976791116,-1.90820675800765,-6.67324659991116));
#40124=CARTESIAN_POINT('Ctrl Pts',(108.603806256302,-4.11994706676328,-6.03487842758105));
#40125=CARTESIAN_POINT('Ctrl Pts',(108.537635721488,-5.98111532696877,-4.21366820860795));
#40126=CARTESIAN_POINT('Ctrl Pts',(108.471465186674,-6.64570211709476,-2.01854778325574));
#40127=CARTESIAN_POINT('Ctrl Pts',(108.451940678984,-6.84179740226082,-1.37084793098864));
#40128=CARTESIAN_POINT('Ctrl Pts',(108.432416171295,-6.93371537062503,-0.690594539326748));
#40129=CARTESIAN_POINT('Ctrl Pts',(108.412891663606,-6.92776634541837,-0.00844704756396031));
#40130=CARTESIAN_POINT('Origin',(-66.51072,1.12618006296016E-15,0.));
#40131=CARTESIAN_POINT('',(-66.51072,1.15821195975198,6.83557123116185));
#40132=CARTESIAN_POINT('Ctrl Pts',(-66.51072,4.88120307569149,-3.85434375923665));
#40133=CARTESIAN_POINT('Ctrl Pts',(-66.51072,4.99039108986081,-3.73103378318323));
#40134=CARTESIAN_POINT('Ctrl Pts',(-66.51072,5.09450400334291,-3.60353370689817));
#40135=CARTESIAN_POINT('Ctrl Pts',(-66.51072,5.19325944155552,-3.47211850304819));
#40136=CARTESIAN_POINT('Ctrl Pts',(-66.51072,5.29755106214915,-3.33333622605954));
#40137=CARTESIAN_POINT('Ctrl Pts',(-66.51072,5.39586868951527,-3.19018760651214));
#40138=CARTESIAN_POINT('Ctrl Pts',(-66.51072,5.48809659704528,-3.04312464176522));
#40139=CARTESIAN_POINT('Ctrl Pts',(-66.51072,5.54643629869445,-2.95009846653529));
#40140=CARTESIAN_POINT('Ctrl Pts',(-66.51072,5.60233858003336,-2.85550523338778));
#40141=CARTESIAN_POINT('Ctrl Pts',(-66.51072,5.65576594679515,-2.75945247809285));
#40142=CARTESIAN_POINT('Ctrl Pts',(-66.51072,5.69253044352725,-2.69335655343509));
#40143=CARTESIAN_POINT('Ctrl Pts',(-66.51072,5.72812290839306,-2.62656942226179));
#40144=CARTESIAN_POINT('Ctrl Pts',(-66.51072,5.76252923331074,-2.55912494345147));
#40145=CARTESIAN_POINT('Ctrl Pts',(-66.51072,5.77883595581305,-2.52715993693293));
#40146=CARTESIAN_POINT('Ctrl Pts',(-66.51072,5.79487826796475,-2.4950428726627));
#40147=CARTESIAN_POINT('Ctrl Pts',(-66.51072,5.81064158940516,-2.46280437671937));
#40148=CARTESIAN_POINT('Ctrl Pts',(-66.51072,5.88832126227673,-2.30393710828132));
#40149=CARTESIAN_POINT('Ctrl Pts',(-66.51072,5.95928765838032,-2.14201350648212));
#40150=CARTESIAN_POINT('Ctrl Pts',(-66.51072,6.02342466627868,-1.97750197757987));
#40151=CARTESIAN_POINT('Ctrl Pts',(-66.51072,6.0877724413544,-1.81244983052706));
#40152=CARTESIAN_POINT('Ctrl Pts',(-66.51072,6.14524621241747,-1.64479206150153));
#40153=CARTESIAN_POINT('Ctrl Pts',(-66.51072,6.19568512368219,-1.47497227311826));
#40154=CARTESIAN_POINT('Ctrl Pts',(-66.51072,6.23895047404685,-1.32930472282772));
#40155=CARTESIAN_POINT('Ctrl Pts',(-66.51072,6.27703911663385,-1.18204567723471));
#40156=CARTESIAN_POINT('Ctrl Pts',(-66.51072,6.30982117183241,-1.03346352641803));
#40157=CARTESIAN_POINT('Ctrl Pts',(-66.51072,6.31481496487166,-1.01082954248961));
#40158=CARTESIAN_POINT('Ctrl Pts',(-66.51072,6.31968556421223,-0.988164840915087));
#40159=CARTESIAN_POINT('Ctrl Pts',(-66.51072,6.32443245356077,-0.965470356345221));
#40160=CARTESIAN_POINT('Ctrl Pts',(-66.51072,6.32944638574867,-0.941499162091915));
#40161=CARTESIAN_POINT('Ctrl Pts',(-66.51072,6.33432061618718,-0.917502689271744));
#40162=CARTESIAN_POINT('Ctrl Pts',(-66.51072,6.33905393823772,-0.893486720876821));
#40163=CARTESIAN_POINT('Ctrl Pts',(-66.51072,6.35925666012823,-0.790981984196606));
#40164=CARTESIAN_POINT('Ctrl Pts',(-66.51072,6.37689836887655,-0.688095730530865));
#40165=CARTESIAN_POINT('Ctrl Pts',(-66.51072,6.39195662158433,-0.584920330828077));
#40166=CARTESIAN_POINT('Ctrl Pts',(-66.51072,6.41738598417301,-0.410684667488666));
#40167=CARTESIAN_POINT('Ctrl Pts',(-66.51072,6.43545071544452,-0.235625365624705));
#40168=CARTESIAN_POINT('Ctrl Pts',(-66.51072,6.44629977206506,-0.0601947746487687));
#40169=CARTESIAN_POINT('Ctrl Pts',(-66.51072,6.45728926013915,0.117506610346195));
#40170=CARTESIAN_POINT('Ctrl Pts',(-66.51072,6.46087513399998,0.29558962059473));
#40171=CARTESIAN_POINT('Ctrl Pts',(-66.51072,6.45716079669616,0.473599419439789));
#40172=CARTESIAN_POINT('Ctrl Pts',(-66.51072,6.4533746861754,0.655048953254274));
#40173=CARTESIAN_POINT('Ctrl Pts',(-66.51072,6.44200365346109,0.836423165438464));
#40174=CARTESIAN_POINT('Ctrl Pts',(-66.51072,6.42310242695258,1.01724540279636));
#40175=CARTESIAN_POINT('Ctrl Pts',(-66.51072,6.4089265070712,1.15286208081478));
#40176=CARTESIAN_POINT('Ctrl Pts',(-66.51072,6.39051371885256,1.28816845488067));
#40177=CARTESIAN_POINT('Ctrl Pts',(-66.51072,6.36786686174987,1.42296130007595));
#40178=CARTESIAN_POINT('Ctrl Pts',(-66.51072,6.36157323512551,1.46042061884357));
#40179=CARTESIAN_POINT('Ctrl Pts',(-66.51072,6.35495250829001,1.49784025576893));
#40180=CARTESIAN_POINT('Ctrl Pts',(-66.51072,6.34800450349549,1.53521578937394));
#40181=CARTESIAN_POINT('Ctrl Pts',(-66.51072,6.34388886263482,1.5573551340985));
#40182=CARTESIAN_POINT('Ctrl Pts',(-66.51072,6.33966014021218,1.57946951451518));
#40183=CARTESIAN_POINT('Ctrl Pts',(-66.51072,6.33531911437619,1.60155545740789));
#40184=CARTESIAN_POINT('Ctrl Pts',(-66.51072,6.3001676131708,1.78039660637772));
#40185=CARTESIAN_POINT('Ctrl Pts',(-66.51072,6.25764647419907,1.95742764186776));
#40186=CARTESIAN_POINT('Ctrl Pts',(-66.51072,6.20788490890828,2.13217995064111));
#40187=CARTESIAN_POINT('Ctrl Pts',(-66.51072,6.16217257165171,2.29271220939));
#40188=CARTESIAN_POINT('Ctrl Pts',(-66.51072,6.11034959729668,2.45132208138385));
#40189=CARTESIAN_POINT('Ctrl Pts',(-66.51072,6.05247743653113,2.60764785511938));
#40190=CARTESIAN_POINT('Ctrl Pts',(-66.51072,5.98976686720135,2.77704326289739));
#40191=CARTESIAN_POINT('Ctrl Pts',(-66.51072,5.91995403238247,2.94375748123564));
#40192=CARTESIAN_POINT('Ctrl Pts',(-66.51072,5.84334750123361,3.10743909866994));
#40193=CARTESIAN_POINT('Ctrl Pts',(-66.51072,5.76633331846032,3.27199172639848));
#40194=CARTESIAN_POINT('Ctrl Pts',(-66.51072,5.6824526225013,3.43348002678122));
#40195=CARTESIAN_POINT('Ctrl Pts',(-66.51072,5.59196984847498,3.59152795464669));
#40196=CARTESIAN_POINT('Ctrl Pts',(-66.51072,5.5455267417669,3.67265098450333));
#40197=CARTESIAN_POINT('Ctrl Pts',(-66.51072,5.49734350565571,3.75286725678217));
#40198=CARTESIAN_POINT('Ctrl Pts',(-66.51072,5.44745134134628,3.83212314758995));
#40199=CARTESIAN_POINT('Ctrl Pts',(-66.51072,5.43459757335987,3.85254192168203));
#40200=CARTESIAN_POINT('Ctrl Pts',(-66.51072,5.42163036231943,3.87289694046096));
#40201=CARTESIAN_POINT('Ctrl Pts',(-66.51072,5.40855021073457,3.89318726281891));
#40202=CARTESIAN_POINT('Ctrl Pts',(-66.51072,5.39793659485858,3.90965142121267));
#40203=CARTESIAN_POINT('Ctrl Pts',(-66.51072,5.38724950512193,3.92607155347971));
#40204=CARTESIAN_POINT('Ctrl Pts',(-66.51072,5.37649448582116,3.94243934362586));
#40205=CARTESIAN_POINT('Ctrl Pts',(-66.51072,5.27546351607111,4.0961958051333));
#40206=CARTESIAN_POINT('Ctrl Pts',(-66.51072,5.16831729088704,4.24552924635349));
#40207=CARTESIAN_POINT('Ctrl Pts',(-66.51072,5.0554088542436,4.39009677447249));
#40208=CARTESIAN_POINT('Ctrl Pts',(-66.51072,4.94170583266791,4.53568168608338));
#40209=CARTESIAN_POINT('Ctrl Pts',(-66.51072,4.82215887167875,4.67643400616859));
#40210=CARTESIAN_POINT('Ctrl Pts',(-66.51072,4.69707874333019,4.81198543660765));
#40211=CARTESIAN_POINT('Ctrl Pts',(-66.51072,4.57220526885852,4.94731291277843));
#40212=CARTESIAN_POINT('Ctrl Pts',(-66.51072,4.44181649197592,5.07745729021896));
#40213=CARTESIAN_POINT('Ctrl Pts',(-66.51072,4.3061778998763,5.2020247050942));
#40214=CARTESIAN_POINT('Ctrl Pts',(-66.51072,4.26374685226021,5.24099241944576));
#40215=CARTESIAN_POINT('Ctrl Pts',(-66.51072,4.22080176452851,5.27941413861846));
#40216=CARTESIAN_POINT('Ctrl Pts',(-66.51072,4.1773499785852,5.31727710454912));
#40217=CARTESIAN_POINT('Ctrl Pts',(-66.51072,4.07025321995506,5.41059895163238));
#40218=CARTESIAN_POINT('Ctrl Pts',(-66.51072,3.96007912027853,5.50052745896816));
#40219=CARTESIAN_POINT('Ctrl Pts',(-66.51072,3.84701398483213,5.58697437177063));
#40220=CARTESIAN_POINT('Ctrl Pts',(-66.51072,3.79754798807433,5.62479489612171));
#40221=CARTESIAN_POINT('Ctrl Pts',(-66.51072,3.7475284815066,5.66194883395774));
#40222=CARTESIAN_POINT('Ctrl Pts',(-66.51072,3.69697043257265,5.69842788582505));
#40223=CARTESIAN_POINT('Ctrl Pts',(-66.51072,3.66885907731644,5.71871101794891));
#40224=CARTESIAN_POINT('Ctrl Pts',(-66.51072,3.64058122006461,5.73878549233668));
#40225=CARTESIAN_POINT('Ctrl Pts',(-66.51072,3.61213938875156,5.75864980418902));
#40226=CARTESIAN_POINT('Ctrl Pts',(-66.51072,3.59288633876352,5.77209649771805));
#40227=CARTESIAN_POINT('Ctrl Pts',(-66.51072,3.57355735859509,5.78544736926076));
#40228=CARTESIAN_POINT('Ctrl Pts',(-66.51072,3.5541671769133,5.79869258258653));
#40229=CARTESIAN_POINT('Ctrl Pts',(-66.51072,3.40184184240323,5.90274429203488));
#40230=CARTESIAN_POINT('Ctrl Pts',(-66.51072,3.24554560446478,6.00041723965922));
#40231=CARTESIAN_POINT('Ctrl Pts',(-66.51072,3.08574808349221,6.09159803735488));
#40232=CARTESIAN_POINT('Ctrl Pts',(-66.51072,2.92308726372841,6.18441263929378));
#40233=CARTESIAN_POINT('Ctrl Pts',(-66.51072,2.75679806121725,6.27050079088333));
#40234=CARTESIAN_POINT('Ctrl Pts',(-66.51072,2.58733626350152,6.34970623172909));
#40235=CARTESIAN_POINT('Ctrl Pts',(-66.51072,2.41755160422378,6.42906257615722));
#40236=CARTESIAN_POINT('Ctrl Pts',(-66.51072,2.24458162584722,6.50151032688276));
#40237=CARTESIAN_POINT('Ctrl Pts',(-66.51072,2.06885406101389,6.5668498761021));
#40238=CARTESIAN_POINT('Ctrl Pts',(-66.51072,1.89493100273515,6.6315184682923));
#40239=CARTESIAN_POINT('Ctrl Pts',(-66.51072,1.71830605202983,6.68922437216728));
#40240=CARTESIAN_POINT('Ctrl Pts',(-66.51072,1.53937345115484,6.73972784852978));
#40241=CARTESIAN_POINT('Ctrl Pts',(-66.51072,1.41341886592483,6.77527835406541));
#40242=CARTESIAN_POINT('Ctrl Pts',(-66.51072,1.28632038834554,6.80725906508397));
#40243=CARTESIAN_POINT('Ctrl Pts',(-66.51072,1.15821195975198,6.83557123116185));
#40244=CARTESIAN_POINT('',(-66.51072,-6.933,-8.4904762584886E-16));
#40245=CARTESIAN_POINT('Origin',(-66.51072,0.,0.));
#40246=CARTESIAN_POINT('',(-66.51072,-4.64229328560453,5.14951358184791));
#40247=CARTESIAN_POINT('Origin',(-66.51072,0.,0.));
#40248=CARTESIAN_POINT('Ctrl Pts',(-66.51072,-4.64244039278575,5.14956429285679));
#40249=CARTESIAN_POINT('Ctrl Pts',(-66.51072,-4.77208351901737,5.020713217228));
#40250=CARTESIAN_POINT('Ctrl Pts',(-66.51072,-4.89641770167796,4.88689155878294));
#40251=CARTESIAN_POINT('Ctrl Pts',(-66.51072,-5.0150831726735,4.74832914407448));
#40252=CARTESIAN_POINT('Ctrl Pts',(-66.51072,-5.13744689549262,4.60544838217897));
#40253=CARTESIAN_POINT('Ctrl Pts',(-66.51072,-5.25378364734574,4.45752634517166));
#40254=CARTESIAN_POINT('Ctrl Pts',(-66.51072,-5.36388377718831,4.30499917290805));
#40255=CARTESIAN_POINT('Ctrl Pts',(-66.51072,-5.43302299971837,4.20921717773608));
#40256=CARTESIAN_POINT('Ctrl Pts',(-66.51072,-5.49970198987414,4.11161858692189));
#40257=CARTESIAN_POINT('Ctrl Pts',(-66.51072,-5.56385938958403,4.01230682937023));
#40258=CARTESIAN_POINT('Ctrl Pts',(-66.51072,-5.60405094939935,3.9500927361861));
#40259=CARTESIAN_POINT('Ctrl Pts',(-66.51072,-5.64325278175659,3.88720626027224));
#40260=CARTESIAN_POINT('Ctrl Pts',(-66.51072,-5.68144825171902,3.82367233499214));
#40261=CARTESIAN_POINT('Ctrl Pts',(-66.51072,-5.69807351632313,3.79601805242516));
#40262=CARTESIAN_POINT('Ctrl Pts',(-66.51072,-5.71450810167693,3.76824110117671));
#40263=CARTESIAN_POINT('Ctrl Pts',(-66.51072,-5.73075056271715,3.74034352052681));
#40264=CARTESIAN_POINT('Ctrl Pts',(-66.51072,-5.74433450921565,3.7170121274548));
#40265=CARTESIAN_POINT('Ctrl Pts',(-66.51072,-5.75777909807329,3.69360490600033));
#40266=CARTESIAN_POINT('Ctrl Pts',(-66.51072,-5.77108339705107,3.67012387995191));
#40267=CARTESIAN_POINT('Ctrl Pts',(-66.51072,-5.86309962123462,3.50772258691574));
#40268=CARTESIAN_POINT('Ctrl Pts',(-66.51072,-5.94841524727953,3.34178186612013));
#40269=CARTESIAN_POINT('Ctrl Pts',(-66.51072,-6.02682780981107,3.17272981240304));
#40270=CARTESIAN_POINT('Ctrl Pts',(-66.51072,-6.10484904738322,3.00452142819397));
#40271=CARTESIAN_POINT('Ctrl Pts',(-66.51072,-6.17603618743261,2.83323201149326));
#40272=CARTESIAN_POINT('Ctrl Pts',(-66.51072,-6.24014138299806,2.65926639348439));
#40273=CARTESIAN_POINT('Ctrl Pts',(-66.51072,-6.29582315113101,2.50815987053205));
#40274=CARTESIAN_POINT('Ctrl Pts',(-66.51072,-6.34616120131628,2.35503373144777));
#40275=CARTESIAN_POINT('Ctrl Pts',(-66.51072,-6.39096108360734,2.2001487288792));
#40276=CARTESIAN_POINT('Ctrl Pts',(-66.51072,-6.39811169003876,2.17542719750771));
#40277=CARTESIAN_POINT('Ctrl Pts',(-66.51072,-6.40512114147276,2.15066085480165));
#40278=CARTESIAN_POINT('Ctrl Pts',(-66.51072,-6.41198857303617,2.12585076007206));
#40279=CARTESIAN_POINT('Ctrl Pts',(-66.51072,-6.41878698647798,2.10129000836384));
#40280=CARTESIAN_POINT('Ctrl Pts',(-66.51072,-6.42544420594425,2.07669356320528));
#40281=CARTESIAN_POINT('Ctrl Pts',(-66.51072,-6.43195802548163,2.05206883857791));
#40282=CARTESIAN_POINT('Ctrl Pts',(-66.51072,-6.46008886107403,1.94572354055036));
#40283=CARTESIAN_POINT('Ctrl Pts',(-66.51072,-6.48555598077592,1.83881391444392));
#40284=CARTESIAN_POINT('Ctrl Pts',(-66.51072,-6.50831913745385,1.73142657942197));
#40285=CARTESIAN_POINT('Ctrl Pts',(-66.51072,-6.54628591077437,1.55231475130603));
#40286=CARTESIAN_POINT('Ctrl Pts',(-66.51072,-6.57673339401698,1.37187431457994));
#40287=CARTESIAN_POINT('Ctrl Pts',(-66.51072,-6.59972567046035,1.19057384607931));
#40288=CARTESIAN_POINT('Ctrl Pts',(-66.51072,-6.62284513108582,1.00827049507335));
#40289=CARTESIAN_POINT('Ctrl Pts',(-66.51072,-6.63842664969771,0.825096833283679));
#40290=CARTESIAN_POINT('Ctrl Pts',(-66.51072,-6.64648284652764,0.641526136489152));
#40291=CARTESIAN_POINT('Ctrl Pts',(-66.51072,-6.65456709998406,0.457316133756397));
#40292=CARTESIAN_POINT('Ctrl Pts',(-66.51072,-6.65507349012932,0.272705573461058));
#40293=CARTESIAN_POINT('Ctrl Pts',(-66.51072,-6.64796251940445,0.0881807892318182));
#40294=CARTESIAN_POINT('Ctrl Pts',(-66.51072,-6.6426292913608,-0.0502127989401112));
#40295=CARTESIAN_POINT('Ctrl Pts',(-66.51072,-6.63301022104618,-0.188558041365239));
#40296=CARTESIAN_POINT('Ctrl Pts',(-66.51072,-6.61906962965593,-0.326642930935964));
#40297=CARTESIAN_POINT('Ctrl Pts',(-66.51072,-6.61533149919028,-0.363670006624603));
#40298=CARTESIAN_POINT('Ctrl Pts',(-66.51072,-6.61128254879057,-0.400678319771744));
#40299=CARTESIAN_POINT('Ctrl Pts',(-66.51072,-6.60692189323121,-0.437663682307064));
#40300=CARTESIAN_POINT('Ctrl Pts',(-66.51072,-6.6043408934228,-0.459554705874133));
#40301=CARTESIAN_POINT('Ctrl Pts',(-66.51072,-6.60165067268052,-0.481437465497591));
#40302=CARTESIAN_POINT('Ctrl Pts',(-66.51072,-6.59885297598377,-0.503297068535974));
#40303=CARTESIAN_POINT('Ctrl Pts',(-66.51072,-6.57583263441499,-0.683164860883122));
#40304=CARTESIAN_POINT('Ctrl Pts',(-66.51072,-6.54551210047545,-0.861707159351045));
#40305=CARTESIAN_POINT('Ctrl Pts',(-66.51072,-6.50792768344902,-1.03847560235939));
#40306=CARTESIAN_POINT('Ctrl Pts',(-66.51072,-6.47145771003767,-1.21000255226383));
#40307=CARTESIAN_POINT('Ctrl Pts',(-66.51072,-6.42814792670735,-1.37985987693613));
#40308=CARTESIAN_POINT('Ctrl Pts',(-66.51072,-6.37798556320937,-1.54762840486411));
#40309=CARTESIAN_POINT('Ctrl Pts',(-66.51072,-6.32617544917501,-1.72090785099064));
#40310=CARTESIAN_POINT('Ctrl Pts',(-66.51072,-6.26705505663415,-1.89195973976835));
#40311=CARTESIAN_POINT('Ctrl Pts',(-66.51072,-6.20086142651017,-2.06037121308545));
#40312=CARTESIAN_POINT('Ctrl Pts',(-66.51072,-6.13492183835158,-2.22813634654181));
#40313=CARTESIAN_POINT('Ctrl Pts',(-66.51072,-6.06196276652256,-2.39328189639218));
#40314=CARTESIAN_POINT('Ctrl Pts',(-66.51072,-5.98217662776493,-2.55536986618945));
#40315=CARTESIAN_POINT('Ctrl Pts',(-66.51072,-5.94262418782639,-2.63572185201049));
#40316=CARTESIAN_POINT('Ctrl Pts',(-66.51072,-5.90139339549068,-2.71532192202713));
#40317=CARTESIAN_POINT('Ctrl Pts',(-66.51072,-5.85850434682744,-2.79411327911155));
#40318=CARTESIAN_POINT('Ctrl Pts',(-66.51072,-5.84639974950909,-2.81635060261018));
#40319=CARTESIAN_POINT('Ctrl Pts',(-66.51072,-5.83416305274489,-2.83852349344844));
#40320=CARTESIAN_POINT('Ctrl Pts',(-66.51072,-5.8217946791383,-2.8606306375173));
#40321=CARTESIAN_POINT('Ctrl Pts',(-66.51072,-5.81057979104184,-2.88067604969119));
#40322=CARTESIAN_POINT('Ctrl Pts',(-66.51072,-5.79926047745952,-2.90066050695198));
#40323=CARTESIAN_POINT('Ctrl Pts',(-66.51072,-5.78784025721056,-2.92057804100683));
#40324=CARTESIAN_POINT('Ctrl Pts',(-66.51072,-5.69892412862028,-3.0756529853261));
#40325=CARTESIAN_POINT('Ctrl Pts',(-66.51072,-5.60383915857374,-3.22677285815348));
#40326=CARTESIAN_POINT('Ctrl Pts',(-66.51072,-5.5028480490352,-3.37356178930185));
#40327=CARTESIAN_POINT('Ctrl Pts',(-66.51072,-5.40197092766091,-3.52018504051196));
#40328=CARTESIAN_POINT('Ctrl Pts',(-66.51072,-5.29520055505474,-3.66248771572367));
#40329=CARTESIAN_POINT('Ctrl Pts',(-66.51072,-5.18275615628646,-3.80006564228537));
#40330=CARTESIAN_POINT('Ctrl Pts',(-66.51072,-5.0716905546549,-3.93595658351658));
#40331=CARTESIAN_POINT('Ctrl Pts',(-66.51072,-4.9550887580849,-4.06723843117073));
#40332=CARTESIAN_POINT('Ctrl Pts',(-66.51072,-4.83312726292506,-4.19348483441543));
#40333=CARTESIAN_POINT('Ctrl Pts',(-66.51072,-4.80127883984523,-4.22645219725052));
#40334=CARTESIAN_POINT('Ctrl Pts',(-66.51072,-4.76906476512282,-4.2590759661899));
#40335=CARTESIAN_POINT('Ctrl Pts',(-66.51072,-4.73648784413042,-4.29134806370339));
#40336=CARTESIAN_POINT('Ctrl Pts',(-66.51072,-4.64348208285574,-4.38348356656057));
#40337=CARTESIAN_POINT('Ctrl Pts',(-66.51072,-4.54751927645066,-4.47275368008218));
#40338=CARTESIAN_POINT('Ctrl Pts',(-66.51072,-4.44874982948056,-4.5590458483051));
#40339=CARTESIAN_POINT('Ctrl Pts',(-66.51072,-4.40553819643115,-4.59679867190263));
#40340=CARTESIAN_POINT('Ctrl Pts',(-66.51072,-4.36178927514179,-4.63398131817575));
#40341=CARTESIAN_POINT('Ctrl Pts',(-66.51072,-4.31751533581933,-4.6705834958155));
#40342=CARTESIAN_POINT('Ctrl Pts',(-66.51072,-4.29129360863923,-4.69226153781842));
#40343=CARTESIAN_POINT('Ctrl Pts',(-66.51072,-4.26488771593151,-4.71373595681972));
#40344=CARTESIAN_POINT('Ctrl Pts',(-66.51072,-4.23830018127736,-4.73500452368828));
#40345=CARTESIAN_POINT('Ctrl Pts',(-66.51072,-4.21784594893157,-4.75136678570506));
#40346=CARTESIAN_POINT('Ctrl Pts',(-66.51072,-4.19728221990606,-4.7676086836443));
#40347=CARTESIAN_POINT('Ctrl Pts',(-66.51072,-4.17662859394966,-4.78371502962124));
#40348=CARTESIAN_POINT('Ctrl Pts',(-66.51072,-4.0386441282523,-4.89131964823186));
#40349=CARTESIAN_POINT('Ctrl Pts',(-66.51072,-3.89647958119171,-4.99301559213152));
#40350=CARTESIAN_POINT('Ctrl Pts',(-66.51072,-3.75054944970173,-5.08861922337019));
#40351=CARTESIAN_POINT('Ctrl Pts',(-66.51072,-3.6038038756398,-5.18475707787137));
#40352=CARTESIAN_POINT('Ctrl Pts',(-66.51072,-3.45324987084959,-5.27473470522527));
#40353=CARTESIAN_POINT('Ctrl Pts',(-66.51072,-3.29928025831541,-5.35832163598663));
#40354=CARTESIAN_POINT('Ctrl Pts',(-66.51072,-3.146240127214,-5.44140397042612));
#40355=CARTESIAN_POINT('Ctrl Pts',(-66.51072,-2.98982483785502,-5.51817280831344));
#40356=CARTESIAN_POINT('Ctrl Pts',(-66.51072,-2.8304017813007,-5.58835410868057));
#40357=CARTESIAN_POINT('Ctrl Pts',(-66.51072,-2.67408193606954,-5.65716931175488));
#40358=CARTESIAN_POINT('Ctrl Pts',(-66.51072,-2.51486966171192,-5.71965108202682));
#40359=CARTESIAN_POINT('Ctrl Pts',(-66.51072,-2.35310307851583,-5.77549214185151));
#40360=CARTESIAN_POINT('Ctrl Pts',(-66.51072,-2.25436054710213,-5.80957759692495));
#40361=CARTESIAN_POINT('Ctrl Pts',(-66.51072,-2.15466618504803,-5.84118782884412));
#40362=CARTESIAN_POINT('Ctrl Pts',(-66.51072,-2.05409679149563,-5.87024334535353));
#40363=CARTESIAN_POINT('Ctrl Pts',(-86.9228037546341,-4.16423880285026,
4.61932741374069));
#40364=CARTESIAN_POINT('Ctrl Pts',(-86.8897744928952,-4.93115421869368,
3.92796725519045));
#40365=CARTESIAN_POINT('Ctrl Pts',(-86.8237159694174,-6.11319170164878,
2.15655013100907));
#40366=CARTESIAN_POINT('Ctrl Pts',(-86.7246281842008,-6.40055386810954,
-1.02634989594538));
#40367=CARTESIAN_POINT('Ctrl Pts',(-86.625540398984,-5.13269180441595,-3.9591844580739));
#40368=CARTESIAN_POINT('Ctrl Pts',(-86.5264526137674,-2.61763940474365,
-5.93031580654633));
#40369=CARTESIAN_POINT('Ctrl Pts',(-86.4273648285507,0.533459855123279,
-6.46029588895267));
#40370=CARTESIAN_POINT('Ctrl Pts',(-86.3282770433341,3.55493808738742,-5.42058662271333));
#40371=CARTESIAN_POINT('Ctrl Pts',(-86.2291892581173,5.71261075920097,-3.06370552006469));
#40372=CARTESIAN_POINT('Ctrl Pts',(-86.1301014729008,6.48219330078747,0.0375972645595515));
#40373=CARTESIAN_POINT('Ctrl Pts',(-86.031013687684,5.67668603654431,3.12977391169855));
#40374=CARTESIAN_POINT('Ctrl Pts',(-85.9319259024675,3.49181736371615,5.46145112616022));
#40375=CARTESIAN_POINT('Ctrl Pts',(-85.8328381172506,0.45848197210095,6.46606838804796));
#40376=CARTESIAN_POINT('Ctrl Pts',(-85.7337503320341,-2.68625859143277,
5.89951319007443));
#40377=CARTESIAN_POINT('Ctrl Pts',(-85.6346625468174,-5.17827294326576,
3.89945285036088));
#40378=CARTESIAN_POINT('Ctrl Pts',(-85.5355747616006,-6.41203366928947,
0.951875425404776));
#40379=CARTESIAN_POINT('Ctrl Pts',(-85.4364869763841,-6.08775282190871,
-2.22699532849796));
#40380=CARTESIAN_POINT('Ctrl Pts',(-85.3373991911673,-4.28422646215156,
-4.86473497443532));
#40381=CARTESIAN_POINT('Ctrl Pts',(-85.2383114059508,-1.43968826503564,
-6.32040665848384));
#40382=CARTESIAN_POINT('Ctrl Pts',(-85.139223620734,1.75467563421941,-6.24030096387333));
#40383=CARTESIAN_POINT('Ctrl Pts',(-85.0401358355174,4.52267595876155,-4.64388251792204));
#40384=CARTESIAN_POINT('Ctrl Pts',(-84.9410480503007,6.19172428905613,-1.919060449145));
#40385=CARTESIAN_POINT('Ctrl Pts',(-84.8419602650839,6.35626338222264,1.27206858835509));
#40386=CARTESIAN_POINT('Ctrl Pts',(-84.7428724798673,4.9763123584096,4.15410134539831));
#40387=CARTESIAN_POINT('Ctrl Pts',(-84.6437846946507,2.38718153906689,6.02674099139694));
#40388=CARTESIAN_POINT('Ctrl Pts',(-84.544696909434,-0.782003641280745,
6.43496021602791));
#40389=CARTESIAN_POINT('Ctrl Pts',(-84.4456091242173,-3.76117201100048,
5.27956700696203));
#40390=CARTESIAN_POINT('Ctrl Pts',(-84.3465213390006,-5.82642403552263,
2.84130702942041));
#40391=CARTESIAN_POINT('Ctrl Pts',(-84.247433553784,-6.47593007859897,-0.287353952968906));
#40392=CARTESIAN_POINT('Ctrl Pts',(-84.1483457685672,-5.55186853905296,
-3.34619162665173));
#40393=CARTESIAN_POINT('Ctrl Pts',(-84.0492579833507,-3.27877446672824,
-5.59194784252432));
#40394=CARTESIAN_POINT('Ctrl Pts',(-83.950170198134,-0.208980437956675,
-6.47893277120133));
#40395=CARTESIAN_POINT('Ctrl Pts',(-83.8510824129173,2.91159314503785,-5.79162050163479));
#40396=CARTESIAN_POINT('Ctrl Pts',(-83.7519946277006,5.32468710252559,-3.6970190609988));
#40397=CARTESIAN_POINT('Ctrl Pts',(-83.652906842484,6.44395068963483,-0.704089615563853));
#40398=CARTESIAN_POINT('Ctrl Pts',(-83.5538190572673,5.9974172736645,2.4599245359849));
#40399=CARTESIAN_POINT('Ctrl Pts',(-83.4547312720506,4.09358872220742,5.02620871538443));
#40400=CARTESIAN_POINT('Ctrl Pts',(-83.3556434868339,1.19507084710563,6.37118892731869));
#40401=CARTESIAN_POINT('Ctrl Pts',(-83.2565557016173,-1.99383384828571,
6.16805230705936));
#40402=CARTESIAN_POINT('Ctrl Pts',(-83.1574679164006,-4.69826260420316,
4.46615843641225));
#40403=CARTESIAN_POINT('Ctrl Pts',(-83.058380131184,-6.26107407289102,1.67904560121576));
#40404=CARTESIAN_POINT('Ctrl Pts',(-82.9592923459673,-6.30252520045134,
-1.51605368469123));
#40405=CARTESIAN_POINT('Ctrl Pts',(-82.8602045607506,-4.8125438968831,-4.34277145585205));
#40406=CARTESIAN_POINT('Ctrl Pts',(-82.7611167755339,-2.15317642419824,
-6.11425170920097));
#40407=CARTESIAN_POINT('Ctrl Pts',(-82.6620289903173,1.02938518116893,-6.40004756435293));
#40408=CARTESIAN_POINT('Ctrl Pts',(-82.5629412051006,3.96181944861569,-5.13071431028474));
#40409=CARTESIAN_POINT('Ctrl Pts',(-82.4638534198839,5.93158262837659,-2.61468357548884));
#40410=CARTESIAN_POINT('Ctrl Pts',(-82.3647656346672,6.46004764333774,0.536681584365129));
#40411=CARTESIAN_POINT('Ctrl Pts',(-82.2656778494506,5.41880430283928,3.55764003304445));
#40412=CARTESIAN_POINT('Ctrl Pts',(-82.1665900642338,3.06086132475543,5.71413778516117));
#40413=CARTESIAN_POINT('Ctrl Pts',(-82.0675022790172,-0.0408315235521791,
6.4821736681359));
#40414=CARTESIAN_POINT('Ctrl Pts',(-81.9684144938005,-3.13260283765064,
5.67512485666467));
#40415=CARTESIAN_POINT('Ctrl Pts',(-81.8693267085839,-5.46319201810528,
3.48909381509022));
#40416=CARTESIAN_POINT('Ctrl Pts',(-81.7702389233672,-6.46629591799175,
0.455257924866117));
#40417=CARTESIAN_POINT('Ctrl Pts',(-81.6711511381505,-5.89817321217138,
-2.68919977621855));
#40418=CARTESIAN_POINT('Ctrl Pts',(-81.5720633529339,-3.89687039929076,
-5.18021657542632));
#40419=CARTESIAN_POINT('Ctrl Pts',(-81.4729755677172,-0.948678281001003,
-6.41250748119229));
#40420=CARTESIAN_POINT('Ctrl Pts',(-81.3738877825005,2.23003043817884,-6.08664167846161));
#40421=CARTESIAN_POINT('Ctrl Pts',(-81.274799997284,4.86687048935458,-4.28180035931612));
#40422=CARTESIAN_POINT('Ctrl Pts',(-81.1757122120671,6.32112370930806,-1.43653671335388));
#40423=CARTESIAN_POINT('Ctrl Pts',(-81.0766244268506,6.23942530007697,1.75778684770072));
#40424=CARTESIAN_POINT('Ctrl Pts',(-80.9775366416338,4.64162692262079,4.52499084953681));
#40425=CARTESIAN_POINT('Ctrl Pts',(-80.8784488564173,1.91597299894771,6.19268036834564));
#40426=CARTESIAN_POINT('Ctrl Pts',(-80.7793610712004,-1.27523768085627,
6.35562833514629));
#40427=CARTESIAN_POINT('Ctrl Pts',(-80.6802732859839,-4.15658203252233,
4.97424049319116));
#40428=CARTESIAN_POINT('Ctrl Pts',(-80.5811855007671,-6.02793049765148,
2.38417629228067));
#40429=CARTESIAN_POINT('Ctrl Pts',(-80.4820977155505,-6.4345695069531,-0.785212033389358));
#40430=CARTESIAN_POINT('Ctrl Pts',(-80.3830099303339,-5.27769101971328,
-3.76380395047722));
#40431=CARTESIAN_POINT('Ctrl Pts',(-80.2839221451171,-2.83840160478908,
-5.82783999498278));
#40432=CARTESIAN_POINT('Ctrl Pts',(-80.1848343599005,0.290582834254973,
-6.47578599813385));
#40433=CARTESIAN_POINT('Ctrl Pts',(-80.0857465746839,3.34895938802227,-5.55019942835999));
#40434=CARTESIAN_POINT('Ctrl Pts',(-79.9866587894671,5.59358195362901,-3.27598589820315));
#40435=CARTESIAN_POINT('Ctrl Pts',(-79.8875710042505,6.47903616408986,-0.205749997827326));
#40436=CARTESIAN_POINT('Ctrl Pts',(-79.7884832190337,5.79016805316885,2.91448050143638));
#40437=CARTESIAN_POINT('Ctrl Pts',(-79.6893954338172,3.69436369744359,5.32652978478494));
#40438=CARTESIAN_POINT('Ctrl Pts',(-79.5903076486004,0.700876556055815,
6.44430094970444));
#40439=CARTESIAN_POINT('Ctrl Pts',(-79.4912198633839,-2.46291455937789,
5.99619000285969));
#40440=CARTESIAN_POINT('Ctrl Pts',(-79.392132078167,-5.0282491654969,4.09108213152337));
#40441=CARTESIAN_POINT('Ctrl Pts',(-79.2930442929505,-6.37178400105954,
1.19189400578732));
#40442=CARTESIAN_POINT('Ctrl Pts',(-79.1939565077337,-6.16705740917563,
-1.99690900872377));
#40443=CARTESIAN_POINT('Ctrl Pts',(-79.0948687225172,-4.46381531427285,
-4.7004888593904));
#40444=CARTESIAN_POINT('Ctrl Pts',(-78.9957809373004,-1.67592360331519,
-6.26191047149678));
#40445=CARTESIAN_POINT('Ctrl Pts',(-78.8966931520838,1.5191959530824,-6.30176850838938));
#40446=CARTESIAN_POINT('Ctrl Pts',(-78.797605366867,4.34517046399522,-4.81037798057634));
#40447=CARTESIAN_POINT('Ctrl Pts',(-78.6985175816505,6.11532452902266,-2.15012757340671));
#40448=CARTESIAN_POINT('Ctrl Pts',(-78.5994297964337,6.39953351445713,1.03257613497986));
#40449=CARTESIAN_POINT('Ctrl Pts',(-78.5003420112172,5.12873829817387,3.96437714477757));
#40450=CARTESIAN_POINT('Ctrl Pts',(-78.4012542260003,2.61172574664976,5.93288557967174));
#40451=CARTESIAN_POINT('Ctrl Pts',(-78.3021664407838,-0.539902515628905,
6.45977924938676));
#40452=CARTESIAN_POINT('Ctrl Pts',(-78.2030786555671,-3.5603414219296,5.41702977991466));
#40453=CARTESIAN_POINT('Ctrl Pts',(-78.1039908703504,-5.71566322896938,
3.0580118590675));
#40454=CARTESIAN_POINT('Ctrl Pts',(-78.0049030851337,-6.4821525036734,-0.0440635485496543));
#40455=CARTESIAN_POINT('Ctrl Pts',(-77.9058152999171,-5.67356222662317,
-3.13543208152));
#40456=CARTESIAN_POINT('Ctrl Pts',(-77.8067275147004,-3.48636941843915,
-5.46493101103411));
#40457=CARTESIAN_POINT('Ctrl Pts',(-77.7076397294838,-0.452033754894525,
-6.46652210710101));
#40458=CARTESIAN_POINT('Ctrl Pts',(-77.608551944267,2.69214028774311,-5.89683163642142));
#40459=CARTESIAN_POINT('Ctrl Pts',(-77.5094641590505,5.18215892208465,-3.89428704430587));
#40460=CARTESIAN_POINT('Ctrl Pts',(-77.4103763738337,6.41297969776877,-0.945480868762339));
#40461=CARTESIAN_POINT('Ctrl Pts',(-77.3112885886171,6.08552902241152,2.23306497768811));
#40462=CARTESIAN_POINT('Ctrl Pts',(-77.2122008034003,4.27937319172577,4.8690048021263));
#40463=CARTESIAN_POINT('Ctrl Pts',(-77.1131130181838,1.43338480467962,6.32183918483408));
#40464=CARTESIAN_POINT('Ctrl Pts',(-77.014025232967,-1.76089762425562,6.2385480870216));
#40465=CARTESIAN_POINT('Ctrl Pts',(-76.9149374477504,-4.52730461534429,
4.63937017245579));
#40466=CARTESIAN_POINT('Ctrl Pts',(-76.8158496625337,-6.19363490812165,
1.91288507289043));
#40467=CARTESIAN_POINT('Ctrl Pts',(-76.7167618773171,-6.35499170802218,
-1.27840645655423));
#40468=CARTESIAN_POINT('Ctrl Pts',(-76.6176740921003,-4.97216739135669,
-4.15906168618827));
#40469=CARTESIAN_POINT('Ctrl Pts',(-76.5185863068837,-2.38117045277481,
-6.02911850538885));
#40470=CARTESIAN_POINT('Ctrl Pts',(-76.419498521667,0.788420230289574,-6.43417719818628));
#40471=CARTESIAN_POINT('Ctrl Pts',(-76.3204107364504,3.76643495425477,-5.27581372041868));
#40472=CARTESIAN_POINT('Ctrl Pts',(-76.2213229512337,5.82925450561374,-2.83549547451091));
#40473=CARTESIAN_POINT('Ctrl Pts',(-76.122235166017,6.47564030775746,0.293811643297502));
#40474=CARTESIAN_POINT('Ctrl Pts',(-76.0231473808003,5.54852893786079,3.3517263168271));
#40475=CARTESIAN_POINT('Ctrl Pts',(-75.9240595955837,3.27319651525233,5.59521467414165));
#40476=CARTESIAN_POINT('Ctrl Pts',(-75.824971810367,0.202519506547572,6.47913794625935));
#40477=CARTESIAN_POINT('Ctrl Pts',(-75.7258840251503,-2.91736713328106,
5.78871416523925));
#40478=CARTESIAN_POINT('Ctrl Pts',(-75.6267962399337,-5.32837114284346,
3.69170741545199));
#40479=CARTESIAN_POINT('Ctrl Pts',(-75.527708454717,-6.44464960768997,0.697663322306493));
#40480=CARTESIAN_POINT('Ctrl Pts',(-75.4286206695003,-5.99496124137334,
-2.4659039704785));
#40481=CARTESIAN_POINT('Ctrl Pts',(-75.3295328842836,-4.08857452377673,
-5.03028836556254));
#40482=CARTESIAN_POINT('Ctrl Pts',(-75.230445099067,-1.18871686815845,-6.37237749074438));
#40483=CARTESIAN_POINT('Ctrl Pts',(-75.1313573138503,1.99998367272066,-6.1660609781319));
#40484=CARTESIAN_POINT('Ctrl Pts',(-75.0322695286336,4.70271394601358,-4.46147108240762));
#40485=CARTESIAN_POINT('Ctrl Pts',(-74.933181743417,6.26274531336161,-1.67280118877204));
#40486=CARTESIAN_POINT('Ctrl Pts',(-74.8340939582003,6.30101024967761,1.52233784379415));
#40487=CARTESIAN_POINT('Ctrl Pts',(-74.7350061729836,4.8082108683866,4.34756839190818));
#40488=CARTESIAN_POINT('Ctrl Pts',(-74.635918387767,2.14707818808318,6.11639582854541));
#40489=CARTESIAN_POINT('Ctrl Pts',(-74.5368306025503,-1.03576683208741,
6.39901787360667));
#40490=CARTESIAN_POINT('Ctrl Pts',(-74.4377428173336,-3.96693385537629,
5.1267610110341));
#40491=CARTESIAN_POINT('Ctrl Pts',(-74.338655032117,-5.93418705602312,2.60876726852318));
#40492=CARTESIAN_POINT('Ctrl Pts',(-74.2395672469002,-6.45950924950371,
-0.543123312670282));
#40493=CARTESIAN_POINT('Ctrl Pts',(-74.1404794616836,-5.41525391029054,
-3.5630419256968));
#40494=CARTESIAN_POINT('Ctrl Pts',(-74.0413916764669,-3.05516163314319,
-5.71718725183634));
#40495=CARTESIAN_POINT('Ctrl Pts',(-73.9423038912502,0.047295562592674,
-6.48212972771674));
#40496=CARTESIAN_POINT('Ctrl Pts',(-73.8432161060336,3.13826054590585,-5.67199818610696));
#40497=CARTESIAN_POINT('Ctrl Pts',(-73.744128320817,5.4666686453549,-3.48364415506002));
#40498=CARTESIAN_POINT('Ctrl Pts',(-73.6450405356003,6.4667466886019,-0.448809472545249));
#40499=CARTESIAN_POINT('Ctrl Pts',(-73.5459527503835,5.89548859469092,2.6950801299886));
#40500=CARTESIAN_POINT('Ctrl Pts',(-73.446864965167,3.89170272118268,5.18409998043338));
#40501=CARTESIAN_POINT('Ctrl Pts',(-73.3477771799502,0.94228322147271,6.4134503200478));
#40502=CARTESIAN_POINT('Ctrl Pts',(-73.2486893947337,-2.23609896204665,
6.0844148534698));
#40503=CARTESIAN_POINT('Ctrl Pts',(-73.1496016095169,-4.87113790444004,
4.27694496026283));
#40504=CARTESIAN_POINT('Ctrl Pts',(-73.0505138243002,-6.32255308872057,
1.43023253965916));
#40505=CARTESIAN_POINT('Ctrl Pts',(-72.9514260390836,-6.23766932303337,
-1.76400796304286));
#40506=CARTESIAN_POINT('Ctrl Pts',(-72.8523382538668,-4.63711226892121,
-4.52961725564207));
#40507=CARTESIAN_POINT('Ctrl Pts',(-72.7532504686503,-1.90979667128091,
-6.19458790813032));
#40508=CARTESIAN_POINT('Ctrl Pts',(-72.6541626834335,1.28157491443408,-6.35435350101671));
#40509=CARTESIAN_POINT('Ctrl Pts',(-72.5550748982169,4.16154030589149,-4.97009305341768));
#40510=CARTESIAN_POINT('Ctrl Pts',(-72.4559871130002,6.03030501425848,-2.37816402129864));
#40511=CARTESIAN_POINT('Ctrl Pts',(-72.3568993277835,6.4337832898522,0.791628231184674));
#40512=CARTESIAN_POINT('Ctrl Pts',(-72.2578115425668,5.27393510953157,3.76906502167849));
#40513=CARTESIAN_POINT('Ctrl Pts',(-72.1587237573503,2.83258863931502,5.83066756706414));
#40514=CARTESIAN_POINT('Ctrl Pts',(-72.0596359721335,-0.297040379296998,
6.47549300750585));
#40515=CARTESIAN_POINT('Ctrl Pts',(-71.9605481869169,-3.35449241237668,
5.54685706797077));
#40516=CARTESIAN_POINT('Ctrl Pts',(-71.8614604017001,-5.59684600365713,
3.27040631856919));
#40517=CARTESIAN_POINT('Ctrl Pts',(-71.7623726164835,-6.47923811768414,
0.19928896492046));
#40518=CARTESIAN_POINT('Ctrl Pts',(-71.6632848312669,-5.78725883820755,
-2.92025303985438));
#40519=CARTESIAN_POINT('Ctrl Pts',(-71.5641970460501,-3.68905021568418,
-5.33021117624344));
#40520=CARTESIAN_POINT('Ctrl Pts',(-71.4651092608335,-0.694449915114697,
-6.44499666350474));
#40521=CARTESIAN_POINT('Ctrl Pts',(-71.3660214756168,2.46889276854356,-5.99373098951091));
#40522=CARTESIAN_POINT('Ctrl Pts',(-71.2669336904001,5.03232631507441,-4.0860658995909));
#40523=CARTESIAN_POINT('Ctrl Pts',(-71.1678459051835,6.37296939622566,-1.1855394350089));
#40524=CARTESIAN_POINT('Ctrl Pts',(-71.0687581199668,6.16506301417589,2.00305783951203));
#40525=CARTESIAN_POINT('Ctrl Pts',(-70.9696703347502,4.4591257413993,4.70493786351959));
#40526=CARTESIAN_POINT('Ctrl Pts',(-70.8705825495335,1.66967835836243,6.26357859827801));
#40527=CARTESIAN_POINT('Ctrl Pts',(-70.7714947643168,-1.5254793560455,6.30025042450449));
#40528=CARTESIAN_POINT('Ctrl Pts',(-70.6724069791001,-4.34996523899484,
4.8060425608526));
#40529=CARTESIAN_POINT('Ctrl Pts',(-70.5733191938834,-6.11746560750284,
2.14402826898574));
#40530=CARTESIAN_POINT('Ctrl Pts',(-70.4742314086668,-6.39850064192973,
-1.03895727169834));
#40531=CARTESIAN_POINT('Ctrl Pts',(-70.3751436234501,-5.12478244935701,
-3.96948957977628));
#40532=CARTESIAN_POINT('Ctrl Pts',(-70.2760558382335,-2.60580814184455,
-5.93548705710717));
#40533=CARTESIAN_POINT('Ctrl Pts',(-70.1769680530168,0.546343974688648,
-6.45923764375577));
#40534=CARTESIAN_POINT('Ctrl Pts',(-70.0778802678002,3.56574154367478,-5.4134766944083));
#40535=CARTESIAN_POINT('Ctrl Pts',(-69.9787924825834,5.71870985338321,-3.05231064769102));
#40536=CARTESIAN_POINT('Ctrl Pts',(-69.8797046973668,6.48210534027158,0.0505275648778713));
#40537=CARTESIAN_POINT('Ctrl Pts',(-69.7806169121501,5.67043273550486,3.14108823010512));
#40538=CARTESIAN_POINT('Ctrl Pts',(-69.6815291269334,3.4809180256302,5.46840492063578));
#40539=CARTESIAN_POINT('Ctrl Pts',(-69.5824413417167,0.445585078619785,
6.46696966243845));
#40540=CARTESIAN_POINT('Ctrl Pts',(-69.4833535565002,-2.69801930222453,
5.89414408731404));
#40541=CARTESIAN_POINT('Ctrl Pts',(-69.3842657712834,-5.18603974998983,
3.88911743056271));
#40542=CARTESIAN_POINT('Ctrl Pts',(-69.2851779860668,-6.41391934791292,
0.939085339928392));
#40543=CARTESIAN_POINT('Ctrl Pts',(-69.1860902008501,-6.08329917191227,
-2.23913239050336));
#40544=CARTESIAN_POINT('Ctrl Pts',(-69.0870024156334,-4.27451566553321,
-4.87326979575939));
#40545=CARTESIAN_POINT('Ctrl Pts',(-68.9879146304167,-1.42707991907126,
-6.32326542080269));
#40546=CARTESIAN_POINT('Ctrl Pts',(-68.8888268452001,1.76711786327968,-6.23678900830517));
#40547=CARTESIAN_POINT('Ctrl Pts',(-68.7897390599834,4.5319287698749,-4.63485321262994));
#40548=CARTESIAN_POINT('Ctrl Pts',(-68.6906512747668,6.19553936809527,-1.90670779478191));
#40549=CARTESIAN_POINT('Ctrl Pts',(-68.5915634895501,6.35371371436876,1.28474305349599));
#40550=CARTESIAN_POINT('Ctrl Pts',(-68.4924757043333,4.96801747972696,4.16401789144663));
#40551=CARTESIAN_POINT('Ctrl Pts',(-68.3933879191168,2.37515699892946,6.03149002309199));
#40552=CARTESIAN_POINT('Ctrl Pts',(-68.2943001338999,-0.794836035946308,
6.43338778381987));
#40553=CARTESIAN_POINT('Ctrl Pts',(-68.1952123486834,-3.77169415073787,
5.27205518392761));
#40554=CARTESIAN_POINT('Ctrl Pts',(-68.0961245634667,-5.83207918173385,
2.82968110720637));
#40555=CARTESIAN_POINT('Ctrl Pts',(-67.99703677825,-6.47534409183691,-0.300269056217778));
#40556=CARTESIAN_POINT('Ctrl Pts',(-67.8979489930334,-5.54518383041795,
-3.35725764403967));
#40557=CARTESIAN_POINT('Ctrl Pts',(-67.7988612078167,-3.26761528590833,
-5.59847600248888));
#40558=CARTESIAN_POINT('Ctrl Pts',(-67.6997734226,-0.196058420264034,-6.47933655521552));
#40559=CARTESIAN_POINT('Ctrl Pts',(-67.6006856373834,2.92313831475997,-5.78580232210167));
#40560=CARTESIAN_POINT('Ctrl Pts',(-67.5015978521667,5.33204969326613,-3.6863915925369));
#40561=CARTESIAN_POINT('Ctrl Pts',(-67.4025100669501,6.44534250489529,-0.691237361863573));
#40562=CARTESIAN_POINT('Ctrl Pts',(-67.3034222817333,5.99249846114462,2.47188303450135));
#40563=CARTESIAN_POINT('Ctrl Pts',(-67.2043344965166,4.08355785429189,5.03435879238504));
#40564=CARTESIAN_POINT('Ctrl Pts',(-67.1052467113001,1.18235847344737,6.37356827685746));
#40565=CARTESIAN_POINT('Ctrl Pts',(-67.0061589260833,-2.0061249511844,6.16404616060605));
#40566=CARTESIAN_POINT('Ctrl Pts',(-66.9070711408667,-4.70717390764343,
4.4568144926439));
#40567=CARTESIAN_POINT('Ctrl Pts',(-66.80798335565,-6.26438336148857,1.66648367303066));
#40568=CARTESIAN_POINT('Ctrl Pts',(-66.7088955704333,-6.29954365018284,
-1.52847431346428));
#40569=CARTESIAN_POINT('Ctrl Pts',(-66.6098077852167,-4.80376045256683,
-4.35266662668044));
#40570=CARTESIAN_POINT('Ctrl Pts',(-66.5437492617389,-3.02869324528072,
-5.529215668825));
#40571=CARTESIAN_POINT('Ctrl Pts',(-66.51072,-2.05409679149563,-5.87024334535353));
#40572=CARTESIAN_POINT('Ctrl Pts',(-86.7854425030894,-4.32354126137468,
4.79603923277341));
#40573=CARTESIAN_POINT('Ctrl Pts',(-86.7524132413505,-5.11979493494255,
4.07823117385119));
#40574=CARTESIAN_POINT('Ctrl Pts',(-86.6863547178727,-6.34705112076694,
2.23904869895045));
#40575=CARTESIAN_POINT('Ctrl Pts',(-86.5872669326561,-6.6454062926175,-1.06561278875027));
#40576=CARTESIAN_POINT('Ctrl Pts',(-86.4881791474394,-5.32904231695911,
-4.11064258710606));
#40577=CARTESIAN_POINT('Ctrl Pts',(-86.3890913622227,-2.71777688783439,
-6.15717933011816));
#40578=CARTESIAN_POINT('Ctrl Pts',(-86.2900035770061,0.553867298228359,
-6.70743373733954));
#40579=CARTESIAN_POINT('Ctrl Pts',(-86.1909157917893,3.69093181974381,-5.62795051717873));
#40580=CARTESIAN_POINT('Ctrl Pts',(-86.0918280065727,5.93114600216325,-3.18090720917224));
#40581=CARTESIAN_POINT('Ctrl Pts',(-85.992740221356,6.73016883205126,0.0390355434291301));
#40582=CARTESIAN_POINT('Ctrl Pts',(-85.8936524361394,5.89384698352793,3.24950303924472));
#40583=CARTESIAN_POINT('Ctrl Pts',(-85.7945646509227,3.62539642032013,5.67037828732898));
#40584=CARTESIAN_POINT('Ctrl Pts',(-85.695476865706,0.476021145237448,6.71342706269893));
#40585=CARTESIAN_POINT('Ctrl Pts',(-85.5963890804893,-2.78902109332259,
6.12519836322853));
#40586=CARTESIAN_POINT('Ctrl Pts',(-85.4973012952727,-5.37636715683683,
4.04862595386722));
#40587=CARTESIAN_POINT('Ctrl Pts',(-85.398213510056,-6.65732525222178,0.988289306225514));
#40588=CARTESIAN_POINT('Ctrl Pts',(-85.2991257248394,-6.32063907971779,
-2.31218876906367));
#40589=CARTESIAN_POINT('Ctrl Pts',(-85.2000379396226,-4.44811903426561,
-5.05083483042026));
#40590=CARTESIAN_POINT('Ctrl Pts',(-85.1009501544061,-1.49476336783044,
-6.56219306105075));
#40591=CARTESIAN_POINT('Ctrl Pts',(-85.0018623691893,1.82180054123787,-6.47902293265117));
#40592=CARTESIAN_POINT('Ctrl Pts',(-84.9027745839727,4.6956903879165,-4.82153368953529));
#40593=CARTESIAN_POINT('Ctrl Pts',(-84.8036867987559,6.42858796293502,-1.99247387764403));
#40594=CARTESIAN_POINT('Ctrl Pts',(-84.7045990135393,6.59942147947774,1.32073142041886));
#40595=CARTESIAN_POINT('Ctrl Pts',(-84.6055112283226,5.16668059390505,4.31301599669751));
#40596=CARTESIAN_POINT('Ctrl Pts',(-84.5064234431061,2.47850288400448,6.25729324890973));
#40597=CARTESIAN_POINT('Ctrl Pts',(-84.4073356578892,-0.811919097268936,
6.6811288512701));
#40598=CARTESIAN_POINT('Ctrl Pts',(-84.3082478726727,-3.90505519749678,
5.48153621285338));
#40599=CARTESIAN_POINT('Ctrl Pts',(-84.2091600874558,-6.04931319179036,
2.95000089080505));
#40600=CARTESIAN_POINT('Ctrl Pts',(-84.1100723022394,-6.72366601104527,
-0.298346644152522));
#40601=CARTESIAN_POINT('Ctrl Pts',(-84.0109845170225,-5.76425460756333,
-3.47419978806038));
#40602=CARTESIAN_POINT('Ctrl Pts',(-83.9118967318061,-3.4042035927283,-5.80586714000668));
#40603=CARTESIAN_POINT('Ctrl Pts',(-83.8128089465891,-0.216974959675104,
-6.72678357129485));
#40604=CARTESIAN_POINT('Ctrl Pts',(-83.7137211613727,3.02297579338882,-6.01317825286643));
#40605=CARTESIAN_POINT('Ctrl Pts',(-83.6146333761559,5.52838237228895,-3.83844808404757));
#40606=CARTESIAN_POINT('Ctrl Pts',(-83.5155455909393,6.6904632543721,-0.731024479795027));
#40607=CARTESIAN_POINT('Ctrl Pts',(-83.4164578057226,6.22684775585439,2.55402865558983));
#40608=CARTESIAN_POINT('Ctrl Pts',(-83.3173700205059,4.25018847032688,5.21848573006226));
#40609=CARTESIAN_POINT('Ctrl Pts',(-83.2182822352893,1.24078813976536,6.61491799952051));
#40610=CARTESIAN_POINT('Ctrl Pts',(-83.1191944500726,-2.07010772424683,
6.40401041209152));
#40611=CARTESIAN_POINT('Ctrl Pts',(-83.0201066648559,-4.8779940795284,4.63701079449345));
#40612=CARTESIAN_POINT('Ctrl Pts',(-82.9210188796392,-6.50059071447566,
1.74327729034592));
#40613=CARTESIAN_POINT('Ctrl Pts',(-82.8219310944226,-6.54362754997485,
-1.57405013750295));
#40614=CARTESIAN_POINT('Ctrl Pts',(-82.7228433092059,-4.99664718942376,
-4.50890365971447));
#40615=CARTESIAN_POINT('Ctrl Pts',(-82.6237555239892,-2.23554593138812,
-6.34815167878155));
#40616=CARTESIAN_POINT('Ctrl Pts',(-82.5246677387726,1.06876418844788,-6.64488062027108));
#40617=CARTESIAN_POINT('Ctrl Pts',(-82.4255799535559,4.11337837889662,-5.32698917402587));
#40618=CARTESIAN_POINT('Ctrl Pts',(-82.3264921683392,6.15849461406638,-2.71470798368413));
#40619=CARTESIAN_POINT('Ctrl Pts',(-82.2274043831226,6.70717599511822,0.557212274337937));
#40620=CARTESIAN_POINT('Ctrl Pts',(-82.1283165979058,5.62610001487058,3.69373712800955));
#40621=CARTESIAN_POINT('Ctrl Pts',(-82.0292288126892,3.17795420951081,5.93273144431935));
#40622=CARTESIAN_POINT('Ctrl Pts',(-81.9301410274726,-0.0423935286136112,
6.73014844835495));
#40623=CARTESIAN_POINT('Ctrl Pts',(-81.8310532422558,-3.25244018542155,
5.89222608089828));
#40624=CARTESIAN_POINT('Ctrl Pts',(-81.7319654570393,-5.67218577688769,
3.62256868266649));
#40625=CARTESIAN_POINT('Ctrl Pts',(-81.6328776718224,-6.71366329677356,
0.47267376246034));
#40626=CARTESIAN_POINT('Ctrl Pts',(-81.5337898866059,-6.1238071246307,-2.7920747927814));
#40627=CARTESIAN_POINT('Ctrl Pts',(-81.4347021013891,-4.04594471143955,
-5.37838514241379));
#40628=CARTESIAN_POINT('Ctrl Pts',(-81.3356143161726,-0.98496985544406,
-6.6578171897424));
#40629=CARTESIAN_POINT('Ctrl Pts',(-81.2365265309558,2.31533998650325,-6.31948542961072));
#40630=CARTESIAN_POINT('Ctrl Pts',(-81.1374387457392,5.05305203920794,-4.44560012115568));
#40631=CARTESIAN_POINT('Ctrl Pts',(-81.0383509605224,6.56293754256869,-1.49149125391514));
#40632=CARTESIAN_POINT('Ctrl Pts',(-80.9392631753059,6.47811377044076,1.82503077381967));
#40633=CARTESIAN_POINT('Ctrl Pts',(-80.8401753900891,4.81919180670493,4.69809383456215));
#40634=CARTESIAN_POINT('Ctrl Pts',(-80.7410876048726,1.98926831740783,6.42958061692366));
#40635=CARTESIAN_POINT('Ctrl Pts',(-80.6419998196558,-1.32402174617554,
6.59876213875127));
#40636=CARTESIAN_POINT('Ctrl Pts',(-80.5429120344392,-4.31559158221147,
5.16452946972989));
#40637=CARTESIAN_POINT('Ctrl Pts',(-80.4438242492225,-6.25852825958411,
2.47538267186104));
#40638=CARTESIAN_POINT('Ctrl Pts',(-80.3447364640058,-6.68072319566625,
-0.815250226034837));
#40639=CARTESIAN_POINT('Ctrl Pts',(-80.2456486787892,-5.47958845993628,
-3.90778782150415));
#40640=CARTESIAN_POINT('Ctrl Pts',(-80.1465608935725,-2.94698431950113,
-6.0507833186107));
#40641=CARTESIAN_POINT('Ctrl Pts',(-80.0474731083558,0.301699045906918,
-6.72351641879915));
#40642=CARTESIAN_POINT('Ctrl Pts',(-79.9483853231392,3.47707342981191,-5.76252164523996));
#40643=CARTESIAN_POINT('Ctrl Pts',(-79.8492975379224,5.8075637638367,-3.40130834784702));
#40644=CARTESIAN_POINT('Ctrl Pts',(-79.7502097527058,6.726890919466,-0.213620939444066));
#40645=CARTESIAN_POINT('Ctrl Pts',(-79.6511219674891,6.01167024115772,3.02597360526186));
#40646=CARTESIAN_POINT('Ctrl Pts',(-79.5520341822725,3.8356911398764,5.53029554613826));
#40647=CARTESIAN_POINT('Ctrl Pts',(-79.4529463970557,0.727688505078893,
6.69082691359887));
#40648=CARTESIAN_POINT('Ctrl Pts',(-79.3538586118392,-2.55713306197095,
6.22557353595137));
#40649=CARTESIAN_POINT('Ctrl Pts',(-79.2547708266223,-5.22060423735031,
4.2475859903153));
#40650=CARTESIAN_POINT('Ctrl Pts',(-79.1556830414058,-6.61553583773633,
1.23748976876148));
#40651=CARTESIAN_POINT('Ctrl Pts',(-79.056595256189,-6.40297745450795,-2.07330052458051));
#40652=CARTESIAN_POINT('Ctrl Pts',(-78.9575074709725,-4.6345780364962,-4.8803054998422));
#40653=CARTESIAN_POINT('Ctrl Pts',(-78.8584196857557,-1.74003586078818,
-6.50145910941029));
#40654=CARTESIAN_POINT('Ctrl Pts',(-78.7593319005392,1.57731261299649,-6.54284191074835));
#40655=CARTESIAN_POINT('Ctrl Pts',(-78.6602441153223,4.5113944416279,-4.99439841624713));
#40656=CARTESIAN_POINT('Ctrl Pts',(-78.5611563301058,6.34926553919752,-2.23238044717335));
#40657=CARTESIAN_POINT('Ctrl Pts',(-78.462068544889,6.64434690545786,1.0720772118161));
#40658=CARTESIAN_POINT('Ctrl Pts',(-78.3629807596725,5.32493756980748,4.11603391941998));
#40659=CARTESIAN_POINT('Ctrl Pts',(-78.2638929744557,2.71163700345574,6.15984740960786));
#40660=CARTESIAN_POINT('Ctrl Pts',(-78.1648051892392,-0.560556421942884,
6.70689733378866));
#40661=CARTESIAN_POINT('Ctrl Pts',(-78.0657174040223,-3.69654185820417,
5.62425760778321));
#40662=CARTESIAN_POINT('Ctrl Pts',(-77.9666296188058,-5.93431524379843,
3.17499573785298));
#40663=CARTESIAN_POINT('Ctrl Pts',(-77.867541833589,-6.73012647424846,-0.0457491943417124));
#40664=CARTESIAN_POINT('Ctrl Pts',(-77.7684540483724,-5.890603672631,-3.25537766167755));
#40665=CARTESIAN_POINT('Ctrl Pts',(-77.6693662631557,-3.6197400645466,-5.67399129478351));
#40666=CARTESIAN_POINT('Ctrl Pts',(-77.570278477939,-0.469326252251199,
-6.71389813872022));
#40667=CARTESIAN_POINT('Ctrl Pts',(-77.4711906927223,2.79512779322348,-6.12241422706049));
#40668=CARTESIAN_POINT('Ctrl Pts',(-77.3721029075058,5.38040179331176,-4.04326253051796));
#40669=CARTESIAN_POINT('Ctrl Pts',(-77.273015122289,6.65830747090767,-0.981650126581718));
#40670=CARTESIAN_POINT('Ctrl Pts',(-77.1739273370724,6.31833020903619,2.31849061195935));
#40671=CARTESIAN_POINT('Ctrl Pts',(-77.0748395518557,4.44308010255877,5.05526799986008));
#40672=CARTESIAN_POINT('Ctrl Pts',(-76.975751766639,1.48821876935064,6.56368038852559));
#40673=CARTESIAN_POINT('Ctrl Pts',(-76.8766639814223,-1.82826055276051,
6.47720299970463));
#40674=CARTESIAN_POINT('Ctrl Pts',(-76.7775761962058,-4.70049611320452,
4.81684872483164));
#40675=CARTESIAN_POINT('Ctrl Pts',(-76.678488410989,-6.4305716725049,1.98606226310769));
#40676=CARTESIAN_POINT('Ctrl Pts',(-76.5794006257724,-6.59810115753248,
-1.32731174300973));
#40677=CARTESIAN_POINT('Ctrl Pts',(-76.4803128405556,-5.1623770616321,-4.31816609473252));
#40678=CARTESIAN_POINT('Ctrl Pts',(-76.381225055339,-2.47226184432355,-6.25976171441573));
#40679=CARTESIAN_POINT('Ctrl Pts',(-76.2821372701223,0.818581152124673,
-6.68031587917437));
#40680=CARTESIAN_POINT('Ctrl Pts',(-76.1830494849057,3.91051947401727,-5.47763934478116));
#40681=CARTESIAN_POINT('Ctrl Pts',(-76.083961699689,6.05225194117708,-2.94396701555592));
#40682=CARTESIAN_POINT('Ctrl Pts',(-75.9848739144723,6.72336515505478,0.305051372654104));
#40683=CARTESIAN_POINT('Ctrl Pts',(-75.8857861292556,5.76078725032604,3.47994620714801));
#40684=CARTESIAN_POINT('Ctrl Pts',(-75.786698344039,3.39841225738424,5.80925894387774));
#40685=CARTESIAN_POINT('Ctrl Pts',(-75.6876105588223,0.210266866105867,
6.72699659530022));
#40686=CARTESIAN_POINT('Ctrl Pts',(-75.5885227736056,-3.02897066486332,
6.01016073491886));
#40687=CARTESIAN_POINT('Ctrl Pts',(-75.489434988389,-5.5322073451296,3.83293324213415));
#40688=CARTESIAN_POINT('Ctrl Pts',(-75.3903472031723,-6.69118890945404,
0.724352349455895));
#40689=CARTESIAN_POINT('Ctrl Pts',(-75.2912594179557,-6.22429776834097,
-2.56023683263652));
#40690=CARTESIAN_POINT('Ctrl Pts',(-75.1921716327389,-4.24498245433352,
-5.22272144677116));
#40691=CARTESIAN_POINT('Ctrl Pts',(-75.0930838475223,-1.23419109011172,
-6.61615203129823));
#40692=CARTESIAN_POINT('Ctrl Pts',(-74.9939960623057,2.07649280948173,-6.40194290511355));
#40693=CARTESIAN_POINT('Ctrl Pts',(-74.8949082770889,4.88261570688864,-4.63214412632067));
#40694=CARTESIAN_POINT('Ctrl Pts',(-74.7958204918723,6.50232588805105,-1.73679399864925));
#40695=CARTESIAN_POINT('Ctrl Pts',(-74.6967327066555,6.54205464494003,1.58057469636253));
#40696=CARTESIAN_POINT('Ctrl Pts',(-74.5976449214389,4.99214840143916,4.51388410198705));
#40697=CARTESIAN_POINT('Ctrl Pts',(-74.4985571362223,2.22921440797812,6.35037782115567));
#40698=CARTESIAN_POINT('Ctrl Pts',(-74.3994693510056,-1.07538996866078,
6.64381153882819));
#40699=CARTESIAN_POINT('Ctrl Pts',(-74.3003815657889,-4.1186884366776,5.3228846417841));
#40700=CARTESIAN_POINT('Ctrl Pts',(-74.2012937805723,-6.16119867378176,
2.70856534910143));
#40701=CARTESIAN_POINT('Ctrl Pts',(-74.1022059953555,-6.70661700509232,
-0.563900430190774));
#40702=CARTESIAN_POINT('Ctrl Pts',(-74.0031182101389,-5.6224138024785,-3.69934566942076));
#40703=CARTESIAN_POINT('Ctrl Pts',(-73.9040304249222,-3.17203647687603,
-5.93589756797832));
#40704=CARTESIAN_POINT('Ctrl Pts',(-73.8049426397056,0.0491048486963081,
-6.73010282700029));
#40705=CARTESIAN_POINT('Ctrl Pts',(-73.7058548544888,3.25831432863099,-5.88897979993147));
#40706=CARTESIAN_POINT('Ctrl Pts',(-73.6067670692723,5.6757954020979,-3.61691054654209));
#40707=CARTESIAN_POINT('Ctrl Pts',(-73.5076792840555,6.71413131155964,-0.465978625365368));
#40708=CARTESIAN_POINT('Ctrl Pts',(-73.4085914988389,6.12101980742883,2.79818009878328));
#40709=CARTESIAN_POINT('Ctrl Pts',(-73.3095037136222,4.04057934442206,5.38241710661602));
#40710=CARTESIAN_POINT('Ctrl Pts',(-73.2104159284055,0.978330153676572,
6.65879609678583));
#40711=CARTESIAN_POINT('Ctrl Pts',(-73.111328143189,-2.32164066102752,6.31717341769455));
#40712=CARTESIAN_POINT('Ctrl Pts',(-73.0122403579722,-5.0574827037483,4.44055897939096));
#40713=CARTESIAN_POINT('Ctrl Pts',(-72.9131525727555,-6.56442160272008,
1.48494591480795));
#40714=CARTESIAN_POINT('Ctrl Pts',(-72.8140647875389,-6.47629061870488,
-1.83148987718692));
#40715=CARTESIAN_POINT('Ctrl Pts',(-72.7149770023222,-4.81450444546676,
-4.70289722328094));
#40716=CARTESIAN_POINT('Ctrl Pts',(-72.6158892171056,-1.9828557150631,-6.4315611294152));
#40717=CARTESIAN_POINT('Ctrl Pts',(-72.5168014318888,1.33060140986772,-6.59743853599417));
#40718=CARTESIAN_POINT('Ctrl Pts',(-72.4177136466722,4.32073953373673,-5.16022337014276));
#40719=CARTESIAN_POINT('Ctrl Pts',(-72.3186258614555,6.26099361304058,-2.46914040216998));
#40720=CARTESIAN_POINT('Ctrl Pts',(-72.2195380762389,6.67990690192397,0.821911874711229));
#40721=CARTESIAN_POINT('Ctrl Pts',(-72.1204502910221,5.47568886785872,3.91325015435648));
#40722=CARTESIAN_POINT('Ctrl Pts',(-72.0213625058056,2.94094897972646,6.05371905912464));
#40723=CARTESIAN_POINT('Ctrl Pts',(-71.9222747205888,-0.308403623564008,
6.72321221984963));
#40724=CARTESIAN_POINT('Ctrl Pts',(-71.8231869353721,-3.48281811935279,
5.75905142325286));
#40725=CARTESIAN_POINT('Ctrl Pts',(-71.7240991501555,-5.81095267970918,
3.39551532205993));
#40726=CARTESIAN_POINT('Ctrl Pts',(-71.6250113649388,-6.72710059877092,
0.206912740494278));
#40727=CARTESIAN_POINT('Ctrl Pts',(-71.5259235797222,-6.00864973452521,
-3.03196697144825));
#40728=CARTESIAN_POINT('Ctrl Pts',(-71.4268357945055,-3.83017439150629,
-5.53411776878775));
#40729=CARTESIAN_POINT('Ctrl Pts',(-71.3277480092887,-0.721016013755397,
-6.69154924184759));
#40730=CARTESIAN_POINT('Ctrl Pts',(-71.2286602240722,2.56333996681492,-6.22302045334035));
#40731=CARTESIAN_POINT('Ctrl Pts',(-71.1295724388554,5.22483735779844,-4.24237786302878));
#40732=CARTESIAN_POINT('Ctrl Pts',(-71.0304846536388,6.61676658005308,-1.23089210463616));
#40733=CARTESIAN_POINT('Ctrl Pts',(-70.9313968684221,6.40090676416547,2.0796845781569));
#40734=CARTESIAN_POINT('Ctrl Pts',(-70.8323090832055,4.62970906457193,4.88492470009349));
#40735=CARTESIAN_POINT('Ctrl Pts',(-70.7332212979887,1.73355170473494,6.50319105018249));
#40736=CARTESIAN_POINT('Ctrl Pts',(-70.6341335127722,-1.58383638679021,
6.54126575274558));
#40737=CARTESIAN_POINT('Ctrl Pts',(-70.5350457275554,-4.51637264017302,
4.98989714555916));
#40738=CARTESIAN_POINT('Ctrl Pts',(-70.4359579423388,-6.35148852437948,
2.22604781458953));
#40739=CARTESIAN_POINT('Ctrl Pts',(-70.3368701571221,-6.64327452051517,
-1.07870245815835));
#40740=CARTESIAN_POINT('Ctrl Pts',(-70.2377823719054,-5.32083039046614,
-4.12134193000955));
#40741=CARTESIAN_POINT('Ctrl Pts',(-70.1386945866887,-2.7054930213848,-6.16254840625216));
#40742=CARTESIAN_POINT('Ctrl Pts',(-70.0396068014721,0.567244298250361,
-6.7063350090989));
#40743=CARTESIAN_POINT('Ctrl Pts',(-69.9405190162554,3.70214856096237,-5.62056859941476));
#40744=CARTESIAN_POINT('Ctrl Pts',(-69.8414312310388,5.93747841646568,-3.16907642731557));
#40745=CARTESIAN_POINT('Ctrl Pts',(-69.7423434458221,6.73007750661633,0.0524604908432818));
#40746=CARTESIAN_POINT('Ctrl Pts',(-69.6432556606054,5.88735446320337,3.26125018555189));
#40747=CARTESIAN_POINT('Ctrl Pts',(-69.5441678753887,3.6140801293562,5.67759809838248));
#40748=CARTESIAN_POINT('Ctrl Pts',(-69.445080090172,0.462630882635026,6.71436281523369));
#40749=CARTESIAN_POINT('Ctrl Pts',(-69.3459923049555,-2.80123170870239,
6.11962386608269));
#40750=CARTESIAN_POINT('Ctrl Pts',(-69.2469045197386,-5.3844310818254,4.0378951538179));
#40751=CARTESIAN_POINT('Ctrl Pts',(-69.1478167345221,-6.65928306725597,
0.975009937555351));
#40752=CARTESIAN_POINT('Ctrl Pts',(-69.0487289493054,-6.31601505587215,
-2.3247901329279));
#40753=CARTESIAN_POINT('Ctrl Pts',(-68.9496411640887,-4.43803675228133,
-5.0596961503157));
#40754=CARTESIAN_POINT('Ctrl Pts',(-68.850553378872,-1.48167269109562,-6.56516118498099));
#40755=CARTESIAN_POINT('Ctrl Pts',(-68.7514655936554,1.83471874628623,-6.4753766276418));
#40756=CARTESIAN_POINT('Ctrl Pts',(-68.6523778084387,4.70529716421494,-4.81215896924662));
#40757=CARTESIAN_POINT('Ctrl Pts',(-68.5532900232221,6.43254898736757,-1.9796486739622));
#40758=CARTESIAN_POINT('Ctrl Pts',(-68.4542022380054,6.59677427438435,1.33389074571141));
#40759=CARTESIAN_POINT('Ctrl Pts',(-68.3551144527886,5.15806839562815,4.32331189903167));
#40760=CARTESIAN_POINT('Ctrl Pts',(-68.256026667572,2.46601834651887,6.26222395424562));
#40761=CARTESIAN_POINT('Ctrl Pts',(-68.1569388823553,-0.825242393661263,
6.67949626585557));
#40762=CARTESIAN_POINT('Ctrl Pts',(-68.0578510971387,-3.91597986043431,
5.47373702592509));
#40763=CARTESIAN_POINT('Ctrl Pts',(-67.9587633119221,-6.0551846749451,2.93793022032393));
#40764=CARTESIAN_POINT('Ctrl Pts',(-67.8596755267053,-6.72305760742956,
-0.311755813135147));
#40765=CARTESIAN_POINT('Ctrl Pts',(-67.7605877414888,-5.7573141761971,-3.48568913462309));
#40766=CARTESIAN_POINT('Ctrl Pts',(-67.6614999562719,-3.39261751877765,
-5.81264503395175));
#40767=CARTESIAN_POINT('Ctrl Pts',(-67.5624121710554,-0.203558611737488,
-6.72720280201832));
#40768=CARTESIAN_POINT('Ctrl Pts',(-67.4633243858386,3.03496262220109,-6.00713749956949));
#40769=CARTESIAN_POINT('Ctrl Pts',(-67.3642366006221,5.53602661805977,-3.82741406304774));
#40770=CARTESIAN_POINT('Ctrl Pts',(-67.2651488154053,6.69190831335928,-0.717680564662976));
#40771=CARTESIAN_POINT('Ctrl Pts',(-67.1660610301887,6.22174077474846,2.56644462504013));
#40772=CARTESIAN_POINT('Ctrl Pts',(-67.066973244972,4.23977387275612,5.22694758728607));
#40773=CARTESIAN_POINT('Ctrl Pts',(-66.9678854597554,1.22758945576965,6.61738837079199));
#40774=CARTESIAN_POINT('Ctrl Pts',(-66.8687976745386,-2.08286902182032,
6.39985101098365));
#40775=CARTESIAN_POINT('Ctrl Pts',(-66.769709889322,-4.88724628381849,4.62730939927117));
#40776=CARTESIAN_POINT('Ctrl Pts',(-66.6706221041053,-6.50402659951364,
1.73023480709699));
#40777=CARTESIAN_POINT('Ctrl Pts',(-66.5715343188887,-6.54053194085659,
-1.58694591594768));
#40778=CARTESIAN_POINT('Ctrl Pts',(-66.4724465336719,-4.98752773549323,
-4.5191773691222));
#40779=CARTESIAN_POINT('Ctrl Pts',(-66.4063880101942,-3.1445555439941,-5.74073515448772));
#40780=CARTESIAN_POINT('Ctrl Pts',(-66.3733587484553,-2.13267601915869,
-6.0948088040903));
#40781=CARTESIAN_POINT('Ctrl Pts',(-86.6480812515447,-4.48284371989911,
4.97275105180613));
#40782=CARTESIAN_POINT('Ctrl Pts',(-86.6150519898058,-5.30843565119142,
4.22849509251194));
#40783=CARTESIAN_POINT('Ctrl Pts',(-86.5489934663281,-6.58091053988509,
2.32154726689182));
#40784=CARTESIAN_POINT('Ctrl Pts',(-86.4499056811113,-6.89025871712545,
-1.10487568155517));
#40785=CARTESIAN_POINT('Ctrl Pts',(-86.3508178958947,-5.52539282950227,
-4.26210071613823));
#40786=CARTESIAN_POINT('Ctrl Pts',(-86.251730110678,-2.81791437092512,-6.38404285368998));
#40787=CARTESIAN_POINT('Ctrl Pts',(-86.1526423254614,0.574274741333435,
-6.9545715857264));
#40788=CARTESIAN_POINT('Ctrl Pts',(-86.0535545402446,3.8269255521002,-5.83531441164414));
#40789=CARTESIAN_POINT('Ctrl Pts',(-85.9544667550281,6.14968124512553,-3.2981088982798));
#40790=CARTESIAN_POINT('Ctrl Pts',(-85.8553789698113,6.97814436331505,0.0404738222987098));
#40791=CARTESIAN_POINT('Ctrl Pts',(-85.7562911845946,6.11100793051157,3.36923216679088));
#40792=CARTESIAN_POINT('Ctrl Pts',(-85.657203399378,3.75897547692409,5.87930544849775));
#40793=CARTESIAN_POINT('Ctrl Pts',(-85.5581156141613,0.49356031837395,6.96078573734991));
#40794=CARTESIAN_POINT('Ctrl Pts',(-85.4590278289446,-2.8917835952124,6.35088353638262));
#40795=CARTESIAN_POINT('Ctrl Pts',(-85.359940043728,-5.5744613704079,4.19779905737357));
#40796=CARTESIAN_POINT('Ctrl Pts',(-85.2608522585113,-6.90261683515409,
1.02470318704625));
#40797=CARTESIAN_POINT('Ctrl Pts',(-85.1617644732947,-6.55352533752688,
-2.39738220962939));
#40798=CARTESIAN_POINT('Ctrl Pts',(-85.0626766880779,-4.61201160637967,
-5.23693468640519));
#40799=CARTESIAN_POINT('Ctrl Pts',(-84.9635889028613,-1.54983847062524,
-6.80397946361766));
#40800=CARTESIAN_POINT('Ctrl Pts',(-84.8645011176447,1.88892544825633,-6.71774490142901));
#40801=CARTESIAN_POINT('Ctrl Pts',(-84.7654133324279,4.86870481707144,-4.99918486114854));
#40802=CARTESIAN_POINT('Ctrl Pts',(-84.6663255472113,6.6654516368139,-2.06588730614305));
#40803=CARTESIAN_POINT('Ctrl Pts',(-84.5672377619945,6.84257957673285,1.36939425248265));
#40804=CARTESIAN_POINT('Ctrl Pts',(-84.4681499767779,5.3570488294005,4.47193064799671));
#40805=CARTESIAN_POINT('Ctrl Pts',(-84.3690621915613,2.56982422894208,6.48784550642254));
#40806=CARTESIAN_POINT('Ctrl Pts',(-84.2699744063446,-0.841834553257127,
6.92729748651229));
#40807=CARTESIAN_POINT('Ctrl Pts',(-84.1708866211279,-4.04893838399307,
5.68350541874474));
#40808=CARTESIAN_POINT('Ctrl Pts',(-84.0717988359113,-6.27220234805808,
3.05869475218969));
#40809=CARTESIAN_POINT('Ctrl Pts',(-83.9727110506946,-6.97140194349158,
-0.309339335336139));
#40810=CARTESIAN_POINT('Ctrl Pts',(-83.8736232654778,-5.9766406760737,-3.60220794946903));
#40811=CARTESIAN_POINT('Ctrl Pts',(-83.7745354802614,-3.52963271872836,
-6.01978643748904));
#40812=CARTESIAN_POINT('Ctrl Pts',(-83.6754476950444,-0.224969481393537,
-6.97463437138838));
#40813=CARTESIAN_POINT('Ctrl Pts',(-83.576359909828,3.1343584417398,-6.23473600409806));
#40814=CARTESIAN_POINT('Ctrl Pts',(-83.4772721246112,5.73207764205231,-3.97987710709635));
#40815=CARTESIAN_POINT('Ctrl Pts',(-83.3781843393946,6.93697581910938,-0.757959344026197));
#40816=CARTESIAN_POINT('Ctrl Pts',(-83.2790965541779,6.45627823804426,2.64813277519475));
#40817=CARTESIAN_POINT('Ctrl Pts',(-83.1800087689611,4.40678821844635,5.4107627447401));
#40818=CARTESIAN_POINT('Ctrl Pts',(-83.0809209837446,1.28650543242509,6.85864707172234));
#40819=CARTESIAN_POINT('Ctrl Pts',(-82.9818331985278,-2.14638160020794,
6.63996851712368));
#40820=CARTESIAN_POINT('Ctrl Pts',(-82.8827454133112,-5.05772555485365,
4.80786315257465));
#40821=CARTESIAN_POINT('Ctrl Pts',(-82.7836576280946,-6.7401073560603,1.80750897947607));
#40822=CARTESIAN_POINT('Ctrl Pts',(-82.6845698428778,-6.78472989949836,
-1.63204659031467));
#40823=CARTESIAN_POINT('Ctrl Pts',(-82.5854820576613,-5.18075048196443,
-4.67503586357689));
#40824=CARTESIAN_POINT('Ctrl Pts',(-82.4863942724445,-2.317915438578,-6.58205164836212));
#40825=CARTESIAN_POINT('Ctrl Pts',(-82.3873064872279,1.10814319572684,-6.88971367618925));
#40826=CARTESIAN_POINT('Ctrl Pts',(-82.2882187020112,4.26493730917755,-5.52326403776699));
#40827=CARTESIAN_POINT('Ctrl Pts',(-82.1891309167945,6.38540659975617,-2.81473239187942));
#40828=CARTESIAN_POINT('Ctrl Pts',(-82.0900431315779,6.9543043468987,0.577742964310748));
#40829=CARTESIAN_POINT('Ctrl Pts',(-81.9909553463612,5.83339572690187,3.82983422297465));
#40830=CARTESIAN_POINT('Ctrl Pts',(-81.8918675611445,3.29504709426618,6.15132510347753));
#40831=CARTESIAN_POINT('Ctrl Pts',(-81.7927797759278,-0.0439555336750358,
6.97812322857401));
#40832=CARTESIAN_POINT('Ctrl Pts',(-81.6936919907111,-3.37227753319247,
6.10932730513189));
#40833=CARTESIAN_POINT('Ctrl Pts',(-81.5946042054945,-5.88117953567009,
3.75604355024275));
#40834=CARTESIAN_POINT('Ctrl Pts',(-81.4955164202778,-6.9610306755554,0.490089600054565));
#40835=CARTESIAN_POINT('Ctrl Pts',(-81.3964286350611,-6.34944103708999,
-2.89494980934425));
#40836=CARTESIAN_POINT('Ctrl Pts',(-81.2973408498445,-4.19501902358835,
-5.57655370940124));
#40837=CARTESIAN_POINT('Ctrl Pts',(-81.1982530646278,-1.02126142988711,
-6.90312689829252));
#40838=CARTESIAN_POINT('Ctrl Pts',(-81.0991652794112,2.40064953482766,-6.55232918075981));
#40839=CARTESIAN_POINT('Ctrl Pts',(-81.0000774941945,5.2392335890613,-4.60939988299525));
#40840=CARTESIAN_POINT('Ctrl Pts',(-80.9009897089778,6.80475137582932,-1.54644579447639));
#40841=CARTESIAN_POINT('Ctrl Pts',(-80.8019019237612,6.71680224080455,1.89227469993862));
#40842=CARTESIAN_POINT('Ctrl Pts',(-80.7028141385443,4.99675669078907,4.8711968195875));
#40843=CARTESIAN_POINT('Ctrl Pts',(-80.603726353328,2.06256363586796,6.66648086550168));
#40844=CARTESIAN_POINT('Ctrl Pts',(-80.504638568111,-1.37280581149482,6.84189594235625));
#40845=CARTESIAN_POINT('Ctrl Pts',(-80.4055507828946,-4.4746011319006,5.35481844626862));
#40846=CARTESIAN_POINT('Ctrl Pts',(-80.3064629976777,-6.48912602151675,
2.56658905144142));
#40847=CARTESIAN_POINT('Ctrl Pts',(-80.2073752124612,-6.9268768843794,-0.845288418680318));
#40848=CARTESIAN_POINT('Ctrl Pts',(-80.1082874272444,-5.68148590015928,
-4.05177169253108));
#40849=CARTESIAN_POINT('Ctrl Pts',(-80.0091996420278,-3.05556703421317,
-6.27372664223861));
#40850=CARTESIAN_POINT('Ctrl Pts',(-79.910111856811,0.312815257558859,-6.97124683946445));
#40851=CARTESIAN_POINT('Ctrl Pts',(-79.8110240715945,3.60518747160154,-5.97484386211992));
#40852=CARTESIAN_POINT('Ctrl Pts',(-79.7119362863777,6.02154557404439,-3.52663079749089));
#40853=CARTESIAN_POINT('Ctrl Pts',(-79.6128485011612,6.97474567484213,-0.221491881060804));
#40854=CARTESIAN_POINT('Ctrl Pts',(-79.5137607159443,6.2331724291466,3.13746670908733));
#40855=CARTESIAN_POINT('Ctrl Pts',(-79.4146729307278,3.97701858230921,5.73406130749159));
#40856=CARTESIAN_POINT('Ctrl Pts',(-79.315585145511,0.754500454101965,6.93735287749331));
#40857=CARTESIAN_POINT('Ctrl Pts',(-79.2164973602945,-2.651351564564,6.45495706904306));
#40858=CARTESIAN_POINT('Ctrl Pts',(-79.1174095750777,-5.41295930920374,
4.40408984910723));
#40859=CARTESIAN_POINT('Ctrl Pts',(-79.0183217898611,-6.85928767441309,
1.28308553173565));
#40860=CARTESIAN_POINT('Ctrl Pts',(-78.9192340046443,-6.63889749984028,
-2.14969204043726));
#40861=CARTESIAN_POINT('Ctrl Pts',(-78.8201462194278,-4.80534075871954,
-5.060122140294));
#40862=CARTESIAN_POINT('Ctrl Pts',(-78.721058434211,-1.80414811826117,-6.74100774732379));
#40863=CARTESIAN_POINT('Ctrl Pts',(-78.6219706489944,1.63542927291058,-6.78391531310733));
#40864=CARTESIAN_POINT('Ctrl Pts',(-78.5228828637777,4.67761841926058,-5.17841885191792));
#40865=CARTESIAN_POINT('Ctrl Pts',(-78.4237950785611,6.58320654937237,-2.31463332093999));
#40866=CARTESIAN_POINT('Ctrl Pts',(-78.3247072933443,6.88916029645859,1.11157828865235));
#40867=CARTESIAN_POINT('Ctrl Pts',(-78.2256195081277,5.52113684144108,4.2676906940624));
#40868=CARTESIAN_POINT('Ctrl Pts',(-78.126531722911,2.81154826026171,6.38680923954397));
#40869=CARTESIAN_POINT('Ctrl Pts',(-78.0274439376944,-0.581210328256866,
6.95401541819058));
#40870=CARTESIAN_POINT('Ctrl Pts',(-77.9283561524777,-3.83274229447874,
5.83148543565175));
#40871=CARTESIAN_POINT('Ctrl Pts',(-77.8292683672611,-6.15296725862748,
3.29197961663846));
#40872=CARTESIAN_POINT('Ctrl Pts',(-77.7301805820443,-6.97810044482352,
-0.0474348401337781));
#40873=CARTESIAN_POINT('Ctrl Pts',(-77.6310927968278,-6.10764511863883,
-3.3753232418351));
#40874=CARTESIAN_POINT('Ctrl Pts',(-77.532005011611,-3.75311071065405,-5.88305157853291));
#40875=CARTESIAN_POINT('Ctrl Pts',(-77.4329172263944,-0.48661874960787,
-6.96127417033943));
#40876=CARTESIAN_POINT('Ctrl Pts',(-77.3338294411776,2.89811529870384,-6.34799681769954));
#40877=CARTESIAN_POINT('Ctrl Pts',(-77.2347416559611,5.57864466453888,-4.19223801673006));
#40878=CARTESIAN_POINT('Ctrl Pts',(-77.1356538707443,6.90363524404658,-1.0178193844011));
#40879=CARTESIAN_POINT('Ctrl Pts',(-77.0365660855277,6.55113139566086,2.40391624623061));
#40880=CARTESIAN_POINT('Ctrl Pts',(-76.937478300311,4.60678701339179,5.24153119759385));
#40881=CARTESIAN_POINT('Ctrl Pts',(-76.8383905150943,1.54305273402164,6.8055215922171));
#40882=CARTESIAN_POINT('Ctrl Pts',(-76.7393027298776,-1.89562348126539,
6.71585791238766));
#40883=CARTESIAN_POINT('Ctrl Pts',(-76.640214944661,-4.87368761106475,4.9943272772075));
#40884=CARTESIAN_POINT('Ctrl Pts',(-76.5411271594443,-6.66750843688816,
2.05923945332494));
#40885=CARTESIAN_POINT('Ctrl Pts',(-76.4420393742277,-6.84121060704279,
-1.37621702946524));
#40886=CARTESIAN_POINT('Ctrl Pts',(-76.3429515890109,-5.35258673190751,
-4.47727050327678));
#40887=CARTESIAN_POINT('Ctrl Pts',(-76.2438638037943,-2.56335323587229,
-6.4904049234426));
#40888=CARTESIAN_POINT('Ctrl Pts',(-76.1447760185776,0.848742073959769,
-6.92645456016245));
#40889=CARTESIAN_POINT('Ctrl Pts',(-76.0456882333609,4.05460399377978,-5.67946496914364));
#40890=CARTESIAN_POINT('Ctrl Pts',(-75.9466004481443,6.27524937674041,-3.05243855660093));
#40891=CARTESIAN_POINT('Ctrl Pts',(-75.8475126629276,6.97109000235212,0.316291102010706));
#40892=CARTESIAN_POINT('Ctrl Pts',(-75.7484248777109,5.97304556279128,3.60816609746892));
#40893=CARTESIAN_POINT('Ctrl Pts',(-75.6493370924943,3.52362799951616,6.02330321361383));
#40894=CARTESIAN_POINT('Ctrl Pts',(-75.5502493072776,0.218014225664164,
6.97485524434111));
#40895=CARTESIAN_POINT('Ctrl Pts',(-75.4511615220609,-3.14057419644558,
6.23160730459846));
#40896=CARTESIAN_POINT('Ctrl Pts',(-75.3520737368443,-5.73604354741575,
3.97415906881632));
#40897=CARTESIAN_POINT('Ctrl Pts',(-75.2529859516275,-6.93772821121811,
0.751041376605294));
#40898=CARTESIAN_POINT('Ctrl Pts',(-75.153898166411,-6.45363429530861,-2.65456969479452));
#40899=CARTESIAN_POINT('Ctrl Pts',(-75.0548103811942,-4.40139038489031,
-5.41515452797977));
#40900=CARTESIAN_POINT('Ctrl Pts',(-74.9557225959776,-1.27966531206499,
-6.85992657185209));
#40901=CARTESIAN_POINT('Ctrl Pts',(-74.8566348107609,2.15300194624281,-6.63782483209519));
#40902=CARTESIAN_POINT('Ctrl Pts',(-74.7575470255443,5.06251746776372,-4.80281717023373));
#40903=CARTESIAN_POINT('Ctrl Pts',(-74.6584592403275,6.74190646274048,-1.80078680852646));
#40904=CARTESIAN_POINT('Ctrl Pts',(-74.5593714551109,6.78309904020246,1.63881154893091));
#40905=CARTESIAN_POINT('Ctrl Pts',(-74.4602836698942,5.17608593449171,4.68019981206593));
#40906=CARTESIAN_POINT('Ctrl Pts',(-74.3611958846776,2.31135062787306,6.58435981376593));
#40907=CARTESIAN_POINT('Ctrl Pts',(-74.2621080994609,-1.11501310523416,
6.88860520404971));
#40908=CARTESIAN_POINT('Ctrl Pts',(-74.1630203142442,-4.27044301797891,
5.5190082725341));
#40909=CARTESIAN_POINT('Ctrl Pts',(-74.0639325290276,-6.3882102915404,2.80836342967968));
#40910=CARTESIAN_POINT('Ctrl Pts',(-73.9648447438108,-6.95372476068093,
-0.584677547711268));
#40911=CARTESIAN_POINT('Ctrl Pts',(-73.8657569585942,-5.82957369466647,
-3.83564941314472));
#40912=CARTESIAN_POINT('Ctrl Pts',(-73.7666691733775,-3.28891132060887,
-6.15460788412029));
#40913=CARTESIAN_POINT('Ctrl Pts',(-73.6675813881609,0.0509141347999404,
-6.97807592628386));
#40914=CARTESIAN_POINT('Ctrl Pts',(-73.5684936029441,3.37836811135612,-6.10596141375596));
#40915=CARTESIAN_POINT('Ctrl Pts',(-73.4694058177276,5.88492215884091,-3.75017693802415));
#40916=CARTESIAN_POINT('Ctrl Pts',(-73.3703180325108,6.96151593451736,-0.483147778185493));
#40917=CARTESIAN_POINT('Ctrl Pts',(-73.2712302472942,6.34655102016675,2.90128006757796));
#40918=CARTESIAN_POINT('Ctrl Pts',(-73.1721424620775,4.18945596766144,5.58073423279865));
#40919=CARTESIAN_POINT('Ctrl Pts',(-73.0730546768608,1.01437708588044,6.90414187352386));
#40920=CARTESIAN_POINT('Ctrl Pts',(-72.9739668916443,-2.4071823600084,6.5499319819193));
#40921=CARTESIAN_POINT('Ctrl Pts',(-72.8748791064274,-5.24382750305657,
4.60417299851909));
#40922=CARTESIAN_POINT('Ctrl Pts',(-72.7757913212108,-6.80629011671958,
1.53965928995673));
#40923=CARTESIAN_POINT('Ctrl Pts',(-72.6767035359942,-6.7149119143764,-1.89897179133098));
#40924=CARTESIAN_POINT('Ctrl Pts',(-72.5776157507775,-4.99189662201232,
-4.87617719091982));
#40925=CARTESIAN_POINT('Ctrl Pts',(-72.4785279655608,-2.05591475884529,
-6.66853435070007));
#40926=CARTESIAN_POINT('Ctrl Pts',(-72.3794401803442,1.37962790530135,-6.84052357097165));
#40927=CARTESIAN_POINT('Ctrl Pts',(-72.2803523951275,4.47993876158198,-5.35035368686783));
#40928=CARTESIAN_POINT('Ctrl Pts',(-72.1812646099109,6.49168221182268,-2.56011678304133));
#40929=CARTESIAN_POINT('Ctrl Pts',(-72.0821768246941,6.92603051399574,0.852195518237787));
#40930=CARTESIAN_POINT('Ctrl Pts',(-71.9830890394775,5.67744262618587,4.05743528703446));
#40931=CARTESIAN_POINT('Ctrl Pts',(-71.8840012542608,3.0493093201379,6.27677055118515));
#40932=CARTESIAN_POINT('Ctrl Pts',(-71.7849134690441,-0.319766867831018,
6.97093143219341));
#40933=CARTESIAN_POINT('Ctrl Pts',(-71.6858256838275,-3.6111438263289,5.97124577853496));
#40934=CARTESIAN_POINT('Ctrl Pts',(-71.5867378986107,-6.02505935576122,
3.52062432555065));
#40935=CARTESIAN_POINT('Ctrl Pts',(-71.4876501133942,-6.97496307985772,
0.214536516068103));
#40936=CARTESIAN_POINT('Ctrl Pts',(-71.3885623281774,-6.23004063084288,
-3.14368090304213));
#40937=CARTESIAN_POINT('Ctrl Pts',(-71.2894745429608,-3.9712985673284,-5.73802436133205));
#40938=CARTESIAN_POINT('Ctrl Pts',(-71.190386757744,-0.747582112396103,
-6.93810182019046));
#40939=CARTESIAN_POINT('Ctrl Pts',(-71.0912989725275,2.65778716508629,-6.45230991716978));
#40940=CARTESIAN_POINT('Ctrl Pts',(-70.9922111873108,5.41734840052245,-4.39868982646668));
#40941=CARTESIAN_POINT('Ctrl Pts',(-70.8931234020941,6.8605637638805,-1.27624477426342));
#40942=CARTESIAN_POINT('Ctrl Pts',(-70.7940356168774,6.63675051415506,2.15631131680177));
#40943=CARTESIAN_POINT('Ctrl Pts',(-70.6949478316608,4.80029238774456,5.0649115366674));
#40944=CARTESIAN_POINT('Ctrl Pts',(-70.5958600464441,1.79742505110744,6.74280350208697));
#40945=CARTESIAN_POINT('Ctrl Pts',(-70.4967722612274,-1.64219341753491,
6.78228108098667));
#40946=CARTESIAN_POINT('Ctrl Pts',(-70.3976844760107,-4.6827800413512,5.17375173026572));
#40947=CARTESIAN_POINT('Ctrl Pts',(-70.2985966907941,-6.58551144125611,
2.30806736019331));
#40948=CARTESIAN_POINT('Ctrl Pts',(-70.1995089055774,-6.8880483991006,-1.11844764461836));
#40949=CARTESIAN_POINT('Ctrl Pts',(-70.1004211203607,-5.51687833157526,
-4.27319428024283));
#40950=CARTESIAN_POINT('Ctrl Pts',(-70.001333335144,-2.80517790092504,-6.38960975539716));
#40951=CARTESIAN_POINT('Ctrl Pts',(-69.9022455499274,0.588144621812076,
-6.95343237444202));
#40952=CARTESIAN_POINT('Ctrl Pts',(-69.8031577647108,3.83855557824996,-5.82766050442122));
#40953=CARTESIAN_POINT('Ctrl Pts',(-69.704069979494,6.15624697954815,-3.28584220694011));
#40954=CARTESIAN_POINT('Ctrl Pts',(-69.6049821942774,6.97804967296109,0.0543934168086905));
#40955=CARTESIAN_POINT('Ctrl Pts',(-69.5058944090607,6.10427619090187,3.38141214099867));
#40956=CARTESIAN_POINT('Ctrl Pts',(-69.406806623844,3.74724223308222,5.88679127612919));
#40957=CARTESIAN_POINT('Ctrl Pts',(-69.3077188386274,0.479676686650263,
6.96175596802892));
#40958=CARTESIAN_POINT('Ctrl Pts',(-69.2086310534108,-2.90444411518026,
6.34510364485133));
#40959=CARTESIAN_POINT('Ctrl Pts',(-69.109543268194,-5.58282241366096,4.18667287707308));
#40960=CARTESIAN_POINT('Ctrl Pts',(-69.0104554829774,-6.90464678659901,
1.01093453518231));
#40961=CARTESIAN_POINT('Ctrl Pts',(-68.9113676977607,-6.54873093983205,
-2.41044787535243));
#40962=CARTESIAN_POINT('Ctrl Pts',(-68.812279912544,-4.60155783902944,-5.24612250487201));
#40963=CARTESIAN_POINT('Ctrl Pts',(-68.7131921273274,-1.53626546311999,
-6.8070569491593));
#40964=CARTESIAN_POINT('Ctrl Pts',(-68.6141043421107,1.90231962929278,-6.71396424697843));
#40965=CARTESIAN_POINT('Ctrl Pts',(-68.515016556894,4.87866555855498,-4.98946472586331));
#40966=CARTESIAN_POINT('Ctrl Pts',(-68.4159287716774,6.66955860663988,-2.05258955314249));
#40967=CARTESIAN_POINT('Ctrl Pts',(-68.3168409864607,6.83983483439994,1.38303843792684));
#40968=CARTESIAN_POINT('Ctrl Pts',(-68.2177532012439,5.34811931152934,4.4826059066167));
#40969=CARTESIAN_POINT('Ctrl Pts',(-68.1186654160274,2.55687969410828,6.49295788539925));
#40970=CARTESIAN_POINT('Ctrl Pts',(-68.0195776308106,-0.85564875137622,
6.92560474789127));
#40971=CARTESIAN_POINT('Ctrl Pts',(-67.920489845594,-4.06026557013075,5.67541886792257));
#40972=CARTESIAN_POINT('Ctrl Pts',(-67.8214020603773,-6.27829016815635,
3.04617933344148));
#40973=CARTESIAN_POINT('Ctrl Pts',(-67.7223142751607,-6.9707711230222,-0.323242570052509));
#40974=CARTESIAN_POINT('Ctrl Pts',(-67.623226489944,-5.96944452197626,-3.61412062520652));
#40975=CARTESIAN_POINT('Ctrl Pts',(-67.5241387047273,-3.51761975164696,
-6.02681406541461));
#40976=CARTESIAN_POINT('Ctrl Pts',(-67.4250509195106,-0.211058803210948,
-6.97506904882113));
#40977=CARTESIAN_POINT('Ctrl Pts',(-67.325963134294,3.1467869296422,-6.22847267703732));
#40978=CARTESIAN_POINT('Ctrl Pts',(-67.2268753490773,5.7400035428534,-3.96843653355858));
#40979=CARTESIAN_POINT('Ctrl Pts',(-67.1277875638606,6.93847412182326,-0.744123767462383));
#40980=CARTESIAN_POINT('Ctrl Pts',(-67.0286997786439,6.45098308835231,2.66100621557892));
#40981=CARTESIAN_POINT('Ctrl Pts',(-66.9296119934273,4.39598989122037,5.41953638218708));
#40982=CARTESIAN_POINT('Ctrl Pts',(-66.8305242082107,1.27282043809193,6.86120846472652));
#40983=CARTESIAN_POINT('Ctrl Pts',(-66.7314364229939,-2.15961309245625,
6.63565586136125));
#40984=CARTESIAN_POINT('Ctrl Pts',(-66.6323486377773,-5.06731865999354,
4.79780430589844));
#40985=CARTESIAN_POINT('Ctrl Pts',(-66.5332608525606,-6.74366983753873,
1.79398594116332));
#40986=CARTESIAN_POINT('Ctrl Pts',(-66.4341730673439,-6.78152023153034,
-1.64541751843109));
#40987=CARTESIAN_POINT('Ctrl Pts',(-66.3350852821273,-5.17129501841962,
-4.68568811156397));
#40988=CARTESIAN_POINT('Ctrl Pts',(-66.2690267586495,-3.26041784270748,
-5.95225464015044));
#40989=CARTESIAN_POINT('Ctrl Pts',(-66.2359974969106,-2.21125524682175,
-6.31937426282706));
#40990=CARTESIAN_POINT('Ctrl Pts',(-86.51072,-4.64214617842353,5.14946287083884));
#40991=CARTESIAN_POINT('Ctrl Pts',(-86.4776907382611,-5.49707636744029,
4.37875901117269));
#40992=CARTESIAN_POINT('Ctrl Pts',(-86.4116322147833,-6.81476995900323,
2.40404583483319));
#40993=CARTESIAN_POINT('Ctrl Pts',(-86.3125444295667,-7.1351111416334,-1.14413857436007));
#40994=CARTESIAN_POINT('Ctrl Pts',(-86.2134566443499,-5.72174334204543,
-4.41355884517039));
#40995=CARTESIAN_POINT('Ctrl Pts',(-86.1143688591333,-2.91805185401586,
-6.61090637726181));
#40996=CARTESIAN_POINT('Ctrl Pts',(-86.0152810739167,0.594682184438515,
-7.20170943411326));
#40997=CARTESIAN_POINT('Ctrl Pts',(-85.9161932886999,3.96291928445659,-6.04267830610954));
#40998=CARTESIAN_POINT('Ctrl Pts',(-85.8171055034833,6.36821648808781,-3.41531058738736));
#40999=CARTESIAN_POINT('Ctrl Pts',(-85.7180177182667,7.22611989457885,0.0419121011682899));
#41000=CARTESIAN_POINT('Ctrl Pts',(-85.6189299330499,6.32816887749518,3.48896129433705));
#41001=CARTESIAN_POINT('Ctrl Pts',(-85.5198421478333,3.89255453352808,6.08823260966652));
#41002=CARTESIAN_POINT('Ctrl Pts',(-85.4207543626166,0.511099491510444,
7.20814441200088));
#41003=CARTESIAN_POINT('Ctrl Pts',(-85.3216665774,-2.99454609710222,6.57656870953671));
#41004=CARTESIAN_POINT('Ctrl Pts',(-85.2225787921833,-5.77255558397897,
4.34697216087991));
#41005=CARTESIAN_POINT('Ctrl Pts',(-85.1234910069666,-7.14790841808639,
1.06111706786699));
#41006=CARTESIAN_POINT('Ctrl Pts',(-85.02440322175,-6.78641159533597,-2.4825756501951));
#41007=CARTESIAN_POINT('Ctrl Pts',(-84.9253154365331,-4.77590417849372,
-5.42303454239013));
#41008=CARTESIAN_POINT('Ctrl Pts',(-84.8262276513167,-1.60491357342004,
-7.04576586618457));
#41009=CARTESIAN_POINT('Ctrl Pts',(-84.7271398660999,1.95605035527479,-6.95646687020684));
#41010=CARTESIAN_POINT('Ctrl Pts',(-84.6280520808833,5.04171924622639,-5.1768360327618));
#41011=CARTESIAN_POINT('Ctrl Pts',(-84.5289642956666,6.90231531069278,-2.13930073464208));
#41012=CARTESIAN_POINT('Ctrl Pts',(-84.4298765104498,7.08573767398796,1.41805708454642));
#41013=CARTESIAN_POINT('Ctrl Pts',(-84.3307887252333,5.54741706489595,4.63084529929592));
#41014=CARTESIAN_POINT('Ctrl Pts',(-84.2317009400165,2.66114557387967,6.71839776393533));
#41015=CARTESIAN_POINT('Ctrl Pts',(-84.1326131547999,-0.871750009245318,
7.17346612175447));
#41016=CARTESIAN_POINT('Ctrl Pts',(-84.0335253695832,-4.19282157048937,
5.88547462463609));
#41017=CARTESIAN_POINT('Ctrl Pts',(-83.9344375843665,-6.4950915043258,3.16738861357433));
#41018=CARTESIAN_POINT('Ctrl Pts',(-83.8353497991499,-7.21913787593788,
-0.320332026519753));
#41019=CARTESIAN_POINT('Ctrl Pts',(-83.7362620139332,-6.18902674458406,
-3.73021611087769));
#41020=CARTESIAN_POINT('Ctrl Pts',(-83.6371742287166,-3.65506184472842,
-6.2337057349714));
#41021=CARTESIAN_POINT('Ctrl Pts',(-83.5380864434999,-0.232964003111965,
-7.2224851714819));
#41022=CARTESIAN_POINT('Ctrl Pts',(-83.4389986582832,3.24574109009077,-6.4562937553297));
#41023=CARTESIAN_POINT('Ctrl Pts',(-83.3399108730665,5.93577291181568,-4.12130613014512));
#41024=CARTESIAN_POINT('Ctrl Pts',(-83.2408230878499,7.18348838384663,-0.784894208257366));
#41025=CARTESIAN_POINT('Ctrl Pts',(-83.1417353026331,6.68570872023415,2.74223689479967));
#41026=CARTESIAN_POINT('Ctrl Pts',(-83.0426475174165,4.56338796656581,5.60303975941794));
#41027=CARTESIAN_POINT('Ctrl Pts',(-82.9435597321999,1.33222272508483,7.10237614392416));
#41028=CARTESIAN_POINT('Ctrl Pts',(-82.8444719469831,-2.22265547616906,
6.87592662215584));
#41029=CARTESIAN_POINT('Ctrl Pts',(-82.7453841617666,-5.2374570301789,4.97871551065585));
#41030=CARTESIAN_POINT('Ctrl Pts',(-82.6462963765498,-6.97962399764495,
1.87174066860623));
#41031=CARTESIAN_POINT('Ctrl Pts',(-82.5472085913332,-7.02583224902186,
-1.6900430431264));
#41032=CARTESIAN_POINT('Ctrl Pts',(-82.4481208061165,-5.3648537745051,-4.84116806743931));
#41033=CARTESIAN_POINT('Ctrl Pts',(-82.3490330208998,-2.40028494576787,
-6.8159516179427));
#41034=CARTESIAN_POINT('Ctrl Pts',(-82.2499452356832,1.14752220300579,-7.13454673210741));
#41035=CARTESIAN_POINT('Ctrl Pts',(-82.1508574504664,4.41649623945849,-5.71953890150811));
#41036=CARTESIAN_POINT('Ctrl Pts',(-82.0517696652499,6.61231858544595,-2.91475680007471));
#41037=CARTESIAN_POINT('Ctrl Pts',(-81.9526818800332,7.20143269867919,0.598273654283556));
#41038=CARTESIAN_POINT('Ctrl Pts',(-81.8535940948164,6.04069143893316,3.96593131793975));
#41039=CARTESIAN_POINT('Ctrl Pts',(-81.7545063095999,3.41213997902156,6.36991876263571));
#41040=CARTESIAN_POINT('Ctrl Pts',(-81.655418524383,-0.0455175387364694,
7.22609800879306));
#41041=CARTESIAN_POINT('Ctrl Pts',(-81.5563307391665,-3.49211488096338,
6.3264285293655));
#41042=CARTESIAN_POINT('Ctrl Pts',(-81.4572429539498,-6.09017329445249,
3.88951841781901));
#41043=CARTESIAN_POINT('Ctrl Pts',(-81.3581551687331,-7.20839805433722,
0.507505437648791));
#41044=CARTESIAN_POINT('Ctrl Pts',(-81.2590673835164,-6.57507494954929,
-2.9978248259071));
#41045=CARTESIAN_POINT('Ctrl Pts',(-81.1599795982998,-4.34409333573713,
-5.7747222763887));
#41046=CARTESIAN_POINT('Ctrl Pts',(-81.0608918130831,-1.05755300433017,
-7.14843660684264));
#41047=CARTESIAN_POINT('Ctrl Pts',(-80.9618040278664,2.48595908315207,-6.78517293190891));
#41048=CARTESIAN_POINT('Ctrl Pts',(-80.8627162426498,5.42541513891466,-4.77319964483483));
#41049=CARTESIAN_POINT('Ctrl Pts',(-80.7636284574331,7.04656520908996,-1.60140033503765));
#41050=CARTESIAN_POINT('Ctrl Pts',(-80.6645406722165,6.95549071116834,1.95951862605758));
#41051=CARTESIAN_POINT('Ctrl Pts',(-80.5654528869997,5.17432157487322,5.04429980461283));
#41052=CARTESIAN_POINT('Ctrl Pts',(-80.4663651017832,2.13585895432808,6.9033811140797));
#41053=CARTESIAN_POINT('Ctrl Pts',(-80.3672773165663,-1.42158987681409,
7.08502974596122));
#41054=CARTESIAN_POINT('Ctrl Pts',(-80.2681895313499,-4.63361068158974,
5.54510742280736));
#41055=CARTESIAN_POINT('Ctrl Pts',(-80.1691017461329,-6.71972378344938,
2.65779543102179));
#41056=CARTESIAN_POINT('Ctrl Pts',(-80.0700139609165,-7.17303057309256,
-0.875326611325795));
#41057=CARTESIAN_POINT('Ctrl Pts',(-79.9709261756997,-5.88338334038227,
-4.19575556355802));
#41058=CARTESIAN_POINT('Ctrl Pts',(-79.8718383904831,-3.16414974892521,
-6.49666996586653));
#41059=CARTESIAN_POINT('Ctrl Pts',(-79.7727506052664,0.323931469210802,
-7.21897726012976));
#41060=CARTESIAN_POINT('Ctrl Pts',(-79.6736628200498,3.73330151339117,-6.18716607899989));
#41061=CARTESIAN_POINT('Ctrl Pts',(-79.574575034833,6.23552738425208,-3.65195324713476));
#41062=CARTESIAN_POINT('Ctrl Pts',(-79.4754872496165,7.22260043021827,-0.22936282267754));
#41063=CARTESIAN_POINT('Ctrl Pts',(-79.3763994643997,6.45467461713548,3.24895981291281));
#41064=CARTESIAN_POINT('Ctrl Pts',(-79.2773116791831,4.11834602474202,5.93782706884491));
#41065=CARTESIAN_POINT('Ctrl Pts',(-79.1782238939663,0.781312403125045,
7.18387884138775));
#41066=CARTESIAN_POINT('Ctrl Pts',(-79.0791361087498,-2.74557006715706,
6.68434060213473));
#41067=CARTESIAN_POINT('Ctrl Pts',(-78.980048323533,-5.60531438105715,4.56059370789917));
#41068=CARTESIAN_POINT('Ctrl Pts',(-78.8809605383164,-7.10303951108988,
1.32868129470981));
#41069=CARTESIAN_POINT('Ctrl Pts',(-78.7818727530996,-6.87481754517261,
-2.226083556294));
#41070=CARTESIAN_POINT('Ctrl Pts',(-78.6827849678831,-4.97610348094288,
-5.2399387807458));
#41071=CARTESIAN_POINT('Ctrl Pts',(-78.5836971826663,-1.86826037573416,
-6.9805563852373));
#41072=CARTESIAN_POINT('Ctrl Pts',(-78.4846093974497,1.69354593282467,-7.02498871546629));
#41073=CARTESIAN_POINT('Ctrl Pts',(-78.385521612233,4.84384239689327,-5.36243928758871));
#41074=CARTESIAN_POINT('Ctrl Pts',(-78.2864338270164,6.81714755954721,-2.39688619470662));
#41075=CARTESIAN_POINT('Ctrl Pts',(-78.1873460417996,7.13397368745932,1.15107936548859));
#41076=CARTESIAN_POINT('Ctrl Pts',(-78.0882582565831,5.71733611307469,4.41934746870483));
#41077=CARTESIAN_POINT('Ctrl Pts',(-77.9891704713662,2.91145951706769,6.61377106948008));
#41078=CARTESIAN_POINT('Ctrl Pts',(-77.8900826861498,-0.601864234570844,
7.20113350259251));
#41079=CARTESIAN_POINT('Ctrl Pts',(-77.7909949009329,-3.96894273075332,
6.03871326352029));
#41080=CARTESIAN_POINT('Ctrl Pts',(-77.6919071157164,-6.37161927345652,
3.40896349542395));
#41081=CARTESIAN_POINT('Ctrl Pts',(-77.5928193304996,-7.22607441539859,
-0.049120485925841));
#41082=CARTESIAN_POINT('Ctrl Pts',(-77.493731545283,-6.32468656464665,-3.49526882199265));
#41083=CARTESIAN_POINT('Ctrl Pts',(-77.3946437600663,-3.8864813567615,-6.0921118622823));
#41084=CARTESIAN_POINT('Ctrl Pts',(-77.2955559748497,-0.503911246964539,
-7.20865020195864));
#41085=CARTESIAN_POINT('Ctrl Pts',(-77.1964681896329,3.0011028041842,-6.57357940833861));
#41086=CARTESIAN_POINT('Ctrl Pts',(-77.0973804044164,5.77688753576599,-4.34121350294215));
#41087=CARTESIAN_POINT('Ctrl Pts',(-76.9982926191996,7.14896301718548,-1.05398864222048));
#41088=CARTESIAN_POINT('Ctrl Pts',(-76.899204833983,6.78393258228553,2.48934188050186));
#41089=CARTESIAN_POINT('Ctrl Pts',(-76.8001170487663,4.77049392422479,5.42779439532762));
#41090=CARTESIAN_POINT('Ctrl Pts',(-76.7010292635497,1.59788669869266,7.04736279590861));
#41091=CARTESIAN_POINT('Ctrl Pts',(-76.6019414783329,-1.96298640977028,
6.95451282507069));
#41092=CARTESIAN_POINT('Ctrl Pts',(-76.5028536931164,-5.04687910892497,
5.17180582958336));
#41093=CARTESIAN_POINT('Ctrl Pts',(-76.4037659078996,-6.90444520127142,
2.1324166435422));
#41094=CARTESIAN_POINT('Ctrl Pts',(-76.304678122683,-7.08432005655309,-1.42512231592074));
#41095=CARTESIAN_POINT('Ctrl Pts',(-76.2055903374662,-5.54279640218294,
-4.63637491182103));
#41096=CARTESIAN_POINT('Ctrl Pts',(-76.1065025522496,-2.65444462742102,
-6.72104813246947));
#41097=CARTESIAN_POINT('Ctrl Pts',(-76.0074147670329,0.878902995794858,
-7.17259324115054));
#41098=CARTESIAN_POINT('Ctrl Pts',(-75.9083269818163,4.19868851354229,-5.88129059350613));
#41099=CARTESIAN_POINT('Ctrl Pts',(-75.8092391965996,6.49824681230373,-3.16091009764594));
#41100=CARTESIAN_POINT('Ctrl Pts',(-75.7101514113829,7.21881484964945,0.327530831367305));
#41101=CARTESIAN_POINT('Ctrl Pts',(-75.6110636261662,6.18530387525653,3.73638598778983));
#41102=CARTESIAN_POINT('Ctrl Pts',(-75.5119758409496,3.64884374164807,6.2373474833499));
#41103=CARTESIAN_POINT('Ctrl Pts',(-75.4128880557329,0.22576158522246,7.22271389338201));
#41104=CARTESIAN_POINT('Ctrl Pts',(-75.3138002705162,-3.25217772802784,
6.45305387427807));
#41105=CARTESIAN_POINT('Ctrl Pts',(-75.2147124852996,-5.93987974970189,
4.11538489549849));
#41106=CARTESIAN_POINT('Ctrl Pts',(-75.1156247000829,-7.18426751298218,
0.777730403754694));
#41107=CARTESIAN_POINT('Ctrl Pts',(-75.0165369148663,-6.68297082227624,
-2.74890255695254));
#41108=CARTESIAN_POINT('Ctrl Pts',(-74.9174491296495,-4.5577983154471,-5.60758760918838));
#41109=CARTESIAN_POINT('Ctrl Pts',(-74.8183613444329,-1.32513953401825,
-7.10370111240595));
#41110=CARTESIAN_POINT('Ctrl Pts',(-74.7192735592163,2.22951108300389,-6.87370675907684));
#41111=CARTESIAN_POINT('Ctrl Pts',(-74.6201857739995,5.24241922863879,-4.97349021414678));
#41112=CARTESIAN_POINT('Ctrl Pts',(-74.5210979887829,6.98148703742991,-1.86477961840367));
#41113=CARTESIAN_POINT('Ctrl Pts',(-74.4220102035662,7.02414343546488,1.69704840149928));
#41114=CARTESIAN_POINT('Ctrl Pts',(-74.3229224183495,5.36002346754426,4.8465155221448));
#41115=CARTESIAN_POINT('Ctrl Pts',(-74.223834633133,2.393486847768,6.8183418063762));
#41116=CARTESIAN_POINT('Ctrl Pts',(-74.1247468479161,-1.15463624180754,
7.13339886927123));
#41117=CARTESIAN_POINT('Ctrl Pts',(-74.0256590626995,-4.42219759928022,
5.71513190328411));
#41118=CARTESIAN_POINT('Ctrl Pts',(-73.9265712774829,-6.61522190929904,
2.90816151025792));
#41119=CARTESIAN_POINT('Ctrl Pts',(-73.8274834922662,-7.20083251626954,
-0.605454665231755));
#41120=CARTESIAN_POINT('Ctrl Pts',(-73.7283957070495,-6.03673358685444,
-3.97195315686868));
#41121=CARTESIAN_POINT('Ctrl Pts',(-73.6293079218328,-3.40578616434171,
-6.37331820026227));
#41122=CARTESIAN_POINT('Ctrl Pts',(-73.5302201366162,0.0527234209035772,
-7.22604902556742));
#41123=CARTESIAN_POINT('Ctrl Pts',(-73.4311323513995,3.49842189408126,-6.32294302758046));
#41124=CARTESIAN_POINT('Ctrl Pts',(-73.3320445661829,6.09404891558392,-3.88344332950621));
#41125=CARTESIAN_POINT('Ctrl Pts',(-73.2329567809661,7.20890055747509,-0.500316931005614));
#41126=CARTESIAN_POINT('Ctrl Pts',(-73.1338689957495,6.57208223290466,3.00438003637265));
#41127=CARTESIAN_POINT('Ctrl Pts',(-73.0347812105329,4.33833259090082,5.77905135898128));
#41128=CARTESIAN_POINT('Ctrl Pts',(-72.9356934253161,1.0504240180843,7.1494876502619));
#41129=CARTESIAN_POINT('Ctrl Pts',(-72.8366056400996,-2.49272405898927,
6.78269054614404));
#41130=CARTESIAN_POINT('Ctrl Pts',(-72.7375178548828,-5.43017230236482,
4.76778701764722));
#41131=CARTESIAN_POINT('Ctrl Pts',(-72.6384300696661,-7.04815863071909,
1.59437266510551));
#41132=CARTESIAN_POINT('Ctrl Pts',(-72.5393422844495,-6.95353321004791,
-1.96645370547505));
#41133=CARTESIAN_POINT('Ctrl Pts',(-72.4402544992328,-5.16928879855788,
-5.04945715855869));
#41134=CARTESIAN_POINT('Ctrl Pts',(-72.3411667140161,-2.12897380262748,
-6.90550757198495));
#41135=CARTESIAN_POINT('Ctrl Pts',(-72.2420789287995,1.42865440073498,-7.08360860594911));
#41136=CARTESIAN_POINT('Ctrl Pts',(-72.1429911435827,4.63913798942724,-5.5404840035929));
#41137=CARTESIAN_POINT('Ctrl Pts',(-72.0439033583662,6.72237081060478,-2.65109316391267));
#41138=CARTESIAN_POINT('Ctrl Pts',(-71.9448155731494,7.17215412606752,0.882479161764341));
#41139=CARTESIAN_POINT('Ctrl Pts',(-71.8457277879328,5.87919638451302,4.20162041971245));
#41140=CARTESIAN_POINT('Ctrl Pts',(-71.7466400027162,3.15766966054934,6.49982204324565));
#41141=CARTESIAN_POINT('Ctrl Pts',(-71.6475522174994,-0.331130112098027,
7.21865064453721));
#41142=CARTESIAN_POINT('Ctrl Pts',(-71.5484644322828,-3.739469533305,6.18344013381704));
#41143=CARTESIAN_POINT('Ctrl Pts',(-71.4493766470661,-6.23916603181327,
3.64573332904139));
#41144=CARTESIAN_POINT('Ctrl Pts',(-71.3502888618495,-7.2228255609445,0.222160291641919));
#41145=CARTESIAN_POINT('Ctrl Pts',(-71.2512010766328,-6.45143152716054,
-3.25539483463601));
#41146=CARTESIAN_POINT('Ctrl Pts',(-71.1521132914161,-4.11242274315051,
-5.94193095387636));
#41147=CARTESIAN_POINT('Ctrl Pts',(-71.0530255061994,-0.774148211036802,
-7.18465439853331));
#41148=CARTESIAN_POINT('Ctrl Pts',(-70.9539377209828,2.75223436335765,-6.68159938099921));
#41149=CARTESIAN_POINT('Ctrl Pts',(-70.854849935766,5.60985944324648,-4.55500178990458));
#41150=CARTESIAN_POINT('Ctrl Pts',(-70.7557621505494,7.1043609477079,-1.32159744389068));
#41151=CARTESIAN_POINT('Ctrl Pts',(-70.6566743653327,6.87259426414465,2.23293805544664));
#41152=CARTESIAN_POINT('Ctrl Pts',(-70.5575865801161,4.97087571091718,5.2448983732413));
#41153=CARTESIAN_POINT('Ctrl Pts',(-70.4584987948994,1.86129839747995,6.98241595399145));
#41154=CARTESIAN_POINT('Ctrl Pts',(-70.3594110096826,-1.70055044827962,
7.02329640922776));
#41155=CARTESIAN_POINT('Ctrl Pts',(-70.2603232244661,-4.84918744252938,
5.35760631497228));
#41156=CARTESIAN_POINT('Ctrl Pts',(-70.1612354392494,-6.81953435813275,
2.3900869057971));
#41157=CARTESIAN_POINT('Ctrl Pts',(-70.0621476540327,-7.13282227768603,
-1.15819283107837));
#41158=CARTESIAN_POINT('Ctrl Pts',(-69.963059868816,-5.7129262726844,-4.42504663047611));
#41159=CARTESIAN_POINT('Ctrl Pts',(-69.8639720835993,-2.90486278046528,
-6.61667110454216));
#41160=CARTESIAN_POINT('Ctrl Pts',(-69.7648842983827,0.60904494537379,-7.20052973978515));
#41161=CARTESIAN_POINT('Ctrl Pts',(-69.6657965131661,3.97496259553755,-6.03475240942767));
#41162=CARTESIAN_POINT('Ctrl Pts',(-69.5667087279493,6.37501554263063,-3.40260798656466));
#41163=CARTESIAN_POINT('Ctrl Pts',(-69.4676209427327,7.22602183930585,0.0563263427741025));
#41164=CARTESIAN_POINT('Ctrl Pts',(-69.368533157516,6.32119791860038,3.50157409644544));
#41165=CARTESIAN_POINT('Ctrl Pts',(-69.2694453722993,3.88040433680823,6.09598445387589));
#41166=CARTESIAN_POINT('Ctrl Pts',(-69.1703575870827,0.496722490665502,
7.20914912082417));
#41167=CARTESIAN_POINT('Ctrl Pts',(-69.0712698018661,-3.00765652165812,
6.57058342361997));
#41168=CARTESIAN_POINT('Ctrl Pts',(-68.9721820166493,-5.78121374549653,
4.33545060032828));
#41169=CARTESIAN_POINT('Ctrl Pts',(-68.8730942314327,-7.15001050594207,
1.04685913280926));
#41170=CARTESIAN_POINT('Ctrl Pts',(-68.774006446216,-6.78144682379192,-2.49610561777696));
#41171=CARTESIAN_POINT('Ctrl Pts',(-68.6749186609993,-4.76507892577756,
-5.43254885942832));
#41172=CARTESIAN_POINT('Ctrl Pts',(-68.5758308757826,-1.59085823514435,
-7.0489527133376));
#41173=CARTESIAN_POINT('Ctrl Pts',(-68.4767430905659,1.96992051229933,-6.95255186631505));
#41174=CARTESIAN_POINT('Ctrl Pts',(-68.3776553053493,5.05203395289501,-5.16677048247999));
#41175=CARTESIAN_POINT('Ctrl Pts',(-68.2785675201327,6.90656822591218,-2.12553043232278));
#41176=CARTESIAN_POINT('Ctrl Pts',(-68.179479734916,7.08289539441553,1.43218613014226));
#41177=CARTESIAN_POINT('Ctrl Pts',(-68.0803919496992,5.53817022743053,4.64189991420173));
#41178=CARTESIAN_POINT('Ctrl Pts',(-67.9813041644827,2.64774104169769,6.72369181655289));
#41179=CARTESIAN_POINT('Ctrl Pts',(-67.8822163792659,-0.886055109091175,
7.17171322992696));
#41180=CARTESIAN_POINT('Ctrl Pts',(-67.7831285940493,-4.2045512798272,5.87710070992006));
#41181=CARTESIAN_POINT('Ctrl Pts',(-67.6840408088326,-6.5013956613676,3.15442844655903));
#41182=CARTESIAN_POINT('Ctrl Pts',(-67.5849530236159,-7.21848463861485,
-0.334729326969879));
#41183=CARTESIAN_POINT('Ctrl Pts',(-67.4858652383994,-6.18157486775541,
-3.74255211578994));
#41184=CARTESIAN_POINT('Ctrl Pts',(-67.3867774531825,-3.64262198451628,
-6.24098309687747));
#41185=CARTESIAN_POINT('Ctrl Pts',(-67.287689667966,-0.218558994684405,
-7.22293529562393));
#41186=CARTESIAN_POINT('Ctrl Pts',(-67.1886018827493,3.25861123708332,-6.44980785450514));
#41187=CARTESIAN_POINT('Ctrl Pts',(-67.0895140975325,5.94398046764703,-4.10945900406941));
#41188=CARTESIAN_POINT('Ctrl Pts',(-66.990426312316,7.18503993028725,-0.770566970261787));
#41189=CARTESIAN_POINT('Ctrl Pts',(-66.8913385270992,6.68022540195615,2.7555678061177));
#41190=CARTESIAN_POINT('Ctrl Pts',(-66.7922507418826,4.5522059096846,5.6121251770881));
#41191=CARTESIAN_POINT('Ctrl Pts',(-66.693162956666,1.31805142041421,7.10502855866105));
#41192=CARTESIAN_POINT('Ctrl Pts',(-66.5940751714492,-2.23635716309218,
6.87146071173886));
#41193=CARTESIAN_POINT('Ctrl Pts',(-66.4949873862326,-5.2473910361686,4.96829921252571));
#41194=CARTESIAN_POINT('Ctrl Pts',(-66.395899601016,-6.9833130755638,1.85773707522965));
#41195=CARTESIAN_POINT('Ctrl Pts',(-66.2968118157991,-7.02250852220407,
-1.70388912091449));
#41196=CARTESIAN_POINT('Ctrl Pts',(-66.1977240305827,-5.35506230134601,
-4.85219885400573));
#41197=CARTESIAN_POINT('Ctrl Pts',(-66.1316655071048,-3.37628014142085,
-6.16377412581316));
#41198=CARTESIAN_POINT('Ctrl Pts',(-66.0986362453659,-2.28983447448481,
-6.54393972156383));
#41199=CARTESIAN_POINT('Ctrl Pts',(-67.5941716636062,-6.9334612849287,-0.000104716709421631));
#41200=CARTESIAN_POINT('Ctrl Pts',(-67.5910987836095,-6.93353940129172,
-0.107169118010251));
#41201=CARTESIAN_POINT('Ctrl Pts',(-67.5880259036127,-6.93111060609849,
-0.214229973520828));
#41202=CARTESIAN_POINT('Ctrl Pts',(-67.5849530236159,-6.92615151393041,
-0.321173496184973));
#41203=CARTESIAN_POINT('Ctrl Pts',(-67.5519237618771,-6.87284804832839,
-1.47067025657647));
#41204=CARTESIAN_POINT('Ctrl Pts',(-67.5188945001382,-6.52721145804193,
-2.60661118618316));
#41205=CARTESIAN_POINT('Ctrl Pts',(-67.4858652383993,-5.93123434902551,
-3.59098681450111));
#41206=CARTESIAN_POINT('Ctrl Pts',(-67.4528359766604,-5.33525724000907,
-4.57536244281908));
#41207=CARTESIAN_POINT('Ctrl Pts',(-67.4198067149215,-4.48893961226268,
-5.40817276984829));
#41208=CARTESIAN_POINT('Ctrl Pts',(-67.3867774531826,-3.49510363341746,
-5.98823663315398));
#41209=CARTESIAN_POINT('Ctrl Pts',(-67.3537481914437,-2.50126765457231,
-6.56830049645963));
#41210=CARTESIAN_POINT('Ctrl Pts',(-67.3207189297048,-1.35991332462838,
-6.89561789604178));
#41211=CARTESIAN_POINT('Ctrl Pts',(-67.2876896679659,-0.209707787695129,
-6.93042202231306));
#41212=CARTESIAN_POINT('Ctrl Pts',(-67.2546604062271,0.940497749238154,
-6.96522614858434));
#41213=CARTESIAN_POINT('Ctrl Pts',(-67.2216311444882,2.09955449316073,-6.70751700154474));
#41214=CARTESIAN_POINT('Ctrl Pts',(-67.1886018827493,3.12664440354932,-6.18860428628565));
#41215=CARTESIAN_POINT('Ctrl Pts',(-67.1555726210104,4.15373431393791,-5.66969157102655));
#41216=CARTESIAN_POINT('Ctrl Pts',(-67.1225433592715,5.04885739079248,-4.88957528754798));
#41217=CARTESIAN_POINT('Ctrl Pts',(-67.0895140975326,5.70326217299314,-3.94303514017407));
#41218=CARTESIAN_POINT('Ctrl Pts',(-67.0564848357937,6.35766695519376,-2.99649499280022));
#41219=CARTESIAN_POINT('Ctrl Pts',(-67.0234555740548,6.77135344274051,-1.88353098153098));
#41220=CARTESIAN_POINT('Ctrl Pts',(-66.9904263123159,6.89406093179203,-0.739359846499843));
#41221=CARTESIAN_POINT('Ctrl Pts',(-66.9573970505771,7.01676842084356,0.404811288531357));
#41222=CARTESIAN_POINT('Ctrl Pts',(-66.9243677888382,6.84849691139986,1.58018954732452));
#41223=CARTESIAN_POINT('Ctrl Pts',(-66.8913385270993,6.40969124129941,2.64397157188285));
#41224=CARTESIAN_POINT('Ctrl Pts',(-66.8583092653603,5.97088557119897,3.70775359644117));
#41225=CARTESIAN_POINT('Ctrl Pts',(-66.8252800036215,5.26154574044179,4.65993938676463));
#41226=CARTESIAN_POINT('Ctrl Pts',(-66.7922507418826,4.36785007685146,5.38484951218853));
#41227=CARTESIAN_POINT('Ctrl Pts',(-66.7592214801437,3.47415441326111,6.10975963761244));
#41228=CARTESIAN_POINT('Ctrl Pts',(-66.7261922184048,2.39610291683771,6.60739409813673));
#41229=CARTESIAN_POINT('Ctrl Pts',(-66.6931629566659,1.26467573804154,6.81728335391186));
#41230=CARTESIAN_POINT('Ctrl Pts',(-66.6601336949271,0.133248559245465,
7.02717260968697));
#41231=CARTESIAN_POINT('Ctrl Pts',(-66.6271044331882,-1.05155430192337,
6.94931666071291));
#41232=CARTESIAN_POINT('Ctrl Pts',(-66.5940751714492,-2.14579471135379,
6.59319510302372));
#41233=CARTESIAN_POINT('Ctrl Pts',(-66.5662901142995,-3.06629764453912,
6.29361656836326));
#41234=CARTESIAN_POINT('Ctrl Pts',(-66.5385050571497,-3.92271312249685,
5.79712049892313));
#41235=CARTESIAN_POINT('Ctrl Pts',(-66.51072,-4.64244039278582,5.14956429285673));
#41236=CARTESIAN_POINT('',(-86.51072,-2.05430500584057,-5.87042930427706));
#41237=CARTESIAN_POINT('Ctrl Pts',(-86.51072,-2.0543050058407,-5.87042930427701));
#41238=CARTESIAN_POINT('Ctrl Pts',(-86.51072,-2.21258203238063,-5.82486884494219));
#41239=CARTESIAN_POINT('Ctrl Pts',(-86.51072,-2.36882106524609,-5.77305057653388));
#41240=CARTESIAN_POINT('Ctrl Pts',(-86.51072,-2.52263632570939,-5.71505524575264));
#41241=CARTESIAN_POINT('Ctrl Pts',(-86.51072,-2.68507439158213,-5.65380872617208));
#41242=CARTESIAN_POINT('Ctrl Pts',(-86.51072,-2.84481012954198,-5.58567374017774));
#41243=CARTESIAN_POINT('Ctrl Pts',(-86.51072,-3.00150353946984,-5.510969810184));
#41244=CARTESIAN_POINT('Ctrl Pts',(-86.51072,-3.10062155384214,-5.46371507745341));
#41245=CARTESIAN_POINT('Ctrl Pts',(-86.51072,-3.19852205088825,-5.41383083132198));
#41246=CARTESIAN_POINT('Ctrl Pts',(-86.51072,-3.29511573121791,-5.36138774998078));
#41247=CARTESIAN_POINT('Ctrl Pts',(-86.51072,-3.36158388237246,-5.32530055829598));
#41248=CARTESIAN_POINT('Ctrl Pts',(-86.51072,-3.42743318663604,-5.28800156865333));
#41249=CARTESIAN_POINT('Ctrl Pts',(-86.51072,-3.49263358329869,-5.24951180053227));
#41250=CARTESIAN_POINT('Ctrl Pts',(-86.51072,-3.5235350127469,-5.23126975117442));
#41251=CARTESIAN_POINT('Ctrl Pts',(-86.51072,-3.55429475124542,-5.21275759435068));
#41252=CARTESIAN_POINT('Ctrl Pts',(-86.51072,-3.5848840724756,-5.19399336730484));
#41253=CARTESIAN_POINT('Ctrl Pts',(-86.51072,-3.73562442368972,-5.10152560203904));
#41254=CARTESIAN_POINT('Ctrl Pts',(-86.51072,-3.88233609651536,-5.00287892045257));
#41255=CARTESIAN_POINT('Ctrl Pts',(-86.51072,-4.02466996944556,-4.89838649052438));
#41256=CARTESIAN_POINT('Ctrl Pts',(-86.51072,-4.16747158240373,-4.79355067577084));
#41257=CARTESIAN_POINT('Ctrl Pts',(-86.51072,-4.30586721806361,-4.68283025738495));
#41258=CARTESIAN_POINT('Ctrl Pts',(-86.51072,-4.43948328000296,-4.56651347834845));
#41259=CARTESIAN_POINT('Ctrl Pts',(-86.51072,-4.55409609756718,-4.46673959202169));
#41260=CARTESIAN_POINT('Ctrl Pts',(-86.51072,-4.66519208352877,-4.36284708277001));
#41261=CARTESIAN_POINT('Ctrl Pts',(-86.51072,-4.7725177187907,-4.25499289066315));
#41262=CARTESIAN_POINT('Ctrl Pts',(-86.51072,-4.78886696746902,-4.23856312527251));
#41263=CARTESIAN_POINT('Ctrl Pts',(-86.51072,-4.80512868733647,-4.222041387261));
#41264=CARTESIAN_POINT('Ctrl Pts',(-86.51072,-4.82130194150653,-4.20542818885453));
#41265=CARTESIAN_POINT('Ctrl Pts',(-86.51072,-4.83838504707905,-4.18788038930284));
#41266=CARTESIAN_POINT('Ctrl Pts',(-86.51072,-4.85536377248283,-4.17023635893039));
#41267=CARTESIAN_POINT('Ctrl Pts',(-86.51072,-4.87223399895435,-4.1525003326935));
#41268=CARTESIAN_POINT('Ctrl Pts',(-86.51072,-4.94423933928611,-4.07679959402962));
#41269=CARTESIAN_POINT('Ctrl Pts',(-86.51072,-5.01428728250921,-3.99940388048743));
#41270=CARTESIAN_POINT('Ctrl Pts',(-86.51072,-5.08230936468395,-3.92037913736578));
#41271=CARTESIAN_POINT('Ctrl Pts',(-86.51072,-5.19718047715216,-3.78692747189664));
#41272=CARTESIAN_POINT('Ctrl Pts',(-86.51072,-5.30627615206813,-3.64883247781431));
#41273=CARTESIAN_POINT('Ctrl Pts',(-86.51072,-5.40947963808152,-3.50655586542704));
#41274=CARTESIAN_POINT('Ctrl Pts',(-86.51072,-5.51401899965164,-3.3624376112879));
#41275=CARTESIAN_POINT('Ctrl Pts',(-86.51072,-5.61251306134529,-3.214028262726));
#41276=CARTESIAN_POINT('Ctrl Pts',(-86.51072,-5.70480528363513,-3.06176720920456));
#41277=CARTESIAN_POINT('Ctrl Pts',(-86.51072,-5.7988808937585,-2.90656397373501));
#41278=CARTESIAN_POINT('Ctrl Pts',(-86.51072,-5.88651318998411,-2.74735818652822));
#41279=CARTESIAN_POINT('Ctrl Pts',(-86.51072,-5.96749284788747,-2.58458156019617));
#41280=CARTESIAN_POINT('Ctrl Pts',(-86.51072,-6.02822759131498,-2.46249909044713));
#41281=CARTESIAN_POINT('Ctrl Pts',(-86.51072,-6.08521936563103,-2.33840726205514));
#41282=CARTESIAN_POINT('Ctrl Pts',(-86.51072,-6.13836158920561,-2.21247913102859));
#41283=CARTESIAN_POINT('Ctrl Pts',(-86.51072,-6.15312996736535,-2.17748333795005));
#41284=CARTESIAN_POINT('Ctrl Pts',(-86.51072,-6.16760094584908,-2.14234569051137));
#41285=CARTESIAN_POINT('Ctrl Pts',(-86.51072,-6.18177200434075,-2.10706982588161));
#41286=CARTESIAN_POINT('Ctrl Pts',(-86.51072,-6.19016620801788,-2.0861742242748));
#41287=CARTESIAN_POINT('Ctrl Pts',(-86.51072,-6.19845156921919,-2.06523907577952));
#41288=CARTESIAN_POINT('Ctrl Pts',(-86.51072,-6.20662688291449,-2.04426772949609));
#41289=CARTESIAN_POINT('Ctrl Pts',(-86.51072,-6.27282658558699,-1.87445199638191));
#41290=CARTESIAN_POINT('Ctrl Pts',(-86.51072,-6.33183472169884,-1.70221357249591));
#41291=CARTESIAN_POINT('Ctrl Pts',(-86.51072,-6.38350915294916,-1.52801731240776));
#41292=CARTESIAN_POINT('Ctrl Pts',(-86.51072,-6.43097870038066,-1.36799585826559));
#41293=CARTESIAN_POINT('Ctrl Pts',(-86.51072,-6.47225930007859,-1.20632141719495));
#41294=CARTESIAN_POINT('Ctrl Pts',(-86.51072,-6.5072089203001,-1.04333227579861));
#41295=CARTESIAN_POINT('Ctrl Pts',(-86.51072,-6.54508051000339,-0.866716397001247));
#41296=CARTESIAN_POINT('Ctrl Pts',(-86.51072,-6.57551927259713,-0.688556492077032));
#41297=CARTESIAN_POINT('Ctrl Pts',(-86.51072,-6.59859730560256,-0.509314630244122));
#41298=CARTESIAN_POINT('Ctrl Pts',(-86.51072,-6.62179814420949,-0.329118965084463));
#41299=CARTESIAN_POINT('Ctrl Pts',(-86.51072,-6.63755977647099,-0.147829089728884));
#41300=CARTESIAN_POINT('Ctrl Pts',(-86.51072,-6.64590383774985,0.0340957911597833));
#41301=CARTESIAN_POINT('Ctrl Pts',(-86.51072,-6.65018668746203,0.127474410721004));
#41302=CARTESIAN_POINT('Ctrl Pts',(-86.51072,-6.65251448290405,0.221020427310341));
#41303=CARTESIAN_POINT('Ctrl Pts',(-86.51072,-6.65288481617016,0.314671846891448));
#41304=CARTESIAN_POINT('Ctrl Pts',(-86.51072,-6.65298022561412,0.338799384669037));
#41305=CARTESIAN_POINT('Ctrl Pts',(-86.51072,-6.65294569190618,0.362933917091072));
#41306=CARTESIAN_POINT('Ctrl Pts',(-86.51072,-6.65278113473496,0.387074380312947));
#41307=CARTESIAN_POINT('Ctrl Pts',(-86.51072,-6.65264760834661,0.406662641602241));
#41308=CARTESIAN_POINT('Ctrl Pts',(-86.51072,-6.65242845612529,0.426253125446996));
#41309=CARTESIAN_POINT('Ctrl Pts',(-86.51072,-6.65212390032766,0.44583583961078));
#41310=CARTESIAN_POINT('Ctrl Pts',(-86.51072,-6.64926295208706,0.629792710789254));
#41311=CARTESIAN_POINT('Ctrl Pts',(-86.51072,-6.63886861132718,0.813294091649382));
#41312=CARTESIAN_POINT('Ctrl Pts',(-86.51072,-6.62105508637465,0.99586126198024));
#41313=CARTESIAN_POINT('Ctrl Pts',(-86.51072,-6.60311620074966,1.17971322817846));
#41314=CARTESIAN_POINT('Ctrl Pts',(-86.51072,-6.57765339445709,1.3626185090582));
#41315=CARTESIAN_POINT('Ctrl Pts',(-86.51072,-6.54473157195455,1.54409959934158));
#41316=CARTESIAN_POINT('Ctrl Pts',(-86.51072,-6.51186414550787,1.72528083212095));
#41317=CARTESIAN_POINT('Ctrl Pts',(-86.51072,-6.47156232283033,1.90504331604601));
#41318=CARTESIAN_POINT('Ctrl Pts',(-86.51072,-6.42383907511914,2.08291224064793));
#41319=CARTESIAN_POINT('Ctrl Pts',(-86.51072,-6.40891009319694,2.13855392656113));
#41320=CARTESIAN_POINT('Ctrl Pts',(-86.51072,-6.39325447880982,2.19401026896043));
#41321=CARTESIAN_POINT('Ctrl Pts',(-86.51072,-6.37687159035412,2.2492665620533));
#41322=CARTESIAN_POINT('Ctrl Pts',(-86.51072,-6.33649222484637,2.38545830024617));
#41323=CARTESIAN_POINT('Ctrl Pts',(-86.51072,-6.29169596317493,2.5204351980553));
#41324=CARTESIAN_POINT('Ctrl Pts',(-86.51072,-6.24259276678192,2.65402287965289));
#41325=CARTESIAN_POINT('Ctrl Pts',(-86.51072,-6.22111011835998,2.71246749035183));
#41326=CARTESIAN_POINT('Ctrl Pts',(-86.51072,-6.19880287065572,2.77064611712136));
#41327=CARTESIAN_POINT('Ctrl Pts',(-86.51072,-6.17567920954438,2.8285437301309));
#41328=CARTESIAN_POINT('Ctrl Pts',(-86.51072,-6.16282195963146,2.86073604069284));
#41329=CARTESIAN_POINT('Ctrl Pts',(-86.51072,-6.14971229671456,2.89284146794668));
#41330=CARTESIAN_POINT('Ctrl Pts',(-86.51072,-6.13635154810387,2.92485738642242));
#41331=CARTESIAN_POINT('Ctrl Pts',(-86.51072,-6.12730729434025,2.94652983155313));
#41332=CARTESIAN_POINT('Ctrl Pts',(-86.51072,-6.11814757446991,2.96816209171322));
#41333=CARTESIAN_POINT('Ctrl Pts',(-86.51072,-6.1088795489188,2.98973796773027));
#41334=CARTESIAN_POINT('Ctrl Pts',(-86.51072,-6.03607183109103,3.15923364771886));
#41335=CARTESIAN_POINT('Ctrl Pts',(-86.51072,-5.95649247563341,3.32547331851885));
#41336=CARTESIAN_POINT('Ctrl Pts',(-86.51072,-5.87047713602277,3.48810950866876));
#41337=CARTESIAN_POINT('Ctrl Pts',(-86.51072,-5.7829205374938,3.65365988226137));
#41338=CARTESIAN_POINT('Ctrl Pts',(-86.51072,-5.68869505582976,3.8154771215784));
#41339=CARTESIAN_POINT('Ctrl Pts',(-86.51072,-5.58810168441886,3.9731849792754));
#41340=CARTESIAN_POINT('Ctrl Pts',(-86.51072,-5.48731664960083,4.13119332223216));
#41341=CARTESIAN_POINT('Ctrl Pts',(-86.51072,-5.38013910716857,4.28507725418091));
#41342=CARTESIAN_POINT('Ctrl Pts',(-86.51072,-5.26682312986106,4.4344389749387));
#41343=CARTESIAN_POINT('Ctrl Pts',(-86.51072,-5.15467074727413,4.58226696220309));
#41344=CARTESIAN_POINT('Ctrl Pts',(-86.51072,-5.03650494943115,4.72566571734121));
#41345=CARTESIAN_POINT('Ctrl Pts',(-86.51072,-4.91253002400078,4.8642215159004));
#41346=CARTESIAN_POINT('Ctrl Pts',(-86.51072,-4.82526136656507,4.96175396835574));
#41347=CARTESIAN_POINT('Ctrl Pts',(-86.51072,-4.73511337439158,5.0568861415784));
#41348=CARTESIAN_POINT('Ctrl Pts',(-86.51072,-4.64214617842369,5.1494628708387));
#41349=CARTESIAN_POINT('Ctrl Pts',(-86.51072,-2.05430500584057,-5.87042930427706));
#41350=CARTESIAN_POINT('Ctrl Pts',(-86.4829349428503,-1.2342747841181,-6.15647891042869));
#41351=CARTESIAN_POINT('Ctrl Pts',(-86.4221206239616,0.693371089156462,
-6.40526944857501));
#41352=CARTESIAN_POINT('Ctrl Pts',(-86.3282770433341,3.55493808738742,-5.42058662271333));
#41353=CARTESIAN_POINT('Ctrl Pts',(-86.2291892581173,5.71261075920097,-3.06370552006469));
#41354=CARTESIAN_POINT('Ctrl Pts',(-86.1301014729008,6.48219330078747,0.0375972645595515));
#41355=CARTESIAN_POINT('Ctrl Pts',(-86.031013687684,5.67668603654431,3.12977391169855));
#41356=CARTESIAN_POINT('Ctrl Pts',(-85.9319259024675,3.49181736371615,5.46145112616022));
#41357=CARTESIAN_POINT('Ctrl Pts',(-85.8328381172506,0.45848197210095,6.46606838804796));
#41358=CARTESIAN_POINT('Ctrl Pts',(-85.7337503320341,-2.68625859143277,
5.89951319007443));
#41359=CARTESIAN_POINT('Ctrl Pts',(-85.6346625468174,-5.17827294326576,
3.89945285036088));
#41360=CARTESIAN_POINT('Ctrl Pts',(-85.5588309088861,-6.12246698761767,
1.64367910817076));
#41361=CARTESIAN_POINT('Ctrl Pts',(-85.5160285326938,-6.21932780933381,
0.305694574820658));
#41362=CARTESIAN_POINT('Ctrl Pts',(-85.5062554182403,-6.21904930984993,
0.000151106537523774));
#41363=CARTESIAN_POINT('Origin',(-86.51072,-1.12618006296016E-15,0.));
#41364=CARTESIAN_POINT('',(-86.51072,4.88092761120804,-3.85429840783598));
#41365=CARTESIAN_POINT('Ctrl Pts',(-86.51072,1.15840596835156,6.83581456945577));
#41366=CARTESIAN_POINT('Ctrl Pts',(-86.51072,1.33692099159029,6.79654210588011));
#41367=CARTESIAN_POINT('Ctrl Pts',(-86.51072,1.51361902021433,6.75022761845211));
#41368=CARTESIAN_POINT('Ctrl Pts',(-86.51072,1.68807314422841,6.69687225419658));
#41369=CARTESIAN_POINT('Ctrl Pts',(-86.51072,1.8679641935395,6.64185405089215));
#41370=CARTESIAN_POINT('Ctrl Pts',(-86.51072,2.04547001034044,6.57934922676145));
#41371=CARTESIAN_POINT('Ctrl Pts',(-86.51072,2.22017980815463,6.5096135659802));
#41372=CARTESIAN_POINT('Ctrl Pts',(-86.51072,2.32989175485023,6.46582188861501));
#41373=CARTESIAN_POINT('Ctrl Pts',(-86.51072,2.43850069933779,6.41917781777568));
#41374=CARTESIAN_POINT('Ctrl Pts',(-86.51072,2.54589939897303,6.36973577164565));
#41375=CARTESIAN_POINT('Ctrl Pts',(-86.51072,2.61317957816801,6.33876268040066));
#41376=CARTESIAN_POINT('Ctrl Pts',(-86.51072,2.67998471465285,6.30669141181624));
#41377=CARTESIAN_POINT('Ctrl Pts',(-86.51072,2.746287399481,6.27353409609559));
#41378=CARTESIAN_POINT('Ctrl Pts',(-86.51072,2.77514683716407,6.25910177726479));
#41379=CARTESIAN_POINT('Ctrl Pts',(-86.51072,2.80391107023024,6.24446368602063));
#41380=CARTESIAN_POINT('Ctrl Pts',(-86.51072,2.8325777855864,6.22962076918156));
#41381=CARTESIAN_POINT('Ctrl Pts',(-86.51072,2.85655241758811,6.21720729715912));
#41382=CARTESIAN_POINT('Ctrl Pts',(-86.51072,2.88045005876997,6.20465510637532));
#41383=CARTESIAN_POINT('Ctrl Pts',(-86.51072,2.9042688372644,6.19196540548103));
#41384=CARTESIAN_POINT('Ctrl Pts',(-86.51072,3.06900614318828,6.10419989984044));
#41385=CARTESIAN_POINT('Ctrl Pts',(-86.51072,3.22998445162522,6.00985446247505));
#41386=CARTESIAN_POINT('Ctrl Pts',(-86.51072,3.3868033547833,5.90918193833376));
#41387=CARTESIAN_POINT('Ctrl Pts',(-86.51072,3.542839639644,5.80901182913002));
#41388=CARTESIAN_POINT('Ctrl Pts',(-86.51072,3.69475849445778,5.70257718309574));
#41389=CARTESIAN_POINT('Ctrl Pts',(-86.51072,3.84213367303502,5.59008687856596));
#41390=CARTESIAN_POINT('Ctrl Pts',(-86.51072,3.9701437417514,5.49237780874973));
#41391=CARTESIAN_POINT('Ctrl Pts',(-86.51072,4.09472550320262,5.3900991786712));
#41392=CARTESIAN_POINT('Ctrl Pts',(-86.51072,4.21557502487895,5.28336686568389));
#41393=CARTESIAN_POINT('Ctrl Pts',(-86.51072,4.23486407962035,5.26633108929578));
#41394=CARTESIAN_POINT('Ctrl Pts',(-86.51072,4.25405799861312,5.24918181409541));
#41395=CARTESIAN_POINT('Ctrl Pts',(-86.51072,4.27315548388442,5.23191947067406));
#41396=CARTESIAN_POINT('Ctrl Pts',(-86.51072,4.29206103730179,5.21483061572666));
#41397=CARTESIAN_POINT('Ctrl Pts',(-86.51072,4.31086653414738,5.19763593809285));
#41398=CARTESIAN_POINT('Ctrl Pts',(-86.51072,4.32956613773457,5.18034051383287));
#41399=CARTESIAN_POINT('Ctrl Pts',(-86.51072,4.41032297928591,5.10564781620356));
#41400=CARTESIAN_POINT('Ctrl Pts',(-86.51072,4.4891337278863,5.0290507628448));
#41401=CARTESIAN_POINT('Ctrl Pts',(-86.51072,4.56591797340772,4.95060089892119));
#41402=CARTESIAN_POINT('Ctrl Pts',(-86.51072,4.6939867687781,4.81975401097639));
#41403=CARTESIAN_POINT('Ctrl Pts',(-86.51072,4.81642027662916,4.6837546034005));
#41404=CARTESIAN_POINT('Ctrl Pts',(-86.51072,4.93302139785161,4.54303258748792));
#41405=CARTESIAN_POINT('Ctrl Pts',(-86.51072,5.05026750854921,4.40153215522537));
#41406=CARTESIAN_POINT('Ctrl Pts',(-86.51072,5.16161690091574,4.25525608476221));
#41407=CARTESIAN_POINT('Ctrl Pts',(-86.51072,5.26682651345902,4.10461066568728));
#41408=CARTESIAN_POINT('Ctrl Pts',(-86.51072,5.37240253202624,3.95344060454123));
#41409=CARTESIAN_POINT('Ctrl Pts',(-86.51072,5.47179630518351,3.79787005449489));
#41410=CARTESIAN_POINT('Ctrl Pts',(-86.51072,5.56471377525825,3.63828838878779));
#41411=CARTESIAN_POINT('Ctrl Pts',(-86.51072,5.63440187781431,3.51860213950746));
#41412=CARTESIAN_POINT('Ctrl Pts',(-86.51072,5.70044609905939,3.39665914206459));
#41413=CARTESIAN_POINT('Ctrl Pts',(-86.51072,5.76270266675695,3.27261923926715));
#41414=CARTESIAN_POINT('Ctrl Pts',(-86.51072,5.77939659018424,3.23935828840188));
#41415=CARTESIAN_POINT('Ctrl Pts',(-86.51072,5.79581807160992,3.2059465515095));
#41416=CARTESIAN_POINT('Ctrl Pts',(-86.51072,5.81196411860362,3.17238708947047));
#41417=CARTESIAN_POINT('Ctrl Pts',(-86.51072,5.82152069713481,3.15252379819144));
#41418=CARTESIAN_POINT('Ctrl Pts',(-86.51072,5.83098064485861,3.13260893175539));
#41419=CARTESIAN_POINT('Ctrl Pts',(-86.51072,5.84033745115676,3.11265599748321));
#41420=CARTESIAN_POINT('Ctrl Pts',(-86.51072,5.91732823406407,2.94847689812347));
#41421=CARTESIAN_POINT('Ctrl Pts',(-86.51072,5.98744586695114,2.78150324016161));
#41422=CARTESIAN_POINT('Ctrl Pts',(-86.51072,6.05048064190744,2.61213298066552));
#41423=CARTESIAN_POINT('Ctrl Pts',(-86.51072,6.11164633069412,2.4477848317392));
#41424=CARTESIAN_POINT('Ctrl Pts',(-86.51072,6.16614302472095,2.28117943087884));
#41425=CARTESIAN_POINT('Ctrl Pts',(-86.51072,6.21373523303752,2.11266378330039));
#41426=CARTESIAN_POINT('Ctrl Pts',(-86.51072,6.26289076481001,1.9386126820444));
#41427=CARTESIAN_POINT('Ctrl Pts',(-86.51072,6.30468105067439,1.76252310782449));
#41428=CARTESIAN_POINT('Ctrl Pts',(-86.51072,6.33908486826123,1.58487065370346));
#41429=CARTESIAN_POINT('Ctrl Pts',(-86.51072,6.37335665238351,1.40789998639134));
#41430=CARTESIAN_POINT('Ctrl Pts',(-86.51072,6.40029851150814,1.22937766976392));
#41431=CARTESIAN_POINT('Ctrl Pts',(-86.51072,6.41983807680747,1.04977659578172));
#41432=CARTESIAN_POINT('Ctrl Pts',(-86.51072,6.42952443815511,0.960742839177272));
#41433=CARTESIAN_POINT('Ctrl Pts',(-86.51072,6.43739090288072,0.871444091179049));
#41434=CARTESIAN_POINT('Ctrl Pts',(-86.51072,6.44342398767677,0.781939070998599));
#41435=CARTESIAN_POINT('Ctrl Pts',(-86.51072,6.44512671191955,0.756677969445425));
#41436=CARTESIAN_POINT('Ctrl Pts',(-86.51072,6.44668338047881,0.731400443643511));
#41437=CARTESIAN_POINT('Ctrl Pts',(-86.51072,6.44809364563389,0.706107829474976));
#41438=CARTESIAN_POINT('Ctrl Pts',(-86.51072,6.44937238190223,0.683174140060691));
#41439=CARTESIAN_POINT('Ctrl Pts',(-86.51072,6.45053028956465,0.660235926315252));
#41440=CARTESIAN_POINT('Ctrl Pts',(-86.51072,6.45156713961303,0.6373001126248));
#41441=CARTESIAN_POINT('Ctrl Pts',(-86.51072,6.45963992153548,0.458724799418353));
#41442=CARTESIAN_POINT('Ctrl Pts',(-86.51072,6.46038493546743,0.280181222650435));
#41443=CARTESIAN_POINT('Ctrl Pts',(-86.51072,6.45382244972886,0.102127507862334));
#41444=CARTESIAN_POINT('Ctrl Pts',(-86.51072,6.4472673704612,-0.0757252541600348));
#41445=CARTESIAN_POINT('Ctrl Pts',(-86.51072,6.43342122692505,-0.25308999531447));
#41446=CARTESIAN_POINT('Ctrl Pts',(-86.51072,6.41225241327616,-0.429508005108766));
#41447=CARTESIAN_POINT('Ctrl Pts',(-86.51072,6.3913431695847,-0.603762794230776));
#41448=CARTESIAN_POINT('Ctrl Pts',(-86.51072,6.36328960685773,-0.777094595050165));
#41449=CARTESIAN_POINT('Ctrl Pts',(-86.51072,6.32801215972376,-0.949048880875677));
#41450=CARTESIAN_POINT('Ctrl Pts',(-86.51072,6.31879999759548,-0.993952094922312));
#41451=CARTESIAN_POINT('Ctrl Pts',(-86.51072,6.30909497216788,-1.03876127814759));
#41452=CARTESIAN_POINT('Ctrl Pts',(-86.51072,6.29889512145856,-1.08346810792257));
#41453=CARTESIAN_POINT('Ctrl Pts',(-86.51072,6.26977492480713,-1.21110445396444));
#41454=CARTESIAN_POINT('Ctrl Pts',(-86.51072,6.23662241077162,-1.33790715393257));
#41455=CARTESIAN_POINT('Ctrl Pts',(-86.51072,6.19950420606752,-1.46370056227431));
#41456=CARTESIAN_POINT('Ctrl Pts',(-86.51072,6.18326499150948,-1.51873517842382));
#41457=CARTESIAN_POINT('Ctrl Pts',(-86.51072,6.16626655521156,-1.57357650063582));
#41458=CARTESIAN_POINT('Ctrl Pts',(-86.51072,6.14851373823978,-1.62820926346126));
#41459=CARTESIAN_POINT('Ctrl Pts',(-86.51072,6.13799943741682,-1.66056611725236));
#41460=CARTESIAN_POINT('Ctrl Pts',(-86.51072,6.1272205118688,-1.69284980717819));
#41461=CARTESIAN_POINT('Ctrl Pts',(-86.51072,6.11617789691174,-1.72505709862759));
#41462=CARTESIAN_POINT('Ctrl Pts',(-86.51072,6.1076826296012,-1.74983470350426));
#41463=CARTESIAN_POINT('Ctrl Pts',(-86.51072,6.09903040399726,-1.77456940026785));
#41464=CARTESIAN_POINT('Ctrl Pts',(-86.51072,6.09022962359805,-1.79923786075214));
#41465=CARTESIAN_POINT('Ctrl Pts',(-86.51072,6.03143262794601,-1.96404499126166));
#41466=CARTESIAN_POINT('Ctrl Pts',(-86.51072,5.96593941819338,-2.12610508285074));
#41467=CARTESIAN_POINT('Ctrl Pts',(-86.51072,5.89400145244168,-2.28504090903752));
#41468=CARTESIAN_POINT('Ctrl Pts',(-86.51072,5.82166151986319,-2.44486481885369));
#41469=CARTESIAN_POINT('Ctrl Pts',(-86.51072,5.74280425690578,-2.60153010257179));
#41470=CARTESIAN_POINT('Ctrl Pts',(-86.51072,5.65763771959783,-2.75463161937262));
#41471=CARTESIAN_POINT('Ctrl Pts',(-86.51072,5.5729853246012,-2.90680887683164));
#41472=CARTESIAN_POINT('Ctrl Pts',(-86.51072,5.48209918836071,-3.05546585368127));
#41473=CARTESIAN_POINT('Ctrl Pts',(-86.51072,5.38514254021834,-3.20017426124779));
#41474=CARTESIAN_POINT('Ctrl Pts',(-86.51072,5.29007319202304,-3.34206586176525));
#41475=CARTESIAN_POINT('Ctrl Pts',(-86.51072,5.18916691890737,-3.48016157013249));
#41476=CARTESIAN_POINT('Ctrl Pts',(-86.51072,5.08254442327496,-3.61402073215818));
#41477=CARTESIAN_POINT('Ctrl Pts',(-86.51072,5.01746184271968,-3.69572862732539));
#41478=CARTESIAN_POINT('Ctrl Pts',(-86.51072,4.95024883314754,-3.77585727781971));
#41479=CARTESIAN_POINT('Ctrl Pts',(-86.51072,4.88092761120814,-3.85429840783586));
#41480=CARTESIAN_POINT('Origin',(-86.51072,0.,0.));
#41481=CARTESIAN_POINT('Origin',(-88.8777445817596,0.,0.));
#41482=CARTESIAN_POINT('Ctrl Pts',(-86.51072,4.88092761120804,-3.85429840783599));
#41483=CARTESIAN_POINT('Ctrl Pts',(-86.4776907382611,5.52083048049534,-3.04395129593469));
#41484=CARTESIAN_POINT('Ctrl Pts',(-86.4116322147833,6.38855598297889,-1.09916744813806));
#41485=CARTESIAN_POINT('Ctrl Pts',(-86.3125444295668,6.13724916597635,2.08678167705531));
#41486=CARTESIAN_POINT('Ctrl Pts',(-86.2134566443499,4.39481025566226,4.7650088956501));
#41487=CARTESIAN_POINT('Ctrl Pts',(-86.1143688591334,1.5844221326576,6.28572095298091));
#41488=CARTESIAN_POINT('Ctrl Pts',(-86.0152810739166,-1.61092755177724,
6.27892628422283));
#41489=CARTESIAN_POINT('Ctrl Pts',(-85.9161932886999,-4.41485865379402,
4.7465110522202));
#41490=CARTESIAN_POINT('Ctrl Pts',(-85.8286811246477,-5.94378959897448,
2.37447606712619));
#41491=CARTESIAN_POINT('Ctrl Pts',(-85.7741982223342,-6.21841544098032,
0.670637576511123));
#41492=CARTESIAN_POINT('Ctrl Pts',(-85.7527445817596,-6.21890566139956,
-0.00012576145485773));
#41493=CARTESIAN_POINT('Ctrl Pts',(-86.9228037546341,5.44108552132573,-4.29663558492217));
#41494=CARTESIAN_POINT('Ctrl Pts',(-86.8897744928952,6.15442661434643,-3.39328927679633));
#41495=CARTESIAN_POINT('Ctrl Pts',(-86.8237159694174,7.12173632351047,-1.22531300686443));
#41496=CARTESIAN_POINT('Ctrl Pts',(-86.7246281842008,6.84158836961276,2.32627042923568));
#41497=CARTESIAN_POINT('Ctrl Pts',(-86.625540398984,4.89917908148197,5.31186343587118));
#41498=CARTESIAN_POINT('Ctrl Pts',(-86.5264526137675,1.76625777155052,7.00709946810573));
#41499=CARTESIAN_POINT('Ctrl Pts',(-86.4273648285506,-1.79580507560737,
6.99952501161989));
#41500=CARTESIAN_POINT('Ctrl Pts',(-86.3282770433341,-4.92152832684868,
5.29124269406165));
#41501=CARTESIAN_POINT('Ctrl Pts',(-86.2291892581174,-6.85137477063435,
2.29721389573782));
#41502=CARTESIAN_POINT('Ctrl Pts',(-86.1301014729007,-7.11642976004538,
-1.25498724546614));
#41503=CARTESIAN_POINT('Ctrl Pts',(-86.0310136876841,-5.65228184978238,
-4.50225302768583));
#41504=CARTESIAN_POINT('Ctrl Pts',(-85.9319259024674,-2.8147033238205,-6.65552420937686));
#41505=CARTESIAN_POINT('Ctrl Pts',(-85.8328381172507,0.706812370959138,
-7.19159127052686));
#41506=CARTESIAN_POINT('Ctrl Pts',(-85.7337503320341,4.05658150791202,-5.98019305530335));
#41507=CARTESIAN_POINT('Ctrl Pts',(-85.6346625468173,6.42065372437976,-3.31568558097902));
#41508=CARTESIAN_POINT('Ctrl Pts',(-85.5355747616008,7.22458973766228,0.154491077408247));
#41509=CARTESIAN_POINT('Ctrl Pts',(-85.4364869763839,6.2730435466505,3.58712824513611));
#41510=CARTESIAN_POINT('Ctrl Pts',(-85.3373991911675,3.79722857138034,6.14813953415812));
#41511=CARTESIAN_POINT('Ctrl Pts',(-85.2383114059506,0.398735978739728,
7.21523208383319));
#41512=CARTESIAN_POINT('Ctrl Pts',(-85.1392236207341,-3.09664432369599,
6.52911620558032));
#41513=CARTESIAN_POINT('Ctrl Pts',(-85.0401358355173,-5.83957994631889,
4.25650919220943));
#41514=CARTESIAN_POINT('Ctrl Pts',(-84.9410480503007,-7.16357287155185,
0.949625284159334));
#41515=CARTESIAN_POINT('Ctrl Pts',(-84.8419602650841,-6.74690987362332,
-2.58800533649108));
#41516=CARTESIAN_POINT('Ctrl Pts',(-84.7428724798672,-4.69083469401064,
-5.49678399941974));
#41517=CARTESIAN_POINT('Ctrl Pts',(-84.6437846946508,-1.49494711354703,
-7.06991496359203));
#41518=CARTESIAN_POINT('Ctrl Pts',(-84.544696909434,2.06419335672799,-6.92514766987085));
#41519=CARTESIAN_POINT('Ctrl Pts',(-84.4456091242173,5.12176143341354,-5.09765870604247));
#41520=CARTESIAN_POINT('Ctrl Pts',(-84.3465213390008,6.93480746310232,-2.0315043474144));
#41521=CARTESIAN_POINT('Ctrl Pts',(-84.2474335537839,7.06278461725108,1.52827939665304));
#41522=CARTESIAN_POINT('Ctrl Pts',(-84.1483457685673,5.47459609606395,4.71671093548111));
#41523=CARTESIAN_POINT('Ctrl Pts',(-84.0492579833507,2.5561512502798,6.75904248023308));
#41524=CARTESIAN_POINT('Ctrl Pts',(-83.9501701981339,-0.983405419582861,
7.15901377597882));
#41525=CARTESIAN_POINT('Ctrl Pts',(-83.8510824129173,-4.28400724125367,
5.81943695049585));
#41526=CARTESIAN_POINT('Ctrl Pts',(-83.7519946277006,-6.54365049222737,
3.06581191521701));
#41527=CARTESIAN_POINT('Ctrl Pts',(-83.652906842484,-7.21327097247888,-0.432765919991988));
#41528=CARTESIAN_POINT('Ctrl Pts',(-83.5538190572673,-6.13015953172498,
-3.82618721177028));
#41529=CARTESIAN_POINT('Ctrl Pts',(-83.4547312720506,-3.55749829683403,
-6.28989430212752));
#41530=CARTESIAN_POINT('Ctrl Pts',(-83.3556434868339,-0.120410805453714,
-7.22523810693066));
#41531=CARTESIAN_POINT('Ctrl Pts',(-83.2565557016174,3.34593496045394,-6.40494213122378));
#41532=CARTESIAN_POINT('Ctrl Pts',(-83.1574679164006,5.99926163513778,-4.02832772960159));
#41533=CARTESIAN_POINT('Ctrl Pts',(-83.058380131184,7.19484501825694,-0.67288158481008));
#41534=CARTESIAN_POINT('Ctrl Pts',(-82.9592923459673,6.64217374987331,2.84606611666121));
#41535=CARTESIAN_POINT('Ctrl Pts',(-82.8602045607506,4.4755398283902,5.67345641636614));
#41536=CARTESIAN_POINT('Ctrl Pts',(-82.7611167755339,1.22140738496329,7.12226989546663));
#41537=CARTESIAN_POINT('Ctrl Pts',(-82.6620289903173,-2.32951131817089,
6.84046354294992));
#41538=CARTESIAN_POINT('Ctrl Pts',(-82.5629412051006,-5.31438878103006,
4.89651267209378));
#41539=CARTESIAN_POINT('Ctrl Pts',(-82.463853419884,-7.00793823296552,1.76277230147661));
#41540=CARTESIAN_POINT('Ctrl Pts',(-82.3647656346673,-6.99864897438848,
-1.79929902940124));
#41541=CARTESIAN_POINT('Ctrl Pts',(-82.2656778494506,-5.28877817546381,
-4.92416387569006));
#41542=CARTESIAN_POINT('Ctrl Pts',(-82.1665900642339,-2.29380241283818,
-6.85252033596187));
#41543=CARTESIAN_POINT('Ctrl Pts',(-82.0675022790173,1.25853778608825,-7.11580263251456));
#41544=CARTESIAN_POINT('Ctrl Pts',(-81.9684144938005,4.50506951616823,-5.6500365590326));
#41545=CARTESIAN_POINT('Ctrl Pts',(-81.8693267085839,6.65692739059195,-2.81138438857082));
#41546=CARTESIAN_POINT('Ctrl Pts',(-81.7702389233673,7.19123766728605,0.710397970520364));
#41547=CARTESIAN_POINT('Ctrl Pts',(-81.6711511381505,5.97816983229143,4.0595627745108));
#41548=CARTESIAN_POINT('Ctrl Pts',(-81.5720633529339,3.31248374210761,6.42230612180593));
#41549=CARTESIAN_POINT('Ctrl Pts',(-81.4729755677172,-0.158093224178774,
7.22451181716674));
#41550=CARTESIAN_POINT('Ctrl Pts',(-81.3738877825005,-3.59025557363318,
6.27125421107364));
#41551=CARTESIAN_POINT('Ctrl Pts',(-81.2747999972839,-6.15003207033319,
3.79416262142076));
#41552=CARTESIAN_POINT('Ctrl Pts',(-81.1757122120672,-7.21543000202332,
0.395138393243329));
#41553=CARTESIAN_POINT('Ctrl Pts',(-81.0766244268506,-6.52757139634248,
-3.09989937410306));
#41554=CARTESIAN_POINT('Ctrl Pts',(-80.9775366416338,-4.25359703309988,
-5.84170152814375));
#41555=CARTESIAN_POINT('Ctrl Pts',(-80.8784488564172,-0.946053387980383,
-7.16404546684372));
#41556=CARTESIAN_POINT('Ctrl Pts',(-80.7793610712005,2.59136904284052,-6.74561864825762));
#41557=CARTESIAN_POINT('Ctrl Pts',(-80.6802732859838,5.49912217968629,-4.68809339889848));
#41558=CARTESIAN_POINT('Ctrl Pts',(-80.5811855007673,7.07065946957171,-1.49142184819354));
#41559=CARTESIAN_POINT('Ctrl Pts',(-80.4820977155504,6.92411759645864,2.06764599830945));
#41560=CARTESIAN_POINT('Ctrl Pts',(-80.383009930334,5.09510434768085,5.12430250377131));
#41561=CARTESIAN_POINT('Ctrl Pts',(-80.2839221451171,2.02804638034109,6.93581951488781));
#41562=CARTESIAN_POINT('Ctrl Pts',(-80.1848343599005,-1.53180073101746,
7.06202173491186));
#41563=CARTESIAN_POINT('Ctrl Pts',(-80.0857465746839,-4.71943999823467,
5.47224365018372));
#41564=CARTESIAN_POINT('Ctrl Pts',(-79.9866587894672,-6.76031614429142,
2.5527808549004));
#41565=CARTESIAN_POINT('Ctrl Pts',(-79.8875710042505,-7.15852255738009,
-0.986974801802736));
#41566=CARTESIAN_POINT('Ctrl Pts',(-79.7884832190338,-5.81730020903324,
-4.2869082964177));
#41567=CARTESIAN_POINT('Ctrl Pts',(-79.6893954338172,-3.06254885153835,
-6.54517830130352));
#41568=CARTESIAN_POINT('Ctrl Pts',(-79.5903076486005,0.436362423448914,
-7.21305429754379));
#41569=CARTESIAN_POINT('Ctrl Pts',(-79.4912198633838,3.82924325099778,-6.1282510219965));
#41570=CARTESIAN_POINT('Ctrl Pts',(-79.3921320781672,6.29166729896275,-3.55436169558977));
#41571=CARTESIAN_POINT('Ctrl Pts',(-79.2930442929505,7.22529724598348,-0.116808266388605));
#41572=CARTESIAN_POINT('Ctrl Pts',(-79.1939565077338,6.40327304246616,3.34912806675697));
#41573=CARTESIAN_POINT('Ctrl Pts',(-79.0948687225171,4.02533598009955,6.00126942498245));
#41574=CARTESIAN_POINT('Ctrl Pts',(-78.9957809373005,0.669294131151232,
7.19517962457642));
#41575=CARTESIAN_POINT('Ctrl Pts',(-78.8966931520838,-2.84937756945328,
6.64075386764256));
#41576=CARTESIAN_POINT('Ctrl Pts',(-78.7976053668671,-5.67568722792293,
4.47271047069959));
#41577=CARTESIAN_POINT('Ctrl Pts',(-78.6985175816505,-7.12287800731837,
1.21785604928229));
#41578=CARTESIAN_POINT('Ctrl Pts',(-78.5994297964338,-6.83930119175066,
-2.33292170302204));
#41579=CARTESIAN_POINT('Ctrl Pts',(-78.500342011217,-4.89386229421091,-5.31682953546696));
#41580=CARTESIAN_POINT('Ctrl Pts',(-78.4012542260005,-1.75927790459205,
-7.00881628510317));
#41581=CARTESIAN_POINT('Ctrl Pts',(-78.3021664407838,1.8027883518613,-6.99775096886895));
#41582=CARTESIAN_POINT('Ctrl Pts',(-78.2030786555671,4.92680026331916,-5.28632231605976));
#41583=CARTESIAN_POINT('Ctrl Pts',(-78.1039908703505,6.85366318052953,-2.29038544174708));
#41584=CARTESIAN_POINT('Ctrl Pts',(-78.0049030851337,7.11517423751361,1.26208558891056));
#41585=CARTESIAN_POINT('Ctrl Pts',(-77.9058152999171,5.64778961635293,4.50788608034069));
#41586=CARTESIAN_POINT('Ctrl Pts',(-77.8067275147004,2.80806487633721,6.65832832730517));
#41587=CARTESIAN_POINT('Ctrl Pts',(-77.7076397294838,-0.713983453598893,
7.19088256696632));
#41588=CARTESIAN_POINT('Ctrl Pts',(-77.6085519442671,-4.06254300223632,
5.97614497974186));
#41589=CARTESIAN_POINT('Ctrl Pts',(-77.5094641590504,-6.42395693723408,
3.30928115041248));
#41590=CARTESIAN_POINT('Ctrl Pts',(-77.4103763738338,-7.22443209341518,
-0.161695366495079));
#41591=CARTESIAN_POINT('Ctrl Pts',(-77.3112885886171,-6.26946331998695,
-3.59338199239259));
#41592=CARTESIAN_POINT('Ctrl Pts',(-77.2122008034004,-3.79109572646178,
-6.15192308605336));
#41593=CARTESIAN_POINT('Ctrl Pts',(-77.1131130181837,-0.391540710377681,
-7.21562612224539));
#41594=CARTESIAN_POINT('Ctrl Pts',(-77.014025232967,3.10315365428635,-6.52602496637903));
#41595=CARTESIAN_POINT('Ctrl Pts',(-76.9149374477504,5.84382165748359,-4.25068381551004));
#41596=CARTESIAN_POINT('Ctrl Pts',(-76.8158496625337,7.16451628122316,-0.942481257108831));
#41597=CARTESIAN_POINT('Ctrl Pts',(-76.7167618773171,6.74432574584776,2.59473210521012));
#41598=CARTESIAN_POINT('Ctrl Pts',(-76.6176740921004,4.68535093832905,5.50145899272296));
#41599=CARTESIAN_POINT('Ctrl Pts',(-76.5185863068837,1.487896212053,7.07140221781165));
#41600=CARTESIAN_POINT('Ctrl Pts',(-76.4194985216671,-2.07109812585812,
6.92308580164801));
#41601=CARTESIAN_POINT('Ctrl Pts',(-76.3204107364503,-5.12684230020594,
5.0925487226665));
#41602=CARTESIAN_POINT('Ctrl Pts',(-76.2213229512338,-6.93682984239387,
2.02458790907854));
#41603=CARTESIAN_POINT('Ctrl Pts',(-76.122235166017,-7.06125709692096,-1.53532168456533));
#41604=CARTESIAN_POINT('Ctrl Pts',(-76.0231473808003,-5.46988984387717,
-4.72216788771455));
#41605=CARTESIAN_POINT('Ctrl Pts',(-75.9240595955837,-2.54940982488769,
-6.76158812770189));
#41606=CARTESIAN_POINT('Ctrl Pts',(-75.824971810367,0.990543938655987,-7.15802955913882));
#41607=CARTESIAN_POINT('Ctrl Pts',(-75.7258840251504,4.28980828583576,-5.81516202136175));
#41608=CARTESIAN_POINT('Ctrl Pts',(-75.6267962399337,6.54670448321702,-3.05928502649549));
#41609=CARTESIAN_POINT('Ctrl Pts',(-75.527708454717,7.21283582940884,0.439958818424079));
#41610=CARTESIAN_POINT('Ctrl Pts',(-75.4286206695004,6.1263409887555,3.83229833825699));
#41611=CARTESIAN_POINT('Ctrl Pts',(-75.3295328842836,3.55122421071421,6.29343873165936));
#41612=CARTESIAN_POINT('Ctrl Pts',(-75.2304450990671,0.113205698284411,
7.2253545887928));
#41613=CARTESIAN_POINT('Ctrl Pts',(-75.1313573138503,-3.35232034045075,
6.40160236182422));
#41614=CARTESIAN_POINT('Ctrl Pts',(-75.0322695286337,-6.00327572288282,
4.02234322987969));
#41615=CARTESIAN_POINT('Ctrl Pts',(-74.9331817434169,-7.1955124421398,0.665706511102669));
#41616=CARTESIAN_POINT('Ctrl Pts',(-74.8340939582003,-6.63933233448859,
-2.85268831387646));
#41617=CARTESIAN_POINT('Ctrl Pts',(-74.7350061729836,-4.46988000107174,
-5.6779166284767));
#41618=CARTESIAN_POINT('Ctrl Pts',(-74.635918387767,-1.21430441083646,-7.12348434838852));
#41619=CARTESIAN_POINT('Ctrl Pts',(-74.5368306025503,2.33633150789764,-6.83813714026838));
#41620=CARTESIAN_POINT('Ctrl Pts',(-74.4377428173337,5.31926896811458,-4.89121069969046));
#41621=CARTESIAN_POINT('Ctrl Pts',(-74.3386550321169,7.00969259481552,-1.75578307034256));
#41622=CARTESIAN_POINT('Ctrl Pts',(-74.2395672469003,6.99685122367504,1.80627722613956));
#41623=CARTESIAN_POINT('Ctrl Pts',(-74.1404794616836,5.28386514245066,4.92943542612214));
#41624=CARTESIAN_POINT('Ctrl Pts',(-74.041391676467,2.28696790125519,6.85480432124371));
#41625=CARTESIAN_POINT('Ctrl Pts',(-73.9423038912502,-1.26563307797238,
7.11454407364629));
#41626=CARTESIAN_POINT('Ctrl Pts',(-73.8432161060337,-4.51070152383107,
5.64554126960569));
#41627=CARTESIAN_POINT('Ctrl Pts',(-73.7441283208169,-6.65972760872605,
2.80474466600528));
#41628=CARTESIAN_POINT('Ctrl Pts',(-73.6450405356003,-7.19052567895877,
-0.717568759177671));
#41629=CARTESIAN_POINT('Ctrl Pts',(-73.5459527503836,-5.97411864149405,
-4.0655222199942));
#41630=CARTESIAN_POINT('Ctrl Pts',(-73.446864965167,-3.30607773601422,-6.42560615563577));
#41631=CARTESIAN_POINT('Ctrl Pts',(-73.3477771799502,0.165297468613132,
-7.2243505736352));
#41632=CARTESIAN_POINT('Ctrl Pts',(-73.2486893947336,3.59650751781999,-6.26767087028167));
#41633=CARTESIAN_POINT('Ctrl Pts',(-73.1496016095169,6.15381257237603,-3.78802788901824));
#41634=CARTESIAN_POINT('Ctrl Pts',(-73.0505138243002,7.21582044862827,-0.387942930173093));
#41635=CARTESIAN_POINT('Ctrl Pts',(-72.9514260390835,6.52447691401449,3.10640716301083));
#41636=CARTESIAN_POINT('Ctrl Pts',(-72.8523382538669,4.24776954117984,5.84594033402139));
#41637=CARTESIAN_POINT('Ctrl Pts',(-72.7532504686502,0.938908891931892,
7.16498531446955));
#41638=CARTESIAN_POINT('Ctrl Pts',(-72.6541626834336,-2.59809452251698,
6.74303116676621));
#41639=CARTESIAN_POINT('Ctrl Pts',(-72.5550748982169,-5.50379443807064,
4.68260731295887));
#41640=CARTESIAN_POINT('Ctrl Pts',(-72.4559871130002,-7.07214320806714,
1.48437020601429));
#41641=CARTESIAN_POINT('Ctrl Pts',(-72.3568993277835,-6.9220522857251,-2.07454973852188));
#41642=CARTESIAN_POINT('Ctrl Pts',(-72.2578115425669,-5.08999183162014,
-5.12938082208305));
#41643=CARTESIAN_POINT('Ctrl Pts',(-72.1587237573501,-2.02112893449372,
-6.93783844537082));
#41644=CARTESIAN_POINT('Ctrl Pts',(-72.0596359721336,1.5388422564249,-7.06049070346774));
#41645=CARTESIAN_POINT('Ctrl Pts',(-71.9605481869168,4.72489460324093,-5.46753467772979));
#41646=CARTESIAN_POINT('Ctrl Pts',(-71.8614604017002,6.76285843014922,-2.54603816107944));
#41647=CARTESIAN_POINT('Ctrl Pts',(-71.7623726164835,7.15753478137712,0.994112829255322));
#41648=CARTESIAN_POINT('Ctrl Pts',(-71.6632848312669,5.81302238801313,4.29270720878692));
#41649=CARTESIAN_POINT('Ctrl Pts',(-71.5641970460502,3.05602044089978,6.5482290375884));
#41650=CARTESIAN_POINT('Ctrl Pts',(-71.4651092608335,-0.443555104023324,
7.21261556812839));
#41651=CARTESIAN_POINT('Ctrl Pts',(-71.3660214756168,-3.83535247278855,
6.12442943247679));
#41652=CARTESIAN_POINT('Ctrl Pts',(-71.2669336904002,-6.29520859977706,
3.5480858429872));
#41653=CARTESIAN_POINT('Ctrl Pts',(-71.1678459051835,-7.22541013534436,
0.109603102036615));
#41654=CARTESIAN_POINT('Ctrl Pts',(-71.0687581199668,-6.39993008971324,
-3.35551178074168));
#41655=CARTESIAN_POINT('Ctrl Pts',(-70.9696703347502,-4.01934947968604,
-6.0052805283401));
#41656=CARTESIAN_POINT('Ctrl Pts',(-70.8705825495335,-0.662118725556255,
-7.19584347086433));
#41657=CARTESIAN_POINT('Ctrl Pts',(-70.7714947643167,2.85599834910767,-6.63790915076483));
#41658=CARTESIAN_POINT('Ctrl Pts',(-70.6724069791002,5.68014461747322,-4.46704842021029));
#41659=CARTESIAN_POINT('Ctrl Pts',(-70.5733191938834,7.12408891852638,-1.21075247050868));
#41660=CARTESIAN_POINT('Ctrl Pts',(-70.4742314086668,6.83697138879244,2.33974073195018));
#41661=CARTESIAN_POINT('Ctrl Pts',(-70.3751436234501,4.88855788919152,5.32170707836653));
#41662=CARTESIAN_POINT('Ctrl Pts',(-70.2760558382335,1.75228779959694,7.01056716188476));
#41663=CARTESIAN_POINT('Ctrl Pts',(-70.1769680530168,-1.80976565136866,
6.99594973903039));
#41664=CARTESIAN_POINT('Ctrl Pts',(-70.0778802678002,-4.93206936344387,
5.28140665524739));
#41665=CARTESIAN_POINT('Ctrl Pts',(-69.9787924825834,-6.85594375782075,
2.2835497922121));
#41666=CARTESIAN_POINT('Ctrl Pts',(-69.8797046973668,-7.1139121410692,-1.26918025239179));
#41667=CARTESIAN_POINT('Ctrl Pts',(-69.7806169121502,-5.64329151934991,
-4.51351584593945));
#41668=CARTESIAN_POINT('Ctrl Pts',(-69.6815291269334,-2.80142375840029,
-6.66112523450688));
#41669=CARTESIAN_POINT('Ctrl Pts',(-69.5824413417168,0.721153886365357,
-7.19016700335191));
#41670=CARTESIAN_POINT('Ctrl Pts',(-69.4833535565001,4.06850042704398,-5.97209081805211));
#41671=CARTESIAN_POINT('Ctrl Pts',(-69.3842657712834,6.42725377660052,-3.3028734997085));
#41672=CARTESIAN_POINT('Ctrl Pts',(-69.2851779860668,7.22426725784799,0.168899529635844));
#41673=CARTESIAN_POINT('Ctrl Pts',(-69.1860902008501,6.26587686240158,3.59963214914153));
#41674=CARTESIAN_POINT('Ctrl Pts',(-69.0870024156334,3.78495910985655,6.15570052882507));
#41675=CARTESIAN_POINT('Ctrl Pts',(-68.9879146304168,0.384345053516504,
7.21601298113648));
#41676=CARTESIAN_POINT('Ctrl Pts',(-68.8888268452,-3.10965989945231,6.52292723960769));
#41677=CARTESIAN_POINT('Ctrl Pts',(-68.7897390599835,-5.84805755726145,
4.24485421088667));
#41678=CARTESIAN_POINT('Ctrl Pts',(-68.6906512747667,-7.16545256640336,
0.935336293230516));
#41679=CARTESIAN_POINT('Ctrl Pts',(-68.5915634895501,-6.74173491146246,
-2.60145629370749));
#41680=CARTESIAN_POINT('Ctrl Pts',(-68.4924757043334,-4.6798625232114,-5.50612851558968));
#41681=CARTESIAN_POINT('Ctrl Pts',(-68.3933879191167,-1.48084383147897,
-7.0728824392594));
#41682=CARTESIAN_POINT('Ctrl Pts',(-68.2943001339001,2.07800083650708,-6.92101705076112));
#41683=CARTESIAN_POINT('Ctrl Pts',(-68.1952123486835,5.13191806661274,-5.08743367149795));
#41684=CARTESIAN_POINT('Ctrl Pts',(-68.0961245634667,6.9388453279461,-2.01766946490889));
#41685=CARTESIAN_POINT('Ctrl Pts',(-67.9970367782501,7.0597225458634,1.54236246085508));
#41686=CARTESIAN_POINT('Ctrl Pts',(-67.8979489930334,5.46517817033512,4.72762011344252));
#41687=CARTESIAN_POINT('Ctrl Pts',(-67.7988612078167,2.54266582779222,6.76412711356621));
#41688=CARTESIAN_POINT('Ctrl Pts',(-67.6997734226,-0.997681398644423,7.15703809797258));
#41689=CARTESIAN_POINT('Ctrl Pts',(-67.6006856373834,-4.29560521476863,
5.8108815655554));
#41690=CARTESIAN_POINT('Ctrl Pts',(-67.5015978521667,-6.54975165938407,
3.0527545763004));
#41691=CARTESIAN_POINT('Ctrl Pts',(-67.4025100669501,-7.21239413162189,
-0.447150226246016));
#41692=CARTESIAN_POINT('Ctrl Pts',(-67.3034222817333,-6.12251510055504,
-3.83840778962029));
#41693=CARTESIAN_POINT('Ctrl Pts',(-67.2043344965167,-3.54494913454001,
-6.29697257132185));
#41694=CARTESIAN_POINT('Ctrl Pts',(-67.1052467113,-0.105995324468443,-7.22547267039505));
#41695=CARTESIAN_POINT('Ctrl Pts',(-67.0061589260834,3.3586919338921,-6.39823840999051));
#41696=CARTESIAN_POINT('Ctrl Pts',(-66.9070711408666,6.00730504114269,-4.01639086919487));
#41697=CARTESIAN_POINT('Ctrl Pts',(-66.8079833556501,7.19612970031069,-0.658457417060504));
#41698=CARTESIAN_POINT('Ctrl Pts',(-66.7088955704333,6.63657172317509,2.85915744447726));
#41699=CARTESIAN_POINT('Ctrl Pts',(-66.6098077852167,4.4640346981544,5.68268549543904));
#41700=CARTESIAN_POINT('Ctrl Pts',(-66.5437492617389,2.29307521661488,6.64328120120947));
#41701=CARTESIAN_POINT('Ctrl Pts',(-66.51072,1.15821195975198,6.83557123116185));
#41702=CARTESIAN_POINT('Ctrl Pts',(-86.7854425030894,5.25436621795317,-4.14918985922678));
#41703=CARTESIAN_POINT('Ctrl Pts',(-86.7524132413505,5.94322790306273,-3.27684328317578));
#41704=CARTESIAN_POINT('Ctrl Pts',(-86.6863547178727,6.87734287666661,-1.18326448728897));
#41705=CARTESIAN_POINT('Ctrl Pts',(-86.587266932656,6.60680863506729,2.24644084517556));
#41706=CARTESIAN_POINT('Ctrl Pts',(-86.4881791474394,4.73105613954207,5.12957858913082));
#41707=CARTESIAN_POINT('Ctrl Pts',(-86.3890913622228,1.70564589191955,6.76663996306412));
#41708=CARTESIAN_POINT('Ctrl Pts',(-86.290003577006,-1.73417923433066,6.75932543582087));
#41709=CARTESIAN_POINT('Ctrl Pts',(-86.1909157917894,-4.75263843583045,
5.1096654801145));
#41710=CARTESIAN_POINT('Ctrl Pts',(-86.0918280065727,-6.6162592005329,2.2183814317692));
#41711=CARTESIAN_POINT('Ctrl Pts',(-85.992740221356,-6.87221841617152,-1.21192040828883));
#41712=CARTESIAN_POINT('Ctrl Pts',(-85.8936524361393,-5.45831501626719,
-4.34775121997823));
#41713=CARTESIAN_POINT('Ctrl Pts',(-85.7945646509228,-2.71811240611401,
-6.42712955557415));
#41714=CARTESIAN_POINT('Ctrl Pts',(-85.6954768657059,0.682557006289124,
-6.94480064264385));
#41715=CARTESIAN_POINT('Ctrl Pts',(-85.5963890804895,3.91737361083659,-5.77497343930147));
#41716=CARTESIAN_POINT('Ctrl Pts',(-85.4973012952726,6.20031901618341,-3.20190267875179));
#41717=CARTESIAN_POINT('Ctrl Pts',(-85.3982135100561,6.97666671611046,0.149189476057238));
#41718=CARTESIAN_POINT('Ctrl Pts',(-85.2991257248392,6.05777431104196,3.4640303661532));
#41719=CARTESIAN_POINT('Ctrl Pts',(-85.2000379396228,3.66692077327355,5.93715657379921));
#41720=CARTESIAN_POINT('Ctrl Pts',(-85.1009501544059,0.385052734120952,
6.96763018471131));
#41721=CARTESIAN_POINT('Ctrl Pts',(-85.0018623691894,-2.99037816253259,
6.30505943882551));
#41722=CARTESIAN_POINT('Ctrl Pts',(-84.9027745839727,-5.63918568761968,
4.11044046602357));
#41723=CARTESIAN_POINT('Ctrl Pts',(-84.8036867987559,-6.91774373856132,
0.917037417119129));
#41724=CARTESIAN_POINT('Ctrl Pts',(-84.7045990135394,-6.51537917876785,
-2.49919391243608));
#41725=CARTESIAN_POINT('Ctrl Pts',(-84.6055112283226,-4.52986141342742,
-5.30815331623375));
#41726=CARTESIAN_POINT('Ctrl Pts',(-84.506423443106,-1.44364568067551,-6.82729984722759));
#41727=CARTESIAN_POINT('Ctrl Pts',(-84.4073356578893,1.993357354595,-6.68750046811258));
#41728=CARTESIAN_POINT('Ctrl Pts',(-84.3082478726727,4.94600023224528,-4.92272462741185));
#41729=CARTESIAN_POINT('Ctrl Pts',(-84.209160087456,6.69682877053108,-1.96179011942424));
#41730=CARTESIAN_POINT('Ctrl Pts',(-84.1100723022392,6.82041418979961,1.47583411469907));
#41731=CARTESIAN_POINT('Ctrl Pts',(-84.0109845170227,5.28672682525449,4.55484967146845));
#41732=CARTESIAN_POINT('Ctrl Pts',(-83.9118967318059,2.46843294868416,6.52709543613163));
#41733=CARTESIAN_POINT('Ctrl Pts',(-83.8128089465894,-0.949658334712104,
6.91334109543625));
#41734=CARTESIAN_POINT('Ctrl Pts',(-83.7137211613725,-4.13699487679171,
5.61973392999406));
#41735=CARTESIAN_POINT('Ctrl Pts',(-83.614633376156,-6.31909495884465,2.96060381605423));
#41736=CARTESIAN_POINT('Ctrl Pts',(-83.5155455909392,-6.96573637194007,
-0.417914885067527));
#41737=CARTESIAN_POINT('Ctrl Pts',(-83.4164578057226,-5.91979358308471,
-3.69488565292608));
#41738=CARTESIAN_POINT('Ctrl Pts',(-83.3173700205059,-3.43541721556255,
-6.07404680666412));
#41739=CARTESIAN_POINT('Ctrl Pts',(-83.2182822352893,-0.11627872158463,
-6.97729283558003));
#41740=CARTESIAN_POINT('Ctrl Pts',(-83.1191944500726,3.23111400377219,-6.18514659075735));
#41741=CARTESIAN_POINT('Ctrl Pts',(-83.0201066648558,5.79338765119243,-3.89008940482619));
#41742=CARTESIAN_POINT('Ctrl Pts',(-82.9210188796393,6.9479427329653,-0.649790607784323));
#41743=CARTESIAN_POINT('Ctrl Pts',(-82.8219310944226,6.41423723783079,2.74839893599067));
#41744=CARTESIAN_POINT('Ctrl Pts',(-82.7228433092059,4.32195472562018,5.47876294470015));
#41745=CARTESIAN_POINT('Ctrl Pts',(-82.6237555239893,1.17949289287146,6.87785813827209));
#41746=CARTESIAN_POINT('Ctrl Pts',(-82.5246677387725,-2.24957051797165,
6.60572240857901));
#41747=CARTESIAN_POINT('Ctrl Pts',(-82.425579953556,-5.132017273147,4.72848123213478));
#41748=CARTESIAN_POINT('Ctrl Pts',(-82.3264921683392,-6.76744994440458,
1.70228003116653));
#41749=CARTESIAN_POINT('Ctrl Pts',(-82.2274043831225,-6.75847946116814,
-1.7375532876716));
#41750=CARTESIAN_POINT('Ctrl Pts',(-82.1283165979059,-5.10728553530141,
-4.75518354171855));
#41751=CARTESIAN_POINT('Ctrl Pts',(-82.0292288126892,-2.21508701920563,
-6.61736545400635));
#41752=CARTESIAN_POINT('Ctrl Pts',(-81.9301410274726,1.21534910659308,-6.87161280949628));
#41753=CARTESIAN_POINT('Ctrl Pts',(-81.8310532422559,4.35047105628243,-5.45614677615795));
#41754=CARTESIAN_POINT('Ctrl Pts',(-81.7319654570392,6.42848458444576,-2.71490736528399));
#41755=CARTESIAN_POINT('Ctrl Pts',(-81.6328776718226,6.94445917384764,0.68601956043053));
#41756=CARTESIAN_POINT('Ctrl Pts',(-81.5337898866059,5.77301964633066,3.92025257064009));
#41757=CARTESIAN_POINT('Ctrl Pts',(-81.4347021013892,3.19881071595589,6.20191470902461));
#41758=CARTESIAN_POINT('Ctrl Pts',(-81.3356143161725,-0.152668009564746,
6.97659146957779));
#41759=CARTESIAN_POINT('Ctrl Pts',(-81.2365265309558,-3.46705037551403,
6.05604637929548));
#41760=CARTESIAN_POINT('Ctrl Pts',(-81.1374387457392,-5.93898416465503,
3.66396003615034));
#41761=CARTESIAN_POINT('Ctrl Pts',(-81.0383509605224,-6.96782131103125,
0.38157860536036));
#41762=CARTESIAN_POINT('Ctrl Pts',(-80.9392631753059,-6.30356764211681,
-2.99352151082763));
#41763=CARTESIAN_POINT('Ctrl Pts',(-80.8401753900891,-4.10762824217843,
-5.64123446406796));
#41764=CARTESIAN_POINT('Ctrl Pts',(-80.7410876048726,-0.913588096107144,
-6.91820011601149));
#41765=CARTESIAN_POINT('Ctrl Pts',(-80.6419998196559,2.502442187976,-6.51413226380673));
#41766=CARTESIAN_POINT('Ctrl Pts',(-80.5429120344391,5.31041125821166,-4.52721419011613));
#41767=CARTESIAN_POINT('Ctrl Pts',(-80.4438242492226,6.82801880432787,-1.44024139027976));
#41768=CARTESIAN_POINT('Ctrl Pts',(-80.3447364640057,6.6865057432699,1.99669151341629));
#41769=CARTESIAN_POINT('Ctrl Pts',(-80.2456486787892,4.92025792582607,4.94845410182571));
#41770=CARTESIAN_POINT('Ctrl Pts',(-80.1465608935724,1.95845081786362,6.69780609218714));
#41771=CARTESIAN_POINT('Ctrl Pts',(-80.0474731083559,-1.47923460900375,
6.81967748695314));
#41772=CARTESIAN_POINT('Ctrl Pts',(-79.9483853231391,-4.55748508219353,
5.28445510720959));
#41773=CARTESIAN_POINT('Ctrl Pts',(-79.8492975379226,-6.52832539242893,
2.46517821365873));
#41774=CARTESIAN_POINT('Ctrl Pts',(-79.7502097527057,-6.91286673376692,
-0.953105228035428));
#41775=CARTESIAN_POINT('Ctrl Pts',(-79.6511219674892,-5.61767051413456,
-4.13979637774047));
#41776=CARTESIAN_POINT('Ctrl Pts',(-79.5520341822724,-2.95745272947546,
-6.32057033877863));
#41777=CARTESIAN_POINT('Ctrl Pts',(-79.4529463970558,0.421387968920513,
-6.96552713254201));
#41778=CARTESIAN_POINT('Ctrl Pts',(-79.3538586118391,3.69783681941937,-5.91795056683278));
#41779=CARTESIAN_POINT('Ctrl Pts',(-79.2547708266225,6.07575896035828,-3.43238825166325));
#41780=CARTESIAN_POINT('Ctrl Pts',(-79.1556830414058,6.97734994518436,-0.112799809244738));
#41781=CARTESIAN_POINT('Ctrl Pts',(-79.0565952561891,6.18353477937369,3.23419753367137));
#41782=CARTESIAN_POINT('Ctrl Pts',(-78.9575074709724,3.88720032185653,5.79532654060911));
#41783=CARTESIAN_POINT('Ctrl Pts',(-78.8584196857559,0.646326263171543,
6.94826585674906));
#41784=CARTESIAN_POINT('Ctrl Pts',(-78.759331900539,-2.75159675113525,6.41286608106483));
#41785=CARTESIAN_POINT('Ctrl Pts',(-78.6602441153225,-5.48091720249239,
4.31922246173463));
#41786=CARTESIAN_POINT('Ctrl Pts',(-78.5611563301058,-6.87844538182083,
1.17606342679199));
#41787=CARTESIAN_POINT('Ctrl Pts',(-78.4620685448891,-6.60459994526706,
-2.25286387016798));
#41788=CARTESIAN_POINT('Ctrl Pts',(-78.3629807596724,-4.7259218060868,-5.13437426930324));
#41789=CARTESIAN_POINT('Ctrl Pts',(-78.2638929744557,-1.69890554994023,
-6.76829786481892));
#41790=CARTESIAN_POINT('Ctrl Pts',(-78.1648051892391,1.74092286861015,-6.75761227210323));
#41791=CARTESIAN_POINT('Ctrl Pts',(-78.0657174040224,4.75772945761006,-5.10491395252843));
#41792=CARTESIAN_POINT('Ctrl Pts',(-77.9666296188058,6.61846908008706,-2.2117873067864));
#41793=CARTESIAN_POINT('Ctrl Pts',(-77.867541833589,6.87100597884612,1.2187751610494));
#41794=CARTESIAN_POINT('Ctrl Pts',(-77.7684540483724,5.45397694080736,4.35319096567927));
#41795=CARTESIAN_POINT('Ctrl Pts',(-77.6693662631557,2.71170176727014,6.42983744583905));
#41796=CARTESIAN_POINT('Ctrl Pts',(-77.5702784779391,-0.689482002086527,
6.94411625934709));
#41797=CARTESIAN_POINT('Ctrl Pts',(-77.4711906927224,-3.9231305272209,5.77106427974229));
#41798=CARTESIAN_POINT('Ctrl Pts',(-77.3721029075058,-6.2035088741565,3.19571802617058));
#41799=CARTESIAN_POINT('Ctrl Pts',(-77.273015122289,-6.97651448167062,-0.15614653877089));
#41800=CARTESIAN_POINT('Ctrl Pts',(-77.1739273370724,-6.0543169454189,-3.47006950635624));
#41801=CARTESIAN_POINT('Ctrl Pts',(-77.0748395518556,-3.66099838645685,
-5.94081028723273));
#41802=CARTESIAN_POINT('Ctrl Pts',(-76.975751766639,-0.3781043825719,-6.96801070108319));
#41803=CARTESIAN_POINT('Ctrl Pts',(-76.8766639814224,2.99666411533033,-6.30207428030022));
#41804=CARTESIAN_POINT('Ctrl Pts',(-76.7775761962057,5.64328183787549,-4.10481499617639));
#41805=CARTESIAN_POINT('Ctrl Pts',(-76.678488410989,6.918654773664,-0.910138548456401));
#41806=CARTESIAN_POINT('Ctrl Pts',(-76.5794006257724,6.51288372935182,2.50568984163527));
#41807=CARTESIAN_POINT('Ctrl Pts',(-76.4803128405557,4.52456584134205,5.31266787987831));
#41808=CARTESIAN_POINT('Ctrl Pts',(-76.381225055339,1.4368367418211,6.82873606400796));
#41809=CARTESIAN_POINT('Ctrl Pts',(-76.2821372701224,-2.00002517584462,
6.68550935610128));
#41810=CARTESIAN_POINT('Ctrl Pts',(-76.1830494849056,-4.95090674119966,
4.91779000105471));
#41811=CARTESIAN_POINT('Ctrl Pts',(-76.083961699689,-6.6987817487351,1.9551110294158));
#41812=CARTESIAN_POINT('Ctrl Pts',(-75.9848739144723,-6.81893908870291,
-1.48263473556018));
#41813=CARTESIAN_POINT('Ctrl Pts',(-75.8857861292556,-5.2821820754235,-4.56011935990765));
#41814=CARTESIAN_POINT('Ctrl Pts',(-75.786698344039,-2.46192286577841,-6.52955372575242));
#41815=CARTESIAN_POINT('Ctrl Pts',(-75.6876105588223,0.956551884412262,
-6.91239065352628));
#41816=CARTESIAN_POINT('Ctrl Pts',(-75.5885227736057,4.14259684951599,-5.61560570169507));
#41817=CARTESIAN_POINT('Ctrl Pts',(-75.489434988389,6.32204414738856,-2.95430090765989));
#41818=CARTESIAN_POINT('Ctrl Pts',(-75.3903472031723,6.96531616148055,0.424860948014456));
#41819=CARTESIAN_POINT('Ctrl Pts',(-75.2912594179557,5.91610607935003,3.70078706661266));
#41820=CARTESIAN_POINT('Ctrl Pts',(-75.1921716327389,3.42935843445585,6.07746960358966));
#41821=CARTESIAN_POINT('Ctrl Pts',(-75.0930838475223,0.10932086886228,6.9774053201861));
#41822=CARTESIAN_POINT('Ctrl Pts',(-74.9939960623056,-3.23728025953358,
6.18192143073367));
#41823=CARTESIAN_POINT('Ctrl Pts',(-74.894908277089,-5.79726398927988,3.88431027251025));
#41824=CARTESIAN_POINT('Ctrl Pts',(-74.7958204918722,-6.94858725316066,
0.642861757878953));
#41825=CARTESIAN_POINT('Ctrl Pts',(-74.6967327066556,-6.41149333002965,
-2.7547938822197));
#41826=CARTESIAN_POINT('Ctrl Pts',(-74.597644921439,-4.3164891240697,-5.48307009770239));
#41827=CARTESIAN_POINT('Ctrl Pts',(-74.4985571362222,-1.17263366833754,
-6.87903091535509));
#41828=CARTESIAN_POINT('Ctrl Pts',(-74.3994693510056,2.25615666229153,-6.60347584001997));
#41829=CARTESIAN_POINT('Ctrl Pts',(-74.3003815657889,5.13672998902946,-4.72336120515205));
#41830=CARTESIAN_POINT('Ctrl Pts',(-74.2012937805723,6.76914410260199,-1.69553064635787));
#41831=CARTESIAN_POINT('Ctrl Pts',(-74.1022059953556,6.75674340306355,1.74429201674696));
#41832=CARTESIAN_POINT('Ctrl Pts',(-74.0031182101389,5.1025411006494,4.76027419070725));
#41833=CARTESIAN_POINT('Ctrl Pts',(-73.9040304249223,2.20848704450624,6.61957106078467));
#41834=CARTESIAN_POINT('Ctrl Pts',(-73.8049426397056,-1.22220091251239,
6.87039744003096));
#41835=CARTESIAN_POINT('Ctrl Pts',(-73.7058548544889,-4.35590979285198,
5.45180574957198));
#41836=CARTESIAN_POINT('Ctrl Pts',(-73.6067670692723,-6.43118870874393,
2.70849549511429));
#41837=CARTESIAN_POINT('Ctrl Pts',(-73.5076792840555,-6.94377161850602,
-0.692944272333947));
#41838=CARTESIAN_POINT('Ctrl Pts',(-73.408591498839,-5.76910747843973,-3.92600750849266));
#41839=CARTESIAN_POINT('Ctrl Pts',(-73.3095037136222,-3.19262454191448,
-6.20510149706638));
#41840=CARTESIAN_POINT('Ctrl Pts',(-73.2104159284056,0.159625029158248,
-6.97643575936854));
#41841=CARTESIAN_POINT('Ctrl Pts',(-73.1113281431889,3.47308777452254,-6.05258600641015));
#41842=CARTESIAN_POINT('Ctrl Pts',(-73.0122403579722,5.94263493289657,-3.65803582662163));
#41843=CARTESIAN_POINT('Ctrl Pts',(-72.9131525727555,6.96819835885431,-0.374630065784826));
#41844=CARTESIAN_POINT('Ctrl Pts',(-72.8140647875388,6.30057935175775,2.99980597484801));
#41845=CARTESIAN_POINT('Ctrl Pts',(-72.7149770023223,4.10200072969768,5.64532780873616));
#41846=CARTESIAN_POINT('Ctrl Pts',(-72.6158892171055,0.906688774540824,
6.91910771130582));
#41847=CARTESIAN_POINT('Ctrl Pts',(-72.5168014318889,-2.50893687236812,
6.51163357576282));
#41848=CARTESIAN_POINT('Ctrl Pts',(-72.4177136466722,-5.31492318079035,
4.52191636773916));
#41849=CARTESIAN_POINT('Ctrl Pts',(-72.3186258614555,-6.82945162603157,
1.4334317361579));
#41850=CARTESIAN_POINT('Ctrl Pts',(-72.2195380762388,-6.68451130688302,
-2.00335834105711));
#41851=CARTESIAN_POINT('Ctrl Pts',(-72.1204502910222,-4.9153208536972,-4.9533581497545));
#41852=CARTESIAN_POINT('Ctrl Pts',(-72.0213625058055,-1.95177075491801,
-6.69975573993386));
#41853=CARTESIAN_POINT('Ctrl Pts',(-71.9222747205888,1.48603449352654,-6.81819899523176));
#41854=CARTESIAN_POINT('Ctrl Pts',(-71.8231869353722,4.56275250395429,-5.27990773046166));
#41855=CARTESIAN_POINT('Ctrl Pts',(-71.7240991501555,6.53078043579762,-2.45866690585223));
#41856=CARTESIAN_POINT('Ctrl Pts',(-71.6250113649389,6.91191285483219,0.959998302985763));
#41857=CARTESIAN_POINT('Ctrl Pts',(-71.5259235797221,5.61353949318912,4.14539629142208));
#41858=CARTESIAN_POINT('Ctrl Pts',(-71.4268357945055,2.95114835139102,6.32351638430802));
#41859=CARTESIAN_POINT('Ctrl Pts',(-71.3277480092889,-0.428333821485886,
6.96510345880816));
#41860=CARTESIAN_POINT('Ctrl Pts',(-71.2286602240721,-3.70373639377261,
5.91426012109497));
#41861=CARTESIAN_POINT('Ctrl Pts',(-71.1295724388556,-6.0791787359331,3.42632776469341));
#41862=CARTESIAN_POINT('Ctrl Pts',(-71.0304846536388,-6.97745896057144,
0.105841901302007));
#41863=CARTESIAN_POINT('Ctrl Pts',(-70.9313968684222,-6.18030654523836,
-3.24036218059244));
#41864=CARTESIAN_POINT('Ctrl Pts',(-70.8323090832054,-3.88141925750582,
-5.79919999672307));
#41865=CARTESIAN_POINT('Ctrl Pts',(-70.7332212979888,-0.639397092767843,
-6.94890692212019));
#41866=CARTESIAN_POINT('Ctrl Pts',(-70.6341335127721,2.75799032844922,-6.41011898506654));
#41867=CARTESIAN_POINT('Ctrl Pts',(-70.5350457275555,5.4852216297949,-4.31375471330489));
#41868=CARTESIAN_POINT('Ctrl Pts',(-70.4359579423388,6.87961473872937,-1.16920361836068));
#41869=CARTESIAN_POINT('Ctrl Pts',(-70.3368701571221,6.60235009311713,2.25944889352386));
#41870=CARTESIAN_POINT('Ctrl Pts',(-70.2377823719054,4.720799429967,5.13908443174007));
#41871=CARTESIAN_POINT('Ctrl Pts',(-70.1386945866888,1.69215532125842,6.76998865754343));
#41872=CARTESIAN_POINT('Ctrl Pts',(-70.0396068014721,-1.74766073124442,
6.75587285426512));
#41873=CARTESIAN_POINT('Ctrl Pts',(-69.9405190162555,-4.76281774037749,
5.1001669802542));
#41874=CARTESIAN_POINT('Ctrl Pts',(-69.8414312310387,-6.62067139582524,
2.20518623318563));
#41875=CARTESIAN_POINT('Ctrl Pts',(-69.7423434458221,-6.86978719320209,
-1.22562636013042));
#41876=CARTESIAN_POINT('Ctrl Pts',(-69.6432556606054,-5.4496332029916,-4.35862753712465));
#41877=CARTESIAN_POINT('Ctrl Pts',(-69.5441678753888,-2.7052885496134,-6.43253837282463));
#41878=CARTESIAN_POINT('Ctrl Pts',(-69.4450800901721,0.696406370312047,
-6.94342525140987));
#41879=CARTESIAN_POINT('Ctrl Pts',(-69.3459923049554,3.92888351374035,-5.7671492429098));
#41880=CARTESIAN_POINT('Ctrl Pts',(-69.2469045197387,6.20669257735784,-3.18953026395594));
#41881=CARTESIAN_POINT('Ctrl Pts',(-69.1478167345221,6.97635530269203,0.163103479860511));
#41882=CARTESIAN_POINT('Ctrl Pts',(-69.0487289493054,6.05085356269778,3.47610517926561));
#41883=CARTESIAN_POINT('Ctrl Pts',(-68.9496411640888,3.65507235738477,5.94445810118679));
#41884=CARTESIAN_POINT('Ctrl Pts',(-68.850553378872,0.371155655855663,6.96838428431038));
#41885=CARTESIAN_POINT('Ctrl Pts',(-68.7514655936554,-3.00294708858478,
6.29908285683592));
#41886=CARTESIAN_POINT('Ctrl Pts',(-68.6523778084387,-5.64737237617125,
4.09918544349301));
#41887=CARTESIAN_POINT('Ctrl Pts',(-68.5532900232221,-6.91955892876356,
0.903238775114562));
#41888=CARTESIAN_POINT('Ctrl Pts',(-68.4542022380054,-6.51038180347379,
-2.51218327915711));
#41889=CARTESIAN_POINT('Ctrl Pts',(-68.3551144527887,-4.5192657697164,-5.31717716081293));
#41890=CARTESIAN_POINT('Ctrl Pts',(-68.2560266675721,-1.43002637464361,
-6.83016548935693));
#41891=CARTESIAN_POINT('Ctrl Pts',(-68.1569388823553,2.00669100925305,-6.68351159761526));
#41892=CARTESIAN_POINT('Ctrl Pts',(-68.0578510971388,4.95580832479609,-4.91285048081417));
#41893=CARTESIAN_POINT('Ctrl Pts',(-67.958763311922,6.70072806976919,-1.94843000240689));
#41894=CARTESIAN_POINT('Ctrl Pts',(-67.8596755267054,6.81745719814908,1.48943389667244));
#41895=CARTESIAN_POINT('Ctrl Pts',(-67.7605877414887,5.27763209027949,4.56538448403874));
#41896=CARTESIAN_POINT('Ctrl Pts',(-67.661499956272,2.45541029942128,6.53200558237203));
#41897=CARTESIAN_POINT('Ctrl Pts',(-67.5624121710554,-0.963444411371859,
6.91143321589037));
#41898=CARTESIAN_POINT('Ctrl Pts',(-67.4633243858387,-4.14819484782596,
5.61147213638018));
#41899=CARTESIAN_POINT('Ctrl Pts',(-67.364236600622,-6.3249867549711,2.94799456000949));
#41900=CARTESIAN_POINT('Ctrl Pts',(-67.2651488154053,-6.96488962123942,
-0.43180557150384));
#41901=CARTESIAN_POINT('Ctrl Pts',(-67.1660610301887,-5.91241148244737,
-3.70668686266028));
#41902=CARTESIAN_POINT('Ctrl Pts',(-67.0669732449719,-3.42329869727003,
-6.08088217405369));
#41903=CARTESIAN_POINT('Ctrl Pts',(-66.9678854597554,-0.102357930226421,
-6.97751934963469));
#41904=CARTESIAN_POINT('Ctrl Pts',(-66.8687976745387,3.24343320184657,-6.17867291813365));
#41905=CARTESIAN_POINT('Ctrl Pts',(-66.769709889322,5.8011550352234,-3.87856217633039));
#41906=CARTESIAN_POINT('Ctrl Pts',(-66.6706221041053,6.94918332915839,-0.635861427761624));
#41907=CARTESIAN_POINT('Ctrl Pts',(-66.5715343188886,6.40882745338248,2.76104101455297));
#41908=CARTESIAN_POINT('Ctrl Pts',(-66.472446533672,4.31084441180371,5.48767531358562));
#41909=CARTESIAN_POINT('Ctrl Pts',(-66.4063880101942,2.21438477785055,6.41530668525375));
#41910=CARTESIAN_POINT('Ctrl Pts',(-66.3733587484553,1.11846611686177,6.60099798407104));
#41911=CARTESIAN_POINT('Ctrl Pts',(-86.6480812515447,5.0676469145806,-4.00174413353138));
#41912=CARTESIAN_POINT('Ctrl Pts',(-86.6150519898058,5.73202919177904,-3.16039728955523));
#41913=CARTESIAN_POINT('Ctrl Pts',(-86.548993466328,6.63294942982275,-1.14121596771352));
#41914=CARTESIAN_POINT('Ctrl Pts',(-86.4499056811114,6.37202890052182,2.16661126111543));
#41915=CARTESIAN_POINT('Ctrl Pts',(-86.3508178958946,4.56293319760216,4.94729374239046));
#41916=CARTESIAN_POINT('Ctrl Pts',(-86.2517301106781,1.64503401228858,6.52618045802251));
#41917=CARTESIAN_POINT('Ctrl Pts',(-86.1526423254613,-1.67255339305395,
6.51912586002186));
#41918=CARTESIAN_POINT('Ctrl Pts',(-86.0535545402447,-4.58374854481224,
4.92808826616734));
#41919=CARTESIAN_POINT('Ctrl Pts',(-85.954466755028,-6.38114363043145,2.13954896780058));
#41920=CARTESIAN_POINT('Ctrl Pts',(-85.8553789698114,-6.62800707229765,
-1.16885357111151));
#41921=CARTESIAN_POINT('Ctrl Pts',(-85.7562911845946,-5.264348182752,-4.19324941227064));
#41922=CARTESIAN_POINT('Ctrl Pts',(-85.657203399378,-2.62152148840752,-6.19873490177144));
#41923=CARTESIAN_POINT('Ctrl Pts',(-85.5581156141612,0.658301641619111,
-6.69801001476086));
#41924=CARTESIAN_POINT('Ctrl Pts',(-85.4590278289447,3.77816571376116,-5.56975382329959));
#41925=CARTESIAN_POINT('Ctrl Pts',(-85.3599400437279,5.97998430798706,-3.08811977652457));
#41926=CARTESIAN_POINT('Ctrl Pts',(-85.2608522585114,6.72874369455863,0.14388787470623));
#41927=CARTESIAN_POINT('Ctrl Pts',(-85.1617644732945,5.84250507543342,3.34093248717029));
#41928=CARTESIAN_POINT('Ctrl Pts',(-85.0626766880781,3.53661297516676,5.7261736134403));
#41929=CARTESIAN_POINT('Ctrl Pts',(-84.9635889028612,0.371369489502175,
6.72002828558944));
#41930=CARTESIAN_POINT('Ctrl Pts',(-84.8645011176447,-2.88411200136919,
6.08100267207071));
#41931=CARTESIAN_POINT('Ctrl Pts',(-84.7654133324279,-5.43879142892048,
3.9643717398377));
#41932=CARTESIAN_POINT('Ctrl Pts',(-84.6663255472113,-6.67191460557079,
0.884449550078927));
#41933=CARTESIAN_POINT('Ctrl Pts',(-84.5672377619947,-6.28384848391239,
-2.41038248838107));
#41934=CARTESIAN_POINT('Ctrl Pts',(-84.4681499767779,-4.3688881328442,-5.11952263304775));
#41935=CARTESIAN_POINT('Ctrl Pts',(-84.3690621915613,-1.392344247804,-6.58468473086316));
#41936=CARTESIAN_POINT('Ctrl Pts',(-84.2699744063445,1.922521352462,-6.44985326635431));
#41937=CARTESIAN_POINT('Ctrl Pts',(-84.170886621128,4.77023903107702,-4.74779054878123));
#41938=CARTESIAN_POINT('Ctrl Pts',(-84.0717988359113,6.45885007795985,-1.89207589143408));
#41939=CARTESIAN_POINT('Ctrl Pts',(-83.9727110506945,6.57804376234814,1.4233888327451));
#41940=CARTESIAN_POINT('Ctrl Pts',(-83.873623265478,5.09885755444503,4.39298840745579));
#41941=CARTESIAN_POINT('Ctrl Pts',(-83.7745354802612,2.38071464708853,6.29514839203017));
#41942=CARTESIAN_POINT('Ctrl Pts',(-83.6754476950446,-0.915911249841352,
6.66766841489367));
#41943=CARTESIAN_POINT('Ctrl Pts',(-83.5763599098279,-3.98998251232974,
5.42003090949228));
#41944=CARTESIAN_POINT('Ctrl Pts',(-83.4772721246113,-6.09453942546194,
2.85539571689145));
#41945=CARTESIAN_POINT('Ctrl Pts',(-83.3781843393945,-6.71820177140126,
-0.403063850143066));
#41946=CARTESIAN_POINT('Ctrl Pts',(-83.2790965541779,-5.70942763444443,
-3.56358409408187));
#41947=CARTESIAN_POINT('Ctrl Pts',(-83.1800087689612,-3.31333613429106,
-5.85819931120072));
#41948=CARTESIAN_POINT('Ctrl Pts',(-83.0809209837446,-0.112146637715546,
-6.7293475642294));
#41949=CARTESIAN_POINT('Ctrl Pts',(-82.981833198528,3.11629304709045,-5.96535105029092));
#41950=CARTESIAN_POINT('Ctrl Pts',(-82.8827454133112,5.58751366724708,-3.75185108005079));
#41951=CARTESIAN_POINT('Ctrl Pts',(-82.7836576280946,6.70104044767366,-0.626699630758572));
#41952=CARTESIAN_POINT('Ctrl Pts',(-82.6845698428779,6.18630072578829,2.65073175532014));
#41953=CARTESIAN_POINT('Ctrl Pts',(-82.5854820576612,4.16836962285014,5.28406947303415));
#41954=CARTESIAN_POINT('Ctrl Pts',(-82.4863942724445,1.13757840077963,6.63344638107755));
#41955=CARTESIAN_POINT('Ctrl Pts',(-82.3873064872278,-2.16962971777241,
6.37098127420809));
#41956=CARTESIAN_POINT('Ctrl Pts',(-82.2882187020112,-4.94964576526393,
4.56044979217578));
#41957=CARTESIAN_POINT('Ctrl Pts',(-82.1891309167946,-6.52696165584364,
1.64178776085645));
#41958=CARTESIAN_POINT('Ctrl Pts',(-82.0900431315779,-6.5183099479478,-1.67580754594197));
#41959=CARTESIAN_POINT('Ctrl Pts',(-81.9909553463612,-4.92579289513902,
-4.58620320774704));
#41960=CARTESIAN_POINT('Ctrl Pts',(-81.8918675611445,-2.13637162557306,
-6.38221057205085));
#41961=CARTESIAN_POINT('Ctrl Pts',(-81.7927797759279,1.17216042709791,-6.62742298647799));
#41962=CARTESIAN_POINT('Ctrl Pts',(-81.6936919907112,4.19587259639663,-5.26225699328331));
#41963=CARTESIAN_POINT('Ctrl Pts',(-81.5946042054945,6.20004177829955,-2.61843034199716));
#41964=CARTESIAN_POINT('Ctrl Pts',(-81.4955164202779,6.69768068040923,0.661641150340698));
#41965=CARTESIAN_POINT('Ctrl Pts',(-81.3964286350611,5.56786946036987,3.7809423667694));
#41966=CARTESIAN_POINT('Ctrl Pts',(-81.2973408498445,3.08513768980417,5.98152329624329));
#41967=CARTESIAN_POINT('Ctrl Pts',(-81.1982530646279,-0.147242794950722,
6.72867112198883));
#41968=CARTESIAN_POINT('Ctrl Pts',(-81.0991652794111,-3.34384517739488,
5.84083854751732));
#41969=CARTESIAN_POINT('Ctrl Pts',(-81.0000774941945,-5.72793625897687,
3.53375745087992));
#41970=CARTESIAN_POINT('Ctrl Pts',(-80.9009897089778,-6.72021262003917,
0.368018817477388));
#41971=CARTESIAN_POINT('Ctrl Pts',(-80.8019019237612,-6.07956388789115,
-2.8871436475522));
#41972=CARTESIAN_POINT('Ctrl Pts',(-80.7028141385445,-3.96165945125696,
-5.44076739999217));
#41973=CARTESIAN_POINT('Ctrl Pts',(-80.6037263533278,-0.881122804233911,
-6.67235476517926));
#41974=CARTESIAN_POINT('Ctrl Pts',(-80.5046385681112,2.41351533311149,-6.28264587935584));
#41975=CARTESIAN_POINT('Ctrl Pts',(-80.4055507828944,5.12170033673702,-4.36633498133378));
#41976=CARTESIAN_POINT('Ctrl Pts',(-80.3064629976779,6.58537813908403,-1.38906093236599));
#41977=CARTESIAN_POINT('Ctrl Pts',(-80.2073752124611,6.44889389008117,1.92573702852313));
#41978=CARTESIAN_POINT('Ctrl Pts',(-80.1082874272445,4.7454115039713,4.77260569988011));
#41979=CARTESIAN_POINT('Ctrl Pts',(-80.0091996420278,1.88885525538614,6.45979266948648));
#41980=CARTESIAN_POINT('Ctrl Pts',(-79.9101118568112,-1.42666848699003,
6.57733323899442));
#41981=CARTESIAN_POINT('Ctrl Pts',(-79.8110240715944,-4.39553016615239,
5.09666656423546));
#41982=CARTESIAN_POINT('Ctrl Pts',(-79.7119362863778,-6.29633464056644,
2.37757557241705));
#41983=CARTESIAN_POINT('Ctrl Pts',(-79.612848501161,-6.66721091015377,-0.919235654268119));
#41984=CARTESIAN_POINT('Ctrl Pts',(-79.5137607159445,-5.41804081923588,
-3.99268445906324));
#41985=CARTESIAN_POINT('Ctrl Pts',(-79.4146729307277,-2.85235660741258,
-6.09596237625374));
#41986=CARTESIAN_POINT('Ctrl Pts',(-79.3155851455112,0.406413514392112,
-6.71799996754024));
#41987=CARTESIAN_POINT('Ctrl Pts',(-79.2164973602944,3.56643038784096,-5.70765011166905));
#41988=CARTESIAN_POINT('Ctrl Pts',(-79.1174095750778,5.85985062175381,-3.31041480773674));
#41989=CARTESIAN_POINT('Ctrl Pts',(-79.018321789861,6.72940264438526,-0.108791352100868));
#41990=CARTESIAN_POINT('Ctrl Pts',(-78.9192340046445,5.96379651628121,3.11926700058577));
#41991=CARTESIAN_POINT('Ctrl Pts',(-78.8201462194277,3.74906466361352,5.58938365623578));
#41992=CARTESIAN_POINT('Ctrl Pts',(-78.7210584342111,0.623358395191846,
6.7013520889217));
#41993=CARTESIAN_POINT('Ctrl Pts',(-78.6219706489944,-2.65381593281721,
6.18497829448711));
#41994=CARTESIAN_POINT('Ctrl Pts',(-78.5228828637778,-5.28614717706186,
4.16573445276967));
#41995=CARTESIAN_POINT('Ctrl Pts',(-78.423795078561,-6.63401275632328,1.1342708043017));
#41996=CARTESIAN_POINT('Ctrl Pts',(-78.3247072933444,-6.36989869878348,
-2.17280603731392));
#41997=CARTESIAN_POINT('Ctrl Pts',(-78.2256195081277,-4.55798131796269,
-4.95191900313952));
#41998=CARTESIAN_POINT('Ctrl Pts',(-78.126531722911,-1.63853319528842,-6.52777944453465));
#41999=CARTESIAN_POINT('Ctrl Pts',(-78.0274439376944,1.67905738535901,-6.51747357533751));
#42000=CARTESIAN_POINT('Ctrl Pts',(-77.9283561524777,4.58865865190096,-4.92350558899711));
#42001=CARTESIAN_POINT('Ctrl Pts',(-77.8292683672611,6.38327497964459,-2.1331891718257));
#42002=CARTESIAN_POINT('Ctrl Pts',(-77.7301805820443,6.62683772017861,1.17546473318823));
#42003=CARTESIAN_POINT('Ctrl Pts',(-77.6310927968278,5.26016426526179,4.19849585101786));
#42004=CARTESIAN_POINT('Ctrl Pts',(-77.532005011611,2.61533865820306,6.20134656437292));
#42005=CARTESIAN_POINT('Ctrl Pts',(-77.4329172263944,-0.664980550574156,
6.69734995172787));
#42006=CARTESIAN_POINT('Ctrl Pts',(-77.3338294411777,-3.78371805220548,
5.56598357974272));
#42007=CARTESIAN_POINT('Ctrl Pts',(-77.2347416559611,-5.98306081107892,
3.08215490192868));
#42008=CARTESIAN_POINT('Ctrl Pts',(-77.1356538707443,-6.72859686992606,
-0.150597711046703));
#42009=CARTESIAN_POINT('Ctrl Pts',(-77.0365660855277,-5.83917057085085,
-3.3467570203199));
#42010=CARTESIAN_POINT('Ctrl Pts',(-76.937478300311,-3.53090104645192,-5.7296974884121));
#42011=CARTESIAN_POINT('Ctrl Pts',(-76.8383905150944,-0.364668054766116,
-6.72039527992099));
#42012=CARTESIAN_POINT('Ctrl Pts',(-76.7393027298777,2.89017457637429,-6.07812359422141));
#42013=CARTESIAN_POINT('Ctrl Pts',(-76.640214944661,5.4427420182674,-3.95894617684274));
#42014=CARTESIAN_POINT('Ctrl Pts',(-76.5411271594444,6.67279326610485,-0.877795839803971));
#42015=CARTESIAN_POINT('Ctrl Pts',(-76.4420393742276,6.28144171285588,2.41664757806042));
#42016=CARTESIAN_POINT('Ctrl Pts',(-76.342951589011,4.36378074435504,5.12387676703367));
#42017=CARTESIAN_POINT('Ctrl Pts',(-76.2438638037943,1.3857772715892,6.58606991020427));
#42018=CARTESIAN_POINT('Ctrl Pts',(-76.1447760185777,-1.92895222583112,
6.44793291055455));
#42019=CARTESIAN_POINT('Ctrl Pts',(-76.0456882333609,-4.77497118219338,
4.74303127944292));
#42020=CARTESIAN_POINT('Ctrl Pts',(-75.9466004481443,-6.46073365507635,
1.88563414975306));
#42021=CARTESIAN_POINT('Ctrl Pts',(-75.8475126629276,-6.57662108048484,
-1.42994778655504));
#42022=CARTESIAN_POINT('Ctrl Pts',(-75.7484248777109,-5.09447430696985,
-4.39807083210074));
#42023=CARTESIAN_POINT('Ctrl Pts',(-75.6493370924943,-2.37443590666912,
-6.29751932380295));
#42024=CARTESIAN_POINT('Ctrl Pts',(-75.5502493072776,0.922559830168535,
-6.66675174791372));
#42025=CARTESIAN_POINT('Ctrl Pts',(-75.451161522061,3.99538541319622,-5.41604938202839));
#42026=CARTESIAN_POINT('Ctrl Pts',(-75.3520737368442,6.09738381156011,-2.84931678882429));
#42027=CARTESIAN_POINT('Ctrl Pts',(-75.2529859516277,6.71779649355226,0.409763077604835));
#42028=CARTESIAN_POINT('Ctrl Pts',(-75.1538981664109,5.70587116994455,3.56927579496832));
#42029=CARTESIAN_POINT('Ctrl Pts',(-75.0548103811943,3.30749265819749,5.86150047551997));
#42030=CARTESIAN_POINT('Ctrl Pts',(-74.9557225959776,0.105436039440141,
6.72945605157939));
#42031=CARTESIAN_POINT('Ctrl Pts',(-74.856634810761,-3.12224017861639,5.96224049964313));
#42032=CARTESIAN_POINT('Ctrl Pts',(-74.7575470255443,-5.59125225567696,
3.7462773151408));
#42033=CARTESIAN_POINT('Ctrl Pts',(-74.6584592403276,-6.7016620641815,0.620017004655243));
#42034=CARTESIAN_POINT('Ctrl Pts',(-74.5593714551108,-6.18365432557073,
-2.65689945056294));
#42035=CARTESIAN_POINT('Ctrl Pts',(-74.4602836698943,-4.16309824706767,
-5.28822356692807));
#42036=CARTESIAN_POINT('Ctrl Pts',(-74.3611958846775,-1.13096292583862,
-6.63457748232167));
#42037=CARTESIAN_POINT('Ctrl Pts',(-74.2621080994609,2.17598181668543,-6.36881453977156));
#42038=CARTESIAN_POINT('Ctrl Pts',(-74.1630203142442,4.95419100994433,-4.55551171061364));
#42039=CARTESIAN_POINT('Ctrl Pts',(-74.0639325290275,6.52859561038844,-1.63527822237319));
#42040=CARTESIAN_POINT('Ctrl Pts',(-73.9648447438109,6.51663558245208,1.68230680735436));
#42041=CARTESIAN_POINT('Ctrl Pts',(-73.8657569585942,4.92121705884814,4.59111295529236));
#42042=CARTESIAN_POINT('Ctrl Pts',(-73.7666691733775,2.13000618775729,6.38433780032563));
#42043=CARTESIAN_POINT('Ctrl Pts',(-73.6675813881609,-1.1787687470524,6.62625080641564));
#42044=CARTESIAN_POINT('Ctrl Pts',(-73.5684936029442,-4.20111806187289,
5.25807022953826));
#42045=CARTESIAN_POINT('Ctrl Pts',(-73.4694058177275,-6.20264980876182,
2.6122463242233));
#42046=CARTESIAN_POINT('Ctrl Pts',(-73.3703180325109,-6.69701755805326,
-0.668319785490224));
#42047=CARTESIAN_POINT('Ctrl Pts',(-73.2712302472942,-5.56409631538542,
-3.78649279699112));
#42048=CARTESIAN_POINT('Ctrl Pts',(-73.1721424620775,-3.07917134781474,
-5.98459683849698));
#42049=CARTESIAN_POINT('Ctrl Pts',(-73.0730546768609,0.153952589703362,
-6.7285209451019));
#42050=CARTESIAN_POINT('Ctrl Pts',(-72.9739668916442,3.34966803122509,-5.83750114253862));
#42051=CARTESIAN_POINT('Ctrl Pts',(-72.8748791064275,5.73145729341713,-3.52804376422502));
#42052=CARTESIAN_POINT('Ctrl Pts',(-72.7757913212109,6.72057626908036,-0.36131720139656));
#42053=CARTESIAN_POINT('Ctrl Pts',(-72.6767035359942,6.076681789501,2.89320478668518));
#42054=CARTESIAN_POINT('Ctrl Pts',(-72.5776157507775,3.95623191821552,5.44471528345093));
#42055=CARTESIAN_POINT('Ctrl Pts',(-72.4785279655609,0.874468657149755,
6.67323010814208));
#42056=CARTESIAN_POINT('Ctrl Pts',(-72.3794401803441,-2.41977922221927,
6.28023598475943));
#42057=CARTESIAN_POINT('Ctrl Pts',(-72.2803523951276,-5.12605192351007,
4.36122542251945));
#42058=CARTESIAN_POINT('Ctrl Pts',(-72.1812646099108,-6.586760043996,1.3824932663015));
#42059=CARTESIAN_POINT('Ctrl Pts',(-72.0821768246942,-6.44697032804094,
-1.93216694359235));
#42060=CARTESIAN_POINT('Ctrl Pts',(-71.9830890394775,-4.74064987577426,
-4.77733547742596));
#42061=CARTESIAN_POINT('Ctrl Pts',(-71.8840012542608,-1.88241257534229,
-6.4616730344969));
#42062=CARTESIAN_POINT('Ctrl Pts',(-71.7849134690441,1.43322673062819,-6.57590728699578));
#42063=CARTESIAN_POINT('Ctrl Pts',(-71.6858256838275,4.40061040466765,-5.09228078319352));
#42064=CARTESIAN_POINT('Ctrl Pts',(-71.5867378986108,6.29870244144603,-2.37129565062501));
#42065=CARTESIAN_POINT('Ctrl Pts',(-71.4876501133941,6.66629092828726,0.925883776716208));
#42066=CARTESIAN_POINT('Ctrl Pts',(-71.3885623281775,5.41405659836511,3.99808537405724));
#42067=CARTESIAN_POINT('Ctrl Pts',(-71.2894745429607,2.84627626188227,6.09880373102764));
#42068=CARTESIAN_POINT('Ctrl Pts',(-71.1903867577442,-0.413112538948448,
6.71759134948792));
#42069=CARTESIAN_POINT('Ctrl Pts',(-71.0912989725275,-3.57212031475667,
5.70409080971315));
#42070=CARTESIAN_POINT('Ctrl Pts',(-70.9922111873108,-5.86314887208913,
3.30456968639962));
#42071=CARTESIAN_POINT('Ctrl Pts',(-70.8931234020941,-6.72950778579852,
0.102080700567402));
#42072=CARTESIAN_POINT('Ctrl Pts',(-70.7940356168774,-5.96068300076348,
-3.1252125804432));
#42073=CARTESIAN_POINT('Ctrl Pts',(-70.6949478316608,-3.74348903532561,
-5.59311946510605));
#42074=CARTESIAN_POINT('Ctrl Pts',(-70.5958600464441,-0.616675459979426,
-6.70197037337605));
#42075=CARTESIAN_POINT('Ctrl Pts',(-70.4967722612274,2.65998230779076,-6.18232881936826));
#42076=CARTESIAN_POINT('Ctrl Pts',(-70.3976844760109,5.2902986421166,-4.16046100639949));
#42077=CARTESIAN_POINT('Ctrl Pts',(-70.298596690794,6.63514055893235,-1.1276547662127));
#42078=CARTESIAN_POINT('Ctrl Pts',(-70.1995089055775,6.36772879744182,2.17915705509754));
#42079=CARTESIAN_POINT('Ctrl Pts',(-70.1004211203607,4.55304097074248,4.95646178511361));
#42080=CARTESIAN_POINT('Ctrl Pts',(-70.0013333351441,1.63202284291991,6.52941015320211));
#42081=CARTESIAN_POINT('Ctrl Pts',(-69.9022455499274,-1.68555581112019,
6.51579596949983));
#42082=CARTESIAN_POINT('Ctrl Pts',(-69.8031577647107,-4.5935661173111,4.91892730526103));
#42083=CARTESIAN_POINT('Ctrl Pts',(-69.704069979494,-6.38539903382975,2.12682267415914));
#42084=CARTESIAN_POINT('Ctrl Pts',(-69.6049821942774,-6.62566224533496,
-1.18207246786906));
#42085=CARTESIAN_POINT('Ctrl Pts',(-69.5058944090607,-5.2559748866333,-4.20373922830985));
#42086=CARTESIAN_POINT('Ctrl Pts',(-69.4068066238441,-2.6091533408265,-6.20395151114239));
#42087=CARTESIAN_POINT('Ctrl Pts',(-69.3077188386274,0.671658854258736,
-6.69668349946783));
#42088=CARTESIAN_POINT('Ctrl Pts',(-69.2086310534107,3.78926660043672,-5.56220766776749));
#42089=CARTESIAN_POINT('Ctrl Pts',(-69.109543268194,5.98613137811518,-3.07618702820339));
#42090=CARTESIAN_POINT('Ctrl Pts',(-69.0104554829774,6.72844334753605,0.157307430085179));
#42091=CARTESIAN_POINT('Ctrl Pts',(-68.9113676977607,5.83583026299398,3.35257820938968));
#42092=CARTESIAN_POINT('Ctrl Pts',(-68.8122799125441,3.52518560491299,5.7332156735485));
#42093=CARTESIAN_POINT('Ctrl Pts',(-68.7131921273274,0.357966258194822,
6.72075558748428));
#42094=CARTESIAN_POINT('Ctrl Pts',(-68.6141043421107,-2.89623427771726,
6.07523847406414));
#42095=CARTESIAN_POINT('Ctrl Pts',(-68.5150165568941,-5.44668719508104,
3.95351667609934));
#42096=CARTESIAN_POINT('Ctrl Pts',(-68.4159287716773,-6.67366529112376,
0.87114125699861));
#42097=CARTESIAN_POINT('Ctrl Pts',(-68.3168409864607,-6.2790286954851,-2.42291026460674));
#42098=CARTESIAN_POINT('Ctrl Pts',(-68.217753201244,-4.3586690162214,-5.12822580603616));
#42099=CARTESIAN_POINT('Ctrl Pts',(-68.1186654160274,-1.37920891780825,
-6.58744853945448));
#42100=CARTESIAN_POINT('Ctrl Pts',(-68.0195776308107,1.93538118199903,-6.44600614446938));
#42101=CARTESIAN_POINT('Ctrl Pts',(-67.920489845594,4.77969858297944,-4.73826729013039));
#42102=CARTESIAN_POINT('Ctrl Pts',(-67.8214020603773,6.4626108115923,-1.87919053990488));
#42103=CARTESIAN_POINT('Ctrl Pts',(-67.7223142751607,6.57519185043476,1.43650533248979));
#42104=CARTESIAN_POINT('Ctrl Pts',(-67.623226489944,5.09008601022387,4.40314885463497));
#42105=CARTESIAN_POINT('Ctrl Pts',(-67.5241387047273,2.36815477105034,6.29988405117785));
#42106=CARTESIAN_POINT('Ctrl Pts',(-67.4250509195107,-0.929207424099301,
6.66582833380815));
#42107=CARTESIAN_POINT('Ctrl Pts',(-67.325963134294,-4.00078448088328,5.41206270720496));
#42108=CARTESIAN_POINT('Ctrl Pts',(-67.2268753490773,-6.10022185055814,
2.84323454371856));
#42109=CARTESIAN_POINT('Ctrl Pts',(-67.1277875638607,-6.71738511085694,
-0.416460916761654));
#42110=CARTESIAN_POINT('Ctrl Pts',(-67.0286997786439,-5.7023078643397,-3.57496593570028));
#42111=CARTESIAN_POINT('Ctrl Pts',(-66.9296119934273,-3.30164826000004,
-5.86479177678551));
#42112=CARTESIAN_POINT('Ctrl Pts',(-66.8305242082106,-0.098720535984401,
-6.72956602887435));
#42113=CARTESIAN_POINT('Ctrl Pts',(-66.731436422994,3.12817446980103,-5.95910742627677));
#42114=CARTESIAN_POINT('Ctrl Pts',(-66.6323486377773,5.59500502930411,-3.74073348346592));
#42115=CARTESIAN_POINT('Ctrl Pts',(-66.5332608525606,6.70223695800609,-0.613265438462746));
#42116=CARTESIAN_POINT('Ctrl Pts',(-66.4341730673439,6.18108318358988,2.66292458462869));
#42117=CARTESIAN_POINT('Ctrl Pts',(-66.3350852821273,4.15765412545302,5.29266513173219));
#42118=CARTESIAN_POINT('Ctrl Pts',(-66.2690267586495,2.13569433908622,6.18733216929803));
#42119=CARTESIAN_POINT('Ctrl Pts',(-66.2359974969106,1.07872027397156,6.36642473698023));
#42120=CARTESIAN_POINT('Ctrl Pts',(-86.51072,4.88092761120804,-3.85429840783599));
#42121=CARTESIAN_POINT('Ctrl Pts',(-86.4776907382611,5.52083048049534,-3.04395129593469));
#42122=CARTESIAN_POINT('Ctrl Pts',(-86.4116322147833,6.38855598297889,-1.09916744813806));
#42123=CARTESIAN_POINT('Ctrl Pts',(-86.3125444295668,6.13724916597635,2.08678167705531));
#42124=CARTESIAN_POINT('Ctrl Pts',(-86.2134566443499,4.39481025566226,4.7650088956501));
#42125=CARTESIAN_POINT('Ctrl Pts',(-86.1143688591334,1.5844221326576,6.28572095298091));
#42126=CARTESIAN_POINT('Ctrl Pts',(-86.0152810739166,-1.61092755177724,
6.27892628422283));
#42127=CARTESIAN_POINT('Ctrl Pts',(-85.9161932886999,-4.41485865379402,
4.7465110522202));
#42128=CARTESIAN_POINT('Ctrl Pts',(-85.8171055034833,-6.14602806032999,
2.06071650383196));
#42129=CARTESIAN_POINT('Ctrl Pts',(-85.7180177182666,-6.38379572842379,
-1.12578673393419));
#42130=CARTESIAN_POINT('Ctrl Pts',(-85.6189299330499,-5.07038134923681,
-4.03874760456303));
#42131=CARTESIAN_POINT('Ctrl Pts',(-85.5198421478334,-2.52493057070103,
-5.97034024796873));
#42132=CARTESIAN_POINT('Ctrl Pts',(-85.4207543626165,0.634046276949095,
-6.45121938687785));
#42133=CARTESIAN_POINT('Ctrl Pts',(-85.3216665774001,3.63895781668574,-5.36453420729772));
#42134=CARTESIAN_POINT('Ctrl Pts',(-85.2225787921832,5.75964959979071,-2.97433687429733));
#42135=CARTESIAN_POINT('Ctrl Pts',(-85.1234910069667,6.48082067300681,0.138586273355216));
#42136=CARTESIAN_POINT('Ctrl Pts',(-85.0244032217499,5.62723583982488,3.21783460818738));
#42137=CARTESIAN_POINT('Ctrl Pts',(-84.9253154365333,3.40630517705998,5.51519065308138));
#42138=CARTESIAN_POINT('Ctrl Pts',(-84.8262276513165,0.357686244883394,
6.47242638646756));
#42139=CARTESIAN_POINT('Ctrl Pts',(-84.7271398660999,-2.77784584020579,
5.85694590531591));
#42140=CARTESIAN_POINT('Ctrl Pts',(-84.6280520808834,-5.23839717022127,
3.81830301365183));
#42141=CARTESIAN_POINT('Ctrl Pts',(-84.5289642956664,-6.42608547258025,
0.851861683038723));
#42142=CARTESIAN_POINT('Ctrl Pts',(-84.4298765104501,-6.05231778905693,
-2.32157106432606));
#42143=CARTESIAN_POINT('Ctrl Pts',(-84.3307887252331,-4.20791485226097,
-4.93089194986176));
#42144=CARTESIAN_POINT('Ctrl Pts',(-84.2317009400167,-1.34104281493249,
-6.34206961449874));
#42145=CARTESIAN_POINT('Ctrl Pts',(-84.1326131547998,1.85168535032901,-6.21220606459603));
#42146=CARTESIAN_POINT('Ctrl Pts',(-84.0335253695833,4.59447782990876,-4.57285647015062));
#42147=CARTESIAN_POINT('Ctrl Pts',(-83.9344375843666,6.22087138538862,-1.82236166344391));
#42148=CARTESIAN_POINT('Ctrl Pts',(-83.8353497991498,6.33567333489668,1.37094355079113));
#42149=CARTESIAN_POINT('Ctrl Pts',(-83.7362620139334,4.91098828363557,4.23112714344313));
#42150=CARTESIAN_POINT('Ctrl Pts',(-83.6371742287164,2.29299634549289,6.06320134792872));
#42151=CARTESIAN_POINT('Ctrl Pts',(-83.5380864435,-0.8821641649706,6.4219957343511));
#42152=CARTESIAN_POINT('Ctrl Pts',(-83.4389986582831,-3.84297014786777,
5.22032788899049));
#42153=CARTESIAN_POINT('Ctrl Pts',(-83.3399108730665,-5.86998389207923,
2.75018761772868));
#42154=CARTESIAN_POINT('Ctrl Pts',(-83.2408230878499,-6.47066717086244,
-0.388212815218607));
#42155=CARTESIAN_POINT('Ctrl Pts',(-83.1417353026332,-5.49906168580417,
-3.43228253523767));
#42156=CARTESIAN_POINT('Ctrl Pts',(-83.0426475174165,-3.19125505301957,
-5.64235181573731));
#42157=CARTESIAN_POINT('Ctrl Pts',(-82.9435597321999,-0.108014553846464,
-6.48140229287878));
#42158=CARTESIAN_POINT('Ctrl Pts',(-82.8444719469832,3.0014720904087,-5.7455555098245));
#42159=CARTESIAN_POINT('Ctrl Pts',(-82.7453841617665,5.38163968330173,-3.61361275527539));
#42160=CARTESIAN_POINT('Ctrl Pts',(-82.6462963765498,6.45413816238201,-0.603608653732817));
#42161=CARTESIAN_POINT('Ctrl Pts',(-82.5472085913332,5.95836421374577,2.5530645746496));
#42162=CARTESIAN_POINT('Ctrl Pts',(-82.4481208061165,4.01478452008011,5.08937600136816));
#42163=CARTESIAN_POINT('Ctrl Pts',(-82.3490330208998,1.0956639086878,6.38903462388301));
#42164=CARTESIAN_POINT('Ctrl Pts',(-82.2499452356833,-2.08968891757316,
6.13624013983718));
#42165=CARTESIAN_POINT('Ctrl Pts',(-82.1508574504665,-4.76727425738086,
4.39241835221678));
#42166=CARTESIAN_POINT('Ctrl Pts',(-82.0517696652499,-6.2864733672827,1.58129549054636));
#42167=CARTESIAN_POINT('Ctrl Pts',(-81.9526818800331,-6.27814043472745,
-1.61406180421233));
#42168=CARTESIAN_POINT('Ctrl Pts',(-81.8535940948165,-4.74430025497663,
-4.41722287377553));
#42169=CARTESIAN_POINT('Ctrl Pts',(-81.7545063095999,-2.0576562319405,-6.14705569009534));
#42170=CARTESIAN_POINT('Ctrl Pts',(-81.6554185243831,1.12897174760274,-6.3832331634597));
#42171=CARTESIAN_POINT('Ctrl Pts',(-81.5563307391665,4.04127413651083,-5.06836721040866));
#42172=CARTESIAN_POINT('Ctrl Pts',(-81.4572429539498,5.97159897215335,-2.52195331871032));
#42173=CARTESIAN_POINT('Ctrl Pts',(-81.3581551687331,6.45090218697082,0.637262740250864));
#42174=CARTESIAN_POINT('Ctrl Pts',(-81.2590673835165,5.36271927440909,3.64163216289869));
#42175=CARTESIAN_POINT('Ctrl Pts',(-81.1599795982997,2.97146466365244,5.76113188346196));
#42176=CARTESIAN_POINT('Ctrl Pts',(-81.0608918130833,-0.141817580336693,
6.48075077439986));
#42177=CARTESIAN_POINT('Ctrl Pts',(-80.9618040278663,-3.22063997927572,
5.62563071573915));
#42178=CARTESIAN_POINT('Ctrl Pts',(-80.8627162426499,-5.5168883532987,3.4035548656095));
#42179=CARTESIAN_POINT('Ctrl Pts',(-80.7636284574331,-6.47260392904711,
0.354459029594419));
#42180=CARTESIAN_POINT('Ctrl Pts',(-80.6645406722165,-5.85556013366548,
-2.78076578427677));
#42181=CARTESIAN_POINT('Ctrl Pts',(-80.5654528869998,-3.81569066033551,
-5.24030033591639));
#42182=CARTESIAN_POINT('Ctrl Pts',(-80.4663651017831,-0.84865751236067,
-6.42650941434701));
#42183=CARTESIAN_POINT('Ctrl Pts',(-80.3672773165665,2.32458847824698,-6.05115949490496));
#42184=CARTESIAN_POINT('Ctrl Pts',(-80.2681895313497,4.9329894152624,-4.20545577255142));
#42185=CARTESIAN_POINT('Ctrl Pts',(-80.1691017461332,6.34273747384018,-1.33788047445222));
#42186=CARTESIAN_POINT('Ctrl Pts',(-80.0700139609164,6.21128203689244,1.85478254362996));
#42187=CARTESIAN_POINT('Ctrl Pts',(-79.9709261756998,4.57056508211651,4.59675729793451));
#42188=CARTESIAN_POINT('Ctrl Pts',(-79.871838390483,1.81925969290868,6.22177924678583));
#42189=CARTESIAN_POINT('Ctrl Pts',(-79.7727506052665,-1.37410236497632,
6.3349889910357));
#42190=CARTESIAN_POINT('Ctrl Pts',(-79.6736628200496,-4.23357525011125,
4.90887802126133));
#42191=CARTESIAN_POINT('Ctrl Pts',(-79.5745750348332,-6.06434388870396,
2.28997293117537));
#42192=CARTESIAN_POINT('Ctrl Pts',(-79.4754872496163,-6.42155508654061,
-0.885366080500809));
#42193=CARTESIAN_POINT('Ctrl Pts',(-79.3763994643998,-5.21841112433719,
-3.84557254038601));
#42194=CARTESIAN_POINT('Ctrl Pts',(-79.2773116791831,-2.7472604853497,-5.87135441372885));
#42195=CARTESIAN_POINT('Ctrl Pts',(-79.1782238939664,0.391439059863712,
-6.47047280253847));
#42196=CARTESIAN_POINT('Ctrl Pts',(-79.0791361087498,3.43502395626256,-5.49734965650533));
#42197=CARTESIAN_POINT('Ctrl Pts',(-78.980048323533,5.64394228314933,-3.18844136381023));
#42198=CARTESIAN_POINT('Ctrl Pts',(-78.8809605383164,6.48145534358615,-0.104782894956996));
#42199=CARTESIAN_POINT('Ctrl Pts',(-78.7818727530997,5.74405825318873,3.00433646750017));
#42200=CARTESIAN_POINT('Ctrl Pts',(-78.682784967883,3.61092900537051,5.38344077186245));
#42201=CARTESIAN_POINT('Ctrl Pts',(-78.5836971826664,0.600390527212153,
6.45443832109432));
#42202=CARTESIAN_POINT('Ctrl Pts',(-78.4846093974497,-2.55603511449917,
5.9570905079094));
#42203=CARTESIAN_POINT('Ctrl Pts',(-78.3855216122331,-5.09137715163132,
4.01224644380471));
#42204=CARTESIAN_POINT('Ctrl Pts',(-78.2864338270163,-6.38958013082574,
1.0924781818114));
#42205=CARTESIAN_POINT('Ctrl Pts',(-78.1873460417997,-6.13519745229988,
-2.09274820445987));
#42206=CARTESIAN_POINT('Ctrl Pts',(-78.088258256583,-4.39004082983858,-4.76946373697579));
#42207=CARTESIAN_POINT('Ctrl Pts',(-77.9891704713664,-1.57816084063661,
-6.2872610242504));
#42208=CARTESIAN_POINT('Ctrl Pts',(-77.8900826861497,1.61719190210787,-6.27733487857178));
#42209=CARTESIAN_POINT('Ctrl Pts',(-77.790994900933,4.41958784619184,-4.74209722546579));
#42210=CARTESIAN_POINT('Ctrl Pts',(-77.6919071157163,6.14808087920214,-2.05459103686501));
#42211=CARTESIAN_POINT('Ctrl Pts',(-77.5928193304997,6.3826694615111,1.13215430532706));
#42212=CARTESIAN_POINT('Ctrl Pts',(-77.493731545283,5.06635158971623,4.04380073635643));
#42213=CARTESIAN_POINT('Ctrl Pts',(-77.3946437600663,2.51897554913599,5.97285568290681));
#42214=CARTESIAN_POINT('Ctrl Pts',(-77.2955559748497,-0.640479099061789,
6.45058364410864));
#42215=CARTESIAN_POINT('Ctrl Pts',(-77.196468189633,-3.64430557719005,5.36090287974316));
#42216=CARTESIAN_POINT('Ctrl Pts',(-77.0973804044164,-5.76261274800134,
2.96859177768677));
#42217=CARTESIAN_POINT('Ctrl Pts',(-76.9982926191996,-6.4806792581815,-0.145048883322511));
#42218=CARTESIAN_POINT('Ctrl Pts',(-76.899204833983,-5.6240241962828,-3.22344453428357));
#42219=CARTESIAN_POINT('Ctrl Pts',(-76.8001170487663,-3.40080370644699,
-5.51858468959146));
#42220=CARTESIAN_POINT('Ctrl Pts',(-76.7010292635497,-0.351231726960331,
-6.47277985875879));
#42221=CARTESIAN_POINT('Ctrl Pts',(-76.6019414783329,2.78368503741827,-5.85417290814259));
#42222=CARTESIAN_POINT('Ctrl Pts',(-76.5028536931163,5.24220219865931,-3.81307735750908));
#42223=CARTESIAN_POINT('Ctrl Pts',(-76.4037659078996,6.42693175854569,-0.845453131151542));
#42224=CARTESIAN_POINT('Ctrl Pts',(-76.304678122683,6.04999969635994,2.32760531448557));
#42225=CARTESIAN_POINT('Ctrl Pts',(-76.2055903374662,4.20299564736804,4.93508565418903));
#42226=CARTESIAN_POINT('Ctrl Pts',(-76.1065025522496,1.3347178013573,6.34340375640058));
#42227=CARTESIAN_POINT('Ctrl Pts',(-76.0074147670329,-1.85787927581762,
6.21035646500782));
#42228=CARTESIAN_POINT('Ctrl Pts',(-75.9083269818163,-4.59903562318709,
4.56827255783114));
#42229=CARTESIAN_POINT('Ctrl Pts',(-75.8092391965996,-6.2226855614176,1.81615727009033));
#42230=CARTESIAN_POINT('Ctrl Pts',(-75.710151411383,-6.33430307226678,-1.37726083754989));
#42231=CARTESIAN_POINT('Ctrl Pts',(-75.6110636261662,-4.90676653851619,
-4.23602230429382));
#42232=CARTESIAN_POINT('Ctrl Pts',(-75.5119758409496,-2.28694894755983,
-6.06548492185348));
#42233=CARTESIAN_POINT('Ctrl Pts',(-75.4128880557329,0.888567775924808,
-6.42111284230117));
#42234=CARTESIAN_POINT('Ctrl Pts',(-75.3138002705162,3.84817397687645,-5.21649306236172));
#42235=CARTESIAN_POINT('Ctrl Pts',(-75.2147124852996,5.87272347573166,-2.7443326699887));
#42236=CARTESIAN_POINT('Ctrl Pts',(-75.1156247000829,6.47027682562396,0.394665207195212));
#42237=CARTESIAN_POINT('Ctrl Pts',(-75.0165369148663,5.49563626053907,3.43776452332399));
#42238=CARTESIAN_POINT('Ctrl Pts',(-74.9174491296495,3.18562688193913,5.64553134745027));
#42239=CARTESIAN_POINT('Ctrl Pts',(-74.8183613444329,0.101551210018007,
6.48150678297269));
#42240=CARTESIAN_POINT('Ctrl Pts',(-74.7192735592163,-3.00720009769922,
5.74255956855258));
#42241=CARTESIAN_POINT('Ctrl Pts',(-74.6201857739996,-5.38524052207403,
3.60824435777137));
#42242=CARTESIAN_POINT('Ctrl Pts',(-74.5210979887829,-6.45473687520237,
0.59717225143153));
#42243=CARTESIAN_POINT('Ctrl Pts',(-74.4220102035662,-5.95581532111178,
-2.55900501890618));
#42244=CARTESIAN_POINT('Ctrl Pts',(-74.3229224183495,-4.00970737006563,
-5.09337703615375));
#42245=CARTESIAN_POINT('Ctrl Pts',(-74.2238346331329,-1.08929218333971,
-6.39012404928824));
#42246=CARTESIAN_POINT('Ctrl Pts',(-74.1247468479162,2.09580697107931,-6.13415323952314));
#42247=CARTESIAN_POINT('Ctrl Pts',(-74.0256590626996,4.77165203085921,-4.38766221607524));
#42248=CARTESIAN_POINT('Ctrl Pts',(-73.9265712774829,6.2880471181749,-1.5750257983885));
#42249=CARTESIAN_POINT('Ctrl Pts',(-73.8274834922662,6.27652776184059,1.62032159796177));
#42250=CARTESIAN_POINT('Ctrl Pts',(-73.7283957070496,4.73989301704688,4.42195171987746));
#42251=CARTESIAN_POINT('Ctrl Pts',(-73.6293079218328,2.05152533100835,6.1491045398666));
#42252=CARTESIAN_POINT('Ctrl Pts',(-73.5302201366162,-1.13533658159241,
6.38210417280031));
#42253=CARTESIAN_POINT('Ctrl Pts',(-73.4311323513995,-4.04632633089381,
5.06433470950454));
#42254=CARTESIAN_POINT('Ctrl Pts',(-73.3320445661828,-5.9741109087797,2.51599715333231));
#42255=CARTESIAN_POINT('Ctrl Pts',(-73.2329567809662,-6.45026349760051,
-0.643695298646502));
#42256=CARTESIAN_POINT('Ctrl Pts',(-73.1338689957495,-5.3590851523311,-3.64697808548958));
#42257=CARTESIAN_POINT('Ctrl Pts',(-73.0347812105328,-2.96571815371499,
-5.7640921799276));
#42258=CARTESIAN_POINT('Ctrl Pts',(-72.9356934253162,0.148280150248475,
-6.48060613083523));
#42259=CARTESIAN_POINT('Ctrl Pts',(-72.8366056400995,3.22624828792765,-5.62241627866711));
#42260=CARTESIAN_POINT('Ctrl Pts',(-72.7375178548829,5.52027965393766,-3.3980517018284));
#42261=CARTESIAN_POINT('Ctrl Pts',(-72.6384300696661,6.47295417930641,-0.348004337008301));
#42262=CARTESIAN_POINT('Ctrl Pts',(-72.5393422844495,5.85278422724426,2.78660359852236));
#42263=CARTESIAN_POINT('Ctrl Pts',(-72.4402544992328,3.81046310673336,5.24410275816569));
#42264=CARTESIAN_POINT('Ctrl Pts',(-72.3411667140162,0.842248539758685,
6.42735250497835));
#42265=CARTESIAN_POINT('Ctrl Pts',(-72.2420789287994,-2.33062157207041,
6.04883839375603));
#42266=CARTESIAN_POINT('Ctrl Pts',(-72.1429911435828,-4.93718066622978,
4.20053447729974));
#42267=CARTESIAN_POINT('Ctrl Pts',(-72.0439033583661,-6.34406846196043,
1.33155479644511));
#42268=CARTESIAN_POINT('Ctrl Pts',(-71.9448155731495,-6.20942934919886,
-1.86097554612759));
#42269=CARTESIAN_POINT('Ctrl Pts',(-71.8457277879328,-4.56597889785132,
-4.60131280509741));
#42270=CARTESIAN_POINT('Ctrl Pts',(-71.7466400027161,-1.81305439576657,
-6.22359032905994));
#42271=CARTESIAN_POINT('Ctrl Pts',(-71.6475522174995,1.38041896772984,-6.33361557875979));
#42272=CARTESIAN_POINT('Ctrl Pts',(-71.5484644322828,4.238468305381,-4.90465383592539));
#42273=CARTESIAN_POINT('Ctrl Pts',(-71.4493766470661,6.06662444709443,-2.28392439539779));
#42274=CARTESIAN_POINT('Ctrl Pts',(-71.3502888618495,6.42066900174233,0.89176925044665));
#42275=CARTESIAN_POINT('Ctrl Pts',(-71.2512010766327,5.2145737035411,3.8507744566924));
#42276=CARTESIAN_POINT('Ctrl Pts',(-71.1521132914161,2.7414041723735,5.87409107774727));
#42277=CARTESIAN_POINT('Ctrl Pts',(-71.0530255061994,-0.397891256411005,
6.47007924016768));
#42278=CARTESIAN_POINT('Ctrl Pts',(-70.9539377209828,-3.44050423574074,
5.49392149833132));
#42279=CARTESIAN_POINT('Ctrl Pts',(-70.854849935766,-5.64711900824516,3.18281160810583));
#42280=CARTESIAN_POINT('Ctrl Pts',(-70.7557621505494,-6.4815566110256,0.0983194998327943));
#42281=CARTESIAN_POINT('Ctrl Pts',(-70.6566743653327,-5.74105945628859,
-3.01006298029397));
#42282=CARTESIAN_POINT('Ctrl Pts',(-70.5575865801161,-3.6055588131454,-5.38703893348903));
#42283=CARTESIAN_POINT('Ctrl Pts',(-70.4584987948994,-0.593953827191011,
-6.45503382463191));
#42284=CARTESIAN_POINT('Ctrl Pts',(-70.3594110096827,2.56197428713231,-5.95453865366998));
#42285=CARTESIAN_POINT('Ctrl Pts',(-70.2603232244661,5.09537565443828,-4.00716729949408));
#42286=CARTESIAN_POINT('Ctrl Pts',(-70.1612354392494,6.39066637913534,-1.08610591406471));
#42287=CARTESIAN_POINT('Ctrl Pts',(-70.0621476540327,6.13310750176651,2.09886521667122));
#42288=CARTESIAN_POINT('Ctrl Pts',(-69.9630598688161,4.38528251151797,4.77383913848715));
#42289=CARTESIAN_POINT('Ctrl Pts',(-69.8639720835993,1.57189036458139,6.28883164886079));
#42290=CARTESIAN_POINT('Ctrl Pts',(-69.7648842983828,-1.62345089099596,
6.27571908473456));
#42291=CARTESIAN_POINT('Ctrl Pts',(-69.665796513166,-4.42431449424472,4.73768763026785));
#42292=CARTESIAN_POINT('Ctrl Pts',(-69.5667087279494,-6.15012667183424,
2.04845911513266));
#42293=CARTESIAN_POINT('Ctrl Pts',(-69.4676209427327,-6.38153729746785,
-1.13851857560769));
#42294=CARTESIAN_POINT('Ctrl Pts',(-69.368533157516,-5.062316570275,-4.04885091949506));
#42295=CARTESIAN_POINT('Ctrl Pts',(-69.2694453722994,-2.5130181320396,-5.97536464946014));
#42296=CARTESIAN_POINT('Ctrl Pts',(-69.1703575870826,0.646911338205425,
-6.44994174752579));
#42297=CARTESIAN_POINT('Ctrl Pts',(-69.0712698018661,3.64964968713308,-5.35726609262518));
#42298=CARTESIAN_POINT('Ctrl Pts',(-68.9721820166493,5.76557017887249,-2.96284379245084));
#42299=CARTESIAN_POINT('Ctrl Pts',(-68.8730942314327,6.48053139238009,0.151511380309847));
#42300=CARTESIAN_POINT('Ctrl Pts',(-68.774006446216,5.62080696329017,3.22905123951376));
#42301=CARTESIAN_POINT('Ctrl Pts',(-68.6749186609993,3.39529885244121,5.52197324591022));
#42302=CARTESIAN_POINT('Ctrl Pts',(-68.5758308757827,0.344776860533978,
6.47312689065817));
#42303=CARTESIAN_POINT('Ctrl Pts',(-68.476743090566,-2.78952146684973,5.85139409129237));
#42304=CARTESIAN_POINT('Ctrl Pts',(-68.3776553053494,-5.24600201399085,
3.80784790870568));
#42305=CARTESIAN_POINT('Ctrl Pts',(-68.2785675201326,-6.42777165348394,
0.839043738882656));
#42306=CARTESIAN_POINT('Ctrl Pts',(-68.179479734916,-6.04767558749643,-2.33363725005636));
#42307=CARTESIAN_POINT('Ctrl Pts',(-68.0803919496993,-4.1980722627264,-4.9392744512594));
#42308=CARTESIAN_POINT('Ctrl Pts',(-67.9813041644827,-1.3283914609729,-6.34473158955201));
#42309=CARTESIAN_POINT('Ctrl Pts',(-67.882216379266,1.864071354745,-6.20850069132352));
#42310=CARTESIAN_POINT('Ctrl Pts',(-67.7831285940493,4.60358884116279,-4.5636840994466));
#42311=CARTESIAN_POINT('Ctrl Pts',(-67.6840408088326,6.22449355341539,-1.80995107740288));
#42312=CARTESIAN_POINT('Ctrl Pts',(-67.584953023616,6.33292650272045,1.38357676830714));
#42313=CARTESIAN_POINT('Ctrl Pts',(-67.4858652383993,4.90253993016824,4.24091322523118));
#42314=CARTESIAN_POINT('Ctrl Pts',(-67.3867774531826,2.2808992426794,6.06776251998367));
#42315=CARTESIAN_POINT('Ctrl Pts',(-67.287689667966,-0.894970436826739,
6.42022345172595));
#42316=CARTESIAN_POINT('Ctrl Pts',(-67.1886018827492,-3.8533741139406,5.21265327802973));
#42317=CARTESIAN_POINT('Ctrl Pts',(-67.0895140975326,-5.87545694614519,
2.73847452742765));
#42318=CARTESIAN_POINT('Ctrl Pts',(-66.990426312316,-6.46988060047446,-0.401116262019477));
#42319=CARTESIAN_POINT('Ctrl Pts',(-66.8913385270993,-5.49220424623203,
-3.44324500874027));
#42320=CARTESIAN_POINT('Ctrl Pts',(-66.7922507418826,-3.17999782273006,
-5.64870137951734));
#42321=CARTESIAN_POINT('Ctrl Pts',(-66.693162956666,-0.0950831417423778,
-6.481612708114));
#42322=CARTESIAN_POINT('Ctrl Pts',(-66.5940751714492,3.01291573775549,-5.73954193441991));
#42323=CARTESIAN_POINT('Ctrl Pts',(-66.4949873862326,5.38885502338481,-3.60290479060144));
#42324=CARTESIAN_POINT('Ctrl Pts',(-66.3958996010159,6.45529058685379,-0.590669449163867));
#42325=CARTESIAN_POINT('Ctrl Pts',(-66.2968118157992,5.95333891379727,2.5648081547044));
#42326=CARTESIAN_POINT('Ctrl Pts',(-66.1977240305826,4.00446383910233,5.09765494987877));
#42327=CARTESIAN_POINT('Ctrl Pts',(-66.1316655071048,2.05700390032189,5.9593576533423));
#42328=CARTESIAN_POINT('Ctrl Pts',(-66.0986362453659,1.03897443108136,6.13185148988943));
#42329=CARTESIAN_POINT('Ctrl Pts',(-66.51072,1.15821195975198,6.83557123116185));
#42330=CARTESIAN_POINT('Ctrl Pts',(-66.5437492617389,2.29307521661488,6.64328120120947));
#42331=CARTESIAN_POINT('Ctrl Pts',(-66.5767785234778,3.37855495738465,6.16298334832425));
#42332=CARTESIAN_POINT('Ctrl Pts',(-66.6098077852167,4.28338433193964,5.45224641338801));
#42333=CARTESIAN_POINT('Ctrl Pts',(-66.6428370469556,5.18821370649464,4.74150947845177));
#42334=CARTESIAN_POINT('Ctrl Pts',(-66.6758663086944,5.91239271483488,3.8003334614645));
#42335=CARTESIAN_POINT('Ctrl Pts',(-66.7088955704333,6.36774188186092,2.74347630938123));
#42336=CARTESIAN_POINT('Ctrl Pts',(-66.7419248321722,6.82309104888695,1.686619157298));
#42337=CARTESIAN_POINT('Ctrl Pts',(-66.7749540939112,7.00961037459882,0.514080870118756));
#42338=CARTESIAN_POINT('Ctrl Pts',(-66.80798335565,6.90473259426009,-0.631843848826572));
#42339=CARTESIAN_POINT('Ctrl Pts',(-66.8410126173889,6.79985481392136,-1.77776856777197));
#42340=CARTESIAN_POINT('Ctrl Pts',(-66.8740418791278,6.403579927532,-2.89707971848347));
#42341=CARTESIAN_POINT('Ctrl Pts',(-66.9070711408667,5.7640069664622,-3.85370988397183));
#42342=CARTESIAN_POINT('Ctrl Pts',(-66.9401004026056,5.12443400539243,-4.81034004946015));
#42343=CARTESIAN_POINT('Ctrl Pts',(-66.9731296643445,4.24156296964229,-5.6042892297253));
#42344=CARTESIAN_POINT('Ctrl Pts',(-67.0061589260834,3.22267957537377,-6.13913619659199));
#42345=CARTESIAN_POINT('Ctrl Pts',(-67.0391881878223,2.20379618110529,-6.67398316345867));
#42346=CARTESIAN_POINT('Ctrl Pts',(-67.0722174495611,1.04890042831847,-6.94972791692685));
#42347=CARTESIAN_POINT('Ctrl Pts',(-67.1052467113,-0.101706416420187,-6.93285027714876));
#42348=CARTESIAN_POINT('Ctrl Pts',(-67.1382759730389,-1.2523132611589,-6.91597263737066));
#42349=CARTESIAN_POINT('Ctrl Pts',(-67.1713052347778,-2.39863119784948,
-6.60647260434626));
#42350=CARTESIAN_POINT('Ctrl Pts',(-67.2043344965167,-3.40138449386395,
-6.04196179088377));
#42351=CARTESIAN_POINT('Ctrl Pts',(-67.2373637582556,-4.40413778987836,
-5.47745097742132));
#42352=CARTESIAN_POINT('Ctrl Pts',(-67.2703930199945,-5.26332644521669,
-4.65792938352081));
#42353=CARTESIAN_POINT('Ctrl Pts',(-67.3034222817334,-5.87456727806366,
-3.68295899267487));
#42354=CARTESIAN_POINT('Ctrl Pts',(-67.3364515434723,-6.48580811091063,
-2.70798860182892));
#42355=CARTESIAN_POINT('Ctrl Pts',(-67.3694808052112,-6.84910112126625,
-1.57756941403751));
#42356=CARTESIAN_POINT('Ctrl Pts',(-67.4025100669501,-6.92030721440444,
-0.429042353050756));
#42357=CARTESIAN_POINT('Ctrl Pts',(-67.4066161567646,-6.92915932306131,
-0.286261224482349));
#42358=CARTESIAN_POINT('Ctrl Pts',(-67.4107222465792,-6.93349733082867,
-0.143200245082971));
#42359=CARTESIAN_POINT('Ctrl Pts',(-67.4148283363937,-6.93337279743796,
-0.000131731084783704));
#42360=CARTESIAN_POINT('Origin',(-87.75,0.,0.));
#42361=CARTESIAN_POINT('Origin',(-66.51072,0.,0.));
#42362=CARTESIAN_POINT('Origin',(-66.,9.38757796099391,-1.49533175231994));
#42363=CARTESIAN_POINT('',(-66.,9.50531436582601,-3.4877820755921));
#42364=CARTESIAN_POINT('',(-66.,10.1030411093822,-0.666472311603392));
#42365=CARTESIAN_POINT('Origin',(-66.,0.,0.));
#42366=CARTESIAN_POINT('',(-66.,7.75912709216827,-0.91164851646916));
#42367=CARTESIAN_POINT('Ctrl Pts',(-66.,7.75912709216827,-0.911648516469152));
#42368=CARTESIAN_POINT('Ctrl Pts',(-66.,7.77914589672304,-0.913085729118069));
#42369=CARTESIAN_POINT('Ctrl Pts',(-66.,7.81916111326106,-0.916160028010783));
#42370=CARTESIAN_POINT('Ctrl Pts',(-66.,7.87911675845826,-0.921371110962998));
#42371=CARTESIAN_POINT('Ctrl Pts',(-66.,7.95892309714082,-0.92951996674881));
#42372=CARTESIAN_POINT('Ctrl Pts',(-66.,8.05846479644172,-0.94163789416019));
#42373=CARTESIAN_POINT('Ctrl Pts',(-66.,8.15781635562219,-0.955460858076408));
#42374=CARTESIAN_POINT('Ctrl Pts',(-66.,8.25703088282646,-0.970525968901249));
#42375=CARTESIAN_POINT('Ctrl Pts',(-66.,8.35619956862638,-0.986039820385861));
#42376=CARTESIAN_POINT('Ctrl Pts',(-66.,8.45545727626546,-1.00082385038912));
#42377=CARTESIAN_POINT('Ctrl Pts',(-66.,8.5549523562227,-1.01352414725572));
#42378=CARTESIAN_POINT('Ctrl Pts',(-66.,8.65481931169516,-1.0227982069947));
#42379=CARTESIAN_POINT('Ctrl Pts',(-66.,8.75515237563664,-1.02749863562185));
#42380=CARTESIAN_POINT('Ctrl Pts',(-66.,8.85597360323765,-1.02688738551608));
#42381=CARTESIAN_POINT('Ctrl Pts',(-66.,8.95721840904376,-1.02074993441888));
#42382=CARTESIAN_POINT('Ctrl Pts',(-66.,9.05876930477337,-1.00922949007046));
#42383=CARTESIAN_POINT('Ctrl Pts',(-66.,9.16048129971873,-0.992712229606096));
#42384=CARTESIAN_POINT('Ctrl Pts',(-66.,9.26220852393388,-0.971700897727075));
#42385=CARTESIAN_POINT('Ctrl Pts',(-66.,9.36383468209953,-0.946679483797828));
#42386=CARTESIAN_POINT('Ctrl Pts',(-66.,9.46528658437238,-0.9180359267008));
#42387=CARTESIAN_POINT('Ctrl Pts',(-66.,9.56651871386955,-0.886087649174329));
#42388=CARTESIAN_POINT('Ctrl Pts',(-66.,9.66750440467984,-0.851083007004113));
#42389=CARTESIAN_POINT('Ctrl Pts',(-66.,9.76822511794956,-0.813212594962941));
#42390=CARTESIAN_POINT('Ctrl Pts',(-66.,9.8686591303367,-0.772616048562836));
#42391=CARTESIAN_POINT('Ctrl Pts',(-66.,9.95571582676883,-0.735030406117664));
#42392=CARTESIAN_POINT('Ctrl Pts',(-66.,10.022551212884,-0.704655396487718));
#42393=CARTESIAN_POINT('Ctrl Pts',(-66.,10.0693164096301,-0.682658849179938));
#42394=CARTESIAN_POINT('Ctrl Pts',(-66.,10.0961259401211,-0.669804263759911));
#42395=CARTESIAN_POINT('Ctrl Pts',(-66.,10.1030411093822,-0.666472311603392));
#42396=CARTESIAN_POINT('',(-66.,7.45911616757565,-2.32308894548002));
#42397=CARTESIAN_POINT('Origin',(-66.,0.,0.));
#42398=CARTESIAN_POINT('Ctrl Pts',(-66.,9.50531436582601,-3.4877820755921));
#42399=CARTESIAN_POINT('Ctrl Pts',(-66.,9.49314968148027,-3.47204626414704));
#42400=CARTESIAN_POINT('Ctrl Pts',(-66.,9.46406244582505,-3.43569488186565));
#42401=CARTESIAN_POINT('Ctrl Pts',(-66.,9.41732601303256,-3.38194356049215));
#42402=CARTESIAN_POINT('Ctrl Pts',(-66.,9.35182499787114,-3.31534545781812));
#42403=CARTESIAN_POINT('Ctrl Pts',(-66.,9.2665602360089,-3.23781625057574));
#42404=CARTESIAN_POINT('Ctrl Pts',(-66.,9.17473495202629,-3.15707031802335));
#42405=CARTESIAN_POINT('Ctrl Pts',(-66.,9.08161987720375,-3.07429102783389));
#42406=CARTESIAN_POINT('Ctrl Pts',(-66.,8.98705347372786,-2.99024137111801));
#42407=CARTESIAN_POINT('Ctrl Pts',(-66.,8.89061125688695,-2.90769272800839));
#42408=CARTESIAN_POINT('Ctrl Pts',(-66.,8.79176831392536,-2.8302457596494));
#42409=CARTESIAN_POINT('Ctrl Pts',(-66.,8.69012855448696,-2.76062472778166));
#42410=CARTESIAN_POINT('Ctrl Pts',(-66.,8.58555140837535,-2.69981100640618));
#42411=CARTESIAN_POINT('Ctrl Pts',(-66.,8.47810818661977,-2.64761048501369));
#42412=CARTESIAN_POINT('Ctrl Pts',(-66.,8.36807155833748,-2.6029226992256));
#42413=CARTESIAN_POINT('Ctrl Pts',(-66.,8.25589807840597,-2.56413168225005));
#42414=CARTESIAN_POINT('Ctrl Pts',(-66.,8.14220082613772,-2.52941102084457));
#42415=CARTESIAN_POINT('Ctrl Pts',(-66.,8.02764802899043,-2.49691117466945));
#42416=CARTESIAN_POINT('Ctrl Pts',(-66.,7.91287572547377,-2.46495249663592));
#42417=CARTESIAN_POINT('Ctrl Pts',(-66.,7.79839054163423,-2.43222686627939));
#42418=CARTESIAN_POINT('Ctrl Pts',(-66.,7.68448877252354,-2.39796845787595));
#42419=CARTESIAN_POINT('Ctrl Pts',(-66.,7.5939515764785,-2.36903210935654));
#42420=CARTESIAN_POINT('Ctrl Pts',(-66.,7.52639813136866,-2.34641563722107));
#42421=CARTESIAN_POINT('Ctrl Pts',(-66.,7.48151763438731,-2.3309321471704));
#42422=CARTESIAN_POINT('Ctrl Pts',(-66.,7.45911616757565,-2.32308894548002));
#42423=CARTESIAN_POINT('Ctrl Pts',(-66.,7.45911616757565,-2.32308894548002));
#42424=CARTESIAN_POINT('Ctrl Pts',(-50.,7.45911616757565,-2.32308894548002));
#42425=CARTESIAN_POINT('Ctrl Pts',(-66.,7.48151763438731,-2.3309321471704));
#42426=CARTESIAN_POINT('Ctrl Pts',(-50.,7.48151763438731,-2.3309321471704));
#42427=CARTESIAN_POINT('Ctrl Pts',(-66.,7.52639813136866,-2.34641563722107));
#42428=CARTESIAN_POINT('Ctrl Pts',(-50.,7.52639813136866,-2.34641563722107));
#42429=CARTESIAN_POINT('Ctrl Pts',(-66.,7.5939515764785,-2.36903210935654));
#42430=CARTESIAN_POINT('Ctrl Pts',(-50.,7.5939515764785,-2.36903210935654));
#42431=CARTESIAN_POINT('Ctrl Pts',(-66.,7.68448877252354,-2.39796845787595));
#42432=CARTESIAN_POINT('Ctrl Pts',(-50.,7.68448877252354,-2.39796845787595));
#42433=CARTESIAN_POINT('Ctrl Pts',(-66.,7.79839054163423,-2.43222686627939));
#42434=CARTESIAN_POINT('Ctrl Pts',(-50.,7.79839054163423,-2.43222686627939));
#42435=CARTESIAN_POINT('Ctrl Pts',(-66.,7.91287572547377,-2.46495249663592));
#42436=CARTESIAN_POINT('Ctrl Pts',(-50.,7.91287572547377,-2.46495249663592));
#42437=CARTESIAN_POINT('Ctrl Pts',(-66.,8.02764802899043,-2.49691117466945));
#42438=CARTESIAN_POINT('Ctrl Pts',(-50.,8.02764802899043,-2.49691117466945));
#42439=CARTESIAN_POINT('Ctrl Pts',(-66.,8.14220082613772,-2.52941102084457));
#42440=CARTESIAN_POINT('Ctrl Pts',(-50.,8.14220082613772,-2.52941102084457));
#42441=CARTESIAN_POINT('Ctrl Pts',(-66.,8.25589807840597,-2.56413168225005));
#42442=CARTESIAN_POINT('Ctrl Pts',(-50.,8.25589807840597,-2.56413168225005));
#42443=CARTESIAN_POINT('Ctrl Pts',(-66.,8.36807155833748,-2.6029226992256));
#42444=CARTESIAN_POINT('Ctrl Pts',(-50.,8.36807155833748,-2.6029226992256));
#42445=CARTESIAN_POINT('Ctrl Pts',(-66.,8.47810818661977,-2.64761048501369));
#42446=CARTESIAN_POINT('Ctrl Pts',(-50.,8.47810818661977,-2.64761048501369));
#42447=CARTESIAN_POINT('Ctrl Pts',(-66.,8.58555140837535,-2.69981100640618));
#42448=CARTESIAN_POINT('Ctrl Pts',(-50.,8.58555140837535,-2.69981100640618));
#42449=CARTESIAN_POINT('Ctrl Pts',(-66.,8.69012855448696,-2.76062472778166));
#42450=CARTESIAN_POINT('Ctrl Pts',(-50.,8.69012855448696,-2.76062472778166));
#42451=CARTESIAN_POINT('Ctrl Pts',(-66.,8.79176831392536,-2.8302457596494));
#42452=CARTESIAN_POINT('Ctrl Pts',(-50.,8.79176831392536,-2.8302457596494));
#42453=CARTESIAN_POINT('Ctrl Pts',(-66.,8.89061125688695,-2.90769272800839));
#42454=CARTESIAN_POINT('Ctrl Pts',(-50.,8.89061125688695,-2.90769272800839));
#42455=CARTESIAN_POINT('Ctrl Pts',(-66.,8.98705347372786,-2.99024137111801));
#42456=CARTESIAN_POINT('Ctrl Pts',(-50.,8.98705347372786,-2.99024137111801));
#42457=CARTESIAN_POINT('Ctrl Pts',(-66.,9.08161987720375,-3.07429102783389));
#42458=CARTESIAN_POINT('Ctrl Pts',(-50.,9.08161987720375,-3.07429102783389));
#42459=CARTESIAN_POINT('Ctrl Pts',(-66.,9.17473495202629,-3.15707031802335));
#42460=CARTESIAN_POINT('Ctrl Pts',(-50.,9.17473495202629,-3.15707031802335));
#42461=CARTESIAN_POINT('Ctrl Pts',(-66.,9.2665602360089,-3.23781625057574));
#42462=CARTESIAN_POINT('Ctrl Pts',(-50.,9.2665602360089,-3.23781625057574));
#42463=CARTESIAN_POINT('Ctrl Pts',(-66.,9.3567226928151,-3.31979881460968));
#42464=CARTESIAN_POINT('Ctrl Pts',(-50.,9.3567226928151,-3.31979881460968));
#42465=CARTESIAN_POINT('Ctrl Pts',(-66.,9.44439430274083,-3.40964474504027));
#42466=CARTESIAN_POINT('Ctrl Pts',(-50.,9.44439430274083,-3.40964474504027));
#42467=CARTESIAN_POINT('Ctrl Pts',(-66.,9.52877945206957,-3.51352466905028));
#42468=CARTESIAN_POINT('Ctrl Pts',(-50.,9.52877945206957,-3.51352466905028));
#42469=CARTESIAN_POINT('Ctrl Pts',(-66.,9.60947298443164,-3.63434129183301));
#42470=CARTESIAN_POINT('Ctrl Pts',(-50.,9.60947298443164,-3.63434129183301));
#42471=CARTESIAN_POINT('Ctrl Pts',(-66.,9.6869239989324,-3.76808784102041));
#42472=CARTESIAN_POINT('Ctrl Pts',(-50.,9.6869239989324,-3.76808784102041));
#42473=CARTESIAN_POINT('Ctrl Pts',(-66.,9.7627049188411,-3.90175231914239));
#42474=CARTESIAN_POINT('Ctrl Pts',(-50.,9.7627049188411,-3.90175231914239));
#42475=CARTESIAN_POINT('Ctrl Pts',(-66.,9.83905157879557,-4.01702660556759));
#42476=CARTESIAN_POINT('Ctrl Pts',(-50.,9.83905157879557,-4.01702660556759));
#42477=CARTESIAN_POINT('Ctrl Pts',(-66.,9.91850412115979,-4.09321456481936));
#42478=CARTESIAN_POINT('Ctrl Pts',(-50.,9.91850412115979,-4.09321456481936));
#42479=CARTESIAN_POINT('Ctrl Pts',(-66.,10.003524961334,-4.11032134692824));
#42480=CARTESIAN_POINT('Ctrl Pts',(-50.,10.003524961334,-4.11032134692824));
#42481=CARTESIAN_POINT('Ctrl Pts',(-66.,10.0960897853042,-4.05236656747314));
#42482=CARTESIAN_POINT('Ctrl Pts',(-50.,10.0960897853042,-4.05236656747314));
#42483=CARTESIAN_POINT('Ctrl Pts',(-66.,10.1977063391542,-3.90721566927367));
#42484=CARTESIAN_POINT('Ctrl Pts',(-50.,10.1977063391542,-3.90721566927367));
#42485=CARTESIAN_POINT('Ctrl Pts',(-66.,10.3094940348316,-3.6659181197565));
#42486=CARTESIAN_POINT('Ctrl Pts',(-50.,10.3094940348316,-3.6659181197565));
#42487=CARTESIAN_POINT('Ctrl Pts',(-66.,10.4322386329331,-3.32224944575216));
#42488=CARTESIAN_POINT('Ctrl Pts',(-50.,10.4322386329331,-3.32224944575216));
#42489=CARTESIAN_POINT('Ctrl Pts',(-66.,10.5664542961036,-2.87219453321856));
#42490=CARTESIAN_POINT('Ctrl Pts',(-50.,10.5664542961036,-2.87219453321856));
#42491=CARTESIAN_POINT('Ctrl Pts',(-66.,10.7124395485472,-2.31348157729569));
#42492=CARTESIAN_POINT('Ctrl Pts',(-50.,10.7124395485472,-2.31348157729569));
#42493=CARTESIAN_POINT('Ctrl Pts',(-66.,10.8703331900164,-1.64511745895776));
#42494=CARTESIAN_POINT('Ctrl Pts',(-50.,10.8703331900164,-1.64511745895776));
#42495=CARTESIAN_POINT('Ctrl Pts',(-66.,11.0062009025174,-1.02257826517791));
#42496=CARTESIAN_POINT('Ctrl Pts',(-50.,11.0062009025174,-1.02257826517791));
#42497=CARTESIAN_POINT('Ctrl Pts',(-66.,11.1134656310101,-0.506367938989212));
#42498=CARTESIAN_POINT('Ctrl Pts',(-50.,11.1134656310101,-0.506367938989212));
#42499=CARTESIAN_POINT('Ctrl Pts',(-66.,11.1873562558614,-0.140343105909661));
#42500=CARTESIAN_POINT('Ctrl Pts',(-50.,11.1873562558614,-0.140343105909661));
#42501=CARTESIAN_POINT('Ctrl Pts',(-66.,11.2248967699273,0.048140466098866));
#42502=CARTESIAN_POINT('Ctrl Pts',(-50.,11.2248967699273,0.048140466098866));
#42503=CARTESIAN_POINT('',(-65.5,9.84017809125458,-4.00768263868202));
#42504=CARTESIAN_POINT('Ctrl Pts',(-66.,9.50531436582601,-3.4877820755921));
#42505=CARTESIAN_POINT('Ctrl Pts',(-65.7982417703064,9.65105196151285,-3.67630314699894));
#42506=CARTESIAN_POINT('Ctrl Pts',(-65.6331946192804,9.7436125308195,-3.89166284380022));
#42507=CARTESIAN_POINT('Ctrl Pts',(-65.5,9.84017809125458,-4.00768263868202));
#42508=CARTESIAN_POINT('',(-50.,7.45911616757565,-2.32308894548002));
#42509=CARTESIAN_POINT('',(-66.,7.45911616757565,-2.32308894548002));
#42510=CARTESIAN_POINT('',(-50.,9.50531436582603,-3.48778207559212));
#42511=CARTESIAN_POINT('Ctrl Pts',(-50.,7.45911616757565,-2.32308894548002));
#42512=CARTESIAN_POINT('Ctrl Pts',(-50.,7.48151763438731,-2.3309321471704));
#42513=CARTESIAN_POINT('Ctrl Pts',(-50.,7.52639813136866,-2.34641563722107));
#42514=CARTESIAN_POINT('Ctrl Pts',(-50.,7.5939515764785,-2.36903210935654));
#42515=CARTESIAN_POINT('Ctrl Pts',(-50.,7.68448877252354,-2.39796845787595));
#42516=CARTESIAN_POINT('Ctrl Pts',(-50.,7.79839054163423,-2.43222686627939));
#42517=CARTESIAN_POINT('Ctrl Pts',(-50.,7.91287572547377,-2.46495249663592));
#42518=CARTESIAN_POINT('Ctrl Pts',(-50.,8.02764802899043,-2.49691117466945));
#42519=CARTESIAN_POINT('Ctrl Pts',(-50.,8.14220082613772,-2.52941102084457));
#42520=CARTESIAN_POINT('Ctrl Pts',(-50.,8.25589807840597,-2.56413168225005));
#42521=CARTESIAN_POINT('Ctrl Pts',(-50.,8.36807155833748,-2.6029226992256));
#42522=CARTESIAN_POINT('Ctrl Pts',(-50.,8.47810818661977,-2.64761048501369));
#42523=CARTESIAN_POINT('Ctrl Pts',(-50.,8.58555140837535,-2.69981100640618));
#42524=CARTESIAN_POINT('Ctrl Pts',(-50.,8.69012855448696,-2.76062472778166));
#42525=CARTESIAN_POINT('Ctrl Pts',(-50.,8.79176831392536,-2.8302457596494));
#42526=CARTESIAN_POINT('Ctrl Pts',(-50.,8.89061125688695,-2.90769272800839));
#42527=CARTESIAN_POINT('Ctrl Pts',(-50.,8.98705347372786,-2.99024137111801));
#42528=CARTESIAN_POINT('Ctrl Pts',(-50.,9.08161987720375,-3.07429102783389));
#42529=CARTESIAN_POINT('Ctrl Pts',(-50.,9.17473495202629,-3.15707031802335));
#42530=CARTESIAN_POINT('Ctrl Pts',(-50.,9.2665602360089,-3.23781625057574));
#42531=CARTESIAN_POINT('Ctrl Pts',(-50.,9.35182499787114,-3.31534545781812));
#42532=CARTESIAN_POINT('Ctrl Pts',(-50.,9.41732601303256,-3.38194356049215));
#42533=CARTESIAN_POINT('Ctrl Pts',(-50.,9.46406244582506,-3.43569488186566));
#42534=CARTESIAN_POINT('Ctrl Pts',(-50.,9.49314968148028,-3.47204626414705));
#42535=CARTESIAN_POINT('Ctrl Pts',(-50.,9.50531436582603,-3.48778207559212));
#42536=CARTESIAN_POINT('',(-50.5,9.84017809125458,-4.00768263868202));
#42537=CARTESIAN_POINT('Ctrl Pts',(-50.5,9.84017809125459,-4.00768263868203));
#42538=CARTESIAN_POINT('Ctrl Pts',(-50.4982567069803,9.83891421086397,-4.00616413515951));
#42539=CARTESIAN_POINT('Ctrl Pts',(-50.4965113438768,9.8376533352101,-4.00463244240549));
#42540=CARTESIAN_POINT('Ctrl Pts',(-50.3581212730785,9.73802153669804,-3.88231384117201));
#42541=CARTESIAN_POINT('Ctrl Pts',(-50.2022201285465,9.65138560851398,-3.67673474112415));
#42542=CARTESIAN_POINT('Ctrl Pts',(-50.,9.50531436582603,-3.48778207559212));
#42543=CARTESIAN_POINT('Ctrl Pts',(-65.5,9.84017809125458,-4.00768263868202));
#42544=CARTESIAN_POINT('Ctrl Pts',(-60.5,9.84017809125458,-4.00768263868202));
#42545=CARTESIAN_POINT('Ctrl Pts',(-55.5,9.84017809125458,-4.00768263868202));
#42546=CARTESIAN_POINT('Ctrl Pts',(-50.5,9.84017809125458,-4.00768263868202));
#42547=CARTESIAN_POINT('Origin',(-66.,0.,0.));
#42548=CARTESIAN_POINT('',(-50.,7.75912709216827,-0.91164851646916));
#42549=CARTESIAN_POINT('',(-66.,7.75912709216827,-0.91164851646916));
#42550=CARTESIAN_POINT('Origin',(-50.,0.,0.));
#42551=CARTESIAN_POINT('Ctrl Pts',(-66.,11.2248967699273,0.048140466098866));
#42552=CARTESIAN_POINT('Ctrl Pts',(-50.,11.2248967699273,0.048140466098866));
#42553=CARTESIAN_POINT('Ctrl Pts',(-66.,11.2063599613097,0.0333893783018618));
#42554=CARTESIAN_POINT('Ctrl Pts',(-50.,11.2063599613097,0.0333893783018618));
#42555=CARTESIAN_POINT('Ctrl Pts',(-66.,11.1692224341001,0.00409091359342473));
#42556=CARTESIAN_POINT('Ctrl Pts',(-50.,11.1692224341001,0.00409091359342473));
#42557=CARTESIAN_POINT('Ctrl Pts',(-66.,11.1133244136114,-0.0392456507517008));
#42558=CARTESIAN_POINT('Ctrl Pts',(-50.,11.1133244136114,-0.0392456507517008));
#42559=CARTESIAN_POINT('Ctrl Pts',(-66.,11.0384097481576,-0.0958038462574695));
#42560=CARTESIAN_POINT('Ctrl Pts',(-50.,11.0384097481576,-0.0958038462574695));
#42561=CARTESIAN_POINT('Ctrl Pts',(-66.,10.9441246976668,-0.164449053510359));
#42562=CARTESIAN_POINT('Ctrl Pts',(-50.,10.9441246976668,-0.164449053510359));
#42563=CARTESIAN_POINT('Ctrl Pts',(-66.,10.8491977491253,-0.231019991472708));
#42564=CARTESIAN_POINT('Ctrl Pts',(-50.,10.8491977491253,-0.231019991472708));
#42565=CARTESIAN_POINT('Ctrl Pts',(-66.,10.7536325411685,-0.295485610415231));
#42566=CARTESIAN_POINT('Ctrl Pts',(-50.,10.7536325411685,-0.295485610415231));
#42567=CARTESIAN_POINT('Ctrl Pts',(-66.,10.6574386110001,-0.357805568812489));
#42568=CARTESIAN_POINT('Ctrl Pts',(-50.,10.6574386110001,-0.357805568812489));
#42569=CARTESIAN_POINT('Ctrl Pts',(-66.,10.5606341069048,-0.417929905154785));
#42570=CARTESIAN_POINT('Ctrl Pts',(-50.,10.5606341069048,-0.417929905154785));
#42571=CARTESIAN_POINT('Ctrl Pts',(-66.,10.4632449048126,-0.475801947946924));
#42572=CARTESIAN_POINT('Ctrl Pts',(-50.,10.4632449048126,-0.475801947946924));
#42573=CARTESIAN_POINT('Ctrl Pts',(-66.,10.3653028555026,-0.531361945998192));
#42574=CARTESIAN_POINT('Ctrl Pts',(-50.,10.3653028555026,-0.531361945998192));
#42575=CARTESIAN_POINT('Ctrl Pts',(-66.,10.2668444511909,-0.584551084436177));
#42576=CARTESIAN_POINT('Ctrl Pts',(-50.,10.2668444511909,-0.584551084436177));
#42577=CARTESIAN_POINT('Ctrl Pts',(-66.,10.1679093574848,-0.635314704999891));
#42578=CARTESIAN_POINT('Ctrl Pts',(-50.,10.1679093574848,-0.635314704999891));
#42579=CARTESIAN_POINT('Ctrl Pts',(-66.,10.0685392194901,-0.683608443201678));
#42580=CARTESIAN_POINT('Ctrl Pts',(-50.,10.0685392194901,-0.683608443201678));
#42581=CARTESIAN_POINT('Ctrl Pts',(-66.,9.96877581793761,-0.729391917885004));
#42582=CARTESIAN_POINT('Ctrl Pts',(-50.,9.96877581793761,-0.729391917885004));
#42583=CARTESIAN_POINT('Ctrl Pts',(-66.,9.8686591303367,-0.772616048562836));
#42584=CARTESIAN_POINT('Ctrl Pts',(-50.,9.8686591303367,-0.772616048562836));
#42585=CARTESIAN_POINT('Ctrl Pts',(-66.,9.76822511794956,-0.813212594962941));
#42586=CARTESIAN_POINT('Ctrl Pts',(-50.,9.76822511794956,-0.813212594962941));
#42587=CARTESIAN_POINT('Ctrl Pts',(-66.,9.66750440467984,-0.851083007004113));
#42588=CARTESIAN_POINT('Ctrl Pts',(-50.,9.66750440467984,-0.851083007004113));
#42589=CARTESIAN_POINT('Ctrl Pts',(-66.,9.56651871386955,-0.886087649174329));
#42590=CARTESIAN_POINT('Ctrl Pts',(-50.,9.56651871386955,-0.886087649174329));
#42591=CARTESIAN_POINT('Ctrl Pts',(-66.,9.46528658437238,-0.9180359267008));
#42592=CARTESIAN_POINT('Ctrl Pts',(-50.,9.46528658437238,-0.9180359267008));
#42593=CARTESIAN_POINT('Ctrl Pts',(-66.,9.36383468209953,-0.946679483797828));
#42594=CARTESIAN_POINT('Ctrl Pts',(-50.,9.36383468209953,-0.946679483797828));
#42595=CARTESIAN_POINT('Ctrl Pts',(-66.,9.26220852393388,-0.971700897727075));
#42596=CARTESIAN_POINT('Ctrl Pts',(-50.,9.26220852393388,-0.971700897727075));
#42597=CARTESIAN_POINT('Ctrl Pts',(-66.,9.16048129971873,-0.992712229606096));
#42598=CARTESIAN_POINT('Ctrl Pts',(-50.,9.16048129971873,-0.992712229606096));
#42599=CARTESIAN_POINT('Ctrl Pts',(-66.,9.05876930477337,-1.00922949007046));
#42600=CARTESIAN_POINT('Ctrl Pts',(-50.,9.05876930477337,-1.00922949007046));
#42601=CARTESIAN_POINT('Ctrl Pts',(-66.,8.95721840904376,-1.02074993441888));
#42602=CARTESIAN_POINT('Ctrl Pts',(-50.,8.95721840904376,-1.02074993441888));
#42603=CARTESIAN_POINT('Ctrl Pts',(-66.,8.85597360323765,-1.02688738551608));
#42604=CARTESIAN_POINT('Ctrl Pts',(-50.,8.85597360323765,-1.02688738551608));
#42605=CARTESIAN_POINT('Ctrl Pts',(-66.,8.75515237563664,-1.02749863562185));
#42606=CARTESIAN_POINT('Ctrl Pts',(-50.,8.75515237563664,-1.02749863562185));
#42607=CARTESIAN_POINT('Ctrl Pts',(-66.,8.65481931169516,-1.0227982069947));
#42608=CARTESIAN_POINT('Ctrl Pts',(-50.,8.65481931169516,-1.0227982069947));
#42609=CARTESIAN_POINT('Ctrl Pts',(-66.,8.5549523562227,-1.01352414725572));
#42610=CARTESIAN_POINT('Ctrl Pts',(-50.,8.5549523562227,-1.01352414725572));
#42611=CARTESIAN_POINT('Ctrl Pts',(-66.,8.45545727626546,-1.00082385038912));
#42612=CARTESIAN_POINT('Ctrl Pts',(-50.,8.45545727626546,-1.00082385038912));
#42613=CARTESIAN_POINT('Ctrl Pts',(-66.,8.35619956862638,-0.986039820385861));
#42614=CARTESIAN_POINT('Ctrl Pts',(-50.,8.35619956862638,-0.986039820385861));
#42615=CARTESIAN_POINT('Ctrl Pts',(-66.,8.25703088282646,-0.970525968901249));
#42616=CARTESIAN_POINT('Ctrl Pts',(-50.,8.25703088282646,-0.970525968901249));
#42617=CARTESIAN_POINT('Ctrl Pts',(-66.,8.15781635562219,-0.955460858076408));
#42618=CARTESIAN_POINT('Ctrl Pts',(-50.,8.15781635562219,-0.955460858076408));
#42619=CARTESIAN_POINT('Ctrl Pts',(-66.,8.05846479644172,-0.94163789416019));
#42620=CARTESIAN_POINT('Ctrl Pts',(-50.,8.05846479644172,-0.94163789416019));
#42621=CARTESIAN_POINT('Ctrl Pts',(-66.,7.95892309714082,-0.92951996674881));
#42622=CARTESIAN_POINT('Ctrl Pts',(-50.,7.95892309714082,-0.92951996674881));
#42623=CARTESIAN_POINT('Ctrl Pts',(-66.,7.87911675845826,-0.921371110962998));
#42624=CARTESIAN_POINT('Ctrl Pts',(-50.,7.87911675845826,-0.921371110962998));
#42625=CARTESIAN_POINT('Ctrl Pts',(-66.,7.81916111326106,-0.916160028010783));
#42626=CARTESIAN_POINT('Ctrl Pts',(-50.,7.81916111326106,-0.916160028010783));
#42627=CARTESIAN_POINT('Ctrl Pts',(-66.,7.77914589672304,-0.913085729118069));
#42628=CARTESIAN_POINT('Ctrl Pts',(-50.,7.77914589672304,-0.913085729118069));
#42629=CARTESIAN_POINT('Ctrl Pts',(-66.,7.75912709216827,-0.911648516469152));
#42630=CARTESIAN_POINT('Ctrl Pts',(-50.,7.75912709216827,-0.911648516469152));
#42631=CARTESIAN_POINT('',(-65.5,10.6181350341134,-0.381881391708805));
#42632=CARTESIAN_POINT('Ctrl Pts',(-65.5,10.6181350341134,-0.381881391708781));
#42633=CARTESIAN_POINT('Ctrl Pts',(-65.5867229745674,10.529368555399,-0.437231194499219));
#42634=CARTESIAN_POINT('Ctrl Pts',(-65.6740389226617,10.4396220830013,-0.489919095176194));
#42635=CARTESIAN_POINT('Ctrl Pts',(-65.762054813772,10.3488859652185,-0.539750997576187));
#42636=CARTESIAN_POINT('Ctrl Pts',(-65.8407843210749,10.2677232370167,-0.584325233824076));
#42637=CARTESIAN_POINT('Ctrl Pts',(-65.9200738638956,10.1857705419182,-0.626610595896924));
#42638=CARTESIAN_POINT('Ctrl Pts',(-66.,10.1030411093822,-0.666472311603393));
#42639=CARTESIAN_POINT('',(-50.5,10.6181350341134,-0.381881391708805));
#42640=CARTESIAN_POINT('Ctrl Pts',(-50.5,10.6181350341134,-0.381881391708804));
#42641=CARTESIAN_POINT('Ctrl Pts',(-55.5,10.6181350341134,-0.381881391708804));
#42642=CARTESIAN_POINT('Ctrl Pts',(-60.5,10.6181350341134,-0.381881391708804));
#42643=CARTESIAN_POINT('Ctrl Pts',(-65.5,10.6181350341134,-0.381881391708804));
#42644=CARTESIAN_POINT('',(-50.,10.1030411093822,-0.666472311603383));
#42645=CARTESIAN_POINT('Ctrl Pts',(-50.,10.1030411093822,-0.666472311603383));
#42646=CARTESIAN_POINT('Ctrl Pts',(-50.1024673395144,10.2091023462276,-0.615368578131412));
#42647=CARTESIAN_POINT('Ctrl Pts',(-50.2038883811707,10.3138858386924,-0.560279576022463));
#42648=CARTESIAN_POINT('Ctrl Pts',(-50.3044244416113,10.4173674225829,-0.501495352008985));
#42649=CARTESIAN_POINT('Ctrl Pts',(-50.369977639336,10.4848412095995,-0.463165882533405));
#42650=CARTESIAN_POINT('Ctrl Pts',(-50.4351545856909,10.5517616293991,-0.423268128173657));
#42651=CARTESIAN_POINT('Ctrl Pts',(-50.5,10.6181350341134,-0.381881391708782));
#42652=CARTESIAN_POINT('Ctrl Pts',(-50.,10.1030411093822,-0.666472311603383));
#42653=CARTESIAN_POINT('Ctrl Pts',(-50.,10.0961259401211,-0.669804263759903));
#42654=CARTESIAN_POINT('Ctrl Pts',(-50.,10.0693164096302,-0.682658849179933));
#42655=CARTESIAN_POINT('Ctrl Pts',(-50.,10.022551212884,-0.704655396487715));
#42656=CARTESIAN_POINT('Ctrl Pts',(-50.,9.95571582676884,-0.735030406117662));
#42657=CARTESIAN_POINT('Ctrl Pts',(-50.,9.8686591303367,-0.772616048562836));
#42658=CARTESIAN_POINT('Ctrl Pts',(-50.,9.76822511794956,-0.813212594962941));
#42659=CARTESIAN_POINT('Ctrl Pts',(-50.,9.66750440467984,-0.851083007004113));
#42660=CARTESIAN_POINT('Ctrl Pts',(-50.,9.56651871386955,-0.886087649174329));
#42661=CARTESIAN_POINT('Ctrl Pts',(-50.,9.46528658437238,-0.9180359267008));
#42662=CARTESIAN_POINT('Ctrl Pts',(-50.,9.36383468209953,-0.946679483797828));
#42663=CARTESIAN_POINT('Ctrl Pts',(-50.,9.26220852393388,-0.971700897727075));
#42664=CARTESIAN_POINT('Ctrl Pts',(-50.,9.16048129971873,-0.992712229606096));
#42665=CARTESIAN_POINT('Ctrl Pts',(-50.,9.05876930477337,-1.00922949007046));
#42666=CARTESIAN_POINT('Ctrl Pts',(-50.,8.95721840904376,-1.02074993441888));
#42667=CARTESIAN_POINT('Ctrl Pts',(-50.,8.85597360323765,-1.02688738551608));
#42668=CARTESIAN_POINT('Ctrl Pts',(-50.,8.75515237563664,-1.02749863562185));
#42669=CARTESIAN_POINT('Ctrl Pts',(-50.,8.65481931169516,-1.0227982069947));
#42670=CARTESIAN_POINT('Ctrl Pts',(-50.,8.5549523562227,-1.01352414725572));
#42671=CARTESIAN_POINT('Ctrl Pts',(-50.,8.45545727626546,-1.00082385038912));
#42672=CARTESIAN_POINT('Ctrl Pts',(-50.,8.35619956862638,-0.986039820385861));
#42673=CARTESIAN_POINT('Ctrl Pts',(-50.,8.25703088282646,-0.970525968901249));
#42674=CARTESIAN_POINT('Ctrl Pts',(-50.,8.15781635562219,-0.955460858076408));
#42675=CARTESIAN_POINT('Ctrl Pts',(-50.,8.05846479644172,-0.94163789416019));
#42676=CARTESIAN_POINT('Ctrl Pts',(-50.,7.95892309714082,-0.92951996674881));
#42677=CARTESIAN_POINT('Ctrl Pts',(-50.,7.87911675845826,-0.921371110962998));
#42678=CARTESIAN_POINT('Ctrl Pts',(-50.,7.81916111326106,-0.916160028010783));
#42679=CARTESIAN_POINT('Ctrl Pts',(-50.,7.77914589672304,-0.913085729118069));
#42680=CARTESIAN_POINT('Ctrl Pts',(-50.,7.75912709216827,-0.911648516469152));
#42681=CARTESIAN_POINT('Origin',(-50.,9.38757796099391,-1.49533175231994));
#42682=CARTESIAN_POINT('Origin',(-50.,0.,0.));
#42683=CARTESIAN_POINT('Origin',(-65.75,0.,0.));
#42684=CARTESIAN_POINT('',(-65.5,9.54482387373331,-4.66765061025465));
#42685=CARTESIAN_POINT('Origin',(-65.5,0.,0.));
#42686=CARTESIAN_POINT('',(-66.,8.95850860312801,-4.71812977859675));
#42687=CARTESIAN_POINT('Ctrl Pts',(-65.5,9.54482387373331,-4.66765061025465));
#42688=CARTESIAN_POINT('Ctrl Pts',(-65.6642917360004,9.34854280324816,-4.69504523834513));
#42689=CARTESIAN_POINT('Ctrl Pts',(-65.8311182354841,9.15245906265275,-4.71228445517344));
#42690=CARTESIAN_POINT('Ctrl Pts',(-66.,8.95850860312801,-4.71812977859675));
#42691=CARTESIAN_POINT('Origin',(-66.,0.,0.));
#42692=CARTESIAN_POINT('Origin',(-65.75,0.,0.));
#42693=CARTESIAN_POINT('',(-66.,10.1021455355716,0.67991218413181));
#42694=CARTESIAN_POINT('Origin',(-66.,0.,0.));
#42695=CARTESIAN_POINT('',(-65.5,10.6195213806306,0.341160733863857));
#42696=CARTESIAN_POINT('Ctrl Pts',(-66.,10.1021455355716,0.679912184131811));
#42697=CARTESIAN_POINT('Ctrl Pts',(-65.798241770306,10.3119618818526,0.566966436117564));
#42698=CARTESIAN_POINT('Ctrl Pts',(-65.6331946192801,10.4841148496301,0.407873338586525));
#42699=CARTESIAN_POINT('Ctrl Pts',(-65.5,10.6195213806305,0.34116073386386));
#42700=CARTESIAN_POINT('Origin',(-65.5,0.,0.));
#42701=CARTESIAN_POINT('Origin',(-58.,0.,0.));
#42702=CARTESIAN_POINT('',(-50.5,9.54482387373331,-4.66765061025465));
#42703=CARTESIAN_POINT('Origin',(-50.5,0.,0.));
#42704=CARTESIAN_POINT('Ctrl Pts',(-50.5,9.54482387373331,-4.66765061025465));
#42705=CARTESIAN_POINT('Ctrl Pts',(-55.5,9.54482387373331,-4.66765061025465));
#42706=CARTESIAN_POINT('Ctrl Pts',(-60.5,9.54482387373331,-4.66765061025465));
#42707=CARTESIAN_POINT('Ctrl Pts',(-65.5,9.54482387373331,-4.66765061025465));
#42708=CARTESIAN_POINT('Origin',(-50.25,0.,0.));
#42709=CARTESIAN_POINT('',(-50.,8.95850860312803,-4.71812977859675));
#42710=CARTESIAN_POINT('Origin',(-50.,0.,0.));
#42711=CARTESIAN_POINT('Ctrl Pts',(-50.,8.95850860312803,-4.71812977859675));
#42712=CARTESIAN_POINT('Ctrl Pts',(-50.1688817645162,9.15245906265309,-4.71228445517342));
#42713=CARTESIAN_POINT('Ctrl Pts',(-50.3357082639999,9.34854280324851,-4.69504523834508));
#42714=CARTESIAN_POINT('Ctrl Pts',(-50.5,9.54482387373333,-4.66765061025465));
#42715=CARTESIAN_POINT('Origin',(-66.,7.96777298730851,-5.18432547646766));
#42716=CARTESIAN_POINT('',(-66.,7.26492798915904,-7.0524071289407));
#42717=CARTESIAN_POINT('Origin',(-66.,0.,0.));
#42718=CARTESIAN_POINT('',(-66.,6.71751445306826,-3.98875366785403));
#42719=CARTESIAN_POINT('Ctrl Pts',(-66.,6.71751445306827,-3.98875366785402));
#42720=CARTESIAN_POINT('Ctrl Pts',(-66.,6.73521797398851,-3.99820900830411));
#42721=CARTESIAN_POINT('Ctrl Pts',(-66.,6.77052326328196,-4.01729317493961));
#42722=CARTESIAN_POINT('Ctrl Pts',(-66.,6.82317593222513,-4.04643989396096));
#42723=CARTESIAN_POINT('Ctrl Pts',(-66.,6.89276821217244,-4.08634440644098));
#42724=CARTESIAN_POINT('Ctrl Pts',(-66.,6.97877527429846,-4.1379019406034));
#42725=CARTESIAN_POINT('Ctrl Pts',(-66.,7.06391513395684,-4.19093976616563));
#42726=CARTESIAN_POINT('Ctrl Pts',(-66.,7.148424582012,-4.24505661346796));
#42727=CARTESIAN_POINT('Ctrl Pts',(-66.,7.23270963259088,-4.29956476038277));
#42728=CARTESIAN_POINT('Ctrl Pts',(-66.,7.31737285380592,-4.35344239064242));
#42729=CARTESIAN_POINT('Ctrl Pts',(-66.,7.40310045604506,-4.40551298397998));
#42730=CARTESIAN_POINT('Ctrl Pts',(-66.,7.4905613596596,-4.4546048093515));
#42731=CARTESIAN_POINT('Ctrl Pts',(-66.,7.58030833791389,-4.49970799818987));
#42732=CARTESIAN_POINT('Ctrl Pts',(-66.,7.67266173023884,-4.54015728109748));
#42733=CARTESIAN_POINT('Ctrl Pts',(-66.,7.76764978894924,-4.57573041296856));
#42734=CARTESIAN_POINT('Ctrl Pts',(-66.,7.86510693532357,-4.60651043379445));
#42735=CARTESIAN_POINT('Ctrl Pts',(-66.,7.96474364136776,-4.63279116090914));
#42736=CARTESIAN_POINT('Ctrl Pts',(-66.,8.06622216356313,-4.65497254379874));
#42737=CARTESIAN_POINT('Ctrl Pts',(-66.,8.16923940463961,-4.67344942718086));
#42738=CARTESIAN_POINT('Ctrl Pts',(-66.,8.27357071338958,-4.68854644186826));
#42739=CARTESIAN_POINT('Ctrl Pts',(-66.,8.37904540061237,-4.70053505457754));
#42740=CARTESIAN_POINT('Ctrl Pts',(-66.,8.48553809038739,-4.7096313036054));
#42741=CARTESIAN_POINT('Ctrl Pts',(-66.,8.59295432475099,-4.71600176550966));
#42742=CARTESIAN_POINT('Ctrl Pts',(-66.,8.70121746356333,-4.71976516799885));
#42743=CARTESIAN_POINT('Ctrl Pts',(-66.,8.79603517118228,-4.72083812353456));
#42744=CARTESIAN_POINT('Ctrl Pts',(-66.,8.86944696402783,-4.72027357204841));
#42745=CARTESIAN_POINT('Ctrl Pts',(-66.,8.92111589890229,-4.71919984530889));
#42746=CARTESIAN_POINT('Ctrl Pts',(-66.,8.95083605462571,-4.71836101562288));
#42747=CARTESIAN_POINT('Ctrl Pts',(-66.,8.95850860312801,-4.71812977859675));
#42748=CARTESIAN_POINT('',(-66.,5.86935629366618,-5.15614322415516));
#42749=CARTESIAN_POINT('Origin',(-66.,0.,0.));
#42750=CARTESIAN_POINT('Ctrl Pts',(-66.,7.26492798915904,-7.0524071289407));
#42751=CARTESIAN_POINT('Ctrl Pts',(-66.,7.26021532815457,-7.03308392699787));
#42752=CARTESIAN_POINT('Ctrl Pts',(-66.,7.24842825534665,-6.98804444224892));
#42753=CARTESIAN_POINT('Ctrl Pts',(-66.,7.227595031479,-6.91993074698252));
#42754=CARTESIAN_POINT('Ctrl Pts',(-66.,7.19484476532416,-6.83244868977223));
#42755=CARTESIAN_POINT('Ctrl Pts',(-66.,7.14848549892204,-6.72694193164882));
#42756=CARTESIAN_POINT('Ctrl Pts',(-66.,7.09744125739136,-6.6158281439859));
#42757=CARTESIAN_POINT('Ctrl Pts',(-66.,7.04604577435704,-6.50233218649336));
#42758=CARTESIAN_POINT('Ctrl Pts',(-66.,6.99384114124033,-6.38708538288662));
#42759=CARTESIAN_POINT('Ctrl Pts',(-66.,6.93931235010921,-6.27244686141061));
#42760=CARTESIAN_POINT('Ctrl Pts',(-66.,6.88051534847335,-6.16149248844613));
#42761=CARTESIAN_POINT('Ctrl Pts',(-66.,6.81598023271187,-6.05654989646995));
#42762=CARTESIAN_POINT('Ctrl Pts',(-66.,6.74517942479359,-5.95845844019316));
#42763=CARTESIAN_POINT('Ctrl Pts',(-66.,6.66825702244228,-5.86706979565036));
#42764=CARTESIAN_POINT('Ctrl Pts',(-66.,6.58590972047863,-5.78148954312863));
#42765=CARTESIAN_POINT('Ctrl Pts',(-66.,6.49921187544537,-5.70042712110381));
#42766=CARTESIAN_POINT('Ctrl Pts',(-66.,6.40946643235469,-5.62246337987595));
#42767=CARTESIAN_POINT('Ctrl Pts',(-66.,6.31803612319428,-5.54618047286195));
#42768=CARTESIAN_POINT('Ctrl Pts',(-66.,6.22618517207396,-5.47030266626172));
#42769=CARTESIAN_POINT('Ctrl Pts',(-66.,6.13490846544372,-5.39384099594422));
#42770=CARTESIAN_POINT('Ctrl Pts',(-66.,6.04478817168633,-5.31621635935271));
#42771=CARTESIAN_POINT('Ctrl Pts',(-66.,5.97384780075134,-5.25295689440918));
#42772=CARTESIAN_POINT('Ctrl Pts',(-66.,5.92133360577774,-5.20481925752974));
#42773=CARTESIAN_POINT('Ctrl Pts',(-66.,5.88663093438999,-5.17241984284373));
#42774=CARTESIAN_POINT('Ctrl Pts',(-66.,5.86935629366618,-5.15614322415516));
#42775=CARTESIAN_POINT('Ctrl Pts',(-66.,5.86935629366618,-5.15614322415516));
#42776=CARTESIAN_POINT('Ctrl Pts',(-50.,5.86935629366618,-5.15614322415516));
#42777=CARTESIAN_POINT('Ctrl Pts',(-66.,5.88663093438999,-5.17241984284373));
#42778=CARTESIAN_POINT('Ctrl Pts',(-50.,5.88663093438999,-5.17241984284373));
#42779=CARTESIAN_POINT('Ctrl Pts',(-66.,5.92133360577774,-5.20481925752974));
#42780=CARTESIAN_POINT('Ctrl Pts',(-50.,5.92133360577774,-5.20481925752974));
#42781=CARTESIAN_POINT('Ctrl Pts',(-66.,5.97384780075134,-5.25295689440918));
#42782=CARTESIAN_POINT('Ctrl Pts',(-50.,5.97384780075134,-5.25295689440918));
#42783=CARTESIAN_POINT('Ctrl Pts',(-66.,6.04478817168633,-5.31621635935271));
#42784=CARTESIAN_POINT('Ctrl Pts',(-50.,6.04478817168633,-5.31621635935271));
#42785=CARTESIAN_POINT('Ctrl Pts',(-66.,6.13490846544372,-5.39384099594422));
#42786=CARTESIAN_POINT('Ctrl Pts',(-50.,6.13490846544372,-5.39384099594422));
#42787=CARTESIAN_POINT('Ctrl Pts',(-66.,6.22618517207396,-5.47030266626172));
#42788=CARTESIAN_POINT('Ctrl Pts',(-50.,6.22618517207396,-5.47030266626172));
#42789=CARTESIAN_POINT('Ctrl Pts',(-66.,6.31803612319428,-5.54618047286195));
#42790=CARTESIAN_POINT('Ctrl Pts',(-50.,6.31803612319428,-5.54618047286195));
#42791=CARTESIAN_POINT('Ctrl Pts',(-66.,6.40946643235469,-5.62246337987595));
#42792=CARTESIAN_POINT('Ctrl Pts',(-50.,6.40946643235469,-5.62246337987595));
#42793=CARTESIAN_POINT('Ctrl Pts',(-66.,6.49921187544537,-5.70042712110381));
#42794=CARTESIAN_POINT('Ctrl Pts',(-50.,6.49921187544537,-5.70042712110381));
#42795=CARTESIAN_POINT('Ctrl Pts',(-66.,6.58590972047863,-5.78148954312863));
#42796=CARTESIAN_POINT('Ctrl Pts',(-50.,6.58590972047863,-5.78148954312863));
#42797=CARTESIAN_POINT('Ctrl Pts',(-66.,6.66825702244228,-5.86706979565036));
#42798=CARTESIAN_POINT('Ctrl Pts',(-50.,6.66825702244228,-5.86706979565036));
#42799=CARTESIAN_POINT('Ctrl Pts',(-66.,6.74517942479359,-5.95845844019316));
#42800=CARTESIAN_POINT('Ctrl Pts',(-50.,6.74517942479359,-5.95845844019316));
#42801=CARTESIAN_POINT('Ctrl Pts',(-66.,6.81598023271187,-6.05654989646995));
#42802=CARTESIAN_POINT('Ctrl Pts',(-50.,6.81598023271187,-6.05654989646995));
#42803=CARTESIAN_POINT('Ctrl Pts',(-66.,6.88051534847335,-6.16149248844613));
#42804=CARTESIAN_POINT('Ctrl Pts',(-50.,6.88051534847335,-6.16149248844613));
#42805=CARTESIAN_POINT('Ctrl Pts',(-66.,6.93931235010921,-6.27244686141061));
#42806=CARTESIAN_POINT('Ctrl Pts',(-50.,6.93931235010921,-6.27244686141061));
#42807=CARTESIAN_POINT('Ctrl Pts',(-66.,6.99384114124033,-6.38708538288662));
#42808=CARTESIAN_POINT('Ctrl Pts',(-50.,6.99384114124033,-6.38708538288662));
#42809=CARTESIAN_POINT('Ctrl Pts',(-66.,7.04604577435704,-6.50233218649336));
#42810=CARTESIAN_POINT('Ctrl Pts',(-50.,7.04604577435704,-6.50233218649336));
#42811=CARTESIAN_POINT('Ctrl Pts',(-66.,7.09744125739136,-6.6158281439859));
#42812=CARTESIAN_POINT('Ctrl Pts',(-50.,7.09744125739136,-6.6158281439859));
#42813=CARTESIAN_POINT('Ctrl Pts',(-66.,7.14848549892204,-6.72694193164882));
#42814=CARTESIAN_POINT('Ctrl Pts',(-50.,7.14848549892204,-6.72694193164882));
#42815=CARTESIAN_POINT('Ctrl Pts',(-66.,7.19750768890132,-6.83850910564074));
#42816=CARTESIAN_POINT('Ctrl Pts',(-50.,7.19750768890132,-6.83850910564074));
#42817=CARTESIAN_POINT('Ctrl Pts',(-66.,7.24105605777582,-6.95624670358752));
#42818=CARTESIAN_POINT('Ctrl Pts',(-50.,7.24105605777582,-6.95624670358752));
#42819=CARTESIAN_POINT('Ctrl Pts',(-66.,7.27589395606278,-7.08546826867055));
#42820=CARTESIAN_POINT('Ctrl Pts',(-50.,7.27589395606278,-7.08546826867055));
#42821=CARTESIAN_POINT('Ctrl Pts',(-66.,7.30047061843489,-7.22866076209231));
#42822=CARTESIAN_POINT('Ctrl Pts',(-50.,7.30047061843489,-7.22866076209231));
#42823=CARTESIAN_POINT('Ctrl Pts',(-66.,7.31682601848242,-7.38234648021868));
#42824=CARTESIAN_POINT('Ctrl Pts',(-50.,7.31682601848242,-7.38234648021868));
#42825=CARTESIAN_POINT('Ctrl Pts',(-66.,7.33168909251117,-7.53527793402804));
#42826=CARTESIAN_POINT('Ctrl Pts',(-50.,7.33168909251117,-7.53527793402804));
#42827=CARTESIAN_POINT('Ctrl Pts',(-66.,7.35454896062522,-7.67163921895471));
#42828=CARTESIAN_POINT('Ctrl Pts',(-50.,7.35454896062522,-7.67163921895471));
#42829=CARTESIAN_POINT('Ctrl Pts',(-66.,7.39614403501135,-7.77355664342129));
#42830=CARTESIAN_POINT('Ctrl Pts',(-50.,7.39614403501135,-7.77355664342129));
#42831=CARTESIAN_POINT('Ctrl Pts',(-66.,7.46685648222862,-7.82376555763565));
#42832=CARTESIAN_POINT('Ctrl Pts',(-50.,7.46685648222862,-7.82376555763565));
#42833=CARTESIAN_POINT('Ctrl Pts',(-66.,7.57499098914986,-7.80847073788432));
#42834=CARTESIAN_POINT('Ctrl Pts',(-50.,7.57499098914986,-7.80847073788432));
#42835=CARTESIAN_POINT('Ctrl Pts',(-66.,7.72686051941396,-7.71719997015535));
#42836=CARTESIAN_POINT('Ctrl Pts',(-50.,7.72686051941396,-7.71719997015535));
#42837=CARTESIAN_POINT('Ctrl Pts',(-66.,7.9271282162934,-7.54223184193065));
#42838=CARTESIAN_POINT('Ctrl Pts',(-50.,7.9271282162934,-7.54223184193065));
#42839=CARTESIAN_POINT('Ctrl Pts',(-66.,8.17904362913404,-7.27819961164743));
#42840=CARTESIAN_POINT('Ctrl Pts',(-50.,8.17904362913404,-7.27819961164743));
#42841=CARTESIAN_POINT('Ctrl Pts',(-66.,8.48470956289165,-6.92164441889879));
#42842=CARTESIAN_POINT('Ctrl Pts',(-50.,8.48470956289165,-6.92164441889879));
#42843=CARTESIAN_POINT('Ctrl Pts',(-66.,8.84532275927927,-6.47061228740683));
#42844=CARTESIAN_POINT('Ctrl Pts',(-50.,8.84532275927927,-6.47061228740683));
#42845=CARTESIAN_POINT('Ctrl Pts',(-66.,9.26141395607925,-5.92425241274213));
#42846=CARTESIAN_POINT('Ctrl Pts',(-50.,9.26141395607925,-5.92425241274213));
#42847=CARTESIAN_POINT('Ctrl Pts',(-66.,9.63874478953592,-5.41079693734509));
#42848=CARTESIAN_POINT('Ctrl Pts',(-50.,9.63874478953592,-5.41079693734509));
#42849=CARTESIAN_POINT('Ctrl Pts',(-66.,9.94669765021079,-4.98284383425478));
#42850=CARTESIAN_POINT('Ctrl Pts',(-50.,9.94669765021079,-4.98284383425478));
#42851=CARTESIAN_POINT('Ctrl Pts',(-66.,10.1630758067952,-4.67851753531735));
#42852=CARTESIAN_POINT('Ctrl Pts',(-50.,10.1630758067952,-4.67851753531735));
#42853=CARTESIAN_POINT('Ctrl Pts',(-66.,10.2740339482513,-4.52159832693919));
#42854=CARTESIAN_POINT('Ctrl Pts',(-50.,10.2740339482513,-4.52159832693919));
#42855=CARTESIAN_POINT('',(-65.5,7.35937861468917,-7.663561274346));
#42856=CARTESIAN_POINT('Ctrl Pts',(-66.,7.26492798915904,-7.0524071289407));
#42857=CARTESIAN_POINT('Ctrl Pts',(-65.7982417703062,7.32138747997352,-7.28390651783422));
#42858=CARTESIAN_POINT('Ctrl Pts',(-65.6331946192802,7.31835108748961,-7.51829516584718));
#42859=CARTESIAN_POINT('Ctrl Pts',(-65.5,7.35937861468917,-7.66356127434599));
#42860=CARTESIAN_POINT('',(-50.,5.86935629366618,-5.15614322415516));
#42861=CARTESIAN_POINT('',(-66.,5.86935629366618,-5.15614322415516));
#42862=CARTESIAN_POINT('',(-50.,7.26492798915904,-7.05240712894072));
#42863=CARTESIAN_POINT('Ctrl Pts',(-50.,5.86935629366618,-5.15614322415516));
#42864=CARTESIAN_POINT('Ctrl Pts',(-50.,5.88663093438999,-5.17241984284373));
#42865=CARTESIAN_POINT('Ctrl Pts',(-50.,5.92133360577774,-5.20481925752974));
#42866=CARTESIAN_POINT('Ctrl Pts',(-50.,5.97384780075134,-5.25295689440918));
#42867=CARTESIAN_POINT('Ctrl Pts',(-50.,6.04478817168633,-5.31621635935271));
#42868=CARTESIAN_POINT('Ctrl Pts',(-50.,6.13490846544372,-5.39384099594422));
#42869=CARTESIAN_POINT('Ctrl Pts',(-50.,6.22618517207396,-5.47030266626172));
#42870=CARTESIAN_POINT('Ctrl Pts',(-50.,6.31803612319428,-5.54618047286195));
#42871=CARTESIAN_POINT('Ctrl Pts',(-50.,6.40946643235469,-5.62246337987595));
#42872=CARTESIAN_POINT('Ctrl Pts',(-50.,6.49921187544537,-5.70042712110381));
#42873=CARTESIAN_POINT('Ctrl Pts',(-50.,6.58590972047863,-5.78148954312863));
#42874=CARTESIAN_POINT('Ctrl Pts',(-50.,6.66825702244228,-5.86706979565036));
#42875=CARTESIAN_POINT('Ctrl Pts',(-50.,6.74517942479359,-5.95845844019316));
#42876=CARTESIAN_POINT('Ctrl Pts',(-50.,6.81598023271187,-6.05654989646995));
#42877=CARTESIAN_POINT('Ctrl Pts',(-50.,6.88051534847335,-6.16149248844613));
#42878=CARTESIAN_POINT('Ctrl Pts',(-50.,6.93931235010921,-6.27244686141061));
#42879=CARTESIAN_POINT('Ctrl Pts',(-50.,6.99384114124033,-6.38708538288662));
#42880=CARTESIAN_POINT('Ctrl Pts',(-50.,7.04604577435704,-6.50233218649336));
#42881=CARTESIAN_POINT('Ctrl Pts',(-50.,7.09744125739136,-6.6158281439859));
#42882=CARTESIAN_POINT('Ctrl Pts',(-50.,7.14848549892204,-6.72694193164882));
#42883=CARTESIAN_POINT('Ctrl Pts',(-50.,7.19484476532416,-6.83244868977223));
#42884=CARTESIAN_POINT('Ctrl Pts',(-50.,7.227595031479,-6.91993074698252));
#42885=CARTESIAN_POINT('Ctrl Pts',(-50.,7.24842825534666,-6.98804444224893));
#42886=CARTESIAN_POINT('Ctrl Pts',(-50.,7.26021532815457,-7.03308392699788));
#42887=CARTESIAN_POINT('Ctrl Pts',(-50.,7.26492798915904,-7.05240712894072));
#42888=CARTESIAN_POINT('',(-50.5,7.35937861468917,-7.663561274346));
#42889=CARTESIAN_POINT('Ctrl Pts',(-50.5,7.35937861468918,-7.66356127434601));
#42890=CARTESIAN_POINT('Ctrl Pts',(-50.4982567069799,7.35884163352443,-7.66165998588276));
#42891=CARTESIAN_POINT('Ctrl Pts',(-50.4965113438759,7.35831276186704,-7.65974787059353));
#42892=CARTESIAN_POINT('Ctrl Pts',(-50.3581212730773,7.31704604215131,-7.50748036478051));
#42893=CARTESIAN_POINT('Ctrl Pts',(-50.2022201285457,7.32151673652989,-7.28443650514684));
#42894=CARTESIAN_POINT('Ctrl Pts',(-50.,7.26492798915904,-7.05240712894072));
#42895=CARTESIAN_POINT('Ctrl Pts',(-65.5,7.35937861468917,-7.663561274346));
#42896=CARTESIAN_POINT('Ctrl Pts',(-60.5,7.35937861468917,-7.663561274346));
#42897=CARTESIAN_POINT('Ctrl Pts',(-55.5,7.35937861468917,-7.663561274346));
#42898=CARTESIAN_POINT('Ctrl Pts',(-50.5,7.35937861468917,-7.663561274346));
#42899=CARTESIAN_POINT('Origin',(-66.,0.,0.));
#42900=CARTESIAN_POINT('',(-50.,6.71751445306826,-3.98875366785403));
#42901=CARTESIAN_POINT('',(-66.,6.71751445306826,-3.98875366785403));
#42902=CARTESIAN_POINT('Origin',(-50.,0.,0.));
#42903=CARTESIAN_POINT('Ctrl Pts',(-66.,10.2740339482513,-4.52159832693919));
#42904=CARTESIAN_POINT('Ctrl Pts',(-50.,10.2740339482513,-4.52159832693919));
#42905=CARTESIAN_POINT('Ctrl Pts',(-66.,10.2510999230073,-4.527534516881));
#42906=CARTESIAN_POINT('Ctrl Pts',(-50.,10.2510999230073,-4.527534516881));
#42907=CARTESIAN_POINT('Ctrl Pts',(-66.,10.2052563445341,-4.53919480308192));
#42908=CARTESIAN_POINT('Ctrl Pts',(-50.,10.2052563445341,-4.53919480308192));
#42909=CARTESIAN_POINT('Ctrl Pts',(-66.,10.1365643931213,-4.55604895138109));
#42910=CARTESIAN_POINT('Ctrl Pts',(-50.,10.1365643931213,-4.55604895138109));
#42911=CARTESIAN_POINT('Ctrl Pts',(-66.,10.0451221502067,-4.57724689443403));
#42912=CARTESIAN_POINT('Ctrl Pts',(-50.,10.0451221502067,-4.57724689443403));
#42913=CARTESIAN_POINT('Ctrl Pts',(-66.,9.93106794944591,-4.60160822677996));
#42914=CARTESIAN_POINT('Ctrl Pts',(-50.,9.93106794944591,-4.60160822677996));
#42915=CARTESIAN_POINT('Ctrl Pts',(-66.,9.81727102696474,-4.62381353637928));
#42916=CARTESIAN_POINT('Ctrl Pts',(-50.,9.81727102696474,-4.62381353637928));
#42917=CARTESIAN_POINT('Ctrl Pts',(-66.,9.70374733588469,-4.64383593785917));
#42918=CARTESIAN_POINT('Ctrl Pts',(-50.,9.70374733588469,-4.64383593785917));
#42919=CARTESIAN_POINT('Ctrl Pts',(-66.,9.59052199725138,-4.66164245653247));
#42920=CARTESIAN_POINT('Ctrl Pts',(-50.,9.59052199725138,-4.66164245653247));
#42921=CARTESIAN_POINT('Ctrl Pts',(-66.,9.47763191152479,-4.67719483186143));
#42922=CARTESIAN_POINT('Ctrl Pts',(-50.,9.47763191152479,-4.67719483186143));
#42923=CARTESIAN_POINT('Ctrl Pts',(-66.,9.36512376791676,-4.69045181654785));
#42924=CARTESIAN_POINT('Ctrl Pts',(-50.,9.36512376791676,-4.69045181654785));
#42925=CARTESIAN_POINT('Ctrl Pts',(-66.,9.25305096656076,-4.70137178004192));
#42926=CARTESIAN_POINT('Ctrl Pts',(-50.,9.25305096656076,-4.70137178004192));
#42927=CARTESIAN_POINT('Ctrl Pts',(-66.,9.14147076691866,-4.7099158350055));
#42928=CARTESIAN_POINT('Ctrl Pts',(-50.,9.14147076691866,-4.7099158350055));
#42929=CARTESIAN_POINT('Ctrl Pts',(-66.,9.03044163684364,-4.7160501820886));
#42930=CARTESIAN_POINT('Ctrl Pts',(-50.,9.03044163684364,-4.7160501820886));
#42931=CARTESIAN_POINT('Ctrl Pts',(-66.,8.92001966569546,-4.71975123090547));
#42932=CARTESIAN_POINT('Ctrl Pts',(-50.,8.92001966569546,-4.71975123090547));
#42933=CARTESIAN_POINT('Ctrl Pts',(-66.,8.81025944656715,-4.72099908518823));
#42934=CARTESIAN_POINT('Ctrl Pts',(-50.,8.81025944656715,-4.72099908518823));
#42935=CARTESIAN_POINT('Ctrl Pts',(-66.,8.70121746356333,-4.71976516799885));
#42936=CARTESIAN_POINT('Ctrl Pts',(-50.,8.70121746356333,-4.71976516799885));
#42937=CARTESIAN_POINT('Ctrl Pts',(-66.,8.59295432475099,-4.71600176550966));
#42938=CARTESIAN_POINT('Ctrl Pts',(-50.,8.59295432475099,-4.71600176550966));
#42939=CARTESIAN_POINT('Ctrl Pts',(-66.,8.48553809038739,-4.7096313036054));
#42940=CARTESIAN_POINT('Ctrl Pts',(-50.,8.48553809038739,-4.7096313036054));
#42941=CARTESIAN_POINT('Ctrl Pts',(-66.,8.37904540061237,-4.70053505457754));
#42942=CARTESIAN_POINT('Ctrl Pts',(-50.,8.37904540061237,-4.70053505457754));
#42943=CARTESIAN_POINT('Ctrl Pts',(-66.,8.27357071338958,-4.68854644186826));
#42944=CARTESIAN_POINT('Ctrl Pts',(-50.,8.27357071338958,-4.68854644186826));
#42945=CARTESIAN_POINT('Ctrl Pts',(-66.,8.16923940463961,-4.67344942718086));
#42946=CARTESIAN_POINT('Ctrl Pts',(-50.,8.16923940463961,-4.67344942718086));
#42947=CARTESIAN_POINT('Ctrl Pts',(-66.,8.06622216356313,-4.65497254379874));
#42948=CARTESIAN_POINT('Ctrl Pts',(-50.,8.06622216356313,-4.65497254379874));
#42949=CARTESIAN_POINT('Ctrl Pts',(-66.,7.96474364136776,-4.63279116090914));
#42950=CARTESIAN_POINT('Ctrl Pts',(-50.,7.96474364136776,-4.63279116090914));
#42951=CARTESIAN_POINT('Ctrl Pts',(-66.,7.86510693532357,-4.60651043379445));
#42952=CARTESIAN_POINT('Ctrl Pts',(-50.,7.86510693532357,-4.60651043379445));
#42953=CARTESIAN_POINT('Ctrl Pts',(-66.,7.76764978894924,-4.57573041296856));
#42954=CARTESIAN_POINT('Ctrl Pts',(-50.,7.76764978894924,-4.57573041296856));
#42955=CARTESIAN_POINT('Ctrl Pts',(-66.,7.67266173023884,-4.54015728109748));
#42956=CARTESIAN_POINT('Ctrl Pts',(-50.,7.67266173023884,-4.54015728109748));
#42957=CARTESIAN_POINT('Ctrl Pts',(-66.,7.58030833791389,-4.49970799818987));
#42958=CARTESIAN_POINT('Ctrl Pts',(-50.,7.58030833791389,-4.49970799818987));
#42959=CARTESIAN_POINT('Ctrl Pts',(-66.,7.4905613596596,-4.4546048093515));
#42960=CARTESIAN_POINT('Ctrl Pts',(-50.,7.4905613596596,-4.4546048093515));
#42961=CARTESIAN_POINT('Ctrl Pts',(-66.,7.40310045604506,-4.40551298397998));
#42962=CARTESIAN_POINT('Ctrl Pts',(-50.,7.40310045604506,-4.40551298397998));
#42963=CARTESIAN_POINT('Ctrl Pts',(-66.,7.31737285380592,-4.35344239064242));
#42964=CARTESIAN_POINT('Ctrl Pts',(-50.,7.31737285380592,-4.35344239064242));
#42965=CARTESIAN_POINT('Ctrl Pts',(-66.,7.23270963259088,-4.29956476038277));
#42966=CARTESIAN_POINT('Ctrl Pts',(-50.,7.23270963259088,-4.29956476038277));
#42967=CARTESIAN_POINT('Ctrl Pts',(-66.,7.148424582012,-4.24505661346796));
#42968=CARTESIAN_POINT('Ctrl Pts',(-50.,7.148424582012,-4.24505661346796));
#42969=CARTESIAN_POINT('Ctrl Pts',(-66.,7.06391513395684,-4.19093976616563));
#42970=CARTESIAN_POINT('Ctrl Pts',(-50.,7.06391513395684,-4.19093976616563));
#42971=CARTESIAN_POINT('Ctrl Pts',(-66.,6.97877527429846,-4.1379019406034));
#42972=CARTESIAN_POINT('Ctrl Pts',(-50.,6.97877527429846,-4.1379019406034));
#42973=CARTESIAN_POINT('Ctrl Pts',(-66.,6.89276821217244,-4.08634440644098));
#42974=CARTESIAN_POINT('Ctrl Pts',(-50.,6.89276821217244,-4.08634440644098));
#42975=CARTESIAN_POINT('Ctrl Pts',(-66.,6.82317593222513,-4.04643989396096));
#42976=CARTESIAN_POINT('Ctrl Pts',(-50.,6.82317593222513,-4.04643989396096));
#42977=CARTESIAN_POINT('Ctrl Pts',(-66.,6.77052326328196,-4.01729317493961));
#42978=CARTESIAN_POINT('Ctrl Pts',(-50.,6.77052326328196,-4.01729317493961));
#42979=CARTESIAN_POINT('Ctrl Pts',(-66.,6.73521797398851,-3.99820900830411));
#42980=CARTESIAN_POINT('Ctrl Pts',(-50.,6.73521797398851,-3.99820900830411));
#42981=CARTESIAN_POINT('Ctrl Pts',(-66.,6.71751445306827,-3.98875366785402));
#42982=CARTESIAN_POINT('Ctrl Pts',(-50.,6.71751445306827,-3.98875366785402));
#42983=CARTESIAN_POINT('Ctrl Pts',(-50.,8.95850860312803,-4.71812977859675));
#42984=CARTESIAN_POINT('Ctrl Pts',(-50.,8.95083605462573,-4.71836101562288));
#42985=CARTESIAN_POINT('Ctrl Pts',(-50.,8.9211158989023,-4.71919984530889));
#42986=CARTESIAN_POINT('Ctrl Pts',(-50.,8.86944696402783,-4.72027357204841));
#42987=CARTESIAN_POINT('Ctrl Pts',(-50.,8.79603517118229,-4.72083812353456));
#42988=CARTESIAN_POINT('Ctrl Pts',(-50.,8.70121746356333,-4.71976516799885));
#42989=CARTESIAN_POINT('Ctrl Pts',(-50.,8.59295432475099,-4.71600176550966));
#42990=CARTESIAN_POINT('Ctrl Pts',(-50.,8.48553809038739,-4.7096313036054));
#42991=CARTESIAN_POINT('Ctrl Pts',(-50.,8.37904540061237,-4.70053505457754));
#42992=CARTESIAN_POINT('Ctrl Pts',(-50.,8.27357071338958,-4.68854644186826));
#42993=CARTESIAN_POINT('Ctrl Pts',(-50.,8.16923940463961,-4.67344942718086));
#42994=CARTESIAN_POINT('Ctrl Pts',(-50.,8.06622216356313,-4.65497254379874));
#42995=CARTESIAN_POINT('Ctrl Pts',(-50.,7.96474364136776,-4.63279116090914));
#42996=CARTESIAN_POINT('Ctrl Pts',(-50.,7.86510693532357,-4.60651043379445));
#42997=CARTESIAN_POINT('Ctrl Pts',(-50.,7.76764978894924,-4.57573041296856));
#42998=CARTESIAN_POINT('Ctrl Pts',(-50.,7.67266173023884,-4.54015728109748));
#42999=CARTESIAN_POINT('Ctrl Pts',(-50.,7.58030833791389,-4.49970799818987));
#43000=CARTESIAN_POINT('Ctrl Pts',(-50.,7.4905613596596,-4.4546048093515));
#43001=CARTESIAN_POINT('Ctrl Pts',(-50.,7.40310045604506,-4.40551298397998));
#43002=CARTESIAN_POINT('Ctrl Pts',(-50.,7.31737285380592,-4.35344239064242));
#43003=CARTESIAN_POINT('Ctrl Pts',(-50.,7.23270963259088,-4.29956476038277));
#43004=CARTESIAN_POINT('Ctrl Pts',(-50.,7.148424582012,-4.24505661346796));
#43005=CARTESIAN_POINT('Ctrl Pts',(-50.,7.06391513395684,-4.19093976616563));
#43006=CARTESIAN_POINT('Ctrl Pts',(-50.,6.97877527429846,-4.1379019406034));
#43007=CARTESIAN_POINT('Ctrl Pts',(-50.,6.89276821217244,-4.08634440644098));
#43008=CARTESIAN_POINT('Ctrl Pts',(-50.,6.82317593222513,-4.04643989396096));
#43009=CARTESIAN_POINT('Ctrl Pts',(-50.,6.77052326328196,-4.01729317493961));
#43010=CARTESIAN_POINT('Ctrl Pts',(-50.,6.73521797398851,-3.99820900830411));
#43011=CARTESIAN_POINT('Ctrl Pts',(-50.,6.71751445306827,-3.98875366785402));
#43012=CARTESIAN_POINT('Origin',(-50.,7.96777298730851,-5.18432547646766));
#43013=CARTESIAN_POINT('Origin',(-50.,0.,0.));
#43014=CARTESIAN_POINT('Origin',(-65.75,0.,0.));
#43015=CARTESIAN_POINT('',(-65.5,6.82112595358204,-8.14634063401289));
#43016=CARTESIAN_POINT('Origin',(-65.5,0.,0.));
#43017=CARTESIAN_POINT('',(-66.,6.26496857389735,-7.95397974400731));
#43018=CARTESIAN_POINT('Ctrl Pts',(-65.5,6.82112595358203,-8.14634063401289));
#43019=CARTESIAN_POINT('Ctrl Pts',(-65.6642917360004,6.6306718741513,-8.09153216836031));
#43020=CARTESIAN_POINT('Ctrl Pts',(-65.831118235484,6.44452864243079,-8.02752653417561));
#43021=CARTESIAN_POINT('Ctrl Pts',(-66.,6.26496857389735,-7.95397974400731));
#43022=CARTESIAN_POINT('Origin',(-66.,0.,0.));
#43023=CARTESIAN_POINT('Origin',(-58.,0.,0.));
#43024=CARTESIAN_POINT('',(-50.5,6.82112595358204,-8.14634063401289));
#43025=CARTESIAN_POINT('Origin',(-50.5,0.,0.));
#43026=CARTESIAN_POINT('Ctrl Pts',(-50.5,6.82112595358204,-8.14634063401289));
#43027=CARTESIAN_POINT('Ctrl Pts',(-55.5,6.82112595358204,-8.14634063401289));
#43028=CARTESIAN_POINT('Ctrl Pts',(-60.5,6.82112595358204,-8.14634063401289));
#43029=CARTESIAN_POINT('Ctrl Pts',(-65.5,6.82112595358204,-8.14634063401289));
#43030=CARTESIAN_POINT('Origin',(-50.25,0.,0.));
#43031=CARTESIAN_POINT('',(-50.,6.26496857389736,-7.95397974400732));
#43032=CARTESIAN_POINT('Origin',(-50.,0.,0.));
#43033=CARTESIAN_POINT('Ctrl Pts',(-50.,6.26496857389736,-7.95397974400732));
#43034=CARTESIAN_POINT('Ctrl Pts',(-50.168881764515,6.44452864242976,-8.02752653417518));
#43035=CARTESIAN_POINT('Ctrl Pts',(-50.3357082639993,6.63067187415095,-8.09153216836019));
#43036=CARTESIAN_POINT('Ctrl Pts',(-50.5,6.82112595358205,-8.14634063401289));
#43037=CARTESIAN_POINT('Origin',(-66.,5.1702676791723,-7.97690222761574));
#43038=CARTESIAN_POINT('',(-66.,3.76836956336765,-9.39760692058804));
#43039=CARTESIAN_POINT('Origin',(-66.,0.,0.));
#43040=CARTESIAN_POINT('',(-66.,4.5143825383298,-6.37616707337747));
#43041=CARTESIAN_POINT('Ctrl Pts',(-66.,4.51438253832981,-6.37616707337746));
#43042=CARTESIAN_POINT('Ctrl Pts',(-66.,4.52670967601697,-6.39200562736583));
#43043=CARTESIAN_POINT('Ctrl Pts',(-66.,4.55120043280854,-6.42379983595862));
#43044=CARTESIAN_POINT('Ctrl Pts',(-66.,4.58744600070291,-6.47184245854068));
#43045=CARTESIAN_POINT('Ctrl Pts',(-66.,4.63479108448607,-6.53660277498602));
#43046=CARTESIAN_POINT('Ctrl Pts',(-66.,4.69239210704599,-6.61868514985729));
#43047=CARTESIAN_POINT('Ctrl Pts',(-66.,4.74859881197601,-6.7017671151923));
#43048=CARTESIAN_POINT('Ctrl Pts',(-66.,4.80379072956909,-6.78557840443743));
#43049=CARTESIAN_POINT('Ctrl Pts',(-66.,4.85861849397619,-6.86965589298989));
#43050=CARTESIAN_POINT('Ctrl Pts',(-66.,4.91404818867789,-6.95331119177114));
#43051=CARTESIAN_POINT('Ctrl Pts',(-66.,4.97118523196097,-7.03574860294511));
#43052=CARTESIAN_POINT('Ctrl Pts',(-66.,5.03111729892527,-7.1161697713572));
#43053=CARTESIAN_POINT('Ctrl Pts',(-66.,5.09476012362649,-7.19387696930703));
#43054=CARTESIAN_POINT('Ctrl Pts',(-66.,5.16267694013817,-7.26839273674309));
#43055=CARTESIAN_POINT('Ctrl Pts',(-66.,5.23498395346241,-7.33952553391019));
#43056=CARTESIAN_POINT('Ctrl Pts',(-66.,5.31149612450297,-7.40728387468187));
#43057=CARTESIAN_POINT('Ctrl Pts',(-66.,5.39182944999988,-7.47181841290458));
#43058=CARTESIAN_POINT('Ctrl Pts',(-66.,5.47551271178446,-7.53335714794964));
#43059=CARTESIAN_POINT('Ctrl Pts',(-66.,5.5621084189074,-7.59213750764915));
#43060=CARTESIAN_POINT('Ctrl Pts',(-66.,5.65127930303142,-7.64836468312946));
#43061=CARTESIAN_POINT('Ctrl Pts',(-66.,5.74275901635157,-7.70221724602392));
#43062=CARTESIAN_POINT('Ctrl Pts',(-66.,5.83634515157351,-7.75384156215611));
#43063=CARTESIAN_POINT('Ctrl Pts',(-66.,5.93188366426367,-7.80335138726874));
#43064=CARTESIAN_POINT('Ctrl Pts',(-66.,6.02925624926082,-7.85082401216739));
#43065=CARTESIAN_POINT('Ctrl Pts',(-66.,6.11544012502743,-7.89037004192436));
#43066=CARTESIAN_POINT('Ctrl Pts',(-66.,6.18273475869519,-7.91971356466277));
#43067=CARTESIAN_POINT('Ctrl Pts',(-66.,6.2303734034606,-7.93974831559927));
#43068=CARTESIAN_POINT('Ctrl Pts',(-66.,6.25786529949277,-7.95107028292051));
#43069=CARTESIAN_POINT('Ctrl Pts',(-66.,6.26496857389735,-7.95397974400731));
#43070=CARTESIAN_POINT('',(-66.,3.26473139515385,-7.09765349728322));
#43071=CARTESIAN_POINT('Origin',(-66.,0.,0.));
#43072=CARTESIAN_POINT('Ctrl Pts',(-66.,3.76836956336765,-9.39760692058804));
#43073=CARTESIAN_POINT('Ctrl Pts',(-66.,3.77192378760531,-9.37803748530914));
#43074=CARTESIAN_POINT('Ctrl Pts',(-66.,3.77947496961539,-9.33209763417661));
#43075=CARTESIAN_POINT('Ctrl Pts',(-66.,3.78814720834319,-9.26139904172235));
#43076=CARTESIAN_POINT('Ctrl Pts',(-66.,3.79381050973993,-9.168159472417));
#43077=CARTESIAN_POINT('Ctrl Pts',(-66.,3.79437267711955,-9.05291824039091));
#43078=CARTESIAN_POINT('Ctrl Pts',(-66.,3.79293549112385,-8.93064918094144));
#43079=CARTESIAN_POINT('Ctrl Pts',(-66.,3.79214634580768,-8.8060610382747));
#43080=CARTESIAN_POINT('Ctrl Pts',(-66.,3.79133013838023,-8.67954430710504));
#43081=CARTESIAN_POINT('Ctrl Pts',(-66.,3.78814329632398,-8.5526379490841));
#43082=CARTESIAN_POINT('Ctrl Pts',(-66.,3.77955877175069,-8.42736119058854));
#43083=CARTESIAN_POINT('Ctrl Pts',(-66.,3.76328700746442,-8.30524256603013));
#43084=CARTESIAN_POINT('Ctrl Pts',(-66.,3.73850464063369,-8.18683427877518));
#43085=CARTESIAN_POINT('Ctrl Pts',(-66.,3.70540363987127,-8.07205943796329));
#43086=CARTESIAN_POINT('Ctrl Pts',(-66.,3.66498426083752,-7.96038432184111));
#43087=CARTESIAN_POINT('Ctrl Pts',(-66.,3.61875289573396,-7.85106692396409));
#43088=CARTESIAN_POINT('Ctrl Pts',(-66.,3.56847706424299,-7.74334074205051));
#43089=CARTESIAN_POINT('Ctrl Pts',(-66.,3.51597837414158,-7.63646478182881));
#43090=CARTESIAN_POINT('Ctrl Pts',(-66.,3.46293063930599,-7.52978780875129));
#43091=CARTESIAN_POINT('Ctrl Pts',(-66.,3.41064498168427,-7.42281101590317));
#43092=CARTESIAN_POINT('Ctrl Pts',(-66.,3.359888780788,-7.31524215598795));
#43093=CARTESIAN_POINT('Ctrl Pts',(-66.,3.32081146957076,-7.22859771080324));
#43094=CARTESIAN_POINT('Ctrl Pts',(-66.,3.29241670612082,-7.16326234391299));
#43095=CARTESIAN_POINT('Ctrl Pts',(-66.,3.27389226747348,-7.11954915773029));
#43096=CARTESIAN_POINT('Ctrl Pts',(-66.,3.26473139515385,-7.09765349728322));
#43097=CARTESIAN_POINT('Ctrl Pts',(-66.,3.26473139515385,-7.09765349728322));
#43098=CARTESIAN_POINT('Ctrl Pts',(-50.,3.26473139515385,-7.09765349728322));
#43099=CARTESIAN_POINT('Ctrl Pts',(-66.,3.27389226747348,-7.11954915773029));
#43100=CARTESIAN_POINT('Ctrl Pts',(-50.,3.27389226747348,-7.11954915773029));
#43101=CARTESIAN_POINT('Ctrl Pts',(-66.,3.29241670612082,-7.16326234391299));
#43102=CARTESIAN_POINT('Ctrl Pts',(-50.,3.29241670612082,-7.16326234391299));
#43103=CARTESIAN_POINT('Ctrl Pts',(-66.,3.32081146957076,-7.22859771080324));
#43104=CARTESIAN_POINT('Ctrl Pts',(-50.,3.32081146957076,-7.22859771080324));
#43105=CARTESIAN_POINT('Ctrl Pts',(-66.,3.359888780788,-7.31524215598795));
#43106=CARTESIAN_POINT('Ctrl Pts',(-50.,3.359888780788,-7.31524215598795));
#43107=CARTESIAN_POINT('Ctrl Pts',(-66.,3.41064498168427,-7.42281101590317));
#43108=CARTESIAN_POINT('Ctrl Pts',(-50.,3.41064498168427,-7.42281101590317));
#43109=CARTESIAN_POINT('Ctrl Pts',(-66.,3.46293063930599,-7.52978780875129));
#43110=CARTESIAN_POINT('Ctrl Pts',(-50.,3.46293063930599,-7.52978780875129));
#43111=CARTESIAN_POINT('Ctrl Pts',(-66.,3.51597837414158,-7.63646478182881));
#43112=CARTESIAN_POINT('Ctrl Pts',(-50.,3.51597837414158,-7.63646478182881));
#43113=CARTESIAN_POINT('Ctrl Pts',(-66.,3.56847706424299,-7.74334074205051));
#43114=CARTESIAN_POINT('Ctrl Pts',(-50.,3.56847706424299,-7.74334074205051));
#43115=CARTESIAN_POINT('Ctrl Pts',(-66.,3.61875289573396,-7.85106692396409));
#43116=CARTESIAN_POINT('Ctrl Pts',(-50.,3.61875289573396,-7.85106692396409));
#43117=CARTESIAN_POINT('Ctrl Pts',(-66.,3.66498426083752,-7.96038432184111));
#43118=CARTESIAN_POINT('Ctrl Pts',(-50.,3.66498426083752,-7.96038432184111));
#43119=CARTESIAN_POINT('Ctrl Pts',(-66.,3.70540363987127,-8.07205943796329));
#43120=CARTESIAN_POINT('Ctrl Pts',(-50.,3.70540363987127,-8.07205943796329));
#43121=CARTESIAN_POINT('Ctrl Pts',(-66.,3.73850464063369,-8.18683427877518));
#43122=CARTESIAN_POINT('Ctrl Pts',(-50.,3.73850464063369,-8.18683427877518));
#43123=CARTESIAN_POINT('Ctrl Pts',(-66.,3.76328700746442,-8.30524256603013));
#43124=CARTESIAN_POINT('Ctrl Pts',(-50.,3.76328700746442,-8.30524256603013));
#43125=CARTESIAN_POINT('Ctrl Pts',(-66.,3.77955877175069,-8.42736119058854));
#43126=CARTESIAN_POINT('Ctrl Pts',(-50.,3.77955877175069,-8.42736119058854));
#43127=CARTESIAN_POINT('Ctrl Pts',(-66.,3.78814329632398,-8.5526379490841));
#43128=CARTESIAN_POINT('Ctrl Pts',(-50.,3.78814329632398,-8.5526379490841));
#43129=CARTESIAN_POINT('Ctrl Pts',(-66.,3.79133013838023,-8.67954430710504));
#43130=CARTESIAN_POINT('Ctrl Pts',(-50.,3.79133013838023,-8.67954430710504));
#43131=CARTESIAN_POINT('Ctrl Pts',(-66.,3.79214634580768,-8.8060610382747));
#43132=CARTESIAN_POINT('Ctrl Pts',(-50.,3.79214634580768,-8.8060610382747));
#43133=CARTESIAN_POINT('Ctrl Pts',(-66.,3.79293549112385,-8.93064918094144));
#43134=CARTESIAN_POINT('Ctrl Pts',(-50.,3.79293549112385,-8.93064918094144));
#43135=CARTESIAN_POINT('Ctrl Pts',(-66.,3.79437267711955,-9.05291824039091));
#43136=CARTESIAN_POINT('Ctrl Pts',(-50.,3.79437267711955,-9.05291824039091));
#43137=CARTESIAN_POINT('Ctrl Pts',(-66.,3.79377821827189,-9.17477904640165));
#43138=CARTESIAN_POINT('Ctrl Pts',(-50.,3.79377821827189,-9.17477904640165));
#43139=CARTESIAN_POINT('Ctrl Pts',(-66.,3.78567343749225,-9.30005041156712));
#43140=CARTESIAN_POINT('Ctrl Pts',(-50.,3.78567343749225,-9.30005041156712));
#43141=CARTESIAN_POINT('Ctrl Pts',(-66.,3.76494029563125,-9.43227003517924));
#43142=CARTESIAN_POINT('Ctrl Pts',(-50.,3.76494029563125,-9.43227003517924));
#43143=CARTESIAN_POINT('Ctrl Pts',(-66.,3.72915055981728,-9.57307911626445));
#43144=CARTESIAN_POINT('Ctrl Pts',(-50.,3.72915055981728,-9.57307911626445));
#43145=CARTESIAN_POINT('Ctrl Pts',(-66.,3.68158234815922,-9.72013034647482));
#43146=CARTESIAN_POINT('Ctrl Pts',(-50.,3.68158234815922,-9.72013034647482));
#43147=CARTESIAN_POINT('Ctrl Pts',(-66.,3.63295761578166,-9.86588553826929));
#43148=CARTESIAN_POINT('Ctrl Pts',(-50.,3.63295761578166,-9.86588553826929));
#43149=CARTESIAN_POINT('Ctrl Pts',(-66.,3.59837801318299,-9.99975571673022));
#43150=CARTESIAN_POINT('Ctrl Pts',(-50.,3.59837801318299,-9.99975571673022));
#43151=CARTESIAN_POINT('Ctrl Pts',(-66.,3.59492345335028,-10.1097801578306));
#43152=CARTESIAN_POINT('Ctrl Pts',(-50.,3.59492345335028,-10.1097801578306));
#43153=CARTESIAN_POINT('Ctrl Pts',(-66.,3.63910068308438,-10.1844096267491));
#43154=CARTESIAN_POINT('Ctrl Pts',(-50.,3.63910068308438,-10.1844096267491));
#43155=CARTESIAN_POINT('Ctrl Pts',(-66.,3.74410743433881,-10.2144193799856));
#43156=CARTESIAN_POINT('Ctrl Pts',(-50.,3.74410743433881,-10.2144193799856));
#43157=CARTESIAN_POINT('Ctrl Pts',(-66.,3.91997031954292,-10.1928102876364));
#43158=CARTESIAN_POINT('Ctrl Pts',(-50.,3.91997031954292,-10.1928102876364));
#43159=CARTESIAN_POINT('Ctrl Pts',(-66.,4.17408991345905,-10.1144251596098));
#43160=CARTESIAN_POINT('Ctrl Pts',(-50.,4.17408991345905,-10.1144251596098));
#43161=CARTESIAN_POINT('Ctrl Pts',(-66.,4.51161767757899,-9.97568294432114));
#43162=CARTESIAN_POINT('Ctrl Pts',(-50.,4.51161767757899,-9.97568294432114));
#43163=CARTESIAN_POINT('Ctrl Pts',(-66.,4.93588146508917,-9.77427910338594));
#43164=CARTESIAN_POINT('Ctrl Pts',(-50.,4.93588146508917,-9.77427910338594));
#43165=CARTESIAN_POINT('Ctrl Pts',(-66.,5.44876930769742,-9.50891534935813));
#43166=CARTESIAN_POINT('Ctrl Pts',(-50.,5.44876930769742,-9.50891534935813));
#43167=CARTESIAN_POINT('Ctrl Pts',(-66.,6.05111211183155,-9.17903030421983));
#43168=CARTESIAN_POINT('Ctrl Pts',(-50.,6.05111211183155,-9.17903030421983));
#43169=CARTESIAN_POINT('Ctrl Pts',(-66.,6.60466213719626,-8.8634396634983));
#43170=CARTESIAN_POINT('Ctrl Pts',(-50.,6.60466213719626,-8.8634396634983));
#43171=CARTESIAN_POINT('Ctrl Pts',(-66.,7.06005528277866,-8.59774076286258));
#43172=CARTESIAN_POINT('Ctrl Pts',(-50.,7.06005528277866,-8.59774076286258));
#43173=CARTESIAN_POINT('Ctrl Pts',(-66.,7.38150722208893,-8.40773377987118));
#43174=CARTESIAN_POINT('Ctrl Pts',(-50.,7.38150722208893,-8.40773377987118));
#43175=CARTESIAN_POINT('Ctrl Pts',(-66.,7.54669732025447,-8.30951169181823));
#43176=CARTESIAN_POINT('Ctrl Pts',(-50.,7.54669732025447,-8.30951169181823));
#43177=CARTESIAN_POINT('',(-65.5,3.6060757177882,-9.99434054440704));
#43178=CARTESIAN_POINT('Ctrl Pts',(-66.,3.76836956336765,-9.39760692058804));
#43179=CARTESIAN_POINT('Ctrl Pts',(-65.7982417703062,3.7257885904294,-9.63205627952235));
#43180=CARTESIAN_POINT('Ctrl Pts',(-65.6331946192803,3.62768025600023,-9.84494595215163));
#43181=CARTESIAN_POINT('Ctrl Pts',(-65.5,3.6060757177882,-9.99434054440703));
#43182=CARTESIAN_POINT('',(-50.,3.26473139515385,-7.09765349728322));
#43183=CARTESIAN_POINT('',(-66.,3.26473139515385,-7.09765349728322));
#43184=CARTESIAN_POINT('',(-50.,3.76836956336765,-9.39760692058806));
#43185=CARTESIAN_POINT('Ctrl Pts',(-50.,3.26473139515385,-7.09765349728322));
#43186=CARTESIAN_POINT('Ctrl Pts',(-50.,3.27389226747348,-7.11954915773029));
#43187=CARTESIAN_POINT('Ctrl Pts',(-50.,3.29241670612082,-7.16326234391299));
#43188=CARTESIAN_POINT('Ctrl Pts',(-50.,3.32081146957076,-7.22859771080324));
#43189=CARTESIAN_POINT('Ctrl Pts',(-50.,3.359888780788,-7.31524215598795));
#43190=CARTESIAN_POINT('Ctrl Pts',(-50.,3.41064498168427,-7.42281101590317));
#43191=CARTESIAN_POINT('Ctrl Pts',(-50.,3.46293063930599,-7.52978780875129));
#43192=CARTESIAN_POINT('Ctrl Pts',(-50.,3.51597837414158,-7.63646478182881));
#43193=CARTESIAN_POINT('Ctrl Pts',(-50.,3.56847706424299,-7.74334074205051));
#43194=CARTESIAN_POINT('Ctrl Pts',(-50.,3.61875289573396,-7.85106692396409));
#43195=CARTESIAN_POINT('Ctrl Pts',(-50.,3.66498426083752,-7.96038432184111));
#43196=CARTESIAN_POINT('Ctrl Pts',(-50.,3.70540363987127,-8.07205943796329));
#43197=CARTESIAN_POINT('Ctrl Pts',(-50.,3.73850464063369,-8.18683427877518));
#43198=CARTESIAN_POINT('Ctrl Pts',(-50.,3.76328700746442,-8.30524256603013));
#43199=CARTESIAN_POINT('Ctrl Pts',(-50.,3.77955877175069,-8.42736119058854));
#43200=CARTESIAN_POINT('Ctrl Pts',(-50.,3.78814329632398,-8.5526379490841));
#43201=CARTESIAN_POINT('Ctrl Pts',(-50.,3.79133013838023,-8.67954430710504));
#43202=CARTESIAN_POINT('Ctrl Pts',(-50.,3.79214634580768,-8.8060610382747));
#43203=CARTESIAN_POINT('Ctrl Pts',(-50.,3.79293549112385,-8.93064918094144));
#43204=CARTESIAN_POINT('Ctrl Pts',(-50.,3.79437267711955,-9.05291824039091));
#43205=CARTESIAN_POINT('Ctrl Pts',(-50.,3.79381050973993,-9.168159472417));
#43206=CARTESIAN_POINT('Ctrl Pts',(-50.,3.78814720834319,-9.26139904172235));
#43207=CARTESIAN_POINT('Ctrl Pts',(-50.,3.77947496961539,-9.33209763417662));
#43208=CARTESIAN_POINT('Ctrl Pts',(-50.,3.77192378760531,-9.37803748530916));
#43209=CARTESIAN_POINT('Ctrl Pts',(-50.,3.76836956336765,-9.39760692058806));
#43210=CARTESIAN_POINT('',(-50.5,3.6060757177882,-9.99434054440704));
#43211=CARTESIAN_POINT('Ctrl Pts',(-50.5,3.6060757177882,-9.99434054440705));
#43212=CARTESIAN_POINT('Ctrl Pts',(-50.4982567069814,3.60635848477112,-9.99238522105314));
#43213=CARTESIAN_POINT('Ctrl Pts',(-50.496511343879,3.60665306382448,-9.99042330533535));
#43214=CARTESIAN_POINT('Ctrl Pts',(-50.3581212730812,3.63088681363861,-9.83453533000683));
#43215=CARTESIAN_POINT('Ctrl Pts',(-50.2022201285476,3.72569110690851,-9.63259302040446));
#43216=CARTESIAN_POINT('Ctrl Pts',(-50.,3.76836956336765,-9.39760692058806));
#43217=CARTESIAN_POINT('Ctrl Pts',(-65.5,3.6060757177882,-9.99434054440703));
#43218=CARTESIAN_POINT('Ctrl Pts',(-60.5,3.6060757177882,-9.99434054440703));
#43219=CARTESIAN_POINT('Ctrl Pts',(-55.5,3.6060757177882,-9.99434054440704));
#43220=CARTESIAN_POINT('Ctrl Pts',(-50.5,3.6060757177882,-9.99434054440704));
#43221=CARTESIAN_POINT('Origin',(-66.,0.,0.));
#43222=CARTESIAN_POINT('',(-50.,4.5143825383298,-6.37616707337747));
#43223=CARTESIAN_POINT('',(-66.,4.5143825383298,-6.37616707337747));
#43224=CARTESIAN_POINT('Origin',(-50.,0.,0.));
#43225=CARTESIAN_POINT('Ctrl Pts',(-66.,7.54669732025447,-8.30951169181823));
#43226=CARTESIAN_POINT('Ctrl Pts',(-50.,7.54669732025447,-8.30951169181823));
#43227=CARTESIAN_POINT('Ctrl Pts',(-66.,7.52333157969776,-8.30560656273532));
#43228=CARTESIAN_POINT('Ctrl Pts',(-50.,7.52333157969776,-8.30560656273532));
#43229=CARTESIAN_POINT('Ctrl Pts',(-66.,7.47670872115481,-8.29761250101419));
#43230=CARTESIAN_POINT('Ctrl Pts',(-50.,7.47670872115481,-8.29761250101419));
#43231=CARTESIAN_POINT('Ctrl Pts',(-66.,7.4071003012639,-8.28506999791136));
#43232=CARTESIAN_POINT('Ctrl Pts',(-50.,7.4071003012639,-8.28506999791136));
#43233=CARTESIAN_POINT('Ctrl Pts',(-66.,7.31494167541519,-8.26724237158035));
#43234=CARTESIAN_POINT('Ctrl Pts',(-50.,7.31494167541519,-8.26724237158035));
#43235=CARTESIAN_POINT('Ctrl Pts',(-66.,7.20083933184586,-8.24310753334095));
#43236=CARTESIAN_POINT('Ctrl Pts',(-50.,7.20083933184586,-8.24310753334095));
#43237=CARTESIAN_POINT('Ctrl Pts',(-66.,7.0878489571346,-8.21710771481861));
#43238=CARTESIAN_POINT('Ctrl Pts',(-50.,7.0878489571346,-8.21710771481861));
#43239=CARTESIAN_POINT('Ctrl Pts',(-66.,6.97599606044936,-8.18922484372218));
#43240=CARTESIAN_POINT('Ctrl Pts',(-50.,6.97599606044936,-8.18922484372218));
#43241=CARTESIAN_POINT('Ctrl Pts',(-66.,6.8653170030208,-8.15943901382578));
#43242=CARTESIAN_POINT('Ctrl Pts',(-50.,6.8653170030208,-8.15943901382578));
#43243=CARTESIAN_POINT('Ctrl Pts',(-66.,6.75586105705924,-8.12773028115812));
#43244=CARTESIAN_POINT('Ctrl Pts',(-50.,6.75586105705924,-8.12773028115812));
#43245=CARTESIAN_POINT('Ctrl Pts',(-66.,6.64768765206965,-8.09407995465062));
#43246=CARTESIAN_POINT('Ctrl Pts',(-50.,6.64768765206965,-8.09407995465062));
#43247=CARTESIAN_POINT('Ctrl Pts',(-66.,6.54086250417151,-8.05847172269461));
#43248=CARTESIAN_POINT('Ctrl Pts',(-50.,6.54086250417151,-8.05847172269461));
#43249=CARTESIAN_POINT('Ctrl Pts',(-66.,6.43545373939148,-8.02089334946028));
#43250=CARTESIAN_POINT('Ctrl Pts',(-50.,6.43545373939148,-8.02089334946028));
#43251=CARTESIAN_POINT('Ctrl Pts',(-66.,6.33152851820538,-7.98133773872331));
#43252=CARTESIAN_POINT('Ctrl Pts',(-50.,6.33152851820538,-7.98133773872331));
#43253=CARTESIAN_POINT('Ctrl Pts',(-66.,6.22914767586739,-7.93980615319185));
#43254=CARTESIAN_POINT('Ctrl Pts',(-50.,6.22914767586739,-7.93980615319185));
#43255=CARTESIAN_POINT('Ctrl Pts',(-66.,6.12836917819085,-7.89630262173216));
#43256=CARTESIAN_POINT('Ctrl Pts',(-50.,6.12836917819085,-7.89630262173216));
#43257=CARTESIAN_POINT('Ctrl Pts',(-66.,6.02925624926082,-7.85082401216739));
#43258=CARTESIAN_POINT('Ctrl Pts',(-50.,6.02925624926082,-7.85082401216739));
#43259=CARTESIAN_POINT('Ctrl Pts',(-66.,5.93188366426367,-7.80335138726874));
#43260=CARTESIAN_POINT('Ctrl Pts',(-50.,5.93188366426367,-7.80335138726874));
#43261=CARTESIAN_POINT('Ctrl Pts',(-66.,5.83634515157351,-7.75384156215611));
#43262=CARTESIAN_POINT('Ctrl Pts',(-50.,5.83634515157351,-7.75384156215611));
#43263=CARTESIAN_POINT('Ctrl Pts',(-66.,5.74275901635157,-7.70221724602392));
#43264=CARTESIAN_POINT('Ctrl Pts',(-50.,5.74275901635157,-7.70221724602392));
#43265=CARTESIAN_POINT('Ctrl Pts',(-66.,5.65127930303142,-7.64836468312946));
#43266=CARTESIAN_POINT('Ctrl Pts',(-50.,5.65127930303142,-7.64836468312946));
#43267=CARTESIAN_POINT('Ctrl Pts',(-66.,5.5621084189074,-7.59213750764915));
#43268=CARTESIAN_POINT('Ctrl Pts',(-50.,5.5621084189074,-7.59213750764915));
#43269=CARTESIAN_POINT('Ctrl Pts',(-66.,5.47551271178446,-7.53335714794964));
#43270=CARTESIAN_POINT('Ctrl Pts',(-50.,5.47551271178446,-7.53335714794964));
#43271=CARTESIAN_POINT('Ctrl Pts',(-66.,5.39182944999988,-7.47181841290458));
#43272=CARTESIAN_POINT('Ctrl Pts',(-50.,5.39182944999988,-7.47181841290458));
#43273=CARTESIAN_POINT('Ctrl Pts',(-66.,5.31149612450297,-7.40728387468187));
#43274=CARTESIAN_POINT('Ctrl Pts',(-50.,5.31149612450297,-7.40728387468187));
#43275=CARTESIAN_POINT('Ctrl Pts',(-66.,5.23498395346241,-7.33952553391019));
#43276=CARTESIAN_POINT('Ctrl Pts',(-50.,5.23498395346241,-7.33952553391019));
#43277=CARTESIAN_POINT('Ctrl Pts',(-66.,5.16267694013817,-7.26839273674309));
#43278=CARTESIAN_POINT('Ctrl Pts',(-50.,5.16267694013817,-7.26839273674309));
#43279=CARTESIAN_POINT('Ctrl Pts',(-66.,5.09476012362649,-7.19387696930703));
#43280=CARTESIAN_POINT('Ctrl Pts',(-50.,5.09476012362649,-7.19387696930703));
#43281=CARTESIAN_POINT('Ctrl Pts',(-66.,5.03111729892527,-7.1161697713572));
#43282=CARTESIAN_POINT('Ctrl Pts',(-50.,5.03111729892527,-7.1161697713572));
#43283=CARTESIAN_POINT('Ctrl Pts',(-66.,4.97118523196097,-7.03574860294511));
#43284=CARTESIAN_POINT('Ctrl Pts',(-50.,4.97118523196097,-7.03574860294511));
#43285=CARTESIAN_POINT('Ctrl Pts',(-66.,4.91404818867789,-6.95331119177114));
#43286=CARTESIAN_POINT('Ctrl Pts',(-50.,4.91404818867789,-6.95331119177114));
#43287=CARTESIAN_POINT('Ctrl Pts',(-66.,4.85861849397619,-6.86965589298989));
#43288=CARTESIAN_POINT('Ctrl Pts',(-50.,4.85861849397619,-6.86965589298989));
#43289=CARTESIAN_POINT('Ctrl Pts',(-66.,4.80379072956909,-6.78557840443743));
#43290=CARTESIAN_POINT('Ctrl Pts',(-50.,4.80379072956909,-6.78557840443743));
#43291=CARTESIAN_POINT('Ctrl Pts',(-66.,4.74859881197601,-6.7017671151923));
#43292=CARTESIAN_POINT('Ctrl Pts',(-50.,4.74859881197601,-6.7017671151923));
#43293=CARTESIAN_POINT('Ctrl Pts',(-66.,4.69239210704599,-6.61868514985729));
#43294=CARTESIAN_POINT('Ctrl Pts',(-50.,4.69239210704599,-6.61868514985729));
#43295=CARTESIAN_POINT('Ctrl Pts',(-66.,4.63479108448607,-6.53660277498602));
#43296=CARTESIAN_POINT('Ctrl Pts',(-50.,4.63479108448607,-6.53660277498602));
#43297=CARTESIAN_POINT('Ctrl Pts',(-66.,4.58744600070291,-6.47184245854068));
#43298=CARTESIAN_POINT('Ctrl Pts',(-50.,4.58744600070291,-6.47184245854068));
#43299=CARTESIAN_POINT('Ctrl Pts',(-66.,4.55120043280854,-6.42379983595862));
#43300=CARTESIAN_POINT('Ctrl Pts',(-50.,4.55120043280854,-6.42379983595862));
#43301=CARTESIAN_POINT('Ctrl Pts',(-66.,4.52670967601697,-6.39200562736583));
#43302=CARTESIAN_POINT('Ctrl Pts',(-50.,4.52670967601697,-6.39200562736583));
#43303=CARTESIAN_POINT('Ctrl Pts',(-66.,4.51438253832981,-6.37616707337746));
#43304=CARTESIAN_POINT('Ctrl Pts',(-50.,4.51438253832981,-6.37616707337746));
#43305=CARTESIAN_POINT('Ctrl Pts',(-50.,6.26496857389736,-7.95397974400732));
#43306=CARTESIAN_POINT('Ctrl Pts',(-50.,6.25786529949278,-7.95107028292052));
#43307=CARTESIAN_POINT('Ctrl Pts',(-50.,6.23037340346061,-7.93974831559927));
#43308=CARTESIAN_POINT('Ctrl Pts',(-50.,6.1827347586952,-7.91971356466277));
#43309=CARTESIAN_POINT('Ctrl Pts',(-50.,6.11544012502743,-7.89037004192437));
#43310=CARTESIAN_POINT('Ctrl Pts',(-50.,6.02925624926082,-7.85082401216739));
#43311=CARTESIAN_POINT('Ctrl Pts',(-50.,5.93188366426367,-7.80335138726874));
#43312=CARTESIAN_POINT('Ctrl Pts',(-50.,5.83634515157351,-7.75384156215611));
#43313=CARTESIAN_POINT('Ctrl Pts',(-50.,5.74275901635157,-7.70221724602392));
#43314=CARTESIAN_POINT('Ctrl Pts',(-50.,5.65127930303142,-7.64836468312946));
#43315=CARTESIAN_POINT('Ctrl Pts',(-50.,5.5621084189074,-7.59213750764915));
#43316=CARTESIAN_POINT('Ctrl Pts',(-50.,5.47551271178446,-7.53335714794964));
#43317=CARTESIAN_POINT('Ctrl Pts',(-50.,5.39182944999988,-7.47181841290458));
#43318=CARTESIAN_POINT('Ctrl Pts',(-50.,5.31149612450297,-7.40728387468187));
#43319=CARTESIAN_POINT('Ctrl Pts',(-50.,5.23498395346241,-7.33952553391019));
#43320=CARTESIAN_POINT('Ctrl Pts',(-50.,5.16267694013817,-7.26839273674309));
#43321=CARTESIAN_POINT('Ctrl Pts',(-50.,5.09476012362649,-7.19387696930703));
#43322=CARTESIAN_POINT('Ctrl Pts',(-50.,5.03111729892527,-7.1161697713572));
#43323=CARTESIAN_POINT('Ctrl Pts',(-50.,4.97118523196097,-7.03574860294511));
#43324=CARTESIAN_POINT('Ctrl Pts',(-50.,4.91404818867789,-6.95331119177114));
#43325=CARTESIAN_POINT('Ctrl Pts',(-50.,4.85861849397619,-6.86965589298989));
#43326=CARTESIAN_POINT('Ctrl Pts',(-50.,4.80379072956909,-6.78557840443743));
#43327=CARTESIAN_POINT('Ctrl Pts',(-50.,4.74859881197601,-6.7017671151923));
#43328=CARTESIAN_POINT('Ctrl Pts',(-50.,4.69239210704599,-6.61868514985729));
#43329=CARTESIAN_POINT('Ctrl Pts',(-50.,4.63479108448607,-6.53660277498602));
#43330=CARTESIAN_POINT('Ctrl Pts',(-50.,4.58744600070291,-6.47184245854068));
#43331=CARTESIAN_POINT('Ctrl Pts',(-50.,4.55120043280854,-6.42379983595862));
#43332=CARTESIAN_POINT('Ctrl Pts',(-50.,4.52670967601697,-6.39200562736583));
#43333=CARTESIAN_POINT('Ctrl Pts',(-50.,4.51438253832981,-6.37616707337746));
#43334=CARTESIAN_POINT('Origin',(-50.,5.1702676791723,-7.97690222761574));
#43335=CARTESIAN_POINT('Origin',(-50.,0.,0.));
#43336=CARTESIAN_POINT('Origin',(-65.75,0.,0.));
#43337=CARTESIAN_POINT('',(-65.5,2.91799338807253,-10.216454354969));
#43338=CARTESIAN_POINT('Origin',(-65.5,0.,0.));
#43339=CARTESIAN_POINT('',(-66.,2.48815856278711,-9.81451435204152));
#43340=CARTESIAN_POINT('Ctrl Pts',(-65.5,2.91799338807253,-10.216454354969));
#43341=CARTESIAN_POINT('Ctrl Pts',(-65.6642587837351,2.76632796613792,-10.0889452570453));
#43342=CARTESIAN_POINT('Ctrl Pts',(-65.8310681634032,2.62232043935157,-9.95477792232024));
#43343=CARTESIAN_POINT('Ctrl Pts',(-66.,2.48815856278711,-9.81451435204153));
#43344=CARTESIAN_POINT('Origin',(-66.,0.,0.));
#43345=CARTESIAN_POINT('Origin',(-58.,0.,0.));
#43346=CARTESIAN_POINT('',(-50.5,2.91799338807254,-10.216454354969));
#43347=CARTESIAN_POINT('Origin',(-50.5,0.,0.));
#43348=CARTESIAN_POINT('Ctrl Pts',(-50.5,2.91799338807254,-10.216454354969));
#43349=CARTESIAN_POINT('Ctrl Pts',(-55.5,2.91799338807254,-10.216454354969));
#43350=CARTESIAN_POINT('Ctrl Pts',(-60.5,2.91799338807253,-10.216454354969));
#43351=CARTESIAN_POINT('Ctrl Pts',(-65.5,2.91799338807253,-10.216454354969));
#43352=CARTESIAN_POINT('Origin',(-50.25,0.,0.));
#43353=CARTESIAN_POINT('',(-50.,2.48815856278712,-9.81451435204154));
#43354=CARTESIAN_POINT('Origin',(-50.,0.,0.));
#43355=CARTESIAN_POINT('Ctrl Pts',(-50.,2.48815856278713,-9.81451435204155));
#43356=CARTESIAN_POINT('Ctrl Pts',(-50.1689318365966,2.62232043935141,-9.95477792232008));
#43357=CARTESIAN_POINT('Ctrl Pts',(-50.3357412162647,2.76632796613773,-10.0889452570451));
#43358=CARTESIAN_POINT('Ctrl Pts',(-50.5,2.91799338807254,-10.216454354969));
#43359=CARTESIAN_POINT('Origin',(-66.,1.47877611889991,-9.39020011572736));
#43360=CARTESIAN_POINT('',(-66.,-0.37977419449274,-10.1178751010871));
#43361=CARTESIAN_POINT('Origin',(-66.,0.,0.));
#43362=CARTESIAN_POINT('',(-66.,1.53067287083626,-7.66108326625458));
#43363=CARTESIAN_POINT('Ctrl Pts',(-66.,1.53067287083627,-7.66108326625457));
#43364=CARTESIAN_POINT('Ctrl Pts',(-66.,1.53549215119571,-7.68056640390788));
#43365=CARTESIAN_POINT('Ctrl Pts',(-66.,1.54493370114459,-7.71957314695095));
#43366=CARTESIAN_POINT('Ctrl Pts',(-66.,1.55850498002059,-7.77820466719577));
#43367=CARTESIAN_POINT('Ctrl Pts',(-66.,1.5754164725369,-7.85662314056401));
#43368=CARTESIAN_POINT('Ctrl Pts',(-66.,1.59465171544125,-7.95503756783394));
#43369=CARTESIAN_POINT('Ctrl Pts',(-66.,1.61220661573863,-8.05379804635934));
#43370=CARTESIAN_POINT('Ctrl Pts',(-66.,1.62853781891495,-8.15281204423512));
#43371=CARTESIAN_POINT('Ctrl Pts',(-66.,1.64442807858968,-8.25192111283452));
#43372=CARTESIAN_POINT('Ctrl Pts',(-66.,1.66103994900115,-8.35088931899355));
#43373=CARTESIAN_POINT('Ctrl Pts',(-66.,1.67970691947077,-8.44943937069158));
#43374=CARTESIAN_POINT('Ctrl Pts',(-66.,1.70174735094098,-8.54728433152241));
#43375=CARTESIAN_POINT('Ctrl Pts',(-66.,1.72828159952138,-8.64415925811045));
#43376=CARTESIAN_POINT('Ctrl Pts',(-66.,1.76001840564001,-8.73985705693077));
#43377=CARTESIAN_POINT('Ctrl Pts',(-66.,1.79714183408573,-8.83425001254252));
#43378=CARTESIAN_POINT('Ctrl Pts',(-66.,1.83947938032835,-8.92727064057537));
#43379=CARTESIAN_POINT('Ctrl Pts',(-66.,1.88661896349422,-9.01890038196952));
#43380=CARTESIAN_POINT('Ctrl Pts',(-66.,1.93803736866688,-9.10915586281889));
#43381=CARTESIAN_POINT('Ctrl Pts',(-66.,1.99323835737743,-9.19807604064094));
#43382=CARTESIAN_POINT('Ctrl Pts',(-66.,2.05183036091841,-9.28571118746575));
#43383=CARTESIAN_POINT('Ctrl Pts',(-66.,2.11349742683576,-9.37211610318578));
#43384=CARTESIAN_POINT('Ctrl Pts',(-66.,2.17799511452139,-9.45734217317086));
#43385=CARTESIAN_POINT('Ctrl Pts',(-66.,2.24513642875384,-9.54143066294722));
#43386=CARTESIAN_POINT('Ctrl Pts',(-66.,2.31478185538763,-9.62440406213512));
#43387=CARTESIAN_POINT('Ctrl Pts',(-66.,2.37742992422592,-9.69558529830397));
#43388=CARTESIAN_POINT('Ctrl Pts',(-66.,2.4269715452022,-9.74976313360791));
#43389=CARTESIAN_POINT('Ctrl Pts',(-66.,2.46234274539511,-9.78744217177351));
#43390=CARTESIAN_POINT('Ctrl Pts',(-66.,2.48285278315603,-9.80896726509533));
#43391=CARTESIAN_POINT('Ctrl Pts',(-66.,2.48815856278711,-9.81451435204152));
#43392=CARTESIAN_POINT('',(-66.,0.0956047792657981,-7.81191500057326));
#43393=CARTESIAN_POINT('Origin',(-66.,0.,0.));
#43394=CARTESIAN_POINT('Ctrl Pts',(-66.,-0.37977419449274,-10.1178751010871));
#43395=CARTESIAN_POINT('Ctrl Pts',(-66.,-0.368567642672759,-10.1014431656146));
#43396=CARTESIAN_POINT('Ctrl Pts',(-66.,-0.342983873814566,-10.0625463657097));
#43397=CARTESIAN_POINT('Ctrl Pts',(-66.,-0.306305681352163,-10.0014873049795));
#43398=CARTESIAN_POINT('Ctrl Pts',(-66.,-0.263208048664822,-9.91861219216684));
#43399=CARTESIAN_POINT('Ctrl Pts',(-66.,-0.215821651350525,-9.8135627421891));
#43400=CARTESIAN_POINT('Ctrl Pts',(-66.,-0.167403279296175,-9.70127984211144));
#43401=CARTESIAN_POINT('Ctrl Pts',(-66.,-0.117449636499862,-9.58714193598532));
#43402=CARTESIAN_POINT('Ctrl Pts',(-66.,-0.0667362885588257,-9.47123116944039));
#43403=CARTESIAN_POINT('Ctrl Pts',(-66.,-0.0180301475971287,-9.35400023708443));
#43404=CARTESIAN_POINT('Ctrl Pts',(-66.,0.025082147178823,-9.23606258270527));
#43405=CARTESIAN_POINT('Ctrl Pts',(-66.,0.0598872702371897,-9.11788334516365));
#43406=CARTESIAN_POINT('Ctrl Pts',(-66.,0.0854084408597768,-8.99963209550245));
#43407=CARTESIAN_POINT('Ctrl Pts',(-66.,0.101852305431236,-8.88131667109455));
#43408=CARTESIAN_POINT('Ctrl Pts',(-66.,0.110349727160855,-8.76285633348602));
#43409=CARTESIAN_POINT('Ctrl Pts',(-66.,0.112578665012154,-8.64418593096713));
#43410=CARTESIAN_POINT('Ctrl Pts',(-66.,0.110465593127282,-8.52532414388232));
#43411=CARTESIAN_POINT('Ctrl Pts',(-66.,0.105976022539028,-8.40633495491286));
#43412=CARTESIAN_POINT('Ctrl Pts',(-66.,0.10090393926479,-8.28730423313303));
#43413=CARTESIAN_POINT('Ctrl Pts',(-66.,0.0966499958546681,-8.16830957709138));
#43414=CARTESIAN_POINT('Ctrl Pts',(-66.,0.0940340960600895,-8.04939612696421));
#43415=CARTESIAN_POINT('Ctrl Pts',(-66.,0.0935766666762872,-7.95434831325083));
#43416=CARTESIAN_POINT('Ctrl Pts',(-66.,0.094211047308826,-7.88311229483827));
#43417=CARTESIAN_POINT('Ctrl Pts',(-66.,0.0950678851332727,-7.8356437441717));
#43418=CARTESIAN_POINT('Ctrl Pts',(-66.,0.0956047792657981,-7.81191500057326));
#43419=CARTESIAN_POINT('Ctrl Pts',(-66.,0.0956047792657981,-7.81191500057326));
#43420=CARTESIAN_POINT('Ctrl Pts',(-50.,0.0956047792657981,-7.81191500057326));
#43421=CARTESIAN_POINT('Ctrl Pts',(-66.,0.0950678851332727,-7.8356437441717));
#43422=CARTESIAN_POINT('Ctrl Pts',(-50.,0.0950678851332727,-7.8356437441717));
#43423=CARTESIAN_POINT('Ctrl Pts',(-66.,0.094211047308826,-7.88311229483827));
#43424=CARTESIAN_POINT('Ctrl Pts',(-50.,0.094211047308826,-7.88311229483827));
#43425=CARTESIAN_POINT('Ctrl Pts',(-66.,0.0935766666762872,-7.95434831325083));
#43426=CARTESIAN_POINT('Ctrl Pts',(-50.,0.0935766666762872,-7.95434831325083));
#43427=CARTESIAN_POINT('Ctrl Pts',(-66.,0.0940340960600895,-8.04939612696421));
#43428=CARTESIAN_POINT('Ctrl Pts',(-50.,0.0940340960600895,-8.04939612696421));
#43429=CARTESIAN_POINT('Ctrl Pts',(-66.,0.0966499958546681,-8.16830957709138));
#43430=CARTESIAN_POINT('Ctrl Pts',(-50.,0.0966499958546681,-8.16830957709138));
#43431=CARTESIAN_POINT('Ctrl Pts',(-66.,0.10090393926479,-8.28730423313303));
#43432=CARTESIAN_POINT('Ctrl Pts',(-50.,0.10090393926479,-8.28730423313303));
#43433=CARTESIAN_POINT('Ctrl Pts',(-66.,0.105976022539028,-8.40633495491286));
#43434=CARTESIAN_POINT('Ctrl Pts',(-50.,0.105976022539028,-8.40633495491286));
#43435=CARTESIAN_POINT('Ctrl Pts',(-66.,0.110465593127282,-8.52532414388232));
#43436=CARTESIAN_POINT('Ctrl Pts',(-50.,0.110465593127282,-8.52532414388232));
#43437=CARTESIAN_POINT('Ctrl Pts',(-66.,0.112578665012154,-8.64418593096713));
#43438=CARTESIAN_POINT('Ctrl Pts',(-50.,0.112578665012154,-8.64418593096713));
#43439=CARTESIAN_POINT('Ctrl Pts',(-66.,0.110349727160855,-8.76285633348602));
#43440=CARTESIAN_POINT('Ctrl Pts',(-50.,0.110349727160855,-8.76285633348602));
#43441=CARTESIAN_POINT('Ctrl Pts',(-66.,0.101852305431236,-8.88131667109455));
#43442=CARTESIAN_POINT('Ctrl Pts',(-50.,0.101852305431236,-8.88131667109455));
#43443=CARTESIAN_POINT('Ctrl Pts',(-66.,0.0854084408597768,-8.99963209550245));
#43444=CARTESIAN_POINT('Ctrl Pts',(-50.,0.0854084408597768,-8.99963209550245));
#43445=CARTESIAN_POINT('Ctrl Pts',(-66.,0.0598872702371897,-9.11788334516365));
#43446=CARTESIAN_POINT('Ctrl Pts',(-50.,0.0598872702371897,-9.11788334516365));
#43447=CARTESIAN_POINT('Ctrl Pts',(-66.,0.025082147178823,-9.23606258270527));
#43448=CARTESIAN_POINT('Ctrl Pts',(-50.,0.025082147178823,-9.23606258270527));
#43449=CARTESIAN_POINT('Ctrl Pts',(-66.,-0.0180301475971287,-9.35400023708443));
#43450=CARTESIAN_POINT('Ctrl Pts',(-50.,-0.0180301475971287,-9.35400023708443));
#43451=CARTESIAN_POINT('Ctrl Pts',(-66.,-0.0667362885588257,-9.47123116944039));
#43452=CARTESIAN_POINT('Ctrl Pts',(-50.,-0.0667362885588257,-9.47123116944039));
#43453=CARTESIAN_POINT('Ctrl Pts',(-66.,-0.117449636499862,-9.58714193598532));
#43454=CARTESIAN_POINT('Ctrl Pts',(-50.,-0.117449636499862,-9.58714193598532));
#43455=CARTESIAN_POINT('Ctrl Pts',(-66.,-0.167403279296175,-9.70127984211144));
#43456=CARTESIAN_POINT('Ctrl Pts',(-50.,-0.167403279296175,-9.70127984211144));
#43457=CARTESIAN_POINT('Ctrl Pts',(-66.,-0.215821651350525,-9.8135627421891));
#43458=CARTESIAN_POINT('Ctrl Pts',(-50.,-0.215821651350525,-9.8135627421891));
#43459=CARTESIAN_POINT('Ctrl Pts',(-66.,-0.26592997168988,-9.92464633978874));
#43460=CARTESIAN_POINT('Ctrl Pts',(-50.,-0.26592997168988,-9.92464633978874));
#43461=CARTESIAN_POINT('Ctrl Pts',(-66.,-0.324286511897233,-10.0357909150812));
#43462=CARTESIAN_POINT('Ctrl Pts',(-50.,-0.324286511897233,-10.0357909150812));
#43463=CARTESIAN_POINT('Ctrl Pts',(-66.,-0.39700574532375,-10.1481466231223));
#43464=CARTESIAN_POINT('Ctrl Pts',(-50.,-0.39700574532375,-10.1481466231223));
#43465=CARTESIAN_POINT('Ctrl Pts',(-66.,-0.486973508862013,-10.262225122541));
#43466=CARTESIAN_POINT('Ctrl Pts',(-50.,-0.486973508862013,-10.262225122541));
#43467=CARTESIAN_POINT('Ctrl Pts',(-66.,-0.590240356286357,-10.3772153712135));
#43468=CARTESIAN_POINT('Ctrl Pts',(-50.,-0.590240356286357,-10.3772153712135));
#43469=CARTESIAN_POINT('Ctrl Pts',(-66.,-0.693945237100309,-10.4905919041874));
#43470=CARTESIAN_POINT('Ctrl Pts',(-50.,-0.693945237100309,-10.4905919041874));
#43471=CARTESIAN_POINT('Ctrl Pts',(-66.,-0.779985182976566,-10.5988236061543));
#43472=CARTESIAN_POINT('Ctrl Pts',(-50.,-0.779985182976566,-10.5988236061543));
#43473=CARTESIAN_POINT('Ctrl Pts',(-66.,-0.827892052249358,-10.6979308384816));
#43474=CARTESIAN_POINT('Ctrl Pts',(-50.,-0.827892052249358,-10.6979308384816));
#43475=CARTESIAN_POINT('Ctrl Pts',(-66.,-0.817888684356991,-10.7840767489408));
#43476=CARTESIAN_POINT('Ctrl Pts',(-50.,-0.817888684356991,-10.7840767489408));
#43477=CARTESIAN_POINT('Ctrl Pts',(-66.,-0.734166310017649,-10.8542021162005));
#43478=CARTESIAN_POINT('Ctrl Pts',(-50.,-0.734166310017649,-10.8542021162005));
#43479=CARTESIAN_POINT('Ctrl Pts',(-66.,-0.564718360389463,-10.9059911076107));
#43480=CARTESIAN_POINT('Ctrl Pts',(-50.,-0.564718360389463,-10.9059911076107));
#43481=CARTESIAN_POINT('Ctrl Pts',(-66.,-0.300686455828779,-10.9377424805244));
#43482=CARTESIAN_POINT('Ctrl Pts',(-50.,-0.300686455828779,-10.9377424805244));
#43483=CARTESIAN_POINT('Ctrl Pts',(-66.,0.0640920428106455,-10.9482800696873));
#43484=CARTESIAN_POINT('Ctrl Pts',(-50.,0.0640920428106455,-10.9482800696873));
#43485=CARTESIAN_POINT('Ctrl Pts',(-66.,0.533594620897368,-10.9368521343596));
#43486=CARTESIAN_POINT('Ctrl Pts',(-50.,0.533594620897368,-10.9368521343596));
#43487=CARTESIAN_POINT('Ctrl Pts',(-66.,1.11007414229951,-10.9030405616214));
#43488=CARTESIAN_POINT('Ctrl Pts',(-50.,1.11007414229951,-10.9030405616214));
#43489=CARTESIAN_POINT('Ctrl Pts',(-66.,1.79451801082041,-10.8466704672255));
#43490=CARTESIAN_POINT('Ctrl Pts',(-50.,1.79451801082041,-10.8466704672255));
#43491=CARTESIAN_POINT('Ctrl Pts',(-66.,2.42857339986351,-10.7835131500112));
#43492=CARTESIAN_POINT('Ctrl Pts',(-50.,2.42857339986351,-10.7835131500112));
#43493=CARTESIAN_POINT('Ctrl Pts',(-66.,2.95266521836539,-10.7260102055487));
#43494=CARTESIAN_POINT('Ctrl Pts',(-50.,2.95266521836539,-10.7260102055487));
#43495=CARTESIAN_POINT('Ctrl Pts',(-66.,3.32360897979558,-10.6831764720218));
#43496=CARTESIAN_POINT('Ctrl Pts',(-50.,3.32360897979558,-10.6831764720218));
#43497=CARTESIAN_POINT('Ctrl Pts',(-66.,3.51446816599279,-10.6606349956381));
#43498=CARTESIAN_POINT('Ctrl Pts',(-50.,3.51446816599279,-10.6606349956381));
#43499=CARTESIAN_POINT('',(-65.5,-0.770750430887795,-10.5970075386067));
#43500=CARTESIAN_POINT('Ctrl Pts',(-66.,-0.37977419449274,-10.1178751010871));
#43501=CARTESIAN_POINT('Ctrl Pts',(-65.798241770306,-0.514032994126835,
-10.3147360059971));
#43502=CARTESIAN_POINT('Ctrl Pts',(-65.6331946192801,-0.690249448192153,
-10.469316144803));
#43503=CARTESIAN_POINT('Ctrl Pts',(-65.5,-0.770750430887792,-10.5970075386067));
#43504=CARTESIAN_POINT('',(-50.,0.0956047792657982,-7.81191500057326));
#43505=CARTESIAN_POINT('',(-66.,0.0956047792657981,-7.81191500057326));
#43506=CARTESIAN_POINT('',(-50.,-0.379774194492752,-10.1178751010871));
#43507=CARTESIAN_POINT('Ctrl Pts',(-50.,0.0956047792657981,-7.81191500057326));
#43508=CARTESIAN_POINT('Ctrl Pts',(-50.,0.0950678851332727,-7.8356437441717));
#43509=CARTESIAN_POINT('Ctrl Pts',(-50.,0.094211047308826,-7.88311229483827));
#43510=CARTESIAN_POINT('Ctrl Pts',(-50.,0.0935766666762872,-7.95434831325083));
#43511=CARTESIAN_POINT('Ctrl Pts',(-50.,0.0940340960600895,-8.04939612696421));
#43512=CARTESIAN_POINT('Ctrl Pts',(-50.,0.0966499958546681,-8.16830957709138));
#43513=CARTESIAN_POINT('Ctrl Pts',(-50.,0.10090393926479,-8.28730423313303));
#43514=CARTESIAN_POINT('Ctrl Pts',(-50.,0.105976022539028,-8.40633495491286));
#43515=CARTESIAN_POINT('Ctrl Pts',(-50.,0.110465593127282,-8.52532414388232));
#43516=CARTESIAN_POINT('Ctrl Pts',(-50.,0.112578665012154,-8.64418593096713));
#43517=CARTESIAN_POINT('Ctrl Pts',(-50.,0.110349727160855,-8.76285633348602));
#43518=CARTESIAN_POINT('Ctrl Pts',(-50.,0.101852305431236,-8.88131667109455));
#43519=CARTESIAN_POINT('Ctrl Pts',(-50.,0.0854084408597768,-8.99963209550245));
#43520=CARTESIAN_POINT('Ctrl Pts',(-50.,0.0598872702371897,-9.11788334516365));
#43521=CARTESIAN_POINT('Ctrl Pts',(-50.,0.025082147178823,-9.23606258270527));
#43522=CARTESIAN_POINT('Ctrl Pts',(-50.,-0.0180301475971287,-9.35400023708443));
#43523=CARTESIAN_POINT('Ctrl Pts',(-50.,-0.0667362885588257,-9.47123116944039));
#43524=CARTESIAN_POINT('Ctrl Pts',(-50.,-0.117449636499862,-9.58714193598532));
#43525=CARTESIAN_POINT('Ctrl Pts',(-50.,-0.167403279296175,-9.70127984211144));
#43526=CARTESIAN_POINT('Ctrl Pts',(-50.,-0.215821651350525,-9.8135627421891));
#43527=CARTESIAN_POINT('Ctrl Pts',(-50.,-0.263208048664824,-9.91861219216685));
#43528=CARTESIAN_POINT('Ctrl Pts',(-50.,-0.306305681352166,-10.0014873049795));
#43529=CARTESIAN_POINT('Ctrl Pts',(-50.,-0.342983873814572,-10.0625463657097));
#43530=CARTESIAN_POINT('Ctrl Pts',(-50.,-0.368567642672767,-10.1014431656146));
#43531=CARTESIAN_POINT('Ctrl Pts',(-50.,-0.379774194492751,-10.1178751010871));
#43532=CARTESIAN_POINT('',(-50.5,-0.770750430887795,-10.5970075386067));
#43533=CARTESIAN_POINT('Ctrl Pts',(-50.5,-0.770750430887802,-10.5970075386067));
#43534=CARTESIAN_POINT('Ctrl Pts',(-50.4694758939836,-0.75230208407391,
-10.5677446024392));
#43535=CARTESIAN_POINT('Ctrl Pts',(-50.437878488726,-0.729472368132695,
-10.5376844269166));
#43536=CARTESIAN_POINT('Ctrl Pts',(-50.2856976867209,-0.610696119298001,
-10.3931263178812));
#43537=CARTESIAN_POINT('Ctrl Pts',(-50.159960596002,-0.48621901035263,-10.2739529360615));
#43538=CARTESIAN_POINT('Ctrl Pts',(-50.,-0.37977419449275,-10.1178751010871));
#43539=CARTESIAN_POINT('Ctrl Pts',(-65.5,-0.770750430887794,-10.5970075386067));
#43540=CARTESIAN_POINT('Ctrl Pts',(-60.5,-0.770750430887794,-10.5970075386067));
#43541=CARTESIAN_POINT('Ctrl Pts',(-55.5,-0.770750430887795,-10.5970075386067));
#43542=CARTESIAN_POINT('Ctrl Pts',(-50.5,-0.770750430887795,-10.5970075386067));
#43543=CARTESIAN_POINT('Origin',(-66.,0.,0.));
#43544=CARTESIAN_POINT('',(-50.,1.53067287083626,-7.66108326625458));
#43545=CARTESIAN_POINT('',(-66.,1.53067287083626,-7.66108326625458));
#43546=CARTESIAN_POINT('Origin',(-50.,0.,0.));
#43547=CARTESIAN_POINT('Ctrl Pts',(-66.,3.51446816599279,-10.6606349956381));
#43548=CARTESIAN_POINT('Ctrl Pts',(-50.,3.51446816599279,-10.6606349956381));
#43549=CARTESIAN_POINT('Ctrl Pts',(-66.,3.49471085893672,-10.6475637798258));
#43550=CARTESIAN_POINT('Ctrl Pts',(-50.,3.49471085893672,-10.6475637798258));
#43551=CARTESIAN_POINT('Ctrl Pts',(-66.,3.45537023612148,-10.621297616078));
#43552=CARTESIAN_POINT('Ctrl Pts',(-50.,3.45537023612148,-10.621297616078));
#43553=CARTESIAN_POINT('Ctrl Pts',(-66.,3.39688127592428,-10.5815271743047));
#43554=CARTESIAN_POINT('Ctrl Pts',(-50.,3.39688127592428,-10.5815271743047));
#43555=CARTESIAN_POINT('Ctrl Pts',(-66.,3.31994133078549,-10.5277565371413));
#43556=CARTESIAN_POINT('Ctrl Pts',(-50.,3.31994133078549,-10.5277565371413));
#43557=CARTESIAN_POINT('Ctrl Pts',(-66.,3.22552017619803,-10.4592986611063));
#43558=CARTESIAN_POINT('Ctrl Pts',(-50.,3.22552017619803,-10.4592986611063));
#43559=CARTESIAN_POINT('Ctrl Pts',(-66.,3.13287341152958,-10.3895893192858));
#43560=CARTESIAN_POINT('Ctrl Pts',(-50.,3.13287341152958,-10.3895893192858));
#43561=CARTESIAN_POINT('Ctrl Pts',(-66.,3.04203169122768,-10.3186223773335));
#43562=CARTESIAN_POINT('Ctrl Pts',(-50.,3.04203169122768,-10.3186223773335));
#43563=CARTESIAN_POINT('Ctrl Pts',(-66.,2.95303632952095,-10.2463944394523));
#43564=CARTESIAN_POINT('Ctrl Pts',(-50.,2.95303632952095,-10.2463944394523));
#43565=CARTESIAN_POINT('Ctrl Pts',(-66.,2.86594045075721,-10.172907326731));
#43566=CARTESIAN_POINT('Ctrl Pts',(-50.,2.86594045075721,-10.172907326731));
#43567=CARTESIAN_POINT('Ctrl Pts',(-66.,2.78080594883332,-10.0981681361864));
#43568=CARTESIAN_POINT('Ctrl Pts',(-50.,2.78080594883332,-10.0981681361864));
#43569=CARTESIAN_POINT('Ctrl Pts',(-66.,2.69769949294062,-10.0221886955761));
#43570=CARTESIAN_POINT('Ctrl Pts',(-50.,2.69769949294062,-10.0221886955761));
#43571=CARTESIAN_POINT('Ctrl Pts',(-66.,2.61668829606168,-9.94498553626488));
#43572=CARTESIAN_POINT('Ctrl Pts',(-50.,2.61668829606168,-9.94498553626488));
#43573=CARTESIAN_POINT('Ctrl Pts',(-66.,2.53783659863859,-9.86657949215571));
#43574=CARTESIAN_POINT('Ctrl Pts',(-50.,2.53783659863859,-9.86657949215571));
#43575=CARTESIAN_POINT('Ctrl Pts',(-66.,2.46119946285178,-9.78699646071692));
#43576=CARTESIAN_POINT('Ctrl Pts',(-50.,2.46119946285178,-9.78699646071692));
#43577=CARTESIAN_POINT('Ctrl Pts',(-66.,2.38682820441919,-9.70626369932132));
#43578=CARTESIAN_POINT('Ctrl Pts',(-50.,2.38682820441919,-9.70626369932132));
#43579=CARTESIAN_POINT('Ctrl Pts',(-66.,2.31478185538763,-9.62440406213512));
#43580=CARTESIAN_POINT('Ctrl Pts',(-50.,2.31478185538763,-9.62440406213512));
#43581=CARTESIAN_POINT('Ctrl Pts',(-66.,2.24513642875384,-9.54143066294722));
#43582=CARTESIAN_POINT('Ctrl Pts',(-50.,2.24513642875384,-9.54143066294722));
#43583=CARTESIAN_POINT('Ctrl Pts',(-66.,2.17799511452139,-9.45734217317086));
#43584=CARTESIAN_POINT('Ctrl Pts',(-50.,2.17799511452139,-9.45734217317086));
#43585=CARTESIAN_POINT('Ctrl Pts',(-66.,2.11349742683576,-9.37211610318578));
#43586=CARTESIAN_POINT('Ctrl Pts',(-50.,2.11349742683576,-9.37211610318578));
#43587=CARTESIAN_POINT('Ctrl Pts',(-66.,2.05183036091841,-9.28571118746575));
#43588=CARTESIAN_POINT('Ctrl Pts',(-50.,2.05183036091841,-9.28571118746575));
#43589=CARTESIAN_POINT('Ctrl Pts',(-66.,1.99323835737743,-9.19807604064094));
#43590=CARTESIAN_POINT('Ctrl Pts',(-50.,1.99323835737743,-9.19807604064094));
#43591=CARTESIAN_POINT('Ctrl Pts',(-66.,1.93803736866688,-9.10915586281889));
#43592=CARTESIAN_POINT('Ctrl Pts',(-50.,1.93803736866688,-9.10915586281889));
#43593=CARTESIAN_POINT('Ctrl Pts',(-66.,1.88661896349422,-9.01890038196952));
#43594=CARTESIAN_POINT('Ctrl Pts',(-50.,1.88661896349422,-9.01890038196952));
#43595=CARTESIAN_POINT('Ctrl Pts',(-66.,1.83947938032835,-8.92727064057537));
#43596=CARTESIAN_POINT('Ctrl Pts',(-50.,1.83947938032835,-8.92727064057537));
#43597=CARTESIAN_POINT('Ctrl Pts',(-66.,1.79714183408573,-8.83425001254252));
#43598=CARTESIAN_POINT('Ctrl Pts',(-50.,1.79714183408573,-8.83425001254252));
#43599=CARTESIAN_POINT('Ctrl Pts',(-66.,1.76001840564001,-8.73985705693077));
#43600=CARTESIAN_POINT('Ctrl Pts',(-50.,1.76001840564001,-8.73985705693077));
#43601=CARTESIAN_POINT('Ctrl Pts',(-66.,1.72828159952138,-8.64415925811045));
#43602=CARTESIAN_POINT('Ctrl Pts',(-50.,1.72828159952138,-8.64415925811045));
#43603=CARTESIAN_POINT('Ctrl Pts',(-66.,1.70174735094098,-8.54728433152241));
#43604=CARTESIAN_POINT('Ctrl Pts',(-50.,1.70174735094098,-8.54728433152241));
#43605=CARTESIAN_POINT('Ctrl Pts',(-66.,1.67970691947077,-8.44943937069158));
#43606=CARTESIAN_POINT('Ctrl Pts',(-50.,1.67970691947077,-8.44943937069158));
#43607=CARTESIAN_POINT('Ctrl Pts',(-66.,1.66103994900115,-8.35088931899355));
#43608=CARTESIAN_POINT('Ctrl Pts',(-50.,1.66103994900115,-8.35088931899355));
#43609=CARTESIAN_POINT('Ctrl Pts',(-66.,1.64442807858968,-8.25192111283452));
#43610=CARTESIAN_POINT('Ctrl Pts',(-50.,1.64442807858968,-8.25192111283452));
#43611=CARTESIAN_POINT('Ctrl Pts',(-66.,1.62853781891495,-8.15281204423512));
#43612=CARTESIAN_POINT('Ctrl Pts',(-50.,1.62853781891495,-8.15281204423512));
#43613=CARTESIAN_POINT('Ctrl Pts',(-66.,1.61220661573863,-8.05379804635934));
#43614=CARTESIAN_POINT('Ctrl Pts',(-50.,1.61220661573863,-8.05379804635934));
#43615=CARTESIAN_POINT('Ctrl Pts',(-66.,1.59465171544125,-7.95503756783394));
#43616=CARTESIAN_POINT('Ctrl Pts',(-50.,1.59465171544125,-7.95503756783394));
#43617=CARTESIAN_POINT('Ctrl Pts',(-66.,1.5754164725369,-7.85662314056401));
#43618=CARTESIAN_POINT('Ctrl Pts',(-50.,1.5754164725369,-7.85662314056401));
#43619=CARTESIAN_POINT('Ctrl Pts',(-66.,1.55850498002059,-7.77820466719577));
#43620=CARTESIAN_POINT('Ctrl Pts',(-50.,1.55850498002059,-7.77820466719577));
#43621=CARTESIAN_POINT('Ctrl Pts',(-66.,1.54493370114459,-7.71957314695095));
#43622=CARTESIAN_POINT('Ctrl Pts',(-50.,1.54493370114459,-7.71957314695095));
#43623=CARTESIAN_POINT('Ctrl Pts',(-66.,1.53549215119571,-7.68056640390788));
#43624=CARTESIAN_POINT('Ctrl Pts',(-50.,1.53549215119571,-7.68056640390788));
#43625=CARTESIAN_POINT('Ctrl Pts',(-66.,1.53067287083627,-7.66108326625457));
#43626=CARTESIAN_POINT('Ctrl Pts',(-50.,1.53067287083627,-7.66108326625457));
#43627=CARTESIAN_POINT('Ctrl Pts',(-50.,2.48815856278712,-9.81451435204154));
#43628=CARTESIAN_POINT('Ctrl Pts',(-50.,2.48285278315604,-9.80896726509534));
#43629=CARTESIAN_POINT('Ctrl Pts',(-50.,2.46234274539512,-9.78744217177353));
#43630=CARTESIAN_POINT('Ctrl Pts',(-50.,2.4269715452022,-9.74976313360792));
#43631=CARTESIAN_POINT('Ctrl Pts',(-50.,2.37742992422592,-9.69558529830397));
#43632=CARTESIAN_POINT('Ctrl Pts',(-50.,2.31478185538763,-9.62440406213512));
#43633=CARTESIAN_POINT('Ctrl Pts',(-50.,2.24513642875384,-9.54143066294722));
#43634=CARTESIAN_POINT('Ctrl Pts',(-50.,2.17799511452139,-9.45734217317086));
#43635=CARTESIAN_POINT('Ctrl Pts',(-50.,2.11349742683576,-9.37211610318578));
#43636=CARTESIAN_POINT('Ctrl Pts',(-50.,2.05183036091841,-9.28571118746575));
#43637=CARTESIAN_POINT('Ctrl Pts',(-50.,1.99323835737743,-9.19807604064094));
#43638=CARTESIAN_POINT('Ctrl Pts',(-50.,1.93803736866688,-9.10915586281889));
#43639=CARTESIAN_POINT('Ctrl Pts',(-50.,1.88661896349422,-9.01890038196952));
#43640=CARTESIAN_POINT('Ctrl Pts',(-50.,1.83947938032835,-8.92727064057537));
#43641=CARTESIAN_POINT('Ctrl Pts',(-50.,1.79714183408573,-8.83425001254252));
#43642=CARTESIAN_POINT('Ctrl Pts',(-50.,1.76001840564001,-8.73985705693077));
#43643=CARTESIAN_POINT('Ctrl Pts',(-50.,1.72828159952138,-8.64415925811045));
#43644=CARTESIAN_POINT('Ctrl Pts',(-50.,1.70174735094098,-8.54728433152241));
#43645=CARTESIAN_POINT('Ctrl Pts',(-50.,1.67970691947077,-8.44943937069158));
#43646=CARTESIAN_POINT('Ctrl Pts',(-50.,1.66103994900115,-8.35088931899355));
#43647=CARTESIAN_POINT('Ctrl Pts',(-50.,1.64442807858968,-8.25192111283452));
#43648=CARTESIAN_POINT('Ctrl Pts',(-50.,1.62853781891495,-8.15281204423512));
#43649=CARTESIAN_POINT('Ctrl Pts',(-50.,1.61220661573863,-8.05379804635934));
#43650=CARTESIAN_POINT('Ctrl Pts',(-50.,1.59465171544125,-7.95503756783394));
#43651=CARTESIAN_POINT('Ctrl Pts',(-50.,1.5754164725369,-7.85662314056401));
#43652=CARTESIAN_POINT('Ctrl Pts',(-50.,1.55850498002059,-7.77820466719577));
#43653=CARTESIAN_POINT('Ctrl Pts',(-50.,1.54493370114459,-7.71957314695095));
#43654=CARTESIAN_POINT('Ctrl Pts',(-50.,1.53549215119571,-7.68056640390788));
#43655=CARTESIAN_POINT('Ctrl Pts',(-50.,1.53067287083627,-7.66108326625457));
#43656=CARTESIAN_POINT('Origin',(-50.,1.47877611889991,-9.39020011572736));
#43657=CARTESIAN_POINT('Origin',(-50.,0.,0.));
#43658=CARTESIAN_POINT('Origin',(-65.75,0.,0.));
#43659=CARTESIAN_POINT('',(-65.5,-1.48968674337242,-10.5200503043769));
#43660=CARTESIAN_POINT('Origin',(-65.5,0.,0.));
#43661=CARTESIAN_POINT('',(-66.,-1.71887666803992,-9.97803026654399));
#43662=CARTESIAN_POINT('Ctrl Pts',(-65.5,-1.48968674337242,-10.5200503043769));
#43663=CARTESIAN_POINT('Ctrl Pts',(-65.6641545839451,-1.57632238482973,
-10.3419900891876));
#43664=CARTESIAN_POINT('Ctrl Pts',(-65.8307068049194,-1.65322389214929,
-10.1611267872057));
#43665=CARTESIAN_POINT('Ctrl Pts',(-66.,-1.71887666803992,-9.97803026654399));
#43666=CARTESIAN_POINT('Origin',(-66.,0.,0.));
#43667=CARTESIAN_POINT('Origin',(-58.,0.,0.));
#43668=CARTESIAN_POINT('',(-50.5,-1.48968674337242,-10.5200503043769));
#43669=CARTESIAN_POINT('Origin',(-50.5,0.,0.));
#43670=CARTESIAN_POINT('Ctrl Pts',(-50.5,-1.48968674337242,-10.5200503043769));
#43671=CARTESIAN_POINT('Ctrl Pts',(-55.5,-1.48968674337242,-10.5200503043769));
#43672=CARTESIAN_POINT('Ctrl Pts',(-60.5,-1.48968674337242,-10.5200503043769));
#43673=CARTESIAN_POINT('Ctrl Pts',(-65.5,-1.48968674337242,-10.5200503043769));
#43674=CARTESIAN_POINT('Origin',(-50.25,0.,0.));
#43675=CARTESIAN_POINT('',(-50.,-1.71887666803992,-9.97803026654401));
#43676=CARTESIAN_POINT('Origin',(-50.,0.,0.));
#43677=CARTESIAN_POINT('Ctrl Pts',(-50.,-1.71887666803992,-9.97803026654401));
#43678=CARTESIAN_POINT('Ctrl Pts',(-50.1692931950804,-1.65322389214937,
-10.1611267872055));
#43679=CARTESIAN_POINT('Ctrl Pts',(-50.3358454160543,-1.57632238483005,
-10.341990089187));
#43680=CARTESIAN_POINT('Ctrl Pts',(-50.5,-1.48968674337242,-10.5200503043769));
#43681=CARTESIAN_POINT('Origin',(-66.,-2.46840926658957,-9.17984709653976));
#43682=CARTESIAN_POINT('',(-66.,-4.46225154398509,-9.08867075859846));
#43683=CARTESIAN_POINT('Origin',(-66.,0.,0.));
#43684=CARTESIAN_POINT('',(-66.,-1.71770404175135,-7.62132856363975));
#43685=CARTESIAN_POINT('Ctrl Pts',(-66.,-1.71770404175134,-7.62132856363975));
#43686=CARTESIAN_POINT('Ctrl Pts',(-66.,-1.72122591607555,-7.64108747345899));
#43687=CARTESIAN_POINT('Ctrl Pts',(-66.,-1.7284661027293,-7.68056213071507));
#43688=CARTESIAN_POINT('Ctrl Pts',(-66.,-1.73991571028055,-7.73964462612166));
#43689=CARTESIAN_POINT('Ctrl Pts',(-66.,-1.75636195972324,-7.81816198995797));
#43690=CARTESIAN_POINT('Ctrl Pts',(-66.,-1.77881844471932,-7.91589172108458));
#43691=CARTESIAN_POINT('Ctrl Pts',(-66.,-1.80295075079726,-8.01325412885256));
#43692=CARTESIAN_POINT('Ctrl Pts',(-66.,-1.8283040754312,-8.11035041561234));
#43693=CARTESIAN_POINT('Ctrl Pts',(-66.,-1.85409889074508,-8.20735420592021));
#43694=CARTESIAN_POINT('Ctrl Pts',(-66.,-1.87917718793209,-8.3045228175142));
#43695=CARTESIAN_POINT('Ctrl Pts',(-66.,-1.90220797905422,-8.40214531049858));
#43696=CARTESIAN_POINT('Ctrl Pts',(-66.,-1.92187017391035,-8.50049578112694));
#43697=CARTESIAN_POINT('Ctrl Pts',(-66.,-1.9370325140864,-8.59978788146503));
#43698=CARTESIAN_POINT('Ctrl Pts',(-66.,-1.94696330045856,-8.70012069286638));
#43699=CARTESIAN_POINT('Ctrl Pts',(-66.,-1.95144243492538,-8.80145240736443));
#43700=CARTESIAN_POINT('Ctrl Pts',(-66.,-1.95060005985058,-8.90365121100569));
#43701=CARTESIAN_POINT('Ctrl Pts',(-66.,-1.94480508119479,-9.00653254085416));
#43702=CARTESIAN_POINT('Ctrl Pts',(-66.,-1.93454224200995,-9.10989877492369));
#43703=CARTESIAN_POINT('Ctrl Pts',(-66.,-1.92028072414509,-9.21358366430839));
#43704=CARTESIAN_POINT('Ctrl Pts',(-66.,-1.90239869089103,-9.31747386945138));
#43705=CARTESIAN_POINT('Ctrl Pts',(-66.,-1.8812070683013,-9.42149094310496));
#43706=CARTESIAN_POINT('Ctrl Pts',(-66.,-1.85695006429591,-9.52558240518797));
#43707=CARTESIAN_POINT('Ctrl Pts',(-66.,-1.82981529171165,-9.6297098958258));
#43708=CARTESIAN_POINT('Ctrl Pts',(-66.,-1.79993935041505,-9.73383721479367));
#43709=CARTESIAN_POINT('Ctrl Pts',(-66.,-1.77165950874705,-9.82434577497958));
#43710=CARTESIAN_POINT('Ctrl Pts',(-66.,-1.74843709680056,-9.89399008293483));
#43711=CARTESIAN_POINT('Ctrl Pts',(-66.,-1.73144934303076,-9.94279836032739));
#43712=CARTESIAN_POINT('Ctrl Pts',(-66.,-1.72146753539781,-9.97080469546509));
#43713=CARTESIAN_POINT('Ctrl Pts',(-66.,-1.71887666803992,-9.97803026654399));
#43714=CARTESIAN_POINT('',(-66.,-3.09005277149946,-7.17542543124437));
#43715=CARTESIAN_POINT('Origin',(-66.,0.,0.));
#43716=CARTESIAN_POINT('Ctrl Pts',(-66.,-4.46225154398509,-9.08867075859846));
#43717=CARTESIAN_POINT('Ctrl Pts',(-66.,-4.44533037920078,-9.07821755385499));
#43718=CARTESIAN_POINT('Ctrl Pts',(-66.,-4.4061376895513,-9.05308941524767));
#43719=CARTESIAN_POINT('Ctrl Pts',(-66.,-4.34779553604197,-9.0122275525459));
#43720=CARTESIAN_POINT('Ctrl Pts',(-66.,-4.27471554428536,-8.95404675612808));
#43721=CARTESIAN_POINT('Ctrl Pts',(-66.,-4.18869845562393,-8.87735309244413));
#43722=CARTESIAN_POINT('Ctrl Pts',(-66.,-4.09879650191483,-8.79447108521983));
#43723=CARTESIAN_POINT('Ctrl Pts',(-66.,-4.00673750966012,-8.71051889651385));
#43724=CARTESIAN_POINT('Ctrl Pts',(-66.,-3.91326340492591,-8.62525611914553));
#43725=CARTESIAN_POINT('Ctrl Pts',(-66.,-3.82108601519994,-8.53797090566847));
#43726=CARTESIAN_POINT('Ctrl Pts',(-66.,-3.73373140850441,-8.44776484727783));
#43727=CARTESIAN_POINT('Ctrl Pts',(-66.,-3.65386752007281,-8.35395926054862));
#43728=CARTESIAN_POINT('Ctrl Pts',(-66.,-3.58245565425011,-8.25631176382647));
#43729=CARTESIAN_POINT('Ctrl Pts',(-66.,-3.519310217917,-8.15491356756456));
#43730=CARTESIAN_POINT('Ctrl Pts',(-66.,-3.46336527683772,-8.05015087702059));
#43731=CARTESIAN_POINT('Ctrl Pts',(-66.,-3.41306143963531,-7.9426466605421));
#43732=CARTESIAN_POINT('Ctrl Pts',(-66.,-3.36664638258854,-7.83320155109845));
#43733=CARTESIAN_POINT('Ctrl Pts',(-66.,-3.32235054612245,-7.72267344513691));
#43734=CARTESIAN_POINT('Ctrl Pts',(-66.,-3.2785699685588,-7.61187046781066));
#43735=CARTESIAN_POINT('Ctrl Pts',(-66.,-3.23405665229585,-7.5014332056376));
#43736=CARTESIAN_POINT('Ctrl Pts',(-66.,-3.18807993814955,-7.39173638112025));
#43737=CARTESIAN_POINT('Ctrl Pts',(-66.,-3.14983839200384,-7.30471982935151));
#43738=CARTESIAN_POINT('Ctrl Pts',(-66.,-3.12028455746335,-7.23990051415909));
#43739=CARTESIAN_POINT('Ctrl Pts',(-66.,-3.1001945982111,-7.19688434265714));
#43740=CARTESIAN_POINT('Ctrl Pts',(-66.,-3.09005277149946,-7.17542543124437));
#43741=CARTESIAN_POINT('Ctrl Pts',(-66.,-3.09005277149946,-7.17542543124437));
#43742=CARTESIAN_POINT('Ctrl Pts',(-50.,-3.09005277149946,-7.17542543124437));
#43743=CARTESIAN_POINT('Ctrl Pts',(-66.,-3.1001945982111,-7.19688434265714));
#43744=CARTESIAN_POINT('Ctrl Pts',(-50.,-3.1001945982111,-7.19688434265714));
#43745=CARTESIAN_POINT('Ctrl Pts',(-66.,-3.12028455746335,-7.23990051415909));
#43746=CARTESIAN_POINT('Ctrl Pts',(-50.,-3.12028455746335,-7.23990051415909));
#43747=CARTESIAN_POINT('Ctrl Pts',(-66.,-3.14983839200384,-7.30471982935151));
#43748=CARTESIAN_POINT('Ctrl Pts',(-50.,-3.14983839200384,-7.30471982935151));
#43749=CARTESIAN_POINT('Ctrl Pts',(-66.,-3.18807993814955,-7.39173638112025));
#43750=CARTESIAN_POINT('Ctrl Pts',(-50.,-3.18807993814955,-7.39173638112025));
#43751=CARTESIAN_POINT('Ctrl Pts',(-66.,-3.23405665229585,-7.5014332056376));
#43752=CARTESIAN_POINT('Ctrl Pts',(-50.,-3.23405665229585,-7.5014332056376));
#43753=CARTESIAN_POINT('Ctrl Pts',(-66.,-3.2785699685588,-7.61187046781066));
#43754=CARTESIAN_POINT('Ctrl Pts',(-50.,-3.2785699685588,-7.61187046781066));
#43755=CARTESIAN_POINT('Ctrl Pts',(-66.,-3.32235054612245,-7.72267344513691));
#43756=CARTESIAN_POINT('Ctrl Pts',(-50.,-3.32235054612245,-7.72267344513691));
#43757=CARTESIAN_POINT('Ctrl Pts',(-66.,-3.36664638258854,-7.83320155109845));
#43758=CARTESIAN_POINT('Ctrl Pts',(-50.,-3.36664638258854,-7.83320155109845));
#43759=CARTESIAN_POINT('Ctrl Pts',(-66.,-3.41306143963531,-7.9426466605421));
#43760=CARTESIAN_POINT('Ctrl Pts',(-50.,-3.41306143963531,-7.9426466605421));
#43761=CARTESIAN_POINT('Ctrl Pts',(-66.,-3.46336527683772,-8.05015087702059));
#43762=CARTESIAN_POINT('Ctrl Pts',(-50.,-3.46336527683772,-8.05015087702059));
#43763=CARTESIAN_POINT('Ctrl Pts',(-66.,-3.519310217917,-8.15491356756456));
#43764=CARTESIAN_POINT('Ctrl Pts',(-50.,-3.519310217917,-8.15491356756456));
#43765=CARTESIAN_POINT('Ctrl Pts',(-66.,-3.58245565425011,-8.25631176382647));
#43766=CARTESIAN_POINT('Ctrl Pts',(-50.,-3.58245565425011,-8.25631176382647));
#43767=CARTESIAN_POINT('Ctrl Pts',(-66.,-3.65386752007281,-8.35395926054862));
#43768=CARTESIAN_POINT('Ctrl Pts',(-50.,-3.65386752007281,-8.35395926054862));
#43769=CARTESIAN_POINT('Ctrl Pts',(-66.,-3.73373140850441,-8.44776484727783));
#43770=CARTESIAN_POINT('Ctrl Pts',(-50.,-3.73373140850441,-8.44776484727783));
#43771=CARTESIAN_POINT('Ctrl Pts',(-66.,-3.82108601519994,-8.53797090566847));
#43772=CARTESIAN_POINT('Ctrl Pts',(-50.,-3.82108601519994,-8.53797090566847));
#43773=CARTESIAN_POINT('Ctrl Pts',(-66.,-3.91326340492591,-8.62525611914553));
#43774=CARTESIAN_POINT('Ctrl Pts',(-50.,-3.91326340492591,-8.62525611914553));
#43775=CARTESIAN_POINT('Ctrl Pts',(-66.,-4.00673750966012,-8.71051889651385));
#43776=CARTESIAN_POINT('Ctrl Pts',(-50.,-4.00673750966012,-8.71051889651385));
#43777=CARTESIAN_POINT('Ctrl Pts',(-66.,-4.09879650191483,-8.79447108521983));
#43778=CARTESIAN_POINT('Ctrl Pts',(-50.,-4.09879650191483,-8.79447108521983));
#43779=CARTESIAN_POINT('Ctrl Pts',(-66.,-4.18869845562393,-8.87735309244413));
#43780=CARTESIAN_POINT('Ctrl Pts',(-50.,-4.18869845562393,-8.87735309244413));
#43781=CARTESIAN_POINT('Ctrl Pts',(-66.,-4.27965645364851,-8.95845211844488));
#43782=CARTESIAN_POINT('Ctrl Pts',(-50.,-4.27965645364851,-8.95845211844488));
#43783=CARTESIAN_POINT('Ctrl Pts',(-66.,-4.3781743773292,-9.03625199707944));
#43784=CARTESIAN_POINT('Ctrl Pts',(-50.,-4.3781743773292,-9.03625199707944));
#43785=CARTESIAN_POINT('Ctrl Pts',(-66.,-4.4903058862283,-9.10931646690967));
#43786=CARTESIAN_POINT('Ctrl Pts',(-50.,-4.4903058862283,-9.10931646690967));
#43787=CARTESIAN_POINT('Ctrl Pts',(-66.,-4.61889543384362,-9.17693917574169));
#43788=CARTESIAN_POINT('Ctrl Pts',(-50.,-4.61889543384362,-9.17693917574169));
#43789=CARTESIAN_POINT('Ctrl Pts',(-66.,-4.76000514096471,-9.23998558422727));
#43790=CARTESIAN_POINT('Ctrl Pts',(-50.,-4.76000514096471,-9.23998558422727));
#43791=CARTESIAN_POINT('Ctrl Pts',(-66.,-4.90085865419307,-9.30137962583606));
#43792=CARTESIAN_POINT('Ctrl Pts',(-50.,-4.90085865419307,-9.30137962583606));
#43793=CARTESIAN_POINT('Ctrl Pts',(-66.,-5.02348185505654,-9.36525860678472));
#43794=CARTESIAN_POINT('Ctrl Pts',(-50.,-5.02348185505654,-9.36525860678472));
#43795=CARTESIAN_POINT('Ctrl Pts',(-66.,-5.10755750085189,-9.43631208950852));
#43796=CARTESIAN_POINT('Ctrl Pts',(-50.,-5.10755750085189,-9.43631208950852));
#43797=CARTESIAN_POINT('Ctrl Pts',(-66.,-5.13345766798759,-9.51907903097904));
#43798=CARTESIAN_POINT('Ctrl Pts',(-50.,-5.13345766798759,-9.51907903097904));
#43799=CARTESIAN_POINT('Ctrl Pts',(-66.,-5.08549602968051,-9.61719469919379));
#43800=CARTESIAN_POINT('Ctrl Pts',(-50.,-5.08549602968051,-9.61719469919379));
#43801=CARTESIAN_POINT('Ctrl Pts',(-66.,-4.95176210550526,-9.73342698726024));
#43802=CARTESIAN_POINT('Ctrl Pts',(-50.,-4.95176210550526,-9.73342698726024));
#43803=CARTESIAN_POINT('Ctrl Pts',(-66.,-4.72347140525311,-9.86982476028545));
#43804=CARTESIAN_POINT('Ctrl Pts',(-50.,-4.72347140525311,-9.86982476028545));
#43805=CARTESIAN_POINT('Ctrl Pts',(-66.,-4.39451568841758,-10.0278201090025));
#43806=CARTESIAN_POINT('Ctrl Pts',(-50.,-4.39451568841758,-10.0278201090025));
#43807=CARTESIAN_POINT('Ctrl Pts',(-66.,-3.96095558080252,-10.2083440731201));
#43808=CARTESIAN_POINT('Ctrl Pts',(-50.,-3.96095558080252,-10.2083440731201));
#43809=CARTESIAN_POINT('Ctrl Pts',(-66.,-3.42056292700896,-10.4119310097664));
#43810=CARTESIAN_POINT('Ctrl Pts',(-50.,-3.42056292700896,-10.4119310097664));
#43811=CARTESIAN_POINT('Ctrl Pts',(-66.,-2.77236455694589,-10.6388227675402));
#43812=CARTESIAN_POINT('Ctrl Pts',(-50.,-2.77236455694589,-10.6388227675402));
#43813=CARTESIAN_POINT('Ctrl Pts',(-66.,-2.16743774120234,-10.8390192477456));
#43814=CARTESIAN_POINT('Ctrl Pts',(-50.,-2.16743774120234,-10.8390192477456));
#43815=CARTESIAN_POINT('Ctrl Pts',(-66.,-1.66526748642465,-10.9996550409518));
#43816=CARTESIAN_POINT('Ctrl Pts',(-50.,-1.66526748642465,-10.9996550409518));
#43817=CARTESIAN_POINT('Ctrl Pts',(-66.,-1.30897144914411,-11.1114008985485));
#43818=CARTESIAN_POINT('Ctrl Pts',(-50.,-1.30897144914411,-11.1114008985485));
#43819=CARTESIAN_POINT('Ctrl Pts',(-66.,-1.12544446210999,-11.1684376598836));
#43820=CARTESIAN_POINT('Ctrl Pts',(-50.,-1.12544446210999,-11.1684376598836));
#43821=CARTESIAN_POINT('',(-65.5,-5.01430682801544,-9.36735565858998));
#43822=CARTESIAN_POINT('Ctrl Pts',(-66.,-4.46225154398508,-9.08867075859845));
#43823=CARTESIAN_POINT('Ctrl Pts',(-65.798241770306,-4.6649736041553,-9.21390417059987));
#43824=CARTESIAN_POINT('Ctrl Pts',(-65.6331946192802,-4.8888287520727,-9.28344646526655));
#43825=CARTESIAN_POINT('Ctrl Pts',(-65.5,-5.01430682801543,-9.36735565858998));
#43826=CARTESIAN_POINT('',(-50.,-3.09005277149946,-7.17542543124437));
#43827=CARTESIAN_POINT('',(-66.,-3.09005277149946,-7.17542543124437));
#43828=CARTESIAN_POINT('',(-50.,-4.46225154398511,-9.08867075859847));
#43829=CARTESIAN_POINT('Ctrl Pts',(-50.,-3.09005277149946,-7.17542543124437));
#43830=CARTESIAN_POINT('Ctrl Pts',(-50.,-3.1001945982111,-7.19688434265714));
#43831=CARTESIAN_POINT('Ctrl Pts',(-50.,-3.12028455746335,-7.23990051415909));
#43832=CARTESIAN_POINT('Ctrl Pts',(-50.,-3.14983839200384,-7.30471982935151));
#43833=CARTESIAN_POINT('Ctrl Pts',(-50.,-3.18807993814955,-7.39173638112025));
#43834=CARTESIAN_POINT('Ctrl Pts',(-50.,-3.23405665229585,-7.5014332056376));
#43835=CARTESIAN_POINT('Ctrl Pts',(-50.,-3.2785699685588,-7.61187046781066));
#43836=CARTESIAN_POINT('Ctrl Pts',(-50.,-3.32235054612245,-7.72267344513691));
#43837=CARTESIAN_POINT('Ctrl Pts',(-50.,-3.36664638258854,-7.83320155109845));
#43838=CARTESIAN_POINT('Ctrl Pts',(-50.,-3.41306143963531,-7.9426466605421));
#43839=CARTESIAN_POINT('Ctrl Pts',(-50.,-3.46336527683772,-8.05015087702059));
#43840=CARTESIAN_POINT('Ctrl Pts',(-50.,-3.519310217917,-8.15491356756456));
#43841=CARTESIAN_POINT('Ctrl Pts',(-50.,-3.58245565425011,-8.25631176382647));
#43842=CARTESIAN_POINT('Ctrl Pts',(-50.,-3.65386752007281,-8.35395926054862));
#43843=CARTESIAN_POINT('Ctrl Pts',(-50.,-3.73373140850441,-8.44776484727783));
#43844=CARTESIAN_POINT('Ctrl Pts',(-50.,-3.82108601519994,-8.53797090566847));
#43845=CARTESIAN_POINT('Ctrl Pts',(-50.,-3.91326340492591,-8.62525611914553));
#43846=CARTESIAN_POINT('Ctrl Pts',(-50.,-4.00673750966012,-8.71051889651385));
#43847=CARTESIAN_POINT('Ctrl Pts',(-50.,-4.09879650191483,-8.79447108521983));
#43848=CARTESIAN_POINT('Ctrl Pts',(-50.,-4.18869845562393,-8.87735309244413));
#43849=CARTESIAN_POINT('Ctrl Pts',(-50.,-4.27471554428537,-8.95404675612808));
#43850=CARTESIAN_POINT('Ctrl Pts',(-50.,-4.34779553604197,-9.01222755254591));
#43851=CARTESIAN_POINT('Ctrl Pts',(-50.,-4.40613768955131,-9.05308941524767));
#43852=CARTESIAN_POINT('Ctrl Pts',(-50.,-4.4453303792008,-9.078217553855));
#43853=CARTESIAN_POINT('Ctrl Pts',(-50.,-4.46225154398511,-9.08867075859847));
#43854=CARTESIAN_POINT('',(-50.5,-5.01430682801544,-9.36735565858998));
#43855=CARTESIAN_POINT('Ctrl Pts',(-50.5,-5.01430682801073,-9.36735565858683));
#43856=CARTESIAN_POINT('Ctrl Pts',(-50.4646931597002,-4.98104387220113,
-9.3451121888133));
#43857=CARTESIAN_POINT('Ctrl Pts',(-50.4273092286687,-4.94135377127855,
-9.3238710729983));
#43858=CARTESIAN_POINT('Ctrl Pts',(-50.3882921463906,-4.89776472393815,
-9.3027242489053));
#43859=CARTESIAN_POINT('Ctrl Pts',(-50.3470342768248,-4.85167231710866,
-9.28036294305628));
#43860=CARTESIAN_POINT('Ctrl Pts',(-50.3039502825837,-4.80121938499207,
-9.25810755978088));
#43861=CARTESIAN_POINT('Ctrl Pts',(-50.2595650675693,-4.74936366142675,
-9.23486526462329));
#43862=CARTESIAN_POINT('Ctrl Pts',(-50.2356844321301,-4.7214636584754,-9.22236018208065));
#43863=CARTESIAN_POINT('Ctrl Pts',(-50.2117779267271,-4.69355955980766,
-9.20974769064843));
#43864=CARTESIAN_POINT('Ctrl Pts',(-50.187514972923,-4.66565475603887,-9.19668496860533));
#43865=CARTESIAN_POINT('Ctrl Pts',(-50.1572202993005,-4.63081287613014,
-9.18037488104914));
#43866=CARTESIAN_POINT('Ctrl Pts',(-50.1263699237746,-4.59596559770358,
-9.16336504760852));
#43867=CARTESIAN_POINT('Ctrl Pts',(-50.0943203555449,-4.5610688467911,-9.14496806771221));
#43868=CARTESIAN_POINT('Ctrl Pts',(-50.0678556302452,-4.53225307866182,
-9.1297768796185));
#43869=CARTESIAN_POINT('Ctrl Pts',(-50.0405732324447,-4.50340555423355,
-9.11363890457985));
#43870=CARTESIAN_POINT('Ctrl Pts',(-50.0121108541095,-4.47448813501866,
-9.09615015924532));
#43871=CARTESIAN_POINT('Ctrl Pts',(-50.0080976999835,-4.47041082078763,
-9.0936842714804));
#43872=CARTESIAN_POINT('Ctrl Pts',(-50.0040610871464,-4.46633203157711,
-9.09119151723395));
#43873=CARTESIAN_POINT('Ctrl Pts',(-50.,-4.46225154398511,-9.08867075859847));
#43874=CARTESIAN_POINT('Ctrl Pts',(-65.5,-5.01430682801544,-9.36735565858998));
#43875=CARTESIAN_POINT('Ctrl Pts',(-60.5,-5.01430682801544,-9.36735565858998));
#43876=CARTESIAN_POINT('Ctrl Pts',(-55.5,-5.01430682801544,-9.36735565858998));
#43877=CARTESIAN_POINT('Ctrl Pts',(-50.5,-5.01430682801544,-9.36735565858998));
#43878=CARTESIAN_POINT('Origin',(-66.,0.,0.));
#43879=CARTESIAN_POINT('',(-50.,-1.71770404175135,-7.62132856363975));
#43880=CARTESIAN_POINT('',(-66.,-1.71770404175135,-7.62132856363975));
#43881=CARTESIAN_POINT('Origin',(-50.,0.,0.));
#43882=CARTESIAN_POINT('Ctrl Pts',(-66.,-1.12544446210999,-11.1684376598836));
#43883=CARTESIAN_POINT('Ctrl Pts',(-50.,-1.12544446210999,-11.1684376598836));
#43884=CARTESIAN_POINT('Ctrl Pts',(-66.,-1.13817711778593,-11.1484604893043));
#43885=CARTESIAN_POINT('Ctrl Pts',(-50.,-1.13817711778593,-11.1484604893043));
#43886=CARTESIAN_POINT('Ctrl Pts',(-66.,-1.16343315379036,-11.1084638818624));
#43887=CARTESIAN_POINT('Ctrl Pts',(-50.,-1.16343315379036,-11.1084638818624));
#43888=CARTESIAN_POINT('Ctrl Pts',(-66.,-1.20068938172024,-11.0483421721043));
#43889=CARTESIAN_POINT('Ctrl Pts',(-50.,-1.20068938172024,-11.0483421721043));
#43890=CARTESIAN_POINT('Ctrl Pts',(-66.,-1.24910703065715,-10.9679259557649));
#43891=CARTESIAN_POINT('Ctrl Pts',(-50.,-1.24910703065715,-10.9679259557649));
#43892=CARTESIAN_POINT('Ctrl Pts',(-66.,-1.30752072084532,-10.8669820306211));
#43893=CARTESIAN_POINT('Ctrl Pts',(-50.,-1.30752072084532,-10.8669820306211));
#43894=CARTESIAN_POINT('Ctrl Pts',(-66.,-1.36380440819035,-10.7656165439926));
#43895=CARTESIAN_POINT('Ctrl Pts',(-50.,-1.36380440819035,-10.7656165439926));
#43896=CARTESIAN_POINT('Ctrl Pts',(-66.,-1.41792759339758,-10.6638363601625));
#43897=CARTESIAN_POINT('Ctrl Pts',(-50.,-1.41792759339758,-10.6638363601625));
#43898=CARTESIAN_POINT('Ctrl Pts',(-66.,-1.46985115284591,-10.5616551809262));
#43899=CARTESIAN_POINT('Ctrl Pts',(-50.,-1.46985115284591,-10.5616551809262));
#43900=CARTESIAN_POINT('Ctrl Pts',(-66.,-1.51952729573235,-10.4590962775504));
#43901=CARTESIAN_POINT('Ctrl Pts',(-50.,-1.51952729573235,-10.4590962775504));
#43902=CARTESIAN_POINT('Ctrl Pts',(-66.,-1.56690236578525,-10.356191307998));
#43903=CARTESIAN_POINT('Ctrl Pts',(-50.,-1.56690236578525,-10.356191307998));
#43904=CARTESIAN_POINT('Ctrl Pts',(-66.,-1.6119202684502,-10.2529781942665));
#43905=CARTESIAN_POINT('Ctrl Pts',(-50.,-1.6119202684502,-10.2529781942665));
#43906=CARTESIAN_POINT('Ctrl Pts',(-66.,-1.65452632552406,-10.149499376492));
#43907=CARTESIAN_POINT('Ctrl Pts',(-50.,-1.65452632552406,-10.149499376492));
#43908=CARTESIAN_POINT('Ctrl Pts',(-66.,-1.69467032435451,-10.0458000163337));
#43909=CARTESIAN_POINT('Ctrl Pts',(-50.,-1.69467032435451,-10.0458000163337));
#43910=CARTESIAN_POINT('Ctrl Pts',(-66.,-1.73231249658609,-9.94192616811245));
#43911=CARTESIAN_POINT('Ctrl Pts',(-50.,-1.73231249658609,-9.94192616811245));
#43912=CARTESIAN_POINT('Ctrl Pts',(-66.,-1.76741704955006,-9.83792360466036));
#43913=CARTESIAN_POINT('Ctrl Pts',(-50.,-1.76741704955006,-9.83792360466036));
#43914=CARTESIAN_POINT('Ctrl Pts',(-66.,-1.79993935041505,-9.73383721479367));
#43915=CARTESIAN_POINT('Ctrl Pts',(-50.,-1.79993935041505,-9.73383721479367));
#43916=CARTESIAN_POINT('Ctrl Pts',(-66.,-1.82981529171165,-9.6297098958258));
#43917=CARTESIAN_POINT('Ctrl Pts',(-50.,-1.82981529171165,-9.6297098958258));
#43918=CARTESIAN_POINT('Ctrl Pts',(-66.,-1.85695006429591,-9.52558240518797));
#43919=CARTESIAN_POINT('Ctrl Pts',(-50.,-1.85695006429591,-9.52558240518797));
#43920=CARTESIAN_POINT('Ctrl Pts',(-66.,-1.8812070683013,-9.42149094310496));
#43921=CARTESIAN_POINT('Ctrl Pts',(-50.,-1.8812070683013,-9.42149094310496));
#43922=CARTESIAN_POINT('Ctrl Pts',(-66.,-1.90239869089103,-9.31747386945138));
#43923=CARTESIAN_POINT('Ctrl Pts',(-50.,-1.90239869089103,-9.31747386945138));
#43924=CARTESIAN_POINT('Ctrl Pts',(-66.,-1.92028072414509,-9.21358366430839));
#43925=CARTESIAN_POINT('Ctrl Pts',(-50.,-1.92028072414509,-9.21358366430839));
#43926=CARTESIAN_POINT('Ctrl Pts',(-66.,-1.93454224200995,-9.10989877492369));
#43927=CARTESIAN_POINT('Ctrl Pts',(-50.,-1.93454224200995,-9.10989877492369));
#43928=CARTESIAN_POINT('Ctrl Pts',(-66.,-1.94480508119479,-9.00653254085416));
#43929=CARTESIAN_POINT('Ctrl Pts',(-50.,-1.94480508119479,-9.00653254085416));
#43930=CARTESIAN_POINT('Ctrl Pts',(-66.,-1.95060005985058,-8.90365121100569));
#43931=CARTESIAN_POINT('Ctrl Pts',(-50.,-1.95060005985058,-8.90365121100569));
#43932=CARTESIAN_POINT('Ctrl Pts',(-66.,-1.95144243492538,-8.80145240736443));
#43933=CARTESIAN_POINT('Ctrl Pts',(-50.,-1.95144243492538,-8.80145240736443));
#43934=CARTESIAN_POINT('Ctrl Pts',(-66.,-1.94696330045856,-8.70012069286638));
#43935=CARTESIAN_POINT('Ctrl Pts',(-50.,-1.94696330045856,-8.70012069286638));
#43936=CARTESIAN_POINT('Ctrl Pts',(-66.,-1.9370325140864,-8.59978788146503));
#43937=CARTESIAN_POINT('Ctrl Pts',(-50.,-1.9370325140864,-8.59978788146503));
#43938=CARTESIAN_POINT('Ctrl Pts',(-66.,-1.92187017391035,-8.50049578112694));
#43939=CARTESIAN_POINT('Ctrl Pts',(-50.,-1.92187017391035,-8.50049578112694));
#43940=CARTESIAN_POINT('Ctrl Pts',(-66.,-1.90220797905422,-8.40214531049858));
#43941=CARTESIAN_POINT('Ctrl Pts',(-50.,-1.90220797905422,-8.40214531049858));
#43942=CARTESIAN_POINT('Ctrl Pts',(-66.,-1.87917718793209,-8.3045228175142));
#43943=CARTESIAN_POINT('Ctrl Pts',(-50.,-1.87917718793209,-8.3045228175142));
#43944=CARTESIAN_POINT('Ctrl Pts',(-66.,-1.85409889074508,-8.20735420592021));
#43945=CARTESIAN_POINT('Ctrl Pts',(-50.,-1.85409889074508,-8.20735420592021));
#43946=CARTESIAN_POINT('Ctrl Pts',(-66.,-1.8283040754312,-8.11035041561234));
#43947=CARTESIAN_POINT('Ctrl Pts',(-50.,-1.8283040754312,-8.11035041561234));
#43948=CARTESIAN_POINT('Ctrl Pts',(-66.,-1.80295075079726,-8.01325412885256));
#43949=CARTESIAN_POINT('Ctrl Pts',(-50.,-1.80295075079726,-8.01325412885256));
#43950=CARTESIAN_POINT('Ctrl Pts',(-66.,-1.77881844471932,-7.91589172108458));
#43951=CARTESIAN_POINT('Ctrl Pts',(-50.,-1.77881844471932,-7.91589172108458));
#43952=CARTESIAN_POINT('Ctrl Pts',(-66.,-1.75636195972324,-7.81816198995797));
#43953=CARTESIAN_POINT('Ctrl Pts',(-50.,-1.75636195972324,-7.81816198995797));
#43954=CARTESIAN_POINT('Ctrl Pts',(-66.,-1.73991571028055,-7.73964462612166));
#43955=CARTESIAN_POINT('Ctrl Pts',(-50.,-1.73991571028055,-7.73964462612166));
#43956=CARTESIAN_POINT('Ctrl Pts',(-66.,-1.7284661027293,-7.68056213071507));
#43957=CARTESIAN_POINT('Ctrl Pts',(-50.,-1.7284661027293,-7.68056213071507));
#43958=CARTESIAN_POINT('Ctrl Pts',(-66.,-1.72122591607555,-7.64108747345899));
#43959=CARTESIAN_POINT('Ctrl Pts',(-50.,-1.72122591607555,-7.64108747345899));
#43960=CARTESIAN_POINT('Ctrl Pts',(-66.,-1.71770404175134,-7.62132856363975));
#43961=CARTESIAN_POINT('Ctrl Pts',(-50.,-1.71770404175134,-7.62132856363975));
#43962=CARTESIAN_POINT('Ctrl Pts',(-50.,-1.71887666803992,-9.97803026654401));
#43963=CARTESIAN_POINT('Ctrl Pts',(-50.,-1.7214675353978,-9.97080469546511));
#43964=CARTESIAN_POINT('Ctrl Pts',(-50.,-1.73144934303076,-9.9427983603274));
#43965=CARTESIAN_POINT('Ctrl Pts',(-50.,-1.74843709680056,-9.89399008293484));
#43966=CARTESIAN_POINT('Ctrl Pts',(-50.,-1.77165950874705,-9.82434577497958));
#43967=CARTESIAN_POINT('Ctrl Pts',(-50.,-1.79993935041505,-9.73383721479367));
#43968=CARTESIAN_POINT('Ctrl Pts',(-50.,-1.82981529171165,-9.6297098958258));
#43969=CARTESIAN_POINT('Ctrl Pts',(-50.,-1.85695006429591,-9.52558240518797));
#43970=CARTESIAN_POINT('Ctrl Pts',(-50.,-1.8812070683013,-9.42149094310496));
#43971=CARTESIAN_POINT('Ctrl Pts',(-50.,-1.90239869089103,-9.31747386945138));
#43972=CARTESIAN_POINT('Ctrl Pts',(-50.,-1.92028072414509,-9.21358366430839));
#43973=CARTESIAN_POINT('Ctrl Pts',(-50.,-1.93454224200995,-9.10989877492369));
#43974=CARTESIAN_POINT('Ctrl Pts',(-50.,-1.94480508119479,-9.00653254085416));
#43975=CARTESIAN_POINT('Ctrl Pts',(-50.,-1.95060005985058,-8.90365121100569));
#43976=CARTESIAN_POINT('Ctrl Pts',(-50.,-1.95144243492538,-8.80145240736443));
#43977=CARTESIAN_POINT('Ctrl Pts',(-50.,-1.94696330045856,-8.70012069286638));
#43978=CARTESIAN_POINT('Ctrl Pts',(-50.,-1.9370325140864,-8.59978788146503));
#43979=CARTESIAN_POINT('Ctrl Pts',(-50.,-1.92187017391035,-8.50049578112694));
#43980=CARTESIAN_POINT('Ctrl Pts',(-50.,-1.90220797905422,-8.40214531049858));
#43981=CARTESIAN_POINT('Ctrl Pts',(-50.,-1.87917718793209,-8.3045228175142));
#43982=CARTESIAN_POINT('Ctrl Pts',(-50.,-1.85409889074508,-8.20735420592021));
#43983=CARTESIAN_POINT('Ctrl Pts',(-50.,-1.8283040754312,-8.11035041561234));
#43984=CARTESIAN_POINT('Ctrl Pts',(-50.,-1.80295075079726,-8.01325412885256));
#43985=CARTESIAN_POINT('Ctrl Pts',(-50.,-1.77881844471932,-7.91589172108458));
#43986=CARTESIAN_POINT('Ctrl Pts',(-50.,-1.75636195972324,-7.81816198995797));
#43987=CARTESIAN_POINT('Ctrl Pts',(-50.,-1.73991571028055,-7.73964462612166));
#43988=CARTESIAN_POINT('Ctrl Pts',(-50.,-1.7284661027293,-7.68056213071507));
#43989=CARTESIAN_POINT('Ctrl Pts',(-50.,-1.72122591607555,-7.64108747345899));
#43990=CARTESIAN_POINT('Ctrl Pts',(-50.,-1.71770404175134,-7.62132856363975));
#43991=CARTESIAN_POINT('Origin',(-50.,-2.46840926658957,-9.17984709653976));
#43992=CARTESIAN_POINT('Origin',(-50.,0.,0.));
#43993=CARTESIAN_POINT('Origin',(-65.75,0.,0.));
#43994=CARTESIAN_POINT('',(-65.5,-5.63978650350908,-9.00463398450136));
#43995=CARTESIAN_POINT('Origin',(-65.5,0.,0.));
#43996=CARTESIAN_POINT('',(-66.,-5.62870250745855,-8.41625410040178));
#43997=CARTESIAN_POINT('Ctrl Pts',(-65.5,-5.63978650350908,-9.00463398450135));
#43998=CARTESIAN_POINT('Ctrl Pts',(-65.6642917360001,-5.64651410229415,
-8.8065646438819));
#43999=CARTESIAN_POINT('Ctrl Pts',(-65.8311182354836,-5.64316254881277,
-8.60975308169117));
#44000=CARTESIAN_POINT('Ctrl Pts',(-66.,-5.62870250745855,-8.41625410040178));
#44001=CARTESIAN_POINT('Origin',(-66.,0.,0.));
#44002=CARTESIAN_POINT('Origin',(-58.,0.,0.));
#44003=CARTESIAN_POINT('',(-50.5,-5.63978650350908,-9.00463398450136));
#44004=CARTESIAN_POINT('Origin',(-50.5,0.,0.));
#44005=CARTESIAN_POINT('Ctrl Pts',(-50.5,-5.63978650350908,-9.00463398450136));
#44006=CARTESIAN_POINT('Ctrl Pts',(-55.5,-5.63978650350908,-9.00463398450136));
#44007=CARTESIAN_POINT('Ctrl Pts',(-60.5,-5.63978650350908,-9.00463398450136));
#44008=CARTESIAN_POINT('Ctrl Pts',(-65.5,-5.63978650350908,-9.00463398450136));
#44009=CARTESIAN_POINT('Origin',(-50.25,0.,0.));
#44010=CARTESIAN_POINT('',(-50.,-5.62870250745855,-8.4162541004018));
#44011=CARTESIAN_POINT('Origin',(-50.,0.,0.));
#44012=CARTESIAN_POINT('Ctrl Pts',(-50.,-5.62870250745855,-8.4162541004018));
#44013=CARTESIAN_POINT('Ctrl Pts',(-50.1688817645161,-5.64316254881275,
-8.6097530816908));
#44014=CARTESIAN_POINT('Ctrl Pts',(-50.3357082639996,-5.64651410229418,
-8.8065646438815));
#44015=CARTESIAN_POINT('Ctrl Pts',(-50.5,-5.63978650350908,-9.00463398450137));
#44016=CARTESIAN_POINT('Origin',(-66.,-5.98878426509152,-7.38221511806768));
#44017=CARTESIAN_POINT('',(-66.,-7.77316506323978,-6.48795267396646));
#44018=CARTESIAN_POINT('Origin',(-66.,0.,0.));
#44019=CARTESIAN_POINT('',(-66.,-4.66907432066882,-6.26377691477522));
#44020=CARTESIAN_POINT('Ctrl Pts',(-66.,-4.66907432066881,-6.26377691477523));
#44021=CARTESIAN_POINT('Ctrl Pts',(-66.,-4.6803283856108,-6.2803951017486));
#44022=CARTESIAN_POINT('Ctrl Pts',(-66.,-4.70299841481972,-6.3135121463621));
#44023=CARTESIAN_POINT('Ctrl Pts',(-66.,-4.73748916763617,-6.36282971672706));
#44024=CARTESIAN_POINT('Ctrl Pts',(-66.,-4.78444945309974,-6.42786960551628));
#44025=CARTESIAN_POINT('Ctrl Pts',(-66.,-4.84471473572967,-6.50801628214104));
#44026=CARTESIAN_POINT('Ctrl Pts',(-66.,-4.90636155322694,-6.5871457743388));
#44027=CARTESIAN_POINT('Ctrl Pts',(-66.,-4.96901558551421,-6.66553551990974));
#44028=CARTESIAN_POINT('Ctrl Pts',(-66.,-5.03203531791038,-6.74366119533008));
#44029=CARTESIAN_POINT('Ctrl Pts',(-66.,-5.09446751728307,-6.82222887666531));
#44030=CARTESIAN_POINT('Ctrl Pts',(-66.,-5.15521383698376,-6.90204399502655));
#44031=CARTESIAN_POINT('Ctrl Pts',(-66.,-5.21317888605016,-6.98389428559481));
#44032=CARTESIAN_POINT('Ctrl Pts',(-66.,-5.26741610862069,-7.06843505349409));
#44033=CARTESIAN_POINT('Ctrl Pts',(-66.,-5.31729736430153,-7.15605442289018));
#44034=CARTESIAN_POINT('Ctrl Pts',(-66.,-5.36260457863992,-7.2468037222681));
#44035=CARTESIAN_POINT('Ctrl Pts',(-66.,-5.40340302903612,-7.34050959992121));
#44036=CARTESIAN_POINT('Ctrl Pts',(-66.,-5.43995465934573,-7.43685340164567));
#44037=CARTESIAN_POINT('Ctrl Pts',(-66.,-5.47262192427873,-7.53545742801198));
#44038=CARTESIAN_POINT('Ctrl Pts',(-66.,-5.50176582326021,-7.63597896963706));
#44039=CARTESIAN_POINT('Ctrl Pts',(-66.,-5.52768572629587,-7.73816067281613));
#44040=CARTESIAN_POINT('Ctrl Pts',(-66.,-5.55063377109937,-7.84180440740311));
#44041=CARTESIAN_POINT('Ctrl Pts',(-66.,-5.57081170713472,-7.94676290214864));
#44042=CARTESIAN_POINT('Ctrl Pts',(-66.,-5.58837532489015,-8.0529248045481));
#44043=CARTESIAN_POINT('Ctrl Pts',(-66.,-5.60343469059531,-8.16020148387941));
#44044=CARTESIAN_POINT('Ctrl Pts',(-66.,-5.6144129176363,-8.25438761578178));
#44045=CARTESIAN_POINT('Ctrl Pts',(-66.,-5.62152508071414,-8.3274562628442));
#44046=CARTESIAN_POINT('Ctrl Pts',(-66.,-5.62585811032315,-8.37895438489326));
#44047=CARTESIAN_POINT('Ctrl Pts',(-66.,-5.62813047803977,-8.40859941207198));
#44048=CARTESIAN_POINT('Ctrl Pts',(-66.,-5.62870250745855,-8.41625410040178));
#44049=CARTESIAN_POINT('',(-66.,-5.74141212582432,-5.29823961815974));
#44050=CARTESIAN_POINT('Origin',(-66.,0.,0.));
#44051=CARTESIAN_POINT('Ctrl Pts',(-66.,-7.77316506323978,-6.48795267396646));
#44052=CARTESIAN_POINT('Ctrl Pts',(-66.,-7.75345510860632,-6.48528565401655));
#44053=CARTESIAN_POINT('Ctrl Pts',(-66.,-7.70743027026035,-6.47827106015396));
#44054=CARTESIAN_POINT('Ctrl Pts',(-66.,-7.63751204406767,-6.46467178276015));
#44055=CARTESIAN_POINT('Ctrl Pts',(-66.,-7.5470858877274,-6.4412452909937));
#44056=CARTESIAN_POINT('Ctrl Pts',(-66.,-7.43731124378912,-6.40616844479457));
#44057=CARTESIAN_POINT('Ctrl Pts',(-66.,-7.32147057295518,-6.3670183824321));
#44058=CARTESIAN_POINT('Ctrl Pts',(-66.,-7.20322406733259,-6.32776800725522));
#44059=CARTESIAN_POINT('Ctrl Pts',(-66.,-7.08315172769933,-6.28789592785851));
#44060=CARTESIAN_POINT('Ctrl Pts',(-66.,-6.96344139729801,-6.24564883963181));
#44061=CARTESIAN_POINT('Ctrl Pts',(-66.,-6.84694888377224,-6.19877182422175));
#44062=CARTESIAN_POINT('Ctrl Pts',(-66.,-6.73583542181789,-6.14555972644743));
#44063=CARTESIAN_POINT('Ctrl Pts',(-66.,-6.63088062115226,-6.08540012194724));
#44064=CARTESIAN_POINT('Ctrl Pts',(-66.,-6.53195203265778,-6.0184518231387));
#44065=CARTESIAN_POINT('Ctrl Pts',(-66.,-6.43823296078527,-5.9455012005935));
#44066=CARTESIAN_POINT('Ctrl Pts',(-66.,-6.34855221468005,-5.86775162582969));
#44067=CARTESIAN_POINT('Ctrl Pts',(-66.,-6.26163461373259,-5.78664724772762));
#44068=CARTESIAN_POINT('Ctrl Pts',(-66.,-6.17621252275219,-5.70369153841107));
#44069=CARTESIAN_POINT('Ctrl Pts',(-66.,-6.09114934394547,-5.62027514693155));
#44070=CARTESIAN_POINT('Ctrl Pts',(-66.,-6.00556552478208,-5.53749088454784));
#44071=CARTESIAN_POINT('Ctrl Pts',(-66.,-5.91894598825613,-5.45597826316371));
#44072=CARTESIAN_POINT('Ctrl Pts',(-66.,-5.84861777732304,-5.392038925661));
#44073=CARTESIAN_POINT('Ctrl Pts',(-66.,-5.79525461535482,-5.34484416215046));
#44074=CARTESIAN_POINT('Ctrl Pts',(-66.,-5.75940527114103,-5.31371825665548));
#44075=CARTESIAN_POINT('Ctrl Pts',(-66.,-5.74141212582432,-5.29823961815974));
#44076=CARTESIAN_POINT('Ctrl Pts',(-66.,-5.74141212582432,-5.29823961815974));
#44077=CARTESIAN_POINT('Ctrl Pts',(-50.,-5.74141212582432,-5.29823961815974));
#44078=CARTESIAN_POINT('Ctrl Pts',(-66.,-5.75940527114103,-5.31371825665548));
#44079=CARTESIAN_POINT('Ctrl Pts',(-50.,-5.75940527114103,-5.31371825665548));
#44080=CARTESIAN_POINT('Ctrl Pts',(-66.,-5.79525461535482,-5.34484416215046));
#44081=CARTESIAN_POINT('Ctrl Pts',(-50.,-5.79525461535482,-5.34484416215046));
#44082=CARTESIAN_POINT('Ctrl Pts',(-66.,-5.84861777732304,-5.392038925661));
#44083=CARTESIAN_POINT('Ctrl Pts',(-50.,-5.84861777732304,-5.392038925661));
#44084=CARTESIAN_POINT('Ctrl Pts',(-66.,-5.91894598825613,-5.45597826316371));
#44085=CARTESIAN_POINT('Ctrl Pts',(-50.,-5.91894598825613,-5.45597826316371));
#44086=CARTESIAN_POINT('Ctrl Pts',(-66.,-6.00556552478208,-5.53749088454784));
#44087=CARTESIAN_POINT('Ctrl Pts',(-50.,-6.00556552478208,-5.53749088454784));
#44088=CARTESIAN_POINT('Ctrl Pts',(-66.,-6.09114934394547,-5.62027514693155));
#44089=CARTESIAN_POINT('Ctrl Pts',(-50.,-6.09114934394547,-5.62027514693155));
#44090=CARTESIAN_POINT('Ctrl Pts',(-66.,-6.17621252275219,-5.70369153841107));
#44091=CARTESIAN_POINT('Ctrl Pts',(-50.,-6.17621252275219,-5.70369153841107));
#44092=CARTESIAN_POINT('Ctrl Pts',(-66.,-6.26163461373259,-5.78664724772762));
#44093=CARTESIAN_POINT('Ctrl Pts',(-50.,-6.26163461373259,-5.78664724772762));
#44094=CARTESIAN_POINT('Ctrl Pts',(-66.,-6.34855221468005,-5.86775162582969));
#44095=CARTESIAN_POINT('Ctrl Pts',(-50.,-6.34855221468005,-5.86775162582969));
#44096=CARTESIAN_POINT('Ctrl Pts',(-66.,-6.43823296078527,-5.9455012005935));
#44097=CARTESIAN_POINT('Ctrl Pts',(-50.,-6.43823296078527,-5.9455012005935));
#44098=CARTESIAN_POINT('Ctrl Pts',(-66.,-6.53195203265778,-6.0184518231387));
#44099=CARTESIAN_POINT('Ctrl Pts',(-50.,-6.53195203265778,-6.0184518231387));
#44100=CARTESIAN_POINT('Ctrl Pts',(-66.,-6.63088062115226,-6.08540012194724));
#44101=CARTESIAN_POINT('Ctrl Pts',(-50.,-6.63088062115226,-6.08540012194724));
#44102=CARTESIAN_POINT('Ctrl Pts',(-66.,-6.73583542181789,-6.14555972644743));
#44103=CARTESIAN_POINT('Ctrl Pts',(-50.,-6.73583542181789,-6.14555972644743));
#44104=CARTESIAN_POINT('Ctrl Pts',(-66.,-6.84694888377224,-6.19877182422175));
#44105=CARTESIAN_POINT('Ctrl Pts',(-50.,-6.84694888377224,-6.19877182422175));
#44106=CARTESIAN_POINT('Ctrl Pts',(-66.,-6.96344139729801,-6.24564883963181));
#44107=CARTESIAN_POINT('Ctrl Pts',(-50.,-6.96344139729801,-6.24564883963181));
#44108=CARTESIAN_POINT('Ctrl Pts',(-66.,-7.08315172769933,-6.28789592785851));
#44109=CARTESIAN_POINT('Ctrl Pts',(-50.,-7.08315172769933,-6.28789592785851));
#44110=CARTESIAN_POINT('Ctrl Pts',(-66.,-7.20322406733259,-6.32776800725522));
#44111=CARTESIAN_POINT('Ctrl Pts',(-50.,-7.20322406733259,-6.32776800725522));
#44112=CARTESIAN_POINT('Ctrl Pts',(-66.,-7.32147057295518,-6.3670183824321));
#44113=CARTESIAN_POINT('Ctrl Pts',(-50.,-7.32147057295518,-6.3670183824321));
#44114=CARTESIAN_POINT('Ctrl Pts',(-66.,-7.43731124378912,-6.40616844479457));
#44115=CARTESIAN_POINT('Ctrl Pts',(-50.,-7.43731124378912,-6.40616844479457));
#44116=CARTESIAN_POINT('Ctrl Pts',(-66.,-7.553391455313,-6.44326014083938));
#44117=CARTESIAN_POINT('Ctrl Pts',(-50.,-7.553391455313,-6.44326014083938));
#44118=CARTESIAN_POINT('Ctrl Pts',(-66.,-7.6750361184554,-6.47426301701044));
#44119=CARTESIAN_POINT('Ctrl Pts',(-50.,-7.6750361184554,-6.47426301701044));
#44120=CARTESIAN_POINT('Ctrl Pts',(-66.,-7.80719134625564,-6.49540273802627));
#44121=CARTESIAN_POINT('Ctrl Pts',(-50.,-7.80719134625564,-6.49540273802627));
#44122=CARTESIAN_POINT('Ctrl Pts',(-66.,-7.95216837696596,-6.50487707558157));
#44123=CARTESIAN_POINT('Ctrl Pts',(-50.,-7.95216837696596,-6.50487707558157));
#44124=CARTESIAN_POINT('Ctrl Pts',(-66.,-8.10672179348113,-6.5050783470944));
#44125=CARTESIAN_POINT('Ctrl Pts',(-50.,-8.10672179348113,-6.5050783470944));
#44126=CARTESIAN_POINT('Ctrl Pts',(-66.,-8.2603690870727,-6.5038743097965));
#44127=CARTESIAN_POINT('Ctrl Pts',(-50.,-8.2603690870727,-6.5038743097965));
#44128=CARTESIAN_POINT('Ctrl Pts',(-66.,-8.39837287749729,-6.51235531359857));
#44129=CARTESIAN_POINT('Ctrl Pts',(-50.,-8.39837287749729,-6.51235531359857));
#44130=CARTESIAN_POINT('Ctrl Pts',(-66.,-8.50407985685393,-6.54306925405535));
#44131=CARTESIAN_POINT('Ctrl Pts',(-50.,-8.50407985685393,-6.54306925405535));
#44132=CARTESIAN_POINT('Ctrl Pts',(-66.,-8.5614051848243,-6.60814607044284));
#44133=CARTESIAN_POINT('Ctrl Pts',(-50.,-8.5614051848243,-6.60814607044284));
#44134=CARTESIAN_POINT('Ctrl Pts',(-66.,-8.55749728553057,-6.71728694922543));
#44135=CARTESIAN_POINT('Ctrl Pts',(-50.,-8.55749728553057,-6.71728694922543));
#44136=CARTESIAN_POINT('Ctrl Pts',(-66.,-8.48260119723272,-6.87786491540434));
#44137=CARTESIAN_POINT('Ctrl Pts',(-50.,-8.48260119723272,-6.87786491540434));
#44138=CARTESIAN_POINT('Ctrl Pts',(-66.,-8.32952523731861,-7.09532467445007));
#44139=CARTESIAN_POINT('Ctrl Pts',(-50.,-8.32952523731861,-7.09532467445007));
#44140=CARTESIAN_POINT('Ctrl Pts',(-66.,-8.0932717341967,-7.37345895158545));
#44141=CARTESIAN_POINT('Ctrl Pts',(-50.,-8.0932717341967,-7.37345895158545));
#44142=CARTESIAN_POINT('Ctrl Pts',(-66.,-7.77062057842988,-7.7147205817437));
#44143=CARTESIAN_POINT('Ctrl Pts',(-50.,-7.77062057842988,-7.7147205817437));
#44144=CARTESIAN_POINT('Ctrl Pts',(-66.,-7.35975359139894,-8.12050399689911));
#44145=CARTESIAN_POINT('Ctrl Pts',(-50.,-7.35975359139894,-8.12050399689911));
#44146=CARTESIAN_POINT('Ctrl Pts',(-66.,-6.85988010667493,-8.59142596067649));
#44147=CARTESIAN_POINT('Ctrl Pts',(-50.,-6.85988010667493,-8.59142596067649));
#44148=CARTESIAN_POINT('Ctrl Pts',(-66.,-6.38867920626058,-9.02036044814632));
#44149=CARTESIAN_POINT('Ctrl Pts',(-50.,-6.38867920626058,-9.02036044814632));
#44150=CARTESIAN_POINT('Ctrl Pts',(-66.,-5.99526031433169,-9.37135959104543));
#44151=CARTESIAN_POINT('Ctrl Pts',(-50.,-5.99526031433169,-9.37135959104543));
#44152=CARTESIAN_POINT('Ctrl Pts',(-66.,-5.71521882289448,-9.61836316580793));
#44153=CARTESIAN_POINT('Ctrl Pts',(-50.,-5.71521882289448,-9.61836316580793));
#44154=CARTESIAN_POINT('Ctrl Pts',(-66.,-5.57075751837199,-9.74511599066435));
#44155=CARTESIAN_POINT('Ctrl Pts',(-50.,-5.57075751837199,-9.74511599066435));
#44156=CARTESIAN_POINT('',(-65.5,-8.39084402103177,-6.51800288544853));
#44157=CARTESIAN_POINT('Ctrl Pts',(-66.,-7.77316506323978,-6.48795267396645));
#44158=CARTESIAN_POINT('Ctrl Pts',(-65.7982417703064,-8.00929789807026,
-6.51990459841432));
#44159=CARTESIAN_POINT('Ctrl Pts',(-65.6331946192803,-8.24208515110479,
-6.49238455442199));
#44160=CARTESIAN_POINT('Ctrl Pts',(-65.5,-8.39084402103177,-6.51800288544853));
#44161=CARTESIAN_POINT('',(-50.,-5.74141212582432,-5.29823961815974));
#44162=CARTESIAN_POINT('',(-66.,-5.74141212582432,-5.29823961815974));
#44163=CARTESIAN_POINT('',(-50.,-7.7731650632398,-6.48795267396646));
#44164=CARTESIAN_POINT('Ctrl Pts',(-50.,-5.74141212582432,-5.29823961815974));
#44165=CARTESIAN_POINT('Ctrl Pts',(-50.,-5.75940527114103,-5.31371825665548));
#44166=CARTESIAN_POINT('Ctrl Pts',(-50.,-5.79525461535482,-5.34484416215046));
#44167=CARTESIAN_POINT('Ctrl Pts',(-50.,-5.84861777732304,-5.392038925661));
#44168=CARTESIAN_POINT('Ctrl Pts',(-50.,-5.91894598825613,-5.45597826316371));
#44169=CARTESIAN_POINT('Ctrl Pts',(-50.,-6.00556552478208,-5.53749088454784));
#44170=CARTESIAN_POINT('Ctrl Pts',(-50.,-6.09114934394547,-5.62027514693155));
#44171=CARTESIAN_POINT('Ctrl Pts',(-50.,-6.17621252275219,-5.70369153841107));
#44172=CARTESIAN_POINT('Ctrl Pts',(-50.,-6.26163461373259,-5.78664724772762));
#44173=CARTESIAN_POINT('Ctrl Pts',(-50.,-6.34855221468005,-5.86775162582969));
#44174=CARTESIAN_POINT('Ctrl Pts',(-50.,-6.43823296078527,-5.9455012005935));
#44175=CARTESIAN_POINT('Ctrl Pts',(-50.,-6.53195203265778,-6.0184518231387));
#44176=CARTESIAN_POINT('Ctrl Pts',(-50.,-6.63088062115226,-6.08540012194724));
#44177=CARTESIAN_POINT('Ctrl Pts',(-50.,-6.73583542181789,-6.14555972644743));
#44178=CARTESIAN_POINT('Ctrl Pts',(-50.,-6.84694888377224,-6.19877182422175));
#44179=CARTESIAN_POINT('Ctrl Pts',(-50.,-6.96344139729801,-6.24564883963181));
#44180=CARTESIAN_POINT('Ctrl Pts',(-50.,-7.08315172769933,-6.28789592785851));
#44181=CARTESIAN_POINT('Ctrl Pts',(-50.,-7.20322406733259,-6.32776800725522));
#44182=CARTESIAN_POINT('Ctrl Pts',(-50.,-7.32147057295518,-6.3670183824321));
#44183=CARTESIAN_POINT('Ctrl Pts',(-50.,-7.43731124378912,-6.40616844479457));
#44184=CARTESIAN_POINT('Ctrl Pts',(-50.,-7.54708588772741,-6.44124529099371));
#44185=CARTESIAN_POINT('Ctrl Pts',(-50.,-7.63751204406767,-6.46467178276015));
#44186=CARTESIAN_POINT('Ctrl Pts',(-50.,-7.70743027026036,-6.47827106015396));
#44187=CARTESIAN_POINT('Ctrl Pts',(-50.,-7.75345510860633,-6.48528565401655));
#44188=CARTESIAN_POINT('Ctrl Pts',(-50.,-7.7731650632398,-6.48795267396646));
#44189=CARTESIAN_POINT('',(-50.5,-8.39084402103177,-6.51800288544853));
#44190=CARTESIAN_POINT('Ctrl Pts',(-50.5,-8.39084402103178,-6.51800288544854));
#44191=CARTESIAN_POINT('Ctrl Pts',(-50.49825670698,-8.38889701820982,-6.5176675846841));
#44192=CARTESIAN_POINT('Ctrl Pts',(-50.4965113438761,-8.3869400955467,-6.51734148071378));
#44193=CARTESIAN_POINT('Ctrl Pts',(-50.3581212730775,-8.23119318026662,
-6.49221711279462));
#44194=CARTESIAN_POINT('Ctrl Pts',(-50.2022201285458,-8.00983849304637,
-6.51997774813044));
#44195=CARTESIAN_POINT('Ctrl Pts',(-50.,-7.7731650632398,-6.48795267396646));
#44196=CARTESIAN_POINT('Ctrl Pts',(-65.5,-8.39084402103177,-6.51800288544853));
#44197=CARTESIAN_POINT('Ctrl Pts',(-60.5,-8.39084402103177,-6.51800288544853));
#44198=CARTESIAN_POINT('Ctrl Pts',(-55.5,-8.39084402103177,-6.51800288544853));
#44199=CARTESIAN_POINT('Ctrl Pts',(-50.5,-8.39084402103177,-6.51800288544853));
#44200=CARTESIAN_POINT('Origin',(-66.,0.,0.));
#44201=CARTESIAN_POINT('',(-50.,-4.66907432066882,-6.26377691477522));
#44202=CARTESIAN_POINT('',(-66.,-4.66907432066882,-6.26377691477522));
#44203=CARTESIAN_POINT('Origin',(-50.,0.,0.));
#44204=CARTESIAN_POINT('Ctrl Pts',(-66.,-5.57075751837199,-9.74511599066435));
#44205=CARTESIAN_POINT('Ctrl Pts',(-50.,-5.57075751837199,-9.74511599066435));
#44206=CARTESIAN_POINT('Ctrl Pts',(-66.,-5.57426393082888,-9.72168709959797));
#44207=CARTESIAN_POINT('Ctrl Pts',(-50.,-5.57426393082888,-9.72168709959797));
#44208=CARTESIAN_POINT('Ctrl Pts',(-66.,-5.58106838195346,-9.67487582524648));
#44209=CARTESIAN_POINT('Ctrl Pts',(-50.,-5.58106838195346,-9.67487582524648));
#44210=CARTESIAN_POINT('Ctrl Pts',(-66.,-5.59064993734473,-9.60479843730945));
#44211=CARTESIAN_POINT('Ctrl Pts',(-50.,-5.59064993734473,-9.60479843730945));
#44212=CARTESIAN_POINT('Ctrl Pts',(-66.,-5.60217343871804,-9.51164133615758));
#44213=CARTESIAN_POINT('Ctrl Pts',(-50.,-5.60217343871804,-9.51164133615758));
#44214=CARTESIAN_POINT('Ctrl Pts',(-66.,-5.61447940680167,-9.39566548360896));
#44215=CARTESIAN_POINT('Ctrl Pts',(-50.,-5.61447940680167,-9.39566548360896));
#44216=CARTESIAN_POINT('Ctrl Pts',(-66.,-5.62466805596007,-9.28017086568711));
#44217=CARTESIAN_POINT('Ctrl Pts',(-50.,-5.62466805596007,-9.28017086568711));
#44218=CARTESIAN_POINT('Ctrl Pts',(-66.,-5.63271431565661,-9.16517615840736));
#44219=CARTESIAN_POINT('Ctrl Pts',(-50.,-5.63271431565661,-9.16517615840736));
#44220=CARTESIAN_POINT('Ctrl Pts',(-66.,-5.63858801770719,-9.05070979199298));
#44221=CARTESIAN_POINT('Ctrl Pts',(-50.,-5.63858801770719,-9.05070979199298));
#44222=CARTESIAN_POINT('Ctrl Pts',(-66.,-5.64225496831767,-8.93681246407458));
#44223=CARTESIAN_POINT('Ctrl Pts',(-50.,-5.64225496831767,-8.93681246407458));
#44224=CARTESIAN_POINT('Ctrl Pts',(-66.,-5.64367902649844,-8.82353491961232));
#44225=CARTESIAN_POINT('Ctrl Pts',(-50.,-5.64367902649844,-8.82353491961232));
#44226=CARTESIAN_POINT('Ctrl Pts',(-66.,-5.64282437159007,-8.71093461778555));
#44227=CARTESIAN_POINT('Ctrl Pts',(-50.,-5.64282437159007,-8.71093461778555));
#44228=CARTESIAN_POINT('Ctrl Pts',(-66.,-5.63965831452689,-8.5990725692165));
#44229=CARTESIAN_POINT('Ctrl Pts',(-50.,-5.63965831452689,-8.5990725692165));
#44230=CARTESIAN_POINT('Ctrl Pts',(-66.,-5.63415335267014,-8.48801045445945));
#44231=CARTESIAN_POINT('Ctrl Pts',(-50.,-5.63415335267014,-8.48801045445945));
#44232=CARTESIAN_POINT('Ctrl Pts',(-66.,-5.62629188779924,-8.37780652147756));
#44233=CARTESIAN_POINT('Ctrl Pts',(-50.,-5.62629188779924,-8.37780652147756));
#44234=CARTESIAN_POINT('Ctrl Pts',(-66.,-5.61605983917227,-8.26851714402347));
#44235=CARTESIAN_POINT('Ctrl Pts',(-50.,-5.61605983917227,-8.26851714402347));
#44236=CARTESIAN_POINT('Ctrl Pts',(-66.,-5.60343469059531,-8.16020148387941));
#44237=CARTESIAN_POINT('Ctrl Pts',(-50.,-5.60343469059531,-8.16020148387941));
#44238=CARTESIAN_POINT('Ctrl Pts',(-66.,-5.58837532489015,-8.0529248045481));
#44239=CARTESIAN_POINT('Ctrl Pts',(-50.,-5.58837532489015,-8.0529248045481));
#44240=CARTESIAN_POINT('Ctrl Pts',(-66.,-5.57081170713472,-7.94676290214864));
#44241=CARTESIAN_POINT('Ctrl Pts',(-50.,-5.57081170713472,-7.94676290214864));
#44242=CARTESIAN_POINT('Ctrl Pts',(-66.,-5.55063377109937,-7.84180440740311));
#44243=CARTESIAN_POINT('Ctrl Pts',(-50.,-5.55063377109937,-7.84180440740311));
#44244=CARTESIAN_POINT('Ctrl Pts',(-66.,-5.52768572629587,-7.73816067281613));
#44245=CARTESIAN_POINT('Ctrl Pts',(-50.,-5.52768572629587,-7.73816067281613));
#44246=CARTESIAN_POINT('Ctrl Pts',(-66.,-5.50176582326021,-7.63597896963706));
#44247=CARTESIAN_POINT('Ctrl Pts',(-50.,-5.50176582326021,-7.63597896963706));
#44248=CARTESIAN_POINT('Ctrl Pts',(-66.,-5.47262192427873,-7.53545742801198));
#44249=CARTESIAN_POINT('Ctrl Pts',(-50.,-5.47262192427873,-7.53545742801198));
#44250=CARTESIAN_POINT('Ctrl Pts',(-66.,-5.43995465934573,-7.43685340164567));
#44251=CARTESIAN_POINT('Ctrl Pts',(-50.,-5.43995465934573,-7.43685340164567));
#44252=CARTESIAN_POINT('Ctrl Pts',(-66.,-5.40340302903612,-7.34050959992121));
#44253=CARTESIAN_POINT('Ctrl Pts',(-50.,-5.40340302903612,-7.34050959992121));
#44254=CARTESIAN_POINT('Ctrl Pts',(-66.,-5.36260457863992,-7.2468037222681));
#44255=CARTESIAN_POINT('Ctrl Pts',(-50.,-5.36260457863992,-7.2468037222681));
#44256=CARTESIAN_POINT('Ctrl Pts',(-66.,-5.31729736430153,-7.15605442289018));
#44257=CARTESIAN_POINT('Ctrl Pts',(-50.,-5.31729736430153,-7.15605442289018));
#44258=CARTESIAN_POINT('Ctrl Pts',(-66.,-5.26741610862069,-7.06843505349409));
#44259=CARTESIAN_POINT('Ctrl Pts',(-50.,-5.26741610862069,-7.06843505349409));
#44260=CARTESIAN_POINT('Ctrl Pts',(-66.,-5.21317888605016,-6.98389428559481));
#44261=CARTESIAN_POINT('Ctrl Pts',(-50.,-5.21317888605016,-6.98389428559481));
#44262=CARTESIAN_POINT('Ctrl Pts',(-66.,-5.15521383698376,-6.90204399502655));
#44263=CARTESIAN_POINT('Ctrl Pts',(-50.,-5.15521383698376,-6.90204399502655));
#44264=CARTESIAN_POINT('Ctrl Pts',(-66.,-5.09446751728307,-6.82222887666531));
#44265=CARTESIAN_POINT('Ctrl Pts',(-50.,-5.09446751728307,-6.82222887666531));
#44266=CARTESIAN_POINT('Ctrl Pts',(-66.,-5.03203531791038,-6.74366119533008));
#44267=CARTESIAN_POINT('Ctrl Pts',(-50.,-5.03203531791038,-6.74366119533008));
#44268=CARTESIAN_POINT('Ctrl Pts',(-66.,-4.96901558551421,-6.66553551990974));
#44269=CARTESIAN_POINT('Ctrl Pts',(-50.,-4.96901558551421,-6.66553551990974));
#44270=CARTESIAN_POINT('Ctrl Pts',(-66.,-4.90636155322694,-6.5871457743388));
#44271=CARTESIAN_POINT('Ctrl Pts',(-50.,-4.90636155322694,-6.5871457743388));
#44272=CARTESIAN_POINT('Ctrl Pts',(-66.,-4.84471473572967,-6.50801628214104));
#44273=CARTESIAN_POINT('Ctrl Pts',(-50.,-4.84471473572967,-6.50801628214104));
#44274=CARTESIAN_POINT('Ctrl Pts',(-66.,-4.78444945309974,-6.42786960551628));
#44275=CARTESIAN_POINT('Ctrl Pts',(-50.,-4.78444945309974,-6.42786960551628));
#44276=CARTESIAN_POINT('Ctrl Pts',(-66.,-4.73748916763617,-6.36282971672706));
#44277=CARTESIAN_POINT('Ctrl Pts',(-50.,-4.73748916763617,-6.36282971672706));
#44278=CARTESIAN_POINT('Ctrl Pts',(-66.,-4.70299841481972,-6.3135121463621));
#44279=CARTESIAN_POINT('Ctrl Pts',(-50.,-4.70299841481972,-6.3135121463621));
#44280=CARTESIAN_POINT('Ctrl Pts',(-66.,-4.6803283856108,-6.2803951017486));
#44281=CARTESIAN_POINT('Ctrl Pts',(-50.,-4.6803283856108,-6.2803951017486));
#44282=CARTESIAN_POINT('Ctrl Pts',(-66.,-4.66907432066881,-6.26377691477523));
#44283=CARTESIAN_POINT('Ctrl Pts',(-50.,-4.66907432066881,-6.26377691477523));
#44284=CARTESIAN_POINT('Ctrl Pts',(-50.,-5.62870250745855,-8.4162541004018));
#44285=CARTESIAN_POINT('Ctrl Pts',(-50.,-5.62813047803977,-8.40859941207199));
#44286=CARTESIAN_POINT('Ctrl Pts',(-50.,-5.62585811032315,-8.37895438489327));
#44287=CARTESIAN_POINT('Ctrl Pts',(-50.,-5.62152508071414,-8.3274562628442));
#44288=CARTESIAN_POINT('Ctrl Pts',(-50.,-5.6144129176363,-8.25438761578178));
#44289=CARTESIAN_POINT('Ctrl Pts',(-50.,-5.60343469059531,-8.16020148387941));
#44290=CARTESIAN_POINT('Ctrl Pts',(-50.,-5.58837532489015,-8.0529248045481));
#44291=CARTESIAN_POINT('Ctrl Pts',(-50.,-5.57081170713472,-7.94676290214864));
#44292=CARTESIAN_POINT('Ctrl Pts',(-50.,-5.55063377109937,-7.84180440740311));
#44293=CARTESIAN_POINT('Ctrl Pts',(-50.,-5.52768572629587,-7.73816067281613));
#44294=CARTESIAN_POINT('Ctrl Pts',(-50.,-5.50176582326021,-7.63597896963706));
#44295=CARTESIAN_POINT('Ctrl Pts',(-50.,-5.47262192427873,-7.53545742801198));
#44296=CARTESIAN_POINT('Ctrl Pts',(-50.,-5.43995465934573,-7.43685340164567));
#44297=CARTESIAN_POINT('Ctrl Pts',(-50.,-5.40340302903612,-7.34050959992121));
#44298=CARTESIAN_POINT('Ctrl Pts',(-50.,-5.36260457863992,-7.2468037222681));
#44299=CARTESIAN_POINT('Ctrl Pts',(-50.,-5.31729736430153,-7.15605442289018));
#44300=CARTESIAN_POINT('Ctrl Pts',(-50.,-5.26741610862069,-7.06843505349409));
#44301=CARTESIAN_POINT('Ctrl Pts',(-50.,-5.21317888605016,-6.98389428559481));
#44302=CARTESIAN_POINT('Ctrl Pts',(-50.,-5.15521383698376,-6.90204399502655));
#44303=CARTESIAN_POINT('Ctrl Pts',(-50.,-5.09446751728307,-6.82222887666531));
#44304=CARTESIAN_POINT('Ctrl Pts',(-50.,-5.03203531791038,-6.74366119533008));
#44305=CARTESIAN_POINT('Ctrl Pts',(-50.,-4.96901558551421,-6.66553551990974));
#44306=CARTESIAN_POINT('Ctrl Pts',(-50.,-4.90636155322694,-6.5871457743388));
#44307=CARTESIAN_POINT('Ctrl Pts',(-50.,-4.84471473572967,-6.50801628214104));
#44308=CARTESIAN_POINT('Ctrl Pts',(-50.,-4.78444945309974,-6.42786960551628));
#44309=CARTESIAN_POINT('Ctrl Pts',(-50.,-4.73748916763617,-6.36282971672706));
#44310=CARTESIAN_POINT('Ctrl Pts',(-50.,-4.70299841481972,-6.3135121463621));
#44311=CARTESIAN_POINT('Ctrl Pts',(-50.,-4.6803283856108,-6.2803951017486));
#44312=CARTESIAN_POINT('Ctrl Pts',(-50.,-4.66907432066881,-6.26377691477523));
#44313=CARTESIAN_POINT('Origin',(-50.,-5.98878426509152,-7.38221511806768));
#44314=CARTESIAN_POINT('Origin',(-50.,0.,0.));
#44315=CARTESIAN_POINT('Origin',(-65.75,0.,0.));
#44316=CARTESIAN_POINT('',(-65.5,-8.81471594133711,-5.93223464417393));
#44317=CARTESIAN_POINT('Origin',(-65.5,0.,0.));
#44318=CARTESIAN_POINT('',(-66.,-8.56527454818064,-5.39923114103193));
#44319=CARTESIAN_POINT('Ctrl Pts',(-65.5,-8.81471594133711,-5.93223464417392));
#44320=CARTESIAN_POINT('Ctrl Pts',(-65.6642917360001,-8.74029984994827,
-5.74855293680691));
#44321=CARTESIAN_POINT('Ctrl Pts',(-65.8311182354827,-8.6571875793658,-5.57011982776901));
#44322=CARTESIAN_POINT('Ctrl Pts',(-66.,-8.56527454818064,-5.39923114103193));
#44323=CARTESIAN_POINT('Origin',(-66.,0.,0.));
#44324=CARTESIAN_POINT('Origin',(-58.,0.,0.));
#44325=CARTESIAN_POINT('',(-50.5,-8.81471594133712,-5.93223464417392));
#44326=CARTESIAN_POINT('Origin',(-50.5,0.,0.));
#44327=CARTESIAN_POINT('Ctrl Pts',(-50.5,-8.81471594133712,-5.93223464417392));
#44328=CARTESIAN_POINT('Ctrl Pts',(-55.5,-8.81471594133712,-5.93223464417392));
#44329=CARTESIAN_POINT('Ctrl Pts',(-60.5,-8.81471594133712,-5.93223464417392));
#44330=CARTESIAN_POINT('Ctrl Pts',(-65.5,-8.81471594133712,-5.93223464417392));
#44331=CARTESIAN_POINT('Origin',(-50.25,0.,0.));
#44332=CARTESIAN_POINT('',(-50.,-8.56527454818065,-5.39923114103194));
#44333=CARTESIAN_POINT('Origin',(-50.,0.,0.));
#44334=CARTESIAN_POINT('Ctrl Pts',(-50.,-8.56527454818065,-5.39923114103195));
#44335=CARTESIAN_POINT('Ctrl Pts',(-50.1688817645164,-8.65718757936533,
-5.57011982776812));
#44336=CARTESIAN_POINT('Ctrl Pts',(-50.335708263999,-8.74029984994787,-5.74855293680593));
#44337=CARTESIAN_POINT('Ctrl Pts',(-50.5,-8.81471594133712,-5.93223464417393));
#44338=CARTESIAN_POINT('Origin',(-66.,-8.4736440577621,-4.30813108036277));
#44339=CARTESIAN_POINT('',(-66.,-9.74002772607264,-2.76540863080598));
#44340=CARTESIAN_POINT('Origin',(-66.,0.,0.));
#44341=CARTESIAN_POINT('',(-66.,-6.81311923233408,-3.82316133271923));
#44342=CARTESIAN_POINT('Ctrl Pts',(-66.,-6.81311923233407,-3.82316133271924));
#44343=CARTESIAN_POINT('Ctrl Pts',(-66.,-6.8301595578254,-3.83376536134756));
#44344=CARTESIAN_POINT('Ctrl Pts',(-66.,-6.86433957558852,-3.8547985554459));
#44345=CARTESIAN_POINT('Ctrl Pts',(-66.,-6.91590770916956,-3.88582374481706));
#44346=CARTESIAN_POINT('Ctrl Pts',(-66.,-6.98526217067656,-3.92614017091869));
#44347=CARTESIAN_POINT('Ctrl Pts',(-66.,-7.0729158360807,-3.97484570454348));
#44348=CARTESIAN_POINT('Ctrl Pts',(-66.,-7.16141787020827,-4.02206007310117));
#44349=CARTESIAN_POINT('Ctrl Pts',(-66.,-7.25053915877239,-4.06818897832557));
#44350=CARTESIAN_POINT('Ctrl Pts',(-66.,-7.33988712400327,-4.11392789982873));
#44351=CARTESIAN_POINT('Ctrl Pts',(-66.,-7.42887813111136,-4.16030958503735));
#44352=CARTESIAN_POINT('Ctrl Pts',(-66.,-7.51683638885138,-4.2085165697132));
#44353=CARTESIAN_POINT('Ctrl Pts',(-66.,-7.60308160854854,-4.25971402139557));
#44354=CARTESIAN_POINT('Ctrl Pts',(-66.,-7.68701560500139,-4.31488559005748));
#44355=CARTESIAN_POINT('Ctrl Pts',(-66.,-7.76822240772673,-4.37464133248276));
#44356=CARTESIAN_POINT('Ctrl Pts',(-66.,-7.84652367297445,-4.43911683844659));
#44357=CARTESIAN_POINT('Ctrl Pts',(-66.,-7.92190852612585,-4.50812719257416));
#44358=CARTESIAN_POINT('Ctrl Pts',(-66.,-7.9944866564592,-4.58127474760048));
#44359=CARTESIAN_POINT('Ctrl Pts',(-66.,-8.06443555863034,-4.65806703431538));
#44360=CARTESIAN_POINT('Ctrl Pts',(-66.,-8.13194562956026,-4.73804414042434));
#44361=CARTESIAN_POINT('Ctrl Pts',(-66.,-8.19718568217584,-4.82084919686819));
#44362=CARTESIAN_POINT('Ctrl Pts',(-66.,-8.26030546894961,-4.90619864910471));
#44363=CARTESIAN_POINT('Ctrl Pts',(-66.,-8.32142939657439,-4.99387589925328));
#44364=CARTESIAN_POINT('Ctrl Pts',(-66.,-8.38065449559913,-5.08371585603889));
#44365=CARTESIAN_POINT('Ctrl Pts',(-66.,-8.43804526716559,-5.17559278329922));
#44366=CARTESIAN_POINT('Ctrl Pts',(-66.,-8.48638332772613,-5.25717084905798));
#44367=CARTESIAN_POINT('Ctrl Pts',(-66.,-8.52260030822015,-5.32102960234266));
#44368=CARTESIAN_POINT('Ctrl Pts',(-66.,-8.54750490102424,-5.36631307590019));
#44369=CARTESIAN_POINT('Ctrl Pts',(-66.,-8.56163853106841,-5.39247090060411));
#44370=CARTESIAN_POINT('Ctrl Pts',(-66.,-8.56527454818064,-5.39923114103193));
#44371=CARTESIAN_POINT('',(-66.,-7.40002916450246,-2.50494004209942));
#44372=CARTESIAN_POINT('Origin',(-66.,0.,0.));
#44373=CARTESIAN_POINT('Ctrl Pts',(-66.,-9.74002772607264,-2.76540863080598));
#44374=CARTESIAN_POINT('Ctrl Pts',(-66.,-9.72093701180546,-2.7709889476281));
#44375=CARTESIAN_POINT('Ctrl Pts',(-66.,-9.67603813743555,-2.78330078551466));
#44376=CARTESIAN_POINT('Ctrl Pts',(-66.,-9.60663333505538,-2.79931553203575));
#44377=CARTESIAN_POINT('Ctrl Pts',(-66.,-9.51449651805853,-2.8146939981701));
#44378=CARTESIAN_POINT('Ctrl Pts',(-66.,-9.39994535205166,-2.82729907482675));
#44379=CARTESIAN_POINT('Ctrl Pts',(-66.,-9.27819586845952,-2.83865035877574));
#44380=CARTESIAN_POINT('Ctrl Pts',(-66.,-9.15420774452698,-2.85088854357451));
#44381=CARTESIAN_POINT('Ctrl Pts',(-66.,-9.02829876834023,-2.86330140690357));
#44382=CARTESIAN_POINT('Ctrl Pts',(-66.,-8.90175450092416,-2.87339734928437));
#44383=CARTESIAN_POINT('Ctrl Pts',(-66.,-8.77626669445802,-2.87795483868359));
#44384=CARTESIAN_POINT('Ctrl Pts',(-66.,-8.65311618598693,-2.87453708498607));
#44385=CARTESIAN_POINT('Ctrl Pts',(-66.,-8.53276608899787,-2.86226751485878));
#44386=CARTESIAN_POINT('Ctrl Pts',(-66.,-8.41516000003073,-2.84134508257382));
#44387=CARTESIAN_POINT('Ctrl Pts',(-66.,-8.29987167630279,-2.81282035340105));
#44388=CARTESIAN_POINT('Ctrl Pts',(-66.,-8.18632063702037,-2.77826902816129));
#44389=CARTESIAN_POINT('Ctrl Pts',(-66.,-8.07392933499764,-2.7395290651848));
#44390=CARTESIAN_POINT('Ctrl Pts',(-66.,-7.96215124506878,-2.69848954828302));
#44391=CARTESIAN_POINT('Ctrl Pts',(-66.,-7.85051366140938,-2.65688319455118));
#44392=CARTESIAN_POINT('Ctrl Pts',(-66.,-7.73865755918351,-2.61606608299436));
#44393=CARTESIAN_POINT('Ctrl Pts',(-66.,-7.62637250505703,-2.5768319374997));
#44394=CARTESIAN_POINT('Ctrl Pts',(-66.,-7.53611801591863,-2.54702550658787));
#44395=CARTESIAN_POINT('Ctrl Pts',(-66.,-7.46817250201609,-2.52561569812117));
#44396=CARTESIAN_POINT('Ctrl Pts',(-66.,-7.42276245013638,-2.5117620104632));
#44397=CARTESIAN_POINT('Ctrl Pts',(-66.,-7.40002916450246,-2.50494004209942));
#44398=CARTESIAN_POINT('Ctrl Pts',(-66.,-7.40002916450246,-2.50494004209942));
#44399=CARTESIAN_POINT('Ctrl Pts',(-50.,-7.40002916450246,-2.50494004209942));
#44400=CARTESIAN_POINT('Ctrl Pts',(-66.,-7.42276245013638,-2.5117620104632));
#44401=CARTESIAN_POINT('Ctrl Pts',(-50.,-7.42276245013638,-2.5117620104632));
#44402=CARTESIAN_POINT('Ctrl Pts',(-66.,-7.46817250201609,-2.52561569812117));
#44403=CARTESIAN_POINT('Ctrl Pts',(-50.,-7.46817250201609,-2.52561569812117));
#44404=CARTESIAN_POINT('Ctrl Pts',(-66.,-7.53611801591863,-2.54702550658787));
#44405=CARTESIAN_POINT('Ctrl Pts',(-50.,-7.53611801591863,-2.54702550658787));
#44406=CARTESIAN_POINT('Ctrl Pts',(-66.,-7.62637250505703,-2.5768319374997));
#44407=CARTESIAN_POINT('Ctrl Pts',(-50.,-7.62637250505703,-2.5768319374997));
#44408=CARTESIAN_POINT('Ctrl Pts',(-66.,-7.73865755918351,-2.61606608299436));
#44409=CARTESIAN_POINT('Ctrl Pts',(-50.,-7.73865755918351,-2.61606608299436));
#44410=CARTESIAN_POINT('Ctrl Pts',(-66.,-7.85051366140938,-2.65688319455118));
#44411=CARTESIAN_POINT('Ctrl Pts',(-50.,-7.85051366140938,-2.65688319455118));
#44412=CARTESIAN_POINT('Ctrl Pts',(-66.,-7.96215124506878,-2.69848954828302));
#44413=CARTESIAN_POINT('Ctrl Pts',(-50.,-7.96215124506878,-2.69848954828302));
#44414=CARTESIAN_POINT('Ctrl Pts',(-66.,-8.07392933499764,-2.7395290651848));
#44415=CARTESIAN_POINT('Ctrl Pts',(-50.,-8.07392933499764,-2.7395290651848));
#44416=CARTESIAN_POINT('Ctrl Pts',(-66.,-8.18632063702037,-2.77826902816129));
#44417=CARTESIAN_POINT('Ctrl Pts',(-50.,-8.18632063702037,-2.77826902816129));
#44418=CARTESIAN_POINT('Ctrl Pts',(-66.,-8.29987167630279,-2.81282035340105));
#44419=CARTESIAN_POINT('Ctrl Pts',(-50.,-8.29987167630279,-2.81282035340105));
#44420=CARTESIAN_POINT('Ctrl Pts',(-66.,-8.41516000003073,-2.84134508257382));
#44421=CARTESIAN_POINT('Ctrl Pts',(-50.,-8.41516000003073,-2.84134508257382));
#44422=CARTESIAN_POINT('Ctrl Pts',(-66.,-8.53276608899787,-2.86226751485878));
#44423=CARTESIAN_POINT('Ctrl Pts',(-50.,-8.53276608899787,-2.86226751485878));
#44424=CARTESIAN_POINT('Ctrl Pts',(-66.,-8.65311618598693,-2.87453708498607));
#44425=CARTESIAN_POINT('Ctrl Pts',(-50.,-8.65311618598693,-2.87453708498607));
#44426=CARTESIAN_POINT('Ctrl Pts',(-66.,-8.77626669445802,-2.87795483868359));
#44427=CARTESIAN_POINT('Ctrl Pts',(-50.,-8.77626669445802,-2.87795483868359));
#44428=CARTESIAN_POINT('Ctrl Pts',(-66.,-8.90175450092416,-2.87339734928437));
#44429=CARTESIAN_POINT('Ctrl Pts',(-50.,-8.90175450092416,-2.87339734928437));
#44430=CARTESIAN_POINT('Ctrl Pts',(-66.,-9.02829876834023,-2.86330140690357));
#44431=CARTESIAN_POINT('Ctrl Pts',(-50.,-9.02829876834023,-2.86330140690357));
#44432=CARTESIAN_POINT('Ctrl Pts',(-66.,-9.15420774452698,-2.85088854357451));
#44433=CARTESIAN_POINT('Ctrl Pts',(-50.,-9.15420774452698,-2.85088854357451));
#44434=CARTESIAN_POINT('Ctrl Pts',(-66.,-9.27819586845952,-2.83865035877574));
#44435=CARTESIAN_POINT('Ctrl Pts',(-50.,-9.27819586845952,-2.83865035877574));
#44436=CARTESIAN_POINT('Ctrl Pts',(-66.,-9.39994535205166,-2.82729907482675));
#44437=CARTESIAN_POINT('Ctrl Pts',(-50.,-9.39994535205166,-2.82729907482675));
#44438=CARTESIAN_POINT('Ctrl Pts',(-66.,-9.52107645394674,-2.813969949702));
#44439=CARTESIAN_POINT('Ctrl Pts',(-50.,-9.52107645394674,-2.813969949702));
#44440=CARTESIAN_POINT('Ctrl Pts',(-66.,-9.64481438918646,-2.7928151444673));
#44441=CARTESIAN_POINT('Ctrl Pts',(-50.,-9.64481438918646,-2.7928151444673));
#44442=CARTESIAN_POINT('Ctrl Pts',(-66.,-9.77414249640863,-2.75837486685676));
#44443=CARTESIAN_POINT('Ctrl Pts',(-50.,-9.77414249640863,-2.75837486685676));
#44444=CARTESIAN_POINT('Ctrl Pts',(-66.,-9.91043916452916,-2.70806263410035));
#44445=CARTESIAN_POINT('Ctrl Pts',(-50.,-9.91043916452916,-2.70806263410035));
#44446=CARTESIAN_POINT('Ctrl Pts',(-66.,-10.0517126006492,-2.64538396696739));
#44447=CARTESIAN_POINT('Ctrl Pts',(-50.,-10.0517126006492,-2.64538396696739));
#44448=CARTESIAN_POINT('Ctrl Pts',(-66.,-10.1915866617002,-2.58179003974993));
#44449=CARTESIAN_POINT('Ctrl Pts',(-50.,-10.1915866617002,-2.58179003974993));
#44450=CARTESIAN_POINT('Ctrl Pts',(-66.,-10.3211089325964,-2.53340662380053));
#44451=CARTESIAN_POINT('Ctrl Pts',(-50.,-10.3211089325964,-2.53340662380053));
#44452=CARTESIAN_POINT('Ctrl Pts',(-66.,-10.4301695484658,-2.51847030265793));
#44453=CARTESIAN_POINT('Ctrl Pts',(-50.,-10.4301695484658,-2.51847030265793));
#44454=CARTESIAN_POINT('Ctrl Pts',(-66.,-10.5090079672805,-2.55460462120467));
#44455=CARTESIAN_POINT('Ctrl Pts',(-50.,-10.5090079672805,-2.55460462120467));
#44456=CARTESIAN_POINT('Ctrl Pts',(-66.,-10.5498295182902,-2.65589926109984));
#44457=CARTESIAN_POINT('Ctrl Pts',(-50.,-10.5498295182902,-2.65589926109984));
#44458=CARTESIAN_POINT('Ctrl Pts',(-66.,-10.546721479946,-2.83305751623384));
#44459=CARTESIAN_POINT('Ctrl Pts',(-50.,-10.546721479946,-2.83305751623384));
#44460=CARTESIAN_POINT('Ctrl Pts',(-66.,-10.4953284844905,-3.09397849340119));
#44461=CARTESIAN_POINT('Ctrl Pts',(-50.,-10.4953284844905,-3.09397849340119));
#44462=CARTESIAN_POINT('Ctrl Pts',(-66.,-10.3926275720677,-3.44415975566763));
#44463=CARTESIAN_POINT('Ctrl Pts',(-50.,-10.3926275720677,-3.44415975566763));
#44464=CARTESIAN_POINT('Ctrl Pts',(-66.,-10.236674684175,-3.88715181574754));
#44465=CARTESIAN_POINT('Ctrl Pts',(-50.,-10.236674684175,-3.88715181574754));
#44466=CARTESIAN_POINT('Ctrl Pts',(-66.,-10.0263759985737,-4.4249680705051));
#44467=CARTESIAN_POINT('Ctrl Pts',(-50.,-10.0263759985737,-4.4249680705051));
#44468=CARTESIAN_POINT('Ctrl Pts',(-66.,-9.76126006590556,-5.0584935545573));
#44469=CARTESIAN_POINT('Ctrl Pts',(-50.,-9.76126006590556,-5.0584935545573));
#44470=CARTESIAN_POINT('Ctrl Pts',(-66.,-9.50525999722784,-5.64199937966045));
#44471=CARTESIAN_POINT('Ctrl Pts',(-50.,-9.50525999722784,-5.64199937966045));
#44472=CARTESIAN_POINT('Ctrl Pts',(-66.,-9.28861816866069,-6.12267093171814));
#44473=CARTESIAN_POINT('Ctrl Pts',(-50.,-9.28861816866069,-6.12267093171814));
#44474=CARTESIAN_POINT('Ctrl Pts',(-66.,-9.13325294103339,-6.46222306161301));
#44475=CARTESIAN_POINT('Ctrl Pts',(-50.,-9.13325294103339,-6.46222306161301));
#44476=CARTESIAN_POINT('Ctrl Pts',(-66.,-9.05283599096422,-6.63677523505979));
#44477=CARTESIAN_POINT('Ctrl Pts',(-50.,-9.05283599096422,-6.63677523505979));
#44478=CARTESIAN_POINT('',(-65.5,-10.3165280543869,-2.54162819921576));
#44479=CARTESIAN_POINT('Ctrl Pts',(-66.,-9.74002772607264,-2.76540863080598));
#44480=CARTESIAN_POINT('Ctrl Pts',(-65.7982417703062,-9.96874182322222,
-2.6985542896893));
#44481=CARTESIAN_POINT('Ctrl Pts',(-65.6331946192802,-10.1702101505182,
-2.5787303726559));
#44482=CARTESIAN_POINT('Ctrl Pts',(-65.5,-10.3165280543869,-2.54162819921576));
#44483=CARTESIAN_POINT('',(-50.,-7.40002916450246,-2.50494004209942));
#44484=CARTESIAN_POINT('',(-66.,-7.40002916450246,-2.50494004209942));
#44485=CARTESIAN_POINT('',(-50.,-9.74002772607266,-2.76540863080597));
#44486=CARTESIAN_POINT('Ctrl Pts',(-50.,-7.40002916450246,-2.50494004209942));
#44487=CARTESIAN_POINT('Ctrl Pts',(-50.,-7.42276245013638,-2.5117620104632));
#44488=CARTESIAN_POINT('Ctrl Pts',(-50.,-7.46817250201609,-2.52561569812117));
#44489=CARTESIAN_POINT('Ctrl Pts',(-50.,-7.53611801591863,-2.54702550658787));
#44490=CARTESIAN_POINT('Ctrl Pts',(-50.,-7.62637250505703,-2.5768319374997));
#44491=CARTESIAN_POINT('Ctrl Pts',(-50.,-7.73865755918351,-2.61606608299436));
#44492=CARTESIAN_POINT('Ctrl Pts',(-50.,-7.85051366140938,-2.65688319455118));
#44493=CARTESIAN_POINT('Ctrl Pts',(-50.,-7.96215124506878,-2.69848954828302));
#44494=CARTESIAN_POINT('Ctrl Pts',(-50.,-8.07392933499764,-2.7395290651848));
#44495=CARTESIAN_POINT('Ctrl Pts',(-50.,-8.18632063702037,-2.77826902816129));
#44496=CARTESIAN_POINT('Ctrl Pts',(-50.,-8.29987167630279,-2.81282035340105));
#44497=CARTESIAN_POINT('Ctrl Pts',(-50.,-8.41516000003073,-2.84134508257382));
#44498=CARTESIAN_POINT('Ctrl Pts',(-50.,-8.53276608899787,-2.86226751485878));
#44499=CARTESIAN_POINT('Ctrl Pts',(-50.,-8.65311618598693,-2.87453708498607));
#44500=CARTESIAN_POINT('Ctrl Pts',(-50.,-8.77626669445802,-2.87795483868359));
#44501=CARTESIAN_POINT('Ctrl Pts',(-50.,-8.90175450092416,-2.87339734928437));
#44502=CARTESIAN_POINT('Ctrl Pts',(-50.,-9.02829876834023,-2.86330140690357));
#44503=CARTESIAN_POINT('Ctrl Pts',(-50.,-9.15420774452698,-2.85088854357451));
#44504=CARTESIAN_POINT('Ctrl Pts',(-50.,-9.27819586845952,-2.83865035877574));
#44505=CARTESIAN_POINT('Ctrl Pts',(-50.,-9.39994535205166,-2.82729907482675));
#44506=CARTESIAN_POINT('Ctrl Pts',(-50.,-9.51449651805853,-2.8146939981701));
#44507=CARTESIAN_POINT('Ctrl Pts',(-50.,-9.60663333505539,-2.79931553203575));
#44508=CARTESIAN_POINT('Ctrl Pts',(-50.,-9.67603813743556,-2.78330078551466));
#44509=CARTESIAN_POINT('Ctrl Pts',(-50.,-9.72093701180547,-2.77098894762809));
#44510=CARTESIAN_POINT('Ctrl Pts',(-50.,-9.74002772607266,-2.76540863080597));
#44511=CARTESIAN_POINT('',(-50.5,-10.3165280543869,-2.54162819921576));
#44512=CARTESIAN_POINT('Ctrl Pts',(-50.5,-10.3165280543869,-2.54162819921576));
#44513=CARTESIAN_POINT('Ctrl Pts',(-50.4982567069806,-10.3146129996962,
-2.54211380411715));
#44514=CARTESIAN_POINT('Ctrl Pts',(-50.4965113438773,-10.3126926234528,
-2.54261184547092));
#44515=CARTESIAN_POINT('Ctrl Pts',(-50.3581212730791,-10.1601917353906,
-2.5830075707719));
#44516=CARTESIAN_POINT('Ctrl Pts',(-50.2022201285467,-9.969265433978,-2.69840123549405));
#44517=CARTESIAN_POINT('Ctrl Pts',(-50.,-9.74002772607266,-2.76540863080597));
#44518=CARTESIAN_POINT('Ctrl Pts',(-65.5,-10.3165280543869,-2.54162819921576));
#44519=CARTESIAN_POINT('Ctrl Pts',(-60.5,-10.3165280543869,-2.54162819921576));
#44520=CARTESIAN_POINT('Ctrl Pts',(-55.5,-10.3165280543869,-2.54162819921576));
#44521=CARTESIAN_POINT('Ctrl Pts',(-50.5,-10.3165280543869,-2.54162819921576));
#44522=CARTESIAN_POINT('Origin',(-66.,0.,0.));
#44523=CARTESIAN_POINT('',(-50.,-6.81311923233408,-3.82316133271923));
#44524=CARTESIAN_POINT('',(-66.,-6.81311923233408,-3.82316133271923));
#44525=CARTESIAN_POINT('Origin',(-50.,0.,0.));
#44526=CARTESIAN_POINT('Ctrl Pts',(-66.,-9.05283599096422,-6.63677523505979));
#44527=CARTESIAN_POINT('Ctrl Pts',(-50.,-9.05283599096422,-6.63677523505979));
#44528=CARTESIAN_POINT('Ctrl Pts',(-66.,-9.04650986963351,-6.61394569161654));
#44529=CARTESIAN_POINT('Ctrl Pts',(-50.,-9.04650986963351,-6.61394569161654));
#44530=CARTESIAN_POINT('Ctrl Pts',(-66.,-9.03368618446229,-6.56841384495789));
#44531=CARTESIAN_POINT('Ctrl Pts',(-50.,-9.03368618446229,-6.56841384495789));
#44532=CARTESIAN_POINT('Ctrl Pts',(-66.,-9.01393632934211,-6.50049779584927));
#44533=CARTESIAN_POINT('Ctrl Pts',(-50.,-9.01393632934211,-6.50049779584927));
#44534=CARTESIAN_POINT('Ctrl Pts',(-66.,-8.98657316507665,-6.41070751897976));
#44535=CARTESIAN_POINT('Ctrl Pts',(-50.,-8.98657316507665,-6.41070751897976));
#44536=CARTESIAN_POINT('Ctrl Pts',(-66.,-8.95064359737786,-6.29975301753961));
#44537=CARTESIAN_POINT('Ctrl Pts',(-50.,-8.95064359737786,-6.29975301753961));
#44538=CARTESIAN_POINT('Ctrl Pts',(-66.,-8.91297549834918,-6.19009933699878));
#44539=CARTESIAN_POINT('Ctrl Pts',(-50.,-8.91297549834918,-6.19009933699878));
#44540=CARTESIAN_POINT('Ctrl Pts',(-66.,-8.87355356113552,-6.08177373585213));
#44541=CARTESIAN_POINT('Ctrl Pts',(-50.,-8.87355356113552,-6.08177373585213));
#44542=CARTESIAN_POINT('Ctrl Pts',(-66.,-8.8323617893429,-5.97481445690694));
#44543=CARTESIAN_POINT('Ctrl Pts',(-50.,-8.8323617893429,-5.97481445690694));
#44544=CARTESIAN_POINT('Ctrl Pts',(-66.,-8.78938549860367,-5.86927258716782));
#44545=CARTESIAN_POINT('Ctrl Pts',(-50.,-8.78938549860367,-5.86927258716782));
#44546=CARTESIAN_POINT('Ctrl Pts',(-66.,-8.74461231231568,-5.76520918432743));
#44547=CARTESIAN_POINT('Ctrl Pts',(-50.,-8.74461231231568,-5.76520918432743));
#44548=CARTESIAN_POINT('Ctrl Pts',(-66.,-8.69803287743194,-5.66269130953282));
#44549=CARTESIAN_POINT('Ctrl Pts',(-50.,-8.69803287743194,-5.66269130953282));
#44550=CARTESIAN_POINT('Ctrl Pts',(-66.,-8.64964214626068,-5.56178799460163));
#44551=CARTESIAN_POINT('Ctrl Pts',(-50.,-8.64964214626068,-5.56178799460163));
#44552=CARTESIAN_POINT('Ctrl Pts',(-66.,-8.59944008163277,-5.46256677385502));
#44553=CARTESIAN_POINT('Ctrl Pts',(-50.,-8.59944008163277,-5.46256677385502));
#44554=CARTESIAN_POINT('Ctrl Pts',(-66.,-8.54743429835474,-5.36508801729631));
#44555=CARTESIAN_POINT('Ctrl Pts',(-50.,-8.54743429835474,-5.36508801729631));
#44556=CARTESIAN_POINT('Ctrl Pts',(-66.,-8.49363486229967,-5.26940895206487));
#44557=CARTESIAN_POINT('Ctrl Pts',(-50.,-8.49363486229967,-5.26940895206487));
#44558=CARTESIAN_POINT('Ctrl Pts',(-66.,-8.43804526716559,-5.17559278329922));
#44559=CARTESIAN_POINT('Ctrl Pts',(-50.,-8.43804526716559,-5.17559278329922));
#44560=CARTESIAN_POINT('Ctrl Pts',(-66.,-8.38065449559913,-5.08371585603889));
#44561=CARTESIAN_POINT('Ctrl Pts',(-50.,-8.38065449559913,-5.08371585603889));
#44562=CARTESIAN_POINT('Ctrl Pts',(-66.,-8.32142939657439,-4.99387589925328));
#44563=CARTESIAN_POINT('Ctrl Pts',(-50.,-8.32142939657439,-4.99387589925328));
#44564=CARTESIAN_POINT('Ctrl Pts',(-66.,-8.26030546894961,-4.90619864910471));
#44565=CARTESIAN_POINT('Ctrl Pts',(-50.,-8.26030546894961,-4.90619864910471));
#44566=CARTESIAN_POINT('Ctrl Pts',(-66.,-8.19718568217584,-4.82084919686819));
#44567=CARTESIAN_POINT('Ctrl Pts',(-50.,-8.19718568217584,-4.82084919686819));
#44568=CARTESIAN_POINT('Ctrl Pts',(-66.,-8.13194562956026,-4.73804414042434));
#44569=CARTESIAN_POINT('Ctrl Pts',(-50.,-8.13194562956026,-4.73804414042434));
#44570=CARTESIAN_POINT('Ctrl Pts',(-66.,-8.06443555863034,-4.65806703431538));
#44571=CARTESIAN_POINT('Ctrl Pts',(-50.,-8.06443555863034,-4.65806703431538));
#44572=CARTESIAN_POINT('Ctrl Pts',(-66.,-7.9944866564592,-4.58127474760048));
#44573=CARTESIAN_POINT('Ctrl Pts',(-50.,-7.9944866564592,-4.58127474760048));
#44574=CARTESIAN_POINT('Ctrl Pts',(-66.,-7.92190852612585,-4.50812719257416));
#44575=CARTESIAN_POINT('Ctrl Pts',(-50.,-7.92190852612585,-4.50812719257416));
#44576=CARTESIAN_POINT('Ctrl Pts',(-66.,-7.84652367297445,-4.43911683844659));
#44577=CARTESIAN_POINT('Ctrl Pts',(-50.,-7.84652367297445,-4.43911683844659));
#44578=CARTESIAN_POINT('Ctrl Pts',(-66.,-7.76822240772673,-4.37464133248276));
#44579=CARTESIAN_POINT('Ctrl Pts',(-50.,-7.76822240772673,-4.37464133248276));
#44580=CARTESIAN_POINT('Ctrl Pts',(-66.,-7.68701560500139,-4.31488559005748));
#44581=CARTESIAN_POINT('Ctrl Pts',(-50.,-7.68701560500139,-4.31488559005748));
#44582=CARTESIAN_POINT('Ctrl Pts',(-66.,-7.60308160854854,-4.25971402139557));
#44583=CARTESIAN_POINT('Ctrl Pts',(-50.,-7.60308160854854,-4.25971402139557));
#44584=CARTESIAN_POINT('Ctrl Pts',(-66.,-7.51683638885138,-4.2085165697132));
#44585=CARTESIAN_POINT('Ctrl Pts',(-50.,-7.51683638885138,-4.2085165697132));
#44586=CARTESIAN_POINT('Ctrl Pts',(-66.,-7.42887813111136,-4.16030958503735));
#44587=CARTESIAN_POINT('Ctrl Pts',(-50.,-7.42887813111136,-4.16030958503735));
#44588=CARTESIAN_POINT('Ctrl Pts',(-66.,-7.33988712400327,-4.11392789982873));
#44589=CARTESIAN_POINT('Ctrl Pts',(-50.,-7.33988712400327,-4.11392789982873));
#44590=CARTESIAN_POINT('Ctrl Pts',(-66.,-7.25053915877239,-4.06818897832557));
#44591=CARTESIAN_POINT('Ctrl Pts',(-50.,-7.25053915877239,-4.06818897832557));
#44592=CARTESIAN_POINT('Ctrl Pts',(-66.,-7.16141787020827,-4.02206007310117));
#44593=CARTESIAN_POINT('Ctrl Pts',(-50.,-7.16141787020827,-4.02206007310117));
#44594=CARTESIAN_POINT('Ctrl Pts',(-66.,-7.0729158360807,-3.97484570454348));
#44595=CARTESIAN_POINT('Ctrl Pts',(-50.,-7.0729158360807,-3.97484570454348));
#44596=CARTESIAN_POINT('Ctrl Pts',(-66.,-6.98526217067656,-3.92614017091869));
#44597=CARTESIAN_POINT('Ctrl Pts',(-50.,-6.98526217067656,-3.92614017091869));
#44598=CARTESIAN_POINT('Ctrl Pts',(-66.,-6.91590770916956,-3.88582374481706));
#44599=CARTESIAN_POINT('Ctrl Pts',(-50.,-6.91590770916956,-3.88582374481706));
#44600=CARTESIAN_POINT('Ctrl Pts',(-66.,-6.86433957558852,-3.8547985554459));
#44601=CARTESIAN_POINT('Ctrl Pts',(-50.,-6.86433957558852,-3.8547985554459));
#44602=CARTESIAN_POINT('Ctrl Pts',(-66.,-6.8301595578254,-3.83376536134756));
#44603=CARTESIAN_POINT('Ctrl Pts',(-50.,-6.8301595578254,-3.83376536134756));
#44604=CARTESIAN_POINT('Ctrl Pts',(-66.,-6.81311923233407,-3.82316133271924));
#44605=CARTESIAN_POINT('Ctrl Pts',(-50.,-6.81311923233407,-3.82316133271924));
#44606=CARTESIAN_POINT('Ctrl Pts',(-50.,-8.56527454818065,-5.39923114103194));
#44607=CARTESIAN_POINT('Ctrl Pts',(-50.,-8.56163853106842,-5.39247090060412));
#44608=CARTESIAN_POINT('Ctrl Pts',(-50.,-8.54750490102424,-5.3663130759002));
#44609=CARTESIAN_POINT('Ctrl Pts',(-50.,-8.52260030822016,-5.32102960234266));
#44610=CARTESIAN_POINT('Ctrl Pts',(-50.,-8.48638332772613,-5.25717084905799));
#44611=CARTESIAN_POINT('Ctrl Pts',(-50.,-8.43804526716559,-5.17559278329922));
#44612=CARTESIAN_POINT('Ctrl Pts',(-50.,-8.38065449559913,-5.08371585603889));
#44613=CARTESIAN_POINT('Ctrl Pts',(-50.,-8.32142939657439,-4.99387589925328));
#44614=CARTESIAN_POINT('Ctrl Pts',(-50.,-8.26030546894961,-4.90619864910471));
#44615=CARTESIAN_POINT('Ctrl Pts',(-50.,-8.19718568217584,-4.82084919686819));
#44616=CARTESIAN_POINT('Ctrl Pts',(-50.,-8.13194562956026,-4.73804414042434));
#44617=CARTESIAN_POINT('Ctrl Pts',(-50.,-8.06443555863034,-4.65806703431538));
#44618=CARTESIAN_POINT('Ctrl Pts',(-50.,-7.9944866564592,-4.58127474760048));
#44619=CARTESIAN_POINT('Ctrl Pts',(-50.,-7.92190852612585,-4.50812719257416));
#44620=CARTESIAN_POINT('Ctrl Pts',(-50.,-7.84652367297445,-4.43911683844659));
#44621=CARTESIAN_POINT('Ctrl Pts',(-50.,-7.76822240772673,-4.37464133248276));
#44622=CARTESIAN_POINT('Ctrl Pts',(-50.,-7.68701560500139,-4.31488559005748));
#44623=CARTESIAN_POINT('Ctrl Pts',(-50.,-7.60308160854854,-4.25971402139557));
#44624=CARTESIAN_POINT('Ctrl Pts',(-50.,-7.51683638885138,-4.2085165697132));
#44625=CARTESIAN_POINT('Ctrl Pts',(-50.,-7.42887813111136,-4.16030958503735));
#44626=CARTESIAN_POINT('Ctrl Pts',(-50.,-7.33988712400327,-4.11392789982873));
#44627=CARTESIAN_POINT('Ctrl Pts',(-50.,-7.25053915877239,-4.06818897832557));
#44628=CARTESIAN_POINT('Ctrl Pts',(-50.,-7.16141787020827,-4.02206007310117));
#44629=CARTESIAN_POINT('Ctrl Pts',(-50.,-7.0729158360807,-3.97484570454348));
#44630=CARTESIAN_POINT('Ctrl Pts',(-50.,-6.98526217067656,-3.92614017091869));
#44631=CARTESIAN_POINT('Ctrl Pts',(-50.,-6.91590770916956,-3.88582374481706));
#44632=CARTESIAN_POINT('Ctrl Pts',(-50.,-6.86433957558852,-3.8547985554459));
#44633=CARTESIAN_POINT('Ctrl Pts',(-50.,-6.8301595578254,-3.83376536134756));
#44634=CARTESIAN_POINT('Ctrl Pts',(-50.,-6.81311923233407,-3.82316133271924));
#44635=CARTESIAN_POINT('Origin',(-50.,-8.4736440577621,-4.30813108036277));
#44636=CARTESIAN_POINT('Origin',(-50.,0.,0.));
#44637=CARTESIAN_POINT('Origin',(-65.75,0.,0.));
#44638=CARTESIAN_POINT('',(-65.5,-10.4655009137276,-1.83409804120896));
#44639=CARTESIAN_POINT('Origin',(-65.5,0.,0.));
#44640=CARTESIAN_POINT('',(-66.,-10.0208328064459,-1.44863206690261));
#44641=CARTESIAN_POINT('Ctrl Pts',(-65.5,-10.4655009137276,-1.83409804120895));
#44642=CARTESIAN_POINT('Ctrl Pts',(-65.6641206711811,-10.3229569256148,
-1.69670740679554));
#44643=CARTESIAN_POINT('Ctrl Pts',(-65.8307448212024,-10.1746455742797,
-1.56762477685534));
#44644=CARTESIAN_POINT('Ctrl Pts',(-66.,-10.0208328064459,-1.44863206690261));
#44645=CARTESIAN_POINT('Origin',(-66.,0.,0.));
#44646=CARTESIAN_POINT('Origin',(-58.,0.,0.));
#44647=CARTESIAN_POINT('',(-50.5,-10.4655009137276,-1.83409804120895));
#44648=CARTESIAN_POINT('Origin',(-50.5,0.,0.));
#44649=CARTESIAN_POINT('Ctrl Pts',(-50.5,-10.4655009137276,-1.83409804120896));
#44650=CARTESIAN_POINT('Ctrl Pts',(-55.5,-10.4655009137276,-1.83409804120896));
#44651=CARTESIAN_POINT('Ctrl Pts',(-60.5,-10.4655009137276,-1.83409804120895));
#44652=CARTESIAN_POINT('Ctrl Pts',(-65.5,-10.4655009137276,-1.83409804120895));
#44653=CARTESIAN_POINT('Origin',(-50.25,0.,0.));
#44654=CARTESIAN_POINT('',(-50.,-10.0208328064459,-1.44863206690262));
#44655=CARTESIAN_POINT('Origin',(-50.,0.,0.));
#44656=CARTESIAN_POINT('Ctrl Pts',(-50.,-10.0208328064459,-1.44863206690262));
#44657=CARTESIAN_POINT('Ctrl Pts',(-50.1692551787974,-10.1746455742796,
-1.56762477685526));
#44658=CARTESIAN_POINT('Ctrl Pts',(-50.3358793288183,-10.3229569256143,
-1.69670740679502));
#44659=CARTESIAN_POINT('Ctrl Pts',(-50.5,-10.4655009137276,-1.83409804120896));
#44660=CARTESIAN_POINT('Origin',(-66.,-9.49333381220606,-0.489132040720954));
#44661=CARTESIAN_POINT('',(-66.,-10.0227511096935,1.43529968756956));
#44662=CARTESIAN_POINT('',(-66.,-10.125,-1.23995488413669E-15));
#44663=CARTESIAN_POINT('Origin',(-66.,0.,0.));
#44664=CARTESIAN_POINT('Origin',(-66.,0.,0.));
#44665=CARTESIAN_POINT('',(-66.,-7.77911393348366,-0.72148642390575));
#44666=CARTESIAN_POINT('Ctrl Pts',(-66.,-7.77911393348366,-0.721486423905757));
#44667=CARTESIAN_POINT('Ctrl Pts',(-66.,-7.79899409244038,-0.724242761304609));
#44668=CARTESIAN_POINT('Ctrl Pts',(-66.,-7.83877406317074,-0.72955527454762));
#44669=CARTESIAN_POINT('Ctrl Pts',(-66.,-7.89850297873842,-0.736923545827707));
#44670=CARTESIAN_POINT('Ctrl Pts',(-66.,-7.97825959982878,-0.745545432905555));
#44671=CARTESIAN_POINT('Ctrl Pts',(-66.,-8.07814553295023,-0.75438819429077));
#44672=CARTESIAN_POINT('Ctrl Pts',(-66.,-8.17819997799169,-0.761523645955682));
#44673=CARTESIAN_POINT('Ctrl Pts',(-66.,-8.27837864239844,-0.767415604052299));
#44674=CARTESIAN_POINT('Ctrl Pts',(-66.,-8.37860576557482,-0.772859096585322));
#44675=CARTESIAN_POINT('Ctrl Pts',(-66.,-8.4787682268314,-0.77903497093039));
#44676=CARTESIAN_POINT('Ctrl Pts',(-66.,-8.57872964077182,-0.787298396323681));
#44677=CARTESIAN_POINT('Ctrl Pts',(-66.,-8.67834244910087,-0.798990504610031));
#44678=CARTESIAN_POINT('Ctrl Pts',(-66.,-8.77746026893294,-0.81525320859497));
#44679=CARTESIAN_POINT('Ctrl Pts',(-66.,-8.8759512247709,-0.836813013320223));
#44680=CARTESIAN_POINT('Ctrl Pts',(-66.,-8.97370754082197,-0.86386632514724));
#44681=CARTESIAN_POINT('Ctrl Pts',(-66.,-9.07064407076881,-0.896248638581227));
#44682=CARTESIAN_POINT('Ctrl Pts',(-66.,-9.16669928303964,-0.933552070120681));
#44683=CARTESIAN_POINT('Ctrl Pts',(-66.,-9.2618350217977,-0.975254533175137));
#44684=CARTESIAN_POINT('Ctrl Pts',(-66.,-9.35603816010254,-1.02085843555253));
#44685=CARTESIAN_POINT('Ctrl Pts',(-66.,-9.44931776451354,-1.0699690987417));
#44686=CARTESIAN_POINT('Ctrl Pts',(-66.,-9.54169530869912,-1.12226657296063));
#44687=CARTESIAN_POINT('Ctrl Pts',(-66.,-9.63319634553357,-1.17750238543874));
#44688=CARTESIAN_POINT('Ctrl Pts',(-66.,-9.7238423681631,-1.23548625191189));
#44689=CARTESIAN_POINT('Ctrl Pts',(-66.,-9.81364115980824,-1.29607707170225));
#44690=CARTESIAN_POINT('Ctrl Pts',(-66.,-9.8909809640799,-1.35094148263425));
#44691=CARTESIAN_POINT('Ctrl Pts',(-66.,-9.95004051704176,-1.3945485835597));
#44692=CARTESIAN_POINT('Ctrl Pts',(-66.,-9.99121044269398,-1.42578748466016));
#44693=CARTESIAN_POINT('Ctrl Pts',(-66.,-10.0147615020311,-1.44393518136159));
#44694=CARTESIAN_POINT('Ctrl Pts',(-66.,-10.0208328064459,-1.44863206690261));
#44695=CARTESIAN_POINT('',(-66.,-7.77911393348366,0.721486423905763));
#44696=CARTESIAN_POINT('Origin',(-66.,0.,0.));
#44697=CARTESIAN_POINT('Ctrl Pts',(-66.,-10.0227511096935,1.43529968756956));
#44698=CARTESIAN_POINT('Ctrl Pts',(-66.,-10.0075805937231,1.42243692144955));
#44699=CARTESIAN_POINT('Ctrl Pts',(-66.,-9.97157110660129,1.39292748043395));
#44700=CARTESIAN_POINT('Ctrl Pts',(-66.,-9.91468044888801,1.35006780516087));
#44701=CARTESIAN_POINT('Ctrl Pts',(-66.,-9.83676426393002,1.29854345762933));
#44702=CARTESIAN_POINT('Ctrl Pts',(-66.,-9.73724351312182,1.24043599038436));
#44703=CARTESIAN_POINT('Ctrl Pts',(-66.,-9.6306368085439,1.18054610024187));
#44704=CARTESIAN_POINT('Ctrl Pts',(-66.,-9.5223457393261,1.11893544879958));
#44705=CARTESIAN_POINT('Ctrl Pts',(-66.,-9.41237093241568,1.05638393958167));
#44706=CARTESIAN_POINT('Ctrl Pts',(-66.,-9.30087338143967,0.995690646749764));
#44707=CARTESIAN_POINT('Ctrl Pts',(-66.,-9.18808826379209,0.940486683861864));
#44708=CARTESIAN_POINT('Ctrl Pts',(-66.,-9.07419455050615,0.893519132818963));
#44709=CARTESIAN_POINT('Ctrl Pts',(-66.,-8.9592587823094,0.855777148432806));
#44710=CARTESIAN_POINT('Ctrl Pts',(-66.,-8.84331035406979,0.8270560355778));
#44711=CARTESIAN_POINT('Ctrl Pts',(-66.,-8.72638717702053,0.80622268656513));
#44712=CARTESIAN_POINT('Ctrl Pts',(-66.,-8.60859985083163,0.791601524257944));
#44713=CARTESIAN_POINT('Ctrl Pts',(-66.,-8.49016832489629,0.781278580568713));
#44714=CARTESIAN_POINT('Ctrl Pts',(-66.,-8.37136168323973,0.773305799751092));
#44715=CARTESIAN_POINT('Ctrl Pts',(-66.,-8.25245284713798,0.765907999193168));
#44716=CARTESIAN_POINT('Ctrl Pts',(-66.,-8.13366539810525,0.757700310523095));
#44717=CARTESIAN_POINT('Ctrl Pts',(-66.,-8.01512993231441,0.747872039941245));
#44718=CARTESIAN_POINT('Ctrl Pts',(-66.,-7.92055498607902,0.738391761574612));
#44719=CARTESIAN_POINT('Ctrl Pts',(-66.,-7.84977551686152,0.730314664611583));
#44720=CARTESIAN_POINT('Ctrl Pts',(-66.,-7.80265656782328,0.724500705979671));
#44721=CARTESIAN_POINT('Ctrl Pts',(-66.,-7.77911393348366,0.721486423905763));
#44722=CARTESIAN_POINT('Ctrl Pts',(-66.,-7.77911393348366,0.721486423905763));
#44723=CARTESIAN_POINT('Ctrl Pts',(-50.,-7.77911393348366,0.721486423905763));
#44724=CARTESIAN_POINT('Ctrl Pts',(-66.,-7.80265656782328,0.724500705979671));
#44725=CARTESIAN_POINT('Ctrl Pts',(-50.,-7.80265656782328,0.724500705979671));
#44726=CARTESIAN_POINT('Ctrl Pts',(-66.,-7.84977551686152,0.730314664611583));
#44727=CARTESIAN_POINT('Ctrl Pts',(-50.,-7.84977551686152,0.730314664611583));
#44728=CARTESIAN_POINT('Ctrl Pts',(-66.,-7.92055498607902,0.738391761574612));
#44729=CARTESIAN_POINT('Ctrl Pts',(-50.,-7.92055498607902,0.738391761574612));
#44730=CARTESIAN_POINT('Ctrl Pts',(-66.,-8.01512993231441,0.747872039941245));
#44731=CARTESIAN_POINT('Ctrl Pts',(-50.,-8.01512993231441,0.747872039941245));
#44732=CARTESIAN_POINT('Ctrl Pts',(-66.,-8.13366539810525,0.757700310523095));
#44733=CARTESIAN_POINT('Ctrl Pts',(-50.,-8.13366539810525,0.757700310523095));
#44734=CARTESIAN_POINT('Ctrl Pts',(-66.,-8.25245284713798,0.765907999193168));
#44735=CARTESIAN_POINT('Ctrl Pts',(-50.,-8.25245284713798,0.765907999193168));
#44736=CARTESIAN_POINT('Ctrl Pts',(-66.,-8.37136168323973,0.773305799751092));
#44737=CARTESIAN_POINT('Ctrl Pts',(-50.,-8.37136168323973,0.773305799751092));
#44738=CARTESIAN_POINT('Ctrl Pts',(-66.,-8.49016832489629,0.781278580568713));
#44739=CARTESIAN_POINT('Ctrl Pts',(-50.,-8.49016832489629,0.781278580568713));
#44740=CARTESIAN_POINT('Ctrl Pts',(-66.,-8.60859985083163,0.791601524257944));
#44741=CARTESIAN_POINT('Ctrl Pts',(-50.,-8.60859985083163,0.791601524257944));
#44742=CARTESIAN_POINT('Ctrl Pts',(-66.,-8.72638717702053,0.80622268656513));
#44743=CARTESIAN_POINT('Ctrl Pts',(-50.,-8.72638717702053,0.80622268656513));
#44744=CARTESIAN_POINT('Ctrl Pts',(-66.,-8.84331035406979,0.8270560355778));
#44745=CARTESIAN_POINT('Ctrl Pts',(-50.,-8.84331035406979,0.8270560355778));
#44746=CARTESIAN_POINT('Ctrl Pts',(-66.,-8.9592587823094,0.855777148432806));
#44747=CARTESIAN_POINT('Ctrl Pts',(-50.,-8.9592587823094,0.855777148432806));
#44748=CARTESIAN_POINT('Ctrl Pts',(-66.,-9.07419455050615,0.893519132818963));
#44749=CARTESIAN_POINT('Ctrl Pts',(-50.,-9.07419455050615,0.893519132818963));
#44750=CARTESIAN_POINT('Ctrl Pts',(-66.,-9.18808826379209,0.940486683861864));
#44751=CARTESIAN_POINT('Ctrl Pts',(-50.,-9.18808826379209,0.940486683861864));
#44752=CARTESIAN_POINT('Ctrl Pts',(-66.,-9.30087338143967,0.995690646749764));
#44753=CARTESIAN_POINT('Ctrl Pts',(-50.,-9.30087338143967,0.995690646749764));
#44754=CARTESIAN_POINT('Ctrl Pts',(-66.,-9.41237093241568,1.05638393958167));
#44755=CARTESIAN_POINT('Ctrl Pts',(-50.,-9.41237093241568,1.05638393958167));
#44756=CARTESIAN_POINT('Ctrl Pts',(-66.,-9.5223457393261,1.11893544879958));
#44757=CARTESIAN_POINT('Ctrl Pts',(-50.,-9.5223457393261,1.11893544879958));
#44758=CARTESIAN_POINT('Ctrl Pts',(-66.,-9.6306368085439,1.18054610024187));
#44759=CARTESIAN_POINT('Ctrl Pts',(-50.,-9.6306368085439,1.18054610024187));
#44760=CARTESIAN_POINT('Ctrl Pts',(-66.,-9.73724351312182,1.24043599038436));
#44761=CARTESIAN_POINT('Ctrl Pts',(-50.,-9.73724351312182,1.24043599038436));
#44762=CARTESIAN_POINT('Ctrl Pts',(-66.,-9.84248083742894,1.30188120985331));
#44763=CARTESIAN_POINT('Ctrl Pts',(-50.,-9.84248083742894,1.30188120985331));
#44764=CARTESIAN_POINT('Ctrl Pts',(-66.,-9.94691663163917,1.37153583848331));
#44765=CARTESIAN_POINT('Ctrl Pts',(-50.,-9.94691663163917,1.37153583848331));
#44766=CARTESIAN_POINT('Ctrl Pts',(-66.,-10.0510556136356,1.45560107784126));
#44767=CARTESIAN_POINT('Ctrl Pts',(-50.,-10.0510556136356,1.45560107784126));
#44768=CARTESIAN_POINT('Ctrl Pts',(-66.,-10.1551049870319,1.5570004387935));
#44769=CARTESIAN_POINT('Ctrl Pts',(-50.,-10.1551049870319,1.5570004387935));
#44770=CARTESIAN_POINT('Ctrl Pts',(-66.,-10.2586709822228,1.67172133360717));
#44771=CARTESIAN_POINT('Ctrl Pts',(-50.,-10.2586709822228,1.67172133360717));
#44772=CARTESIAN_POINT('Ctrl Pts',(-66.,-10.3605863148615,1.78670918299558));
#44773=CARTESIAN_POINT('Ctrl Pts',(-50.,-10.3605863148615,1.78670918299558));
#44774=CARTESIAN_POINT('Ctrl Pts',(-66.,-10.4592314889185,1.88359108652926));
#44775=CARTESIAN_POINT('Ctrl Pts',(-50.,-10.4592314889185,1.88359108652926));
#44776=CARTESIAN_POINT('Ctrl Pts',(-66.,-10.5527881700323,1.94159504365348));
#44777=CARTESIAN_POINT('Ctrl Pts',(-50.,-10.5527881700323,1.94159504365348));
#44778=CARTESIAN_POINT('Ctrl Pts',(-66.,-10.6395078008537,1.94065117489419));
#44779=CARTESIAN_POINT('Ctrl Pts',(-50.,-10.6395078008537,1.94065117489419));
#44780=CARTESIAN_POINT('Ctrl Pts',(-66.,-10.7180003851451,1.86471753735723));
#44781=CARTESIAN_POINT('Ctrl Pts',(-50.,-10.7180003851451,1.86471753735723));
#44782=CARTESIAN_POINT('Ctrl Pts',(-66.,-10.78721780482,1.70161126501303));
#44783=CARTESIAN_POINT('Ctrl Pts',(-50.,-10.78721780482,1.70161126501303));
#44784=CARTESIAN_POINT('Ctrl Pts',(-66.,-10.8463940896281,1.44234467706895));
#44785=CARTESIAN_POINT('Ctrl Pts',(-50.,-10.8463940896281,1.44234467706895));
#44786=CARTESIAN_POINT('Ctrl Pts',(-66.,-10.8950036886707,1.08066595121422));
#44787=CARTESIAN_POINT('Ctrl Pts',(-50.,-10.8950036886707,1.08066595121422));
#44788=CARTESIAN_POINT('Ctrl Pts',(-66.,-10.9327147397562,0.612540812857));
#44789=CARTESIAN_POINT('Ctrl Pts',(-50.,-10.9327147397562,0.612540812857));
#44790=CARTESIAN_POINT('Ctrl Pts',(-66.,-10.9593469088286,0.0356850348521551));
#44791=CARTESIAN_POINT('Ctrl Pts',(-50.,-10.9593469088286,0.0356850348521551));
#44792=CARTESIAN_POINT('Ctrl Pts',(-66.,-10.9748294814774,-0.650901657883903));
#44793=CARTESIAN_POINT('Ctrl Pts',(-50.,-10.9748294814774,-0.650901657883903));
#44794=CARTESIAN_POINT('Ctrl Pts',(-66.,-10.9782949820983,-1.28808536247603));
#44795=CARTESIAN_POINT('Ctrl Pts',(-50.,-10.9782949820983,-1.28808536247603));
#44796=CARTESIAN_POINT('Ctrl Pts',(-66.,-10.9758895571813,-1.81531684557756));
#44797=CARTESIAN_POINT('Ctrl Pts',(-50.,-10.9758895571813,-1.81531684557756));
#44798=CARTESIAN_POINT('Ctrl Pts',(-66.,-10.9720646526695,-2.18870588261173));
#44799=CARTESIAN_POINT('Ctrl Pts',(-50.,-10.9720646526695,-2.18870588261173));
#44800=CARTESIAN_POINT('Ctrl Pts',(-66.,-10.9695968782856,-2.3808757481032));
#44801=CARTESIAN_POINT('Ctrl Pts',(-50.,-10.9695968782856,-2.3808757481032));
#44802=CARTESIAN_POINT('',(-65.5,-10.4583906644234,1.87421709262873));
#44803=CARTESIAN_POINT('Ctrl Pts',(-66.,-10.0227511096935,1.43529968756956));
#44804=CARTESIAN_POINT('Ctrl Pts',(-65.8225584213011,-10.1825947061167,
1.57082776061481));
#44805=CARTESIAN_POINT('Ctrl Pts',(-65.6845963763178,-10.2971553372475,
1.72560541037367));
#44806=CARTESIAN_POINT('Ctrl Pts',(-65.5373483115606,-10.4253681088298,
1.84668138012166));
#44807=CARTESIAN_POINT('Ctrl Pts',(-65.518392043377,-10.4420170465692,1.86131903035675));
#44808=CARTESIAN_POINT('Ctrl Pts',(-65.5,-10.4583906644234,1.87421709262873));
#44809=CARTESIAN_POINT('',(-50.,-7.77911393348366,0.721486423905763));
#44810=CARTESIAN_POINT('',(-66.,-7.77911393348366,0.721486423905763));
#44811=CARTESIAN_POINT('',(-50.,-10.0227511096935,1.43529968756957));
#44812=CARTESIAN_POINT('Ctrl Pts',(-50.,-7.77911393348366,0.721486423905763));
#44813=CARTESIAN_POINT('Ctrl Pts',(-50.,-7.80265656782328,0.724500705979671));
#44814=CARTESIAN_POINT('Ctrl Pts',(-50.,-7.84977551686152,0.730314664611583));
#44815=CARTESIAN_POINT('Ctrl Pts',(-50.,-7.92055498607902,0.738391761574612));
#44816=CARTESIAN_POINT('Ctrl Pts',(-50.,-8.01512993231441,0.747872039941245));
#44817=CARTESIAN_POINT('Ctrl Pts',(-50.,-8.13366539810525,0.757700310523095));
#44818=CARTESIAN_POINT('Ctrl Pts',(-50.,-8.25245284713798,0.765907999193168));
#44819=CARTESIAN_POINT('Ctrl Pts',(-50.,-8.37136168323973,0.773305799751092));
#44820=CARTESIAN_POINT('Ctrl Pts',(-50.,-8.49016832489629,0.781278580568713));
#44821=CARTESIAN_POINT('Ctrl Pts',(-50.,-8.60859985083163,0.791601524257944));
#44822=CARTESIAN_POINT('Ctrl Pts',(-50.,-8.72638717702053,0.80622268656513));
#44823=CARTESIAN_POINT('Ctrl Pts',(-50.,-8.84331035406979,0.8270560355778));
#44824=CARTESIAN_POINT('Ctrl Pts',(-50.,-8.9592587823094,0.855777148432806));
#44825=CARTESIAN_POINT('Ctrl Pts',(-50.,-9.07419455050615,0.893519132818963));
#44826=CARTESIAN_POINT('Ctrl Pts',(-50.,-9.18808826379209,0.940486683861864));
#44827=CARTESIAN_POINT('Ctrl Pts',(-50.,-9.30087338143967,0.995690646749764));
#44828=CARTESIAN_POINT('Ctrl Pts',(-50.,-9.41237093241568,1.05638393958167));
#44829=CARTESIAN_POINT('Ctrl Pts',(-50.,-9.5223457393261,1.11893544879958));
#44830=CARTESIAN_POINT('Ctrl Pts',(-50.,-9.6306368085439,1.18054610024187));
#44831=CARTESIAN_POINT('Ctrl Pts',(-50.,-9.73724351312182,1.24043599038436));
#44832=CARTESIAN_POINT('Ctrl Pts',(-50.,-9.83676426393003,1.29854345762933));
#44833=CARTESIAN_POINT('Ctrl Pts',(-50.,-9.91468044888801,1.35006780516087));
#44834=CARTESIAN_POINT('Ctrl Pts',(-50.,-9.9715711066013,1.39292748043396));
#44835=CARTESIAN_POINT('Ctrl Pts',(-50.,-10.0075805937231,1.42243692144956));
#44836=CARTESIAN_POINT('Ctrl Pts',(-50.,-10.0227511096935,1.43529968756957));
#44837=CARTESIAN_POINT('',(-50.5,-10.4583906644234,1.87421709262873));
#44838=CARTESIAN_POINT('Ctrl Pts',(-50.5,-10.4583906644234,1.87421709262874));
#44839=CARTESIAN_POINT('Ctrl Pts',(-50.4735369152344,-10.4348317575466,
1.85565893091618));
#44840=CARTESIAN_POINT('Ctrl Pts',(-50.4463054701399,-10.4110560430942,
1.83378829126636));
#44841=CARTESIAN_POINT('Ctrl Pts',(-50.2958361627283,-10.280846856736,1.70451692542734));
#44842=CARTESIAN_POINT('Ctrl Pts',(-50.1659505682738,-10.1722433304901,
1.5620510437276));
#44843=CARTESIAN_POINT('Ctrl Pts',(-50.,-10.0227511096935,1.43529968756958));
#44844=CARTESIAN_POINT('Ctrl Pts',(-65.5,-10.4583906644234,1.87421709262873));
#44845=CARTESIAN_POINT('Ctrl Pts',(-60.5,-10.4583906644234,1.87421709262873));
#44846=CARTESIAN_POINT('Ctrl Pts',(-55.5,-10.4583906644234,1.87421709262873));
#44847=CARTESIAN_POINT('Ctrl Pts',(-50.5,-10.4583906644234,1.87421709262873));
#44848=CARTESIAN_POINT('Origin',(-66.,0.,0.));
#44849=CARTESIAN_POINT('',(-50.,-7.77911393348366,-0.72148642390575));
#44850=CARTESIAN_POINT('',(-66.,-7.77911393348366,-0.72148642390575));
#44851=CARTESIAN_POINT('Origin',(-50.,0.,0.));
#44852=CARTESIAN_POINT('Ctrl Pts',(-66.,-10.9695968782856,-2.3808757481032));
#44853=CARTESIAN_POINT('Ctrl Pts',(-50.,-10.9695968782856,-2.3808757481032));
#44854=CARTESIAN_POINT('Ctrl Pts',(-66.,-10.9545320670164,-2.36259298774431));
#44855=CARTESIAN_POINT('Ctrl Pts',(-50.,-10.9545320670164,-2.36259298774431));
#44856=CARTESIAN_POINT('Ctrl Pts',(-66.,-10.924297577215,-2.32621343870963));
#44857=CARTESIAN_POINT('Ctrl Pts',(-50.,-10.924297577215,-2.32621343870963));
#44858=CARTESIAN_POINT('Ctrl Pts',(-66.,-10.8786312409555,-2.27220203031823));
#44859=CARTESIAN_POINT('Ctrl Pts',(-50.,-10.8786312409555,-2.27220203031823));
#44860=CARTESIAN_POINT('Ctrl Pts',(-66.,-10.8171127507393,-2.20130413232088));
#44861=CARTESIAN_POINT('Ctrl Pts',(-50.,-10.8171127507393,-2.20130413232088));
#44862=CARTESIAN_POINT('Ctrl Pts',(-66.,-10.7391601959231,-2.1145560232782));
#44863=CARTESIAN_POINT('Ctrl Pts',(-50.,-10.7391601959231,-2.1145560232782));
#44864=CARTESIAN_POINT('Ctrl Pts',(-66.,-10.6601485052333,-2.0297033976563));
#44865=CARTESIAN_POINT('Ctrl Pts',(-50.,-10.6601485052333,-2.0297033976563));
#44866=CARTESIAN_POINT('Ctrl Pts',(-66.,-10.5800747821907,-1.94677738318821));
#44867=CARTESIAN_POINT('Ctrl Pts',(-50.,-10.5800747821907,-1.94677738318821));
#44868=CARTESIAN_POINT('Ctrl Pts',(-66.,-10.4989399681134,-1.86581942273637));
#44869=CARTESIAN_POINT('Ctrl Pts',(-50.,-10.4989399681134,-1.86581942273637));
#44870=CARTESIAN_POINT('Ctrl Pts',(-66.,-10.4167514271206,-1.78688215927222));
#44871=CARTESIAN_POINT('Ctrl Pts',(-50.,-10.4167514271206,-1.78688215927222));
#44872=CARTESIAN_POINT('Ctrl Pts',(-66.,-10.3335226870247,-1.71002640579114));
#44873=CARTESIAN_POINT('Ctrl Pts',(-50.,-10.3335226870247,-1.71002640579114));
#44874=CARTESIAN_POINT('Ctrl Pts',(-66.,-10.2492724796178,-1.63531722992632));
#44875=CARTESIAN_POINT('Ctrl Pts',(-50.,-10.2492724796178,-1.63531722992632));
#44876=CARTESIAN_POINT('Ctrl Pts',(-66.,-10.164024271374,-1.56281974846243));
#44877=CARTESIAN_POINT('Ctrl Pts',(-50.,-10.164024271374,-1.56281974846243));
#44878=CARTESIAN_POINT('Ctrl Pts',(-66.,-10.0778054970205,-1.49259567218985));
#44879=CARTESIAN_POINT('Ctrl Pts',(-50.,-10.0778054970205,-1.49259567218985));
#44880=CARTESIAN_POINT('Ctrl Pts',(-66.,-9.99064766772184,-1.42469705463002));
#44881=CARTESIAN_POINT('Ctrl Pts',(-50.,-9.99064766772184,-1.42469705463002));
#44882=CARTESIAN_POINT('Ctrl Pts',(-66.,-9.90258325548514,-1.35917208121676));
#44883=CARTESIAN_POINT('Ctrl Pts',(-50.,-9.90258325548514,-1.35917208121676));
#44884=CARTESIAN_POINT('Ctrl Pts',(-66.,-9.81364115980824,-1.29607707170225));
#44885=CARTESIAN_POINT('Ctrl Pts',(-50.,-9.81364115980824,-1.29607707170225));
#44886=CARTESIAN_POINT('Ctrl Pts',(-66.,-9.7238423681631,-1.23548625191189));
#44887=CARTESIAN_POINT('Ctrl Pts',(-50.,-9.7238423681631,-1.23548625191189));
#44888=CARTESIAN_POINT('Ctrl Pts',(-66.,-9.63319634553357,-1.17750238543874));
#44889=CARTESIAN_POINT('Ctrl Pts',(-50.,-9.63319634553357,-1.17750238543874));
#44890=CARTESIAN_POINT('Ctrl Pts',(-66.,-9.54169530869912,-1.12226657296063));
#44891=CARTESIAN_POINT('Ctrl Pts',(-50.,-9.54169530869912,-1.12226657296063));
#44892=CARTESIAN_POINT('Ctrl Pts',(-66.,-9.44931776451354,-1.0699690987417));
#44893=CARTESIAN_POINT('Ctrl Pts',(-50.,-9.44931776451354,-1.0699690987417));
#44894=CARTESIAN_POINT('Ctrl Pts',(-66.,-9.35603816010254,-1.02085843555253));
#44895=CARTESIAN_POINT('Ctrl Pts',(-50.,-9.35603816010254,-1.02085843555253));
#44896=CARTESIAN_POINT('Ctrl Pts',(-66.,-9.2618350217977,-0.975254533175137));
#44897=CARTESIAN_POINT('Ctrl Pts',(-50.,-9.2618350217977,-0.975254533175137));
#44898=CARTESIAN_POINT('Ctrl Pts',(-66.,-9.16669928303964,-0.933552070120681));
#44899=CARTESIAN_POINT('Ctrl Pts',(-50.,-9.16669928303964,-0.933552070120681));
#44900=CARTESIAN_POINT('Ctrl Pts',(-66.,-9.07064407076881,-0.896248638581227));
#44901=CARTESIAN_POINT('Ctrl Pts',(-50.,-9.07064407076881,-0.896248638581227));
#44902=CARTESIAN_POINT('Ctrl Pts',(-66.,-8.97370754082197,-0.86386632514724));
#44903=CARTESIAN_POINT('Ctrl Pts',(-50.,-8.97370754082197,-0.86386632514724));
#44904=CARTESIAN_POINT('Ctrl Pts',(-66.,-8.8759512247709,-0.836813013320223));
#44905=CARTESIAN_POINT('Ctrl Pts',(-50.,-8.8759512247709,-0.836813013320223));
#44906=CARTESIAN_POINT('Ctrl Pts',(-66.,-8.77746026893294,-0.81525320859497));
#44907=CARTESIAN_POINT('Ctrl Pts',(-50.,-8.77746026893294,-0.81525320859497));
#44908=CARTESIAN_POINT('Ctrl Pts',(-66.,-8.67834244910087,-0.798990504610031));
#44909=CARTESIAN_POINT('Ctrl Pts',(-50.,-8.67834244910087,-0.798990504610031));
#44910=CARTESIAN_POINT('Ctrl Pts',(-66.,-8.57872964077182,-0.787298396323681));
#44911=CARTESIAN_POINT('Ctrl Pts',(-50.,-8.57872964077182,-0.787298396323681));
#44912=CARTESIAN_POINT('Ctrl Pts',(-66.,-8.4787682268314,-0.77903497093039));
#44913=CARTESIAN_POINT('Ctrl Pts',(-50.,-8.4787682268314,-0.77903497093039));
#44914=CARTESIAN_POINT('Ctrl Pts',(-66.,-8.37860576557482,-0.772859096585322));
#44915=CARTESIAN_POINT('Ctrl Pts',(-50.,-8.37860576557482,-0.772859096585322));
#44916=CARTESIAN_POINT('Ctrl Pts',(-66.,-8.27837864239844,-0.767415604052299));
#44917=CARTESIAN_POINT('Ctrl Pts',(-50.,-8.27837864239844,-0.767415604052299));
#44918=CARTESIAN_POINT('Ctrl Pts',(-66.,-8.17819997799169,-0.761523645955682));
#44919=CARTESIAN_POINT('Ctrl Pts',(-50.,-8.17819997799169,-0.761523645955682));
#44920=CARTESIAN_POINT('Ctrl Pts',(-66.,-8.07814553295023,-0.75438819429077));
#44921=CARTESIAN_POINT('Ctrl Pts',(-50.,-8.07814553295023,-0.75438819429077));
#44922=CARTESIAN_POINT('Ctrl Pts',(-66.,-7.97825959982878,-0.745545432905555));
#44923=CARTESIAN_POINT('Ctrl Pts',(-50.,-7.97825959982878,-0.745545432905555));
#44924=CARTESIAN_POINT('Ctrl Pts',(-66.,-7.89850297873842,-0.736923545827707));
#44925=CARTESIAN_POINT('Ctrl Pts',(-50.,-7.89850297873842,-0.736923545827707));
#44926=CARTESIAN_POINT('Ctrl Pts',(-66.,-7.83877406317074,-0.72955527454762));
#44927=CARTESIAN_POINT('Ctrl Pts',(-50.,-7.83877406317074,-0.72955527454762));
#44928=CARTESIAN_POINT('Ctrl Pts',(-66.,-7.79899409244038,-0.724242761304609));
#44929=CARTESIAN_POINT('Ctrl Pts',(-50.,-7.79899409244038,-0.724242761304609));
#44930=CARTESIAN_POINT('Ctrl Pts',(-66.,-7.77911393348366,-0.721486423905757));
#44931=CARTESIAN_POINT('Ctrl Pts',(-50.,-7.77911393348366,-0.721486423905757));
#44932=CARTESIAN_POINT('Ctrl Pts',(-50.,-10.0208328064459,-1.44863206690262));
#44933=CARTESIAN_POINT('Ctrl Pts',(-50.,-10.0147615020311,-1.4439351813616));
#44934=CARTESIAN_POINT('Ctrl Pts',(-50.,-9.99121044269398,-1.42578748466017));
#44935=CARTESIAN_POINT('Ctrl Pts',(-50.,-9.95004051704177,-1.39454858355971));
#44936=CARTESIAN_POINT('Ctrl Pts',(-50.,-9.8909809640799,-1.35094148263425));
#44937=CARTESIAN_POINT('Ctrl Pts',(-50.,-9.81364115980824,-1.29607707170225));
#44938=CARTESIAN_POINT('Ctrl Pts',(-50.,-9.7238423681631,-1.23548625191189));
#44939=CARTESIAN_POINT('Ctrl Pts',(-50.,-9.63319634553357,-1.17750238543874));
#44940=CARTESIAN_POINT('Ctrl Pts',(-50.,-9.54169530869912,-1.12226657296063));
#44941=CARTESIAN_POINT('Ctrl Pts',(-50.,-9.44931776451354,-1.0699690987417));
#44942=CARTESIAN_POINT('Ctrl Pts',(-50.,-9.35603816010254,-1.02085843555253));
#44943=CARTESIAN_POINT('Ctrl Pts',(-50.,-9.2618350217977,-0.975254533175137));
#44944=CARTESIAN_POINT('Ctrl Pts',(-50.,-9.16669928303964,-0.933552070120681));
#44945=CARTESIAN_POINT('Ctrl Pts',(-50.,-9.07064407076881,-0.896248638581227));
#44946=CARTESIAN_POINT('Ctrl Pts',(-50.,-8.97370754082197,-0.86386632514724));
#44947=CARTESIAN_POINT('Ctrl Pts',(-50.,-8.8759512247709,-0.836813013320223));
#44948=CARTESIAN_POINT('Ctrl Pts',(-50.,-8.77746026893294,-0.81525320859497));
#44949=CARTESIAN_POINT('Ctrl Pts',(-50.,-8.67834244910087,-0.798990504610031));
#44950=CARTESIAN_POINT('Ctrl Pts',(-50.,-8.57872964077182,-0.787298396323681));
#44951=CARTESIAN_POINT('Ctrl Pts',(-50.,-8.4787682268314,-0.77903497093039));
#44952=CARTESIAN_POINT('Ctrl Pts',(-50.,-8.37860576557482,-0.772859096585322));
#44953=CARTESIAN_POINT('Ctrl Pts',(-50.,-8.27837864239844,-0.767415604052299));
#44954=CARTESIAN_POINT('Ctrl Pts',(-50.,-8.17819997799169,-0.761523645955682));
#44955=CARTESIAN_POINT('Ctrl Pts',(-50.,-8.07814553295023,-0.75438819429077));
#44956=CARTESIAN_POINT('Ctrl Pts',(-50.,-7.97825959982878,-0.745545432905555));
#44957=CARTESIAN_POINT('Ctrl Pts',(-50.,-7.89850297873842,-0.736923545827707));
#44958=CARTESIAN_POINT('Ctrl Pts',(-50.,-7.83877406317074,-0.72955527454762));
#44959=CARTESIAN_POINT('Ctrl Pts',(-50.,-7.79899409244038,-0.724242761304609));
#44960=CARTESIAN_POINT('Ctrl Pts',(-50.,-7.77911393348366,-0.721486423905757));
#44961=CARTESIAN_POINT('Origin',(-50.,-9.49333381220606,-0.489132040720954));
#44962=CARTESIAN_POINT('',(-50.,-10.125,-1.2399548841367E-15));
#44963=CARTESIAN_POINT('Origin',(-50.,0.,0.));
#44964=CARTESIAN_POINT('Origin',(-50.,0.,0.));
#44965=CARTESIAN_POINT('Origin',(-65.75,0.,0.));
#44966=CARTESIAN_POINT('',(-65.5,-10.3067057020436,2.58117077533865));
#44967=CARTESIAN_POINT('Origin',(-65.5,0.,0.));
#44968=CARTESIAN_POINT('',(-66.,-9.74369803606849,2.75244865200334));
#44969=CARTESIAN_POINT('Ctrl Pts',(-65.5,-10.3067057020436,2.58117077533865));
#44970=CARTESIAN_POINT('Ctrl Pts',(-65.66413580978,-10.1205863175662,2.64871173156175));
#44971=CARTESIAN_POINT('Ctrl Pts',(-65.8308421033592,-9.93250310566509,
2.70633121317366));
#44972=CARTESIAN_POINT('Ctrl Pts',(-66.,-9.74369803606849,2.75244865200334));
#44973=CARTESIAN_POINT('Origin',(-66.,0.,0.));
#44974=CARTESIAN_POINT('Origin',(-58.,0.,0.));
#44975=CARTESIAN_POINT('',(-50.5,-10.3067057020436,2.58117077533865));
#44976=CARTESIAN_POINT('Origin',(-50.5,0.,0.));
#44977=CARTESIAN_POINT('Ctrl Pts',(-50.5,-10.3067057020436,2.58117077533865));
#44978=CARTESIAN_POINT('Ctrl Pts',(-55.5,-10.3067057020436,2.58117077533865));
#44979=CARTESIAN_POINT('Ctrl Pts',(-60.5,-10.3067057020436,2.58117077533865));
#44980=CARTESIAN_POINT('Ctrl Pts',(-65.5,-10.3067057020436,2.58117077533865));
#44981=CARTESIAN_POINT('Origin',(-50.25,0.,0.));
#44982=CARTESIAN_POINT('',(-50.,-9.74369803606851,2.75244865200334));
#44983=CARTESIAN_POINT('Origin',(-50.,0.,0.));
#44984=CARTESIAN_POINT('Ctrl Pts',(-50.,-9.74369803606851,2.75244865200334));
#44985=CARTESIAN_POINT('Ctrl Pts',(-50.1691578966406,-9.93250310566499,
2.70633121317368));
#44986=CARTESIAN_POINT('Ctrl Pts',(-50.3358641902207,-10.120586317567,2.64871173156144));
#44987=CARTESIAN_POINT('Ctrl Pts',(-50.5,-10.3067057020436,2.58117077533865));
#44988=CARTESIAN_POINT('Origin',(-66.,-8.87153990628942,3.4144423723866));
#44989=CARTESIAN_POINT('',(-66.,-8.57244977261306,5.38783165067601));
#44990=CARTESIAN_POINT('Origin',(-66.,0.,0.));
#44991=CARTESIAN_POINT('',(-66.,-7.40002916450246,2.50494004209942));
#44992=CARTESIAN_POINT('Ctrl Pts',(-66.,-7.40002916450246,2.50494004209942));
#44993=CARTESIAN_POINT('Ctrl Pts',(-66.,-7.41931169683537,2.51050799170683));
#44994=CARTESIAN_POINT('Ctrl Pts',(-66.,-7.45781330220401,2.52183474112154));
#44995=CARTESIAN_POINT('Ctrl Pts',(-66.,-7.51537532763652,2.53939742897549));
#44996=CARTESIAN_POINT('Ctrl Pts',(-66.,-7.59174346395756,2.56396088352458));
#44997=CARTESIAN_POINT('Ctrl Pts',(-66.,-7.68659047952439,2.59650988815641));
#44998=CARTESIAN_POINT('Ctrl Pts',(-66.,-7.78089701296599,2.63068713780068));
#44999=CARTESIAN_POINT('Ctrl Pts',(-66.,-7.87481125204483,2.66605089991351));
#45000=CARTESIAN_POINT('Ctrl Pts',(-66.,-7.96858735303469,2.70184406566216));
#45001=CARTESIAN_POINT('Ctrl Pts',(-66.,-8.06260226894112,2.73694186696096));
#45002=CARTESIAN_POINT('Ctrl Pts',(-66.,-8.15728260249069,2.77005082217159));
#45003=CARTESIAN_POINT('Ctrl Pts',(-66.,-8.25303903993759,2.79988572902344));
#45004=CARTESIAN_POINT('Ctrl Pts',(-66.,-8.35020231164278,2.8253438589765));
#45005=CARTESIAN_POINT('Ctrl Pts',(-66.,-8.44894743956675,2.84570787805295));
#45006=CARTESIAN_POINT('Ctrl Pts',(-66.,-8.54925585128769,2.86075452374925));
#45007=CARTESIAN_POINT('Ctrl Pts',(-66.,-8.65098285136142,2.87059944718567));
#45008=CARTESIAN_POINT('Ctrl Pts',(-66.,-8.7539063267339,2.87559024133729));
#45009=CARTESIAN_POINT('Ctrl Pts',(-66.,-8.85777906856656,2.87618833666037));
#45010=CARTESIAN_POINT('Ctrl Pts',(-66.,-8.96238669582476,2.87284296703405));
#45011=CARTESIAN_POINT('Ctrl Pts',(-66.,-9.06757696100992,2.86591837692133));
#45012=CARTESIAN_POINT('Ctrl Pts',(-66.,-9.17323934599399,2.85571558912008));
#45013=CARTESIAN_POINT('Ctrl Pts',(-66.,-9.27929613150859,2.8424719880915));
#45014=CARTESIAN_POINT('Ctrl Pts',(-66.,-9.38568955693702,2.82637014921091));
#45015=CARTESIAN_POINT('Ctrl Pts',(-66.,-9.49236934178897,2.80754214008259));
#45016=CARTESIAN_POINT('Ctrl Pts',(-66.,-9.58533813500313,2.78887793905502));
#45017=CARTESIAN_POINT('Ctrl Pts',(-66.,-9.65702832718653,2.77306255439687));
#45018=CARTESIAN_POINT('Ctrl Pts',(-66.,-9.70734493152456,2.76126971555027));
#45019=CARTESIAN_POINT('Ctrl Pts',(-66.,-9.73624122804054,2.75427004847764));
#45020=CARTESIAN_POINT('Ctrl Pts',(-66.,-9.74369803606849,2.75244865200334));
#45021=CARTESIAN_POINT('',(-66.,-6.81311923233407,3.82316133271924));
#45022=CARTESIAN_POINT('Origin',(-66.,0.,0.));
#45023=CARTESIAN_POINT('Ctrl Pts',(-66.,-8.57244977261306,5.38783165067601));
#45024=CARTESIAN_POINT('Ctrl Pts',(-66.,-8.56382257497052,5.36991052437482));
#45025=CARTESIAN_POINT('Ctrl Pts',(-66.,-8.54292884255608,5.32830593066664));
#45026=CARTESIAN_POINT('Ctrl Pts',(-66.,-8.5083892410637,5.2660121538642));
#45027=CARTESIAN_POINT('Ctrl Pts',(-66.,-8.45816610437014,5.18725095270768));
#45028=CARTESIAN_POINT('Ctrl Pts',(-66.,-8.39088381069298,5.09368840385081));
#45029=CARTESIAN_POINT('Ctrl Pts',(-66.,-8.31785315284231,4.99561541360302));
#45030=CARTESIAN_POINT('Ctrl Pts',(-66.,-8.24398364800048,4.89528533686678));
#45031=CARTESIAN_POINT('Ctrl Pts',(-66.,-8.16895865357096,4.79341090596642));
#45032=CARTESIAN_POINT('Ctrl Pts',(-66.,-8.09178675852221,4.69261468439531));
#45033=CARTESIAN_POINT('Ctrl Pts',(-66.,-8.01120590115509,4.59630951471431));
#45034=CARTESIAN_POINT('Ctrl Pts',(-66.,-7.92626224077336,4.50707777519311));
#45035=CARTESIAN_POINT('Ctrl Pts',(-66.,-7.8366142398488,4.42585016826903));
#45036=CARTESIAN_POINT('Ctrl Pts',(-66.,-7.74237200893774,4.35245165160981));
#45037=CARTESIAN_POINT('Ctrl Pts',(-66.,-7.64403105809269,4.28586249972102));
#45038=CARTESIAN_POINT('Ctrl Pts',(-66.,-7.54237394375965,4.22459698165889));
#45039=CARTESIAN_POINT('Ctrl Pts',(-66.,-7.43838008066255,4.16699606204881));
#45040=CARTESIAN_POINT('Ctrl Pts',(-66.,-7.33308763494517,4.1113895497456));
#45041=CARTESIAN_POINT('Ctrl Pts',(-66.,-7.22746796441592,4.05626674182128));
#45042=CARTESIAN_POINT('Ctrl Pts',(-66.,-7.1222885976642,4.00045343685988));
#45043=CARTESIAN_POINT('Ctrl Pts',(-66.,-7.01799857910513,3.94326214747216));
#45044=CARTESIAN_POINT('Ctrl Pts',(-66.,-6.93545604316326,3.89613438608228));
#45045=CARTESIAN_POINT('Ctrl Pts',(-66.,-6.8740810318698,3.85996698713255));
#45046=CARTESIAN_POINT('Ctrl Pts',(-66.,-6.83340048002394,3.83549066847637));
#45047=CARTESIAN_POINT('Ctrl Pts',(-66.,-6.81311923233407,3.82316133271924));
#45048=CARTESIAN_POINT('Ctrl Pts',(-66.,-6.81311923233407,3.82316133271924));
#45049=CARTESIAN_POINT('Ctrl Pts',(-50.,-6.81311923233407,3.82316133271924));
#45050=CARTESIAN_POINT('Ctrl Pts',(-66.,-6.83340048002394,3.83549066847637));
#45051=CARTESIAN_POINT('Ctrl Pts',(-50.,-6.83340048002394,3.83549066847637));
#45052=CARTESIAN_POINT('Ctrl Pts',(-66.,-6.8740810318698,3.85996698713255));
#45053=CARTESIAN_POINT('Ctrl Pts',(-50.,-6.8740810318698,3.85996698713255));
#45054=CARTESIAN_POINT('Ctrl Pts',(-66.,-6.93545604316326,3.89613438608228));
#45055=CARTESIAN_POINT('Ctrl Pts',(-50.,-6.93545604316326,3.89613438608228));
#45056=CARTESIAN_POINT('Ctrl Pts',(-66.,-7.01799857910513,3.94326214747216));
#45057=CARTESIAN_POINT('Ctrl Pts',(-50.,-7.01799857910513,3.94326214747216));
#45058=CARTESIAN_POINT('Ctrl Pts',(-66.,-7.1222885976642,4.00045343685988));
#45059=CARTESIAN_POINT('Ctrl Pts',(-50.,-7.1222885976642,4.00045343685988));
#45060=CARTESIAN_POINT('Ctrl Pts',(-66.,-7.22746796441592,4.05626674182128));
#45061=CARTESIAN_POINT('Ctrl Pts',(-50.,-7.22746796441592,4.05626674182128));
#45062=CARTESIAN_POINT('Ctrl Pts',(-66.,-7.33308763494517,4.1113895497456));
#45063=CARTESIAN_POINT('Ctrl Pts',(-50.,-7.33308763494517,4.1113895497456));
#45064=CARTESIAN_POINT('Ctrl Pts',(-66.,-7.43838008066255,4.16699606204881));
#45065=CARTESIAN_POINT('Ctrl Pts',(-50.,-7.43838008066255,4.16699606204881));
#45066=CARTESIAN_POINT('Ctrl Pts',(-66.,-7.54237394375965,4.22459698165889));
#45067=CARTESIAN_POINT('Ctrl Pts',(-50.,-7.54237394375965,4.22459698165889));
#45068=CARTESIAN_POINT('Ctrl Pts',(-66.,-7.64403105809269,4.28586249972102));
#45069=CARTESIAN_POINT('Ctrl Pts',(-50.,-7.64403105809269,4.28586249972102));
#45070=CARTESIAN_POINT('Ctrl Pts',(-66.,-7.74237200893774,4.35245165160981));
#45071=CARTESIAN_POINT('Ctrl Pts',(-50.,-7.74237200893774,4.35245165160981));
#45072=CARTESIAN_POINT('Ctrl Pts',(-66.,-7.8366142398488,4.42585016826903));
#45073=CARTESIAN_POINT('Ctrl Pts',(-50.,-7.8366142398488,4.42585016826903));
#45074=CARTESIAN_POINT('Ctrl Pts',(-66.,-7.92626224077336,4.50707777519311));
#45075=CARTESIAN_POINT('Ctrl Pts',(-50.,-7.92626224077336,4.50707777519311));
#45076=CARTESIAN_POINT('Ctrl Pts',(-66.,-8.01120590115509,4.59630951471431));
#45077=CARTESIAN_POINT('Ctrl Pts',(-50.,-8.01120590115509,4.59630951471431));
#45078=CARTESIAN_POINT('Ctrl Pts',(-66.,-8.09178675852221,4.69261468439531));
#45079=CARTESIAN_POINT('Ctrl Pts',(-50.,-8.09178675852221,4.69261468439531));
#45080=CARTESIAN_POINT('Ctrl Pts',(-66.,-8.16895865357096,4.79341090596642));
#45081=CARTESIAN_POINT('Ctrl Pts',(-50.,-8.16895865357096,4.79341090596642));
#45082=CARTESIAN_POINT('Ctrl Pts',(-66.,-8.24398364800048,4.89528533686678));
#45083=CARTESIAN_POINT('Ctrl Pts',(-50.,-8.24398364800048,4.89528533686678));
#45084=CARTESIAN_POINT('Ctrl Pts',(-66.,-8.31785315284231,4.99561541360302));
#45085=CARTESIAN_POINT('Ctrl Pts',(-50.,-8.31785315284231,4.99561541360302));
#45086=CARTESIAN_POINT('Ctrl Pts',(-66.,-8.39088381069298,5.09368840385081));
#45087=CARTESIAN_POINT('Ctrl Pts',(-50.,-8.39088381069298,5.09368840385081));
#45088=CARTESIAN_POINT('Ctrl Pts',(-66.,-8.46203086798835,5.19262528100548));
#45089=CARTESIAN_POINT('Ctrl Pts',(-50.,-8.46203086798835,5.19262528100548));
#45090=CARTESIAN_POINT('Ctrl Pts',(-66.,-8.52910662358075,5.29873581494822));
#45091=CARTESIAN_POINT('Ctrl Pts',(-50.,-8.52910662358075,5.29873581494822));
#45092=CARTESIAN_POINT('Ctrl Pts',(-66.,-8.59004990429128,5.41789037245987));
#45093=CARTESIAN_POINT('Ctrl Pts',(-50.,-8.59004990429128,5.41789037245987));
#45094=CARTESIAN_POINT('Ctrl Pts',(-66.,-8.64386090104433,5.55284399091502));
#45095=CARTESIAN_POINT('Ctrl Pts',(-50.,-8.64386090104433,5.55284399091502));
#45096=CARTESIAN_POINT('Ctrl Pts',(-66.,-8.69181195387006,5.6997708284895));
#45097=CARTESIAN_POINT('Ctrl Pts',(-50.,-8.69181195387006,5.6997708284895));
#45098=CARTESIAN_POINT('Ctrl Pts',(-66.,-8.73814647121154,5.8462701562578));
#45099=CARTESIAN_POINT('Ctrl Pts',(-50.,-8.73814647121154,5.8462701562578));
#45100=CARTESIAN_POINT('Ctrl Pts',(-66.,-8.78885790167157,5.97489878611032));
#45101=CARTESIAN_POINT('Ctrl Pts',(-50.,-8.78885790167157,5.97489878611032));
#45102=CARTESIAN_POINT('Ctrl Pts',(-66.,-8.85073384792934,6.06594096807997));
#45103=CARTESIAN_POINT('Ctrl Pts',(-50.,-8.85073384792934,6.06594096807997));
#45104=CARTESIAN_POINT('Ctrl Pts',(-66.,-8.93034007876537,6.10035075259139));
#45105=CARTESIAN_POINT('Ctrl Pts',(-50.,-8.93034007876537,6.10035075259139));
#45106=CARTESIAN_POINT('Ctrl Pts',(-66.,-9.03293161543166,6.06290773317823));
#45107=CARTESIAN_POINT('Ctrl Pts',(-50.,-9.03293161543166,6.06290773317823));
#45108=CARTESIAN_POINT('Ctrl Pts',(-66.,-9.1625061724433,5.9420559998861));
#45109=CARTESIAN_POINT('Ctrl Pts',(-50.,-9.1625061724433,5.9420559998861));
#45110=CARTESIAN_POINT('Ctrl Pts',(-66.,-9.32201962027199,5.72927334958384));
#45111=CARTESIAN_POINT('Ctrl Pts',(-50.,-9.32201962027199,5.72927334958384));
#45112=CARTESIAN_POINT('Ctrl Pts',(-66.,-9.51353468950136,5.41863469758916));
#45113=CARTESIAN_POINT('Ctrl Pts',(-50.,-9.51353468950136,5.41863469758916));
#45114=CARTESIAN_POINT('Ctrl Pts',(-66.,-9.7383890962382,5.00631957015997));
#45115=CARTESIAN_POINT('Ctrl Pts',(-50.,-9.7383890962382,5.00631957015997));
#45116=CARTESIAN_POINT('Ctrl Pts',(-66.,-9.99734717600606,4.4901678734951));
#45117=CARTESIAN_POINT('Ctrl Pts',(-50.,-9.99734717600606,4.4901678734951));
#45118=CARTESIAN_POINT('Ctrl Pts',(-66.,-10.2907511765059,3.86923704869354));
#45119=CARTESIAN_POINT('Ctrl Pts',(-50.,-10.2907511765059,3.86923704869354));
#45120=CARTESIAN_POINT('Ctrl Pts',(-66.,-10.553083029885,3.28855031576864));
#45121=CARTESIAN_POINT('Ctrl Pts',(-50.,-10.553083029885,3.28855031576864));
#45122=CARTESIAN_POINT('Ctrl Pts',(-66.,-10.765329928439,2.80592201479919));
#45123=CARTESIAN_POINT('Ctrl Pts',(-50.,-10.765329928439,2.80592201479919));
#45124=CARTESIAN_POINT('Ctrl Pts',(-66.,-10.9137067077809,2.46325842726184));
#45125=CARTESIAN_POINT('Ctrl Pts',(-50.,-10.9137067077809,2.46325842726184));
#45126=CARTESIAN_POINT('Ctrl Pts',(-66.,-10.9896148096924,2.28669878527756));
#45127=CARTESIAN_POINT('Ctrl Pts',(-50.,-10.9896148096924,2.28669878527756));
#45128=CARTESIAN_POINT('',(-65.5,-8.79190251708467,5.96599322242996));
#45129=CARTESIAN_POINT('Ctrl Pts',(-66.,-8.57244977261307,5.38783165067601));
#45130=CARTESIAN_POINT('Ctrl Pts',(-65.7982417703062,-8.67580691746,5.60253363429554));
#45131=CARTESIAN_POINT('Ctrl Pts',(-65.6331946192803,-8.72156901755385,
5.83243162948398));
#45132=CARTESIAN_POINT('Ctrl Pts',(-65.5,-8.79190251708467,5.96599322242995));
#45133=CARTESIAN_POINT('',(-50.,-6.81311923233407,3.82316133271924));
#45134=CARTESIAN_POINT('',(-66.,-6.81311923233407,3.82316133271924));
#45135=CARTESIAN_POINT('',(-50.,-8.57244977261307,5.38783165067603));
#45136=CARTESIAN_POINT('Ctrl Pts',(-50.,-6.81311923233407,3.82316133271924));
#45137=CARTESIAN_POINT('Ctrl Pts',(-50.,-6.83340048002394,3.83549066847637));
#45138=CARTESIAN_POINT('Ctrl Pts',(-50.,-6.8740810318698,3.85996698713255));
#45139=CARTESIAN_POINT('Ctrl Pts',(-50.,-6.93545604316326,3.89613438608228));
#45140=CARTESIAN_POINT('Ctrl Pts',(-50.,-7.01799857910513,3.94326214747216));
#45141=CARTESIAN_POINT('Ctrl Pts',(-50.,-7.1222885976642,4.00045343685988));
#45142=CARTESIAN_POINT('Ctrl Pts',(-50.,-7.22746796441592,4.05626674182128));
#45143=CARTESIAN_POINT('Ctrl Pts',(-50.,-7.33308763494517,4.1113895497456));
#45144=CARTESIAN_POINT('Ctrl Pts',(-50.,-7.43838008066255,4.16699606204881));
#45145=CARTESIAN_POINT('Ctrl Pts',(-50.,-7.54237394375965,4.22459698165889));
#45146=CARTESIAN_POINT('Ctrl Pts',(-50.,-7.64403105809269,4.28586249972102));
#45147=CARTESIAN_POINT('Ctrl Pts',(-50.,-7.74237200893774,4.35245165160981));
#45148=CARTESIAN_POINT('Ctrl Pts',(-50.,-7.8366142398488,4.42585016826903));
#45149=CARTESIAN_POINT('Ctrl Pts',(-50.,-7.92626224077336,4.50707777519311));
#45150=CARTESIAN_POINT('Ctrl Pts',(-50.,-8.01120590115509,4.59630951471431));
#45151=CARTESIAN_POINT('Ctrl Pts',(-50.,-8.09178675852221,4.69261468439531));
#45152=CARTESIAN_POINT('Ctrl Pts',(-50.,-8.16895865357096,4.79341090596642));
#45153=CARTESIAN_POINT('Ctrl Pts',(-50.,-8.24398364800048,4.89528533686678));
#45154=CARTESIAN_POINT('Ctrl Pts',(-50.,-8.31785315284231,4.99561541360302));
#45155=CARTESIAN_POINT('Ctrl Pts',(-50.,-8.39088381069298,5.09368840385081));
#45156=CARTESIAN_POINT('Ctrl Pts',(-50.,-8.45816610437014,5.18725095270769));
#45157=CARTESIAN_POINT('Ctrl Pts',(-50.,-8.5083892410637,5.26601215386421));
#45158=CARTESIAN_POINT('Ctrl Pts',(-50.,-8.54292884255608,5.32830593066665));
#45159=CARTESIAN_POINT('Ctrl Pts',(-50.,-8.56382257497053,5.36991052437484));
#45160=CARTESIAN_POINT('Ctrl Pts',(-50.,-8.57244977261307,5.38783165067603));
#45161=CARTESIAN_POINT('',(-50.5,-8.79190251708467,5.96599322242996));
#45162=CARTESIAN_POINT('Ctrl Pts',(-50.5,-8.79190251708468,5.96599322242997));
#45163=CARTESIAN_POINT('Ctrl Pts',(-50.4513355279182,-8.76620521307325,
5.91719467151072));
#45164=CARTESIAN_POINT('Ctrl Pts',(-50.3988319785486,-8.74374680112151,
5.85659632440327));
#45165=CARTESIAN_POINT('Ctrl Pts',(-50.2385977000686,-8.67884981036978,
5.66466221597345));
#45166=CARTESIAN_POINT('Ctrl Pts',(-50.1319260151113,-8.64003311864876,
5.52822134966582));
#45167=CARTESIAN_POINT('Ctrl Pts',(-50.,-8.57244977261307,5.38783165067603));
#45168=CARTESIAN_POINT('Ctrl Pts',(-65.5,-8.79190251708467,5.96599322242996));
#45169=CARTESIAN_POINT('Ctrl Pts',(-60.5,-8.79190251708467,5.96599322242996));
#45170=CARTESIAN_POINT('Ctrl Pts',(-55.5,-8.79190251708467,5.96599322242996));
#45171=CARTESIAN_POINT('Ctrl Pts',(-50.5,-8.79190251708467,5.96599322242996));
#45172=CARTESIAN_POINT('Origin',(-66.,0.,0.));
#45173=CARTESIAN_POINT('',(-50.,-7.40002916450246,2.50494004209942));
#45174=CARTESIAN_POINT('',(-66.,-7.40002916450246,2.50494004209942));
#45175=CARTESIAN_POINT('Origin',(-50.,0.,0.));
#45176=CARTESIAN_POINT('Ctrl Pts',(-66.,-10.9896148096924,2.28669878527756));
#45177=CARTESIAN_POINT('Ctrl Pts',(-50.,-10.9896148096924,2.28669878527756));
#45178=CARTESIAN_POINT('Ctrl Pts',(-66.,-10.9684161512126,2.29727350719238));
#45179=CARTESIAN_POINT('Ctrl Pts',(-50.,-10.9684161512126,2.29727350719238));
#45180=CARTESIAN_POINT('Ctrl Pts',(-66.,-10.9259986747394,2.31821040407718));
#45181=CARTESIAN_POINT('Ctrl Pts',(-50.,-10.9259986747394,2.31821040407718));
#45182=CARTESIAN_POINT('Ctrl Pts',(-66.,-10.8623119817454,2.34897810856224));
#45183=CARTESIAN_POINT('Ctrl Pts',(-50.,-10.8623119817454,2.34897810856224));
#45184=CARTESIAN_POINT('Ctrl Pts',(-66.,-10.7772752714148,2.3887247370365));
#45185=CARTESIAN_POINT('Ctrl Pts',(-50.,-10.7772752714148,2.3887247370365));
#45186=CARTESIAN_POINT('Ctrl Pts',(-66.,-10.6707784343856,2.4362669175464));
#45187=CARTESIAN_POINT('Ctrl Pts',(-50.,-10.6707784343856,2.4362669175464));
#45188=CARTESIAN_POINT('Ctrl Pts',(-66.,-10.5640849911537,2.48164669841744));
#45189=CARTESIAN_POINT('Ctrl Pts',(-50.,-10.5640849911537,2.48164669841744));
#45190=CARTESIAN_POINT('Ctrl Pts',(-66.,-10.4572049564432,2.52483446494625));
#45191=CARTESIAN_POINT('Ctrl Pts',(-50.,-10.4572049564432,2.52483446494625));
#45192=CARTESIAN_POINT('Ctrl Pts',(-66.,-10.3501560465217,2.56579274006262));
#45193=CARTESIAN_POINT('Ctrl Pts',(-50.,-10.3501560465217,2.56579274006262));
#45194=CARTESIAN_POINT('Ctrl Pts',(-66.,-10.2429664006725,2.60447642727633));
#45195=CARTESIAN_POINT('Ctrl Pts',(-50.,-10.2429664006725,2.60447642727633));
#45196=CARTESIAN_POINT('Ctrl Pts',(-66.,-10.1356731120406,2.64083547340864));
#45197=CARTESIAN_POINT('Ctrl Pts',(-50.,-10.1356731120406,2.64083547340864));
#45198=CARTESIAN_POINT('Ctrl Pts',(-66.,-10.0283197583604,2.67481805512507));
#45199=CARTESIAN_POINT('Ctrl Pts',(-50.,-10.0283197583604,2.67481805512507));
#45200=CARTESIAN_POINT('Ctrl Pts',(-66.,-9.92095426270504,2.70637422995761));
#45201=CARTESIAN_POINT('Ctrl Pts',(-50.,-9.92095426270504,2.70637422995761));
#45202=CARTESIAN_POINT('Ctrl Pts',(-66.,-9.8136267879847,2.73545878100293));
#45203=CARTESIAN_POINT('Ctrl Pts',(-50.,-9.8136267879847,2.73545878100293));
#45204=CARTESIAN_POINT('Ctrl Pts',(-66.,-9.70638729315513,2.7620369717482));
#45205=CARTESIAN_POINT('Ctrl Pts',(-50.,-9.70638729315513,2.7620369717482));
#45206=CARTESIAN_POINT('Ctrl Pts',(-66.,-9.59928504165258,2.78607799016444));
#45207=CARTESIAN_POINT('Ctrl Pts',(-50.,-9.59928504165258,2.78607799016444));
#45208=CARTESIAN_POINT('Ctrl Pts',(-66.,-9.49236934178897,2.80754214008259));
#45209=CARTESIAN_POINT('Ctrl Pts',(-50.,-9.49236934178897,2.80754214008259));
#45210=CARTESIAN_POINT('Ctrl Pts',(-66.,-9.38568955693702,2.82637014921091));
#45211=CARTESIAN_POINT('Ctrl Pts',(-50.,-9.38568955693702,2.82637014921091));
#45212=CARTESIAN_POINT('Ctrl Pts',(-66.,-9.27929613150859,2.8424719880915));
#45213=CARTESIAN_POINT('Ctrl Pts',(-50.,-9.27929613150859,2.8424719880915));
#45214=CARTESIAN_POINT('Ctrl Pts',(-66.,-9.17323934599399,2.85571558912008));
#45215=CARTESIAN_POINT('Ctrl Pts',(-50.,-9.17323934599399,2.85571558912008));
#45216=CARTESIAN_POINT('Ctrl Pts',(-66.,-9.06757696100992,2.86591837692133));
#45217=CARTESIAN_POINT('Ctrl Pts',(-50.,-9.06757696100992,2.86591837692133));
#45218=CARTESIAN_POINT('Ctrl Pts',(-66.,-8.96238669582476,2.87284296703405));
#45219=CARTESIAN_POINT('Ctrl Pts',(-50.,-8.96238669582476,2.87284296703405));
#45220=CARTESIAN_POINT('Ctrl Pts',(-66.,-8.85777906856656,2.87618833666037));
#45221=CARTESIAN_POINT('Ctrl Pts',(-50.,-8.85777906856656,2.87618833666037));
#45222=CARTESIAN_POINT('Ctrl Pts',(-66.,-8.7539063267339,2.87559024133729));
#45223=CARTESIAN_POINT('Ctrl Pts',(-50.,-8.7539063267339,2.87559024133729));
#45224=CARTESIAN_POINT('Ctrl Pts',(-66.,-8.65098285136142,2.87059944718567));
#45225=CARTESIAN_POINT('Ctrl Pts',(-50.,-8.65098285136142,2.87059944718567));
#45226=CARTESIAN_POINT('Ctrl Pts',(-66.,-8.54925585128769,2.86075452374925));
#45227=CARTESIAN_POINT('Ctrl Pts',(-50.,-8.54925585128769,2.86075452374925));
#45228=CARTESIAN_POINT('Ctrl Pts',(-66.,-8.44894743956675,2.84570787805295));
#45229=CARTESIAN_POINT('Ctrl Pts',(-50.,-8.44894743956675,2.84570787805295));
#45230=CARTESIAN_POINT('Ctrl Pts',(-66.,-8.35020231164278,2.8253438589765));
#45231=CARTESIAN_POINT('Ctrl Pts',(-50.,-8.35020231164278,2.8253438589765));
#45232=CARTESIAN_POINT('Ctrl Pts',(-66.,-8.25303903993759,2.79988572902344));
#45233=CARTESIAN_POINT('Ctrl Pts',(-50.,-8.25303903993759,2.79988572902344));
#45234=CARTESIAN_POINT('Ctrl Pts',(-66.,-8.15728260249069,2.77005082217159));
#45235=CARTESIAN_POINT('Ctrl Pts',(-50.,-8.15728260249069,2.77005082217159));
#45236=CARTESIAN_POINT('Ctrl Pts',(-66.,-8.06260226894112,2.73694186696096));
#45237=CARTESIAN_POINT('Ctrl Pts',(-50.,-8.06260226894112,2.73694186696096));
#45238=CARTESIAN_POINT('Ctrl Pts',(-66.,-7.96858735303469,2.70184406566216));
#45239=CARTESIAN_POINT('Ctrl Pts',(-50.,-7.96858735303469,2.70184406566216));
#45240=CARTESIAN_POINT('Ctrl Pts',(-66.,-7.87481125204483,2.66605089991351));
#45241=CARTESIAN_POINT('Ctrl Pts',(-50.,-7.87481125204483,2.66605089991351));
#45242=CARTESIAN_POINT('Ctrl Pts',(-66.,-7.78089701296599,2.63068713780068));
#45243=CARTESIAN_POINT('Ctrl Pts',(-50.,-7.78089701296599,2.63068713780068));
#45244=CARTESIAN_POINT('Ctrl Pts',(-66.,-7.68659047952439,2.59650988815641));
#45245=CARTESIAN_POINT('Ctrl Pts',(-50.,-7.68659047952439,2.59650988815641));
#45246=CARTESIAN_POINT('Ctrl Pts',(-66.,-7.59174346395756,2.56396088352458));
#45247=CARTESIAN_POINT('Ctrl Pts',(-50.,-7.59174346395756,2.56396088352458));
#45248=CARTESIAN_POINT('Ctrl Pts',(-66.,-7.51537532763652,2.53939742897549));
#45249=CARTESIAN_POINT('Ctrl Pts',(-50.,-7.51537532763652,2.53939742897549));
#45250=CARTESIAN_POINT('Ctrl Pts',(-66.,-7.45781330220401,2.52183474112154));
#45251=CARTESIAN_POINT('Ctrl Pts',(-50.,-7.45781330220401,2.52183474112154));
#45252=CARTESIAN_POINT('Ctrl Pts',(-66.,-7.41931169683537,2.51050799170683));
#45253=CARTESIAN_POINT('Ctrl Pts',(-50.,-7.41931169683537,2.51050799170683));
#45254=CARTESIAN_POINT('Ctrl Pts',(-66.,-7.40002916450246,2.50494004209942));
#45255=CARTESIAN_POINT('Ctrl Pts',(-50.,-7.40002916450246,2.50494004209942));
#45256=CARTESIAN_POINT('Ctrl Pts',(-50.,-9.74369803606851,2.75244865200334));
#45257=CARTESIAN_POINT('Ctrl Pts',(-50.,-9.73624122804056,2.75427004847764));
#45258=CARTESIAN_POINT('Ctrl Pts',(-50.,-9.70734493152457,2.76126971555026));
#45259=CARTESIAN_POINT('Ctrl Pts',(-50.,-9.65702832718653,2.77306255439687));
#45260=CARTESIAN_POINT('Ctrl Pts',(-50.,-9.58533813500313,2.78887793905502));
#45261=CARTESIAN_POINT('Ctrl Pts',(-50.,-9.49236934178897,2.80754214008259));
#45262=CARTESIAN_POINT('Ctrl Pts',(-50.,-9.38568955693702,2.82637014921091));
#45263=CARTESIAN_POINT('Ctrl Pts',(-50.,-9.27929613150859,2.8424719880915));
#45264=CARTESIAN_POINT('Ctrl Pts',(-50.,-9.17323934599399,2.85571558912008));
#45265=CARTESIAN_POINT('Ctrl Pts',(-50.,-9.06757696100992,2.86591837692133));
#45266=CARTESIAN_POINT('Ctrl Pts',(-50.,-8.96238669582476,2.87284296703405));
#45267=CARTESIAN_POINT('Ctrl Pts',(-50.,-8.85777906856656,2.87618833666037));
#45268=CARTESIAN_POINT('Ctrl Pts',(-50.,-8.7539063267339,2.87559024133729));
#45269=CARTESIAN_POINT('Ctrl Pts',(-50.,-8.65098285136142,2.87059944718567));
#45270=CARTESIAN_POINT('Ctrl Pts',(-50.,-8.54925585128769,2.86075452374925));
#45271=CARTESIAN_POINT('Ctrl Pts',(-50.,-8.44894743956675,2.84570787805295));
#45272=CARTESIAN_POINT('Ctrl Pts',(-50.,-8.35020231164278,2.8253438589765));
#45273=CARTESIAN_POINT('Ctrl Pts',(-50.,-8.25303903993759,2.79988572902344));
#45274=CARTESIAN_POINT('Ctrl Pts',(-50.,-8.15728260249069,2.77005082217159));
#45275=CARTESIAN_POINT('Ctrl Pts',(-50.,-8.06260226894112,2.73694186696096));
#45276=CARTESIAN_POINT('Ctrl Pts',(-50.,-7.96858735303469,2.70184406566216));
#45277=CARTESIAN_POINT('Ctrl Pts',(-50.,-7.87481125204483,2.66605089991351));
#45278=CARTESIAN_POINT('Ctrl Pts',(-50.,-7.78089701296599,2.63068713780068));
#45279=CARTESIAN_POINT('Ctrl Pts',(-50.,-7.68659047952439,2.59650988815641));
#45280=CARTESIAN_POINT('Ctrl Pts',(-50.,-7.59174346395756,2.56396088352458));
#45281=CARTESIAN_POINT('Ctrl Pts',(-50.,-7.51537532763652,2.53939742897549));
#45282=CARTESIAN_POINT('Ctrl Pts',(-50.,-7.45781330220401,2.52183474112154));
#45283=CARTESIAN_POINT('Ctrl Pts',(-50.,-7.41931169683537,2.51050799170683));
#45284=CARTESIAN_POINT('Ctrl Pts',(-50.,-7.40002916450246,2.50494004209942));
#45285=CARTESIAN_POINT('Origin',(-50.,-8.87153990628942,3.4144423723866));
#45286=CARTESIAN_POINT('Origin',(-50.,0.,0.));
#45287=CARTESIAN_POINT('Origin',(-65.75,0.,0.));
#45288=CARTESIAN_POINT('',(-65.5,-8.3657874409944,6.55013171562987));
#45289=CARTESIAN_POINT('Origin',(-65.5,0.,0.));
#45290=CARTESIAN_POINT('',(-66.,-7.78178935653715,6.47760599376692));
#45291=CARTESIAN_POINT('Ctrl Pts',(-65.5,-8.36578744099439,6.55013171562987));
#45292=CARTESIAN_POINT('Ctrl Pts',(-65.6642917360002,-8.16809991938447,
6.5361185761295));
#45293=CARTESIAN_POINT('Ctrl Pts',(-65.831118235484,-7.97271684425891,6.51221297265958));
#45294=CARTESIAN_POINT('Ctrl Pts',(-66.,-7.78178935653715,6.47760599376692));
#45295=CARTESIAN_POINT('Origin',(-66.,0.,0.));
#45296=CARTESIAN_POINT('Origin',(-58.,0.,0.));
#45297=CARTESIAN_POINT('',(-50.5,-8.3657874409944,6.55013171562987));
#45298=CARTESIAN_POINT('Origin',(-50.5,0.,0.));
#45299=CARTESIAN_POINT('Ctrl Pts',(-50.5,-8.3657874409944,6.55013171562987));
#45300=CARTESIAN_POINT('Ctrl Pts',(-55.5,-8.3657874409944,6.55013171562987));
#45301=CARTESIAN_POINT('Ctrl Pts',(-60.5,-8.3657874409944,6.55013171562987));
#45302=CARTESIAN_POINT('Ctrl Pts',(-65.5,-8.3657874409944,6.55013171562987));
#45303=CARTESIAN_POINT('Origin',(-50.25,0.,0.));
#45304=CARTESIAN_POINT('',(-50.,-7.78178935653717,6.47760599376692));
#45305=CARTESIAN_POINT('Origin',(-50.,0.,0.));
#45306=CARTESIAN_POINT('Ctrl Pts',(-50.,-7.78178935653716,6.47760599376692));
#45307=CARTESIAN_POINT('Ctrl Pts',(-50.1688817645156,-7.97271684425845,
6.5122129726595));
#45308=CARTESIAN_POINT('Ctrl Pts',(-50.3357082639993,-8.16809991938399,
6.53611857612945));
#45309=CARTESIAN_POINT('Ctrl Pts',(-50.5,-8.36578744099441,6.55013171562987));
#45310=CARTESIAN_POINT('Origin',(-66.,-6.71577615516547,6.72762868007336));
#45311=CARTESIAN_POINT('',(-66.,-5.63989399158651,8.40875857446665));
#45312=CARTESIAN_POINT('Origin',(-66.,0.,0.));
#45313=CARTESIAN_POINT('',(-66.,-5.74141212582432,5.29823961815974));
#45314=CARTESIAN_POINT('Ctrl Pts',(-66.,-5.74141212582432,5.29823961815974));
#45315=CARTESIAN_POINT('Ctrl Pts',(-66.,-5.75676290651676,5.31116910570307));
#45316=CARTESIAN_POINT('Ctrl Pts',(-66.,-5.78732886917933,5.33717661990139));
#45317=CARTESIAN_POINT('Ctrl Pts',(-66.,-5.8327710073448,5.37663351860743));
#45318=CARTESIAN_POINT('Ctrl Pts',(-66.,-5.89254591434388,5.43013507033993));
#45319=CARTESIAN_POINT('Ctrl Pts',(-66.,-5.96595410170651,5.49844782238954));
#45320=CARTESIAN_POINT('Ctrl Pts',(-66.,-6.03820626716823,5.56802821638893));
#45321=CARTESIAN_POINT('Ctrl Pts',(-66.,-6.10961745579836,5.63853298297221));
#45322=CARTESIAN_POINT('Ctrl Pts',(-66.,-6.18072779481142,5.70937384347389));
#45323=CARTESIAN_POINT('Ctrl Pts',(-66.,-6.25233913230877,5.77967659171849));
#45324=CARTESIAN_POINT('Ctrl Pts',(-66.,-6.32536729565295,5.8484330883917));
#45325=CARTESIAN_POINT('Ctrl Pts',(-66.,-6.4007102042632,5.91463628394544));
#45326=CARTESIAN_POINT('Ctrl Pts',(-66.,-6.47911851546308,5.97741330588777));
#45327=CARTESIAN_POINT('Ctrl Pts',(-66.,-6.56104388578368,6.03618002486629));
#45328=CARTESIAN_POINT('Ctrl Pts',(-66.,-6.64656015751461,6.09072492635055));
#45329=CARTESIAN_POINT('Ctrl Pts',(-66.,-6.73548810524172,6.14109480995689));
#45330=CARTESIAN_POINT('Ctrl Pts',(-66.,-6.82748343979352,6.18751687615083));
#45331=CARTESIAN_POINT('Ctrl Pts',(-66.,-6.92213264398368,6.23031211373657));
#45332=CARTESIAN_POINT('Ctrl Pts',(-66.,-7.01905715111184,6.26980372166142));
#45333=CARTESIAN_POINT('Ctrl Pts',(-66.,-7.11796972459708,6.30626252916358));
#45334=CARTESIAN_POINT('Ctrl Pts',(-66.,-7.21864696410326,6.33991858248025));
#45335=CARTESIAN_POINT('Ctrl Pts',(-66.,-7.3209213165869,6.37095713183339));
#45336=CARTESIAN_POINT('Ctrl Pts',(-66.,-7.42466575500371,6.39952147476842));
#45337=CARTESIAN_POINT('Ctrl Pts',(-66.,-7.52978062910616,6.42571181012752));
#45338=CARTESIAN_POINT('Ctrl Pts',(-66.,-7.62230326232111,6.44647502892099));
#45339=CARTESIAN_POINT('Ctrl Pts',(-66.,-7.69422820821259,6.46118598421581));
#45340=CARTESIAN_POINT('Ctrl Pts',(-66.,-7.7449912932344,6.47087829659421));
#45341=CARTESIAN_POINT('Ctrl Pts',(-66.,-7.77423639474703,6.47623696517724));
#45342=CARTESIAN_POINT('Ctrl Pts',(-66.,-7.78178935653715,6.47760599376692));
#45343=CARTESIAN_POINT('',(-66.,-4.66907432066881,6.26377691477523));
#45344=CARTESIAN_POINT('Origin',(-66.,0.,0.));
#45345=CARTESIAN_POINT('Ctrl Pts',(-66.,-5.63989399158651,8.40875857446665));
#45346=CARTESIAN_POINT('Ctrl Pts',(-66.,-5.63930183311986,8.38887781353008));
#45347=CARTESIAN_POINT('Ctrl Pts',(-66.,-5.63713657156084,8.34237187934733));
#45348=CARTESIAN_POINT('Ctrl Pts',(-66.,-5.63092023716983,8.27141516094587));
#45349=CARTESIAN_POINT('Ctrl Pts',(-66.,-5.61707418533788,8.17903563336739));
#45350=CARTESIAN_POINT('Ctrl Pts',(-66.,-5.593664068609,8.06619581758504));
#45351=CARTESIAN_POINT('Ctrl Pts',(-66.,-5.56683712169066,7.94689743821095));
#45352=CARTESIAN_POINT('Ctrl Pts',(-66.,-5.54016188969533,7.82519591791858));
#45353=CARTESIAN_POINT('Ctrl Pts',(-66.,-5.51305921086426,7.70161357993859));
#45354=CARTESIAN_POINT('Ctrl Pts',(-66.,-5.48355669348136,7.57814301204284));
#45355=CARTESIAN_POINT('Ctrl Pts',(-66.,-5.44911325868757,7.45738867431159));
#45356=CARTESIAN_POINT('Ctrl Pts',(-66.,-5.40780718177897,7.34132172472021));
#45357=CARTESIAN_POINT('Ctrl Pts',(-66.,-5.35894790191298,7.23065348642503));
#45358=CARTESIAN_POINT('Ctrl Pts',(-66.,-5.3027072062188,7.12526883629655));
#45359=CARTESIAN_POINT('Ctrl Pts',(-66.,-5.23995252537855,7.02443775083668));
#45360=CARTESIAN_POINT('Ctrl Pts',(-66.,-5.17200306149544,6.92712124167231));
#45361=CARTESIAN_POINT('Ctrl Pts',(-66.,-5.10042834492066,6.83220206842988));
#45362=CARTESIAN_POINT('Ctrl Pts',(-66.,-5.02685611555883,6.7385766957876));
#45363=CARTESIAN_POINT('Ctrl Pts',(-66.,-4.95278821116117,6.645260114762));
#45364=CARTESIAN_POINT('Ctrl Pts',(-66.,-4.87940339472638,6.55149182098506));
#45365=CARTESIAN_POINT('Ctrl Pts',(-66.,-4.80739151505302,6.45682640629315));
#45366=CARTESIAN_POINT('Ctrl Pts',(-66.,-4.75115374374443,6.3801999799666));
#45367=CARTESIAN_POINT('Ctrl Pts',(-66.,-4.70979548740211,6.32219595087909));
#45368=CARTESIAN_POINT('Ctrl Pts',(-66.,-4.68258736973401,6.28328945005467));
#45369=CARTESIAN_POINT('Ctrl Pts',(-66.,-4.66907432066881,6.26377691477523));
#45370=CARTESIAN_POINT('Ctrl Pts',(-66.,-4.66907432066881,6.26377691477523));
#45371=CARTESIAN_POINT('Ctrl Pts',(-50.,-4.66907432066881,6.26377691477523));
#45372=CARTESIAN_POINT('Ctrl Pts',(-66.,-4.68258736973401,6.28328945005467));
#45373=CARTESIAN_POINT('Ctrl Pts',(-50.,-4.68258736973401,6.28328945005467));
#45374=CARTESIAN_POINT('Ctrl Pts',(-66.,-4.70979548740211,6.32219595087909));
#45375=CARTESIAN_POINT('Ctrl Pts',(-50.,-4.70979548740211,6.32219595087909));
#45376=CARTESIAN_POINT('Ctrl Pts',(-66.,-4.75115374374443,6.3801999799666));
#45377=CARTESIAN_POINT('Ctrl Pts',(-50.,-4.75115374374443,6.3801999799666));
#45378=CARTESIAN_POINT('Ctrl Pts',(-66.,-4.80739151505302,6.45682640629315));
#45379=CARTESIAN_POINT('Ctrl Pts',(-50.,-4.80739151505302,6.45682640629315));
#45380=CARTESIAN_POINT('Ctrl Pts',(-66.,-4.87940339472638,6.55149182098506));
#45381=CARTESIAN_POINT('Ctrl Pts',(-50.,-4.87940339472638,6.55149182098506));
#45382=CARTESIAN_POINT('Ctrl Pts',(-66.,-4.95278821116117,6.645260114762));
#45383=CARTESIAN_POINT('Ctrl Pts',(-50.,-4.95278821116117,6.645260114762));
#45384=CARTESIAN_POINT('Ctrl Pts',(-66.,-5.02685611555883,6.7385766957876));
#45385=CARTESIAN_POINT('Ctrl Pts',(-50.,-5.02685611555883,6.7385766957876));
#45386=CARTESIAN_POINT('Ctrl Pts',(-66.,-5.10042834492066,6.83220206842988));
#45387=CARTESIAN_POINT('Ctrl Pts',(-50.,-5.10042834492066,6.83220206842988));
#45388=CARTESIAN_POINT('Ctrl Pts',(-66.,-5.17200306149544,6.92712124167231));
#45389=CARTESIAN_POINT('Ctrl Pts',(-50.,-5.17200306149544,6.92712124167231));
#45390=CARTESIAN_POINT('Ctrl Pts',(-66.,-5.23995252537855,7.02443775083668));
#45391=CARTESIAN_POINT('Ctrl Pts',(-50.,-5.23995252537855,7.02443775083668));
#45392=CARTESIAN_POINT('Ctrl Pts',(-66.,-5.3027072062188,7.12526883629655));
#45393=CARTESIAN_POINT('Ctrl Pts',(-50.,-5.3027072062188,7.12526883629655));
#45394=CARTESIAN_POINT('Ctrl Pts',(-66.,-5.35894790191298,7.23065348642503));
#45395=CARTESIAN_POINT('Ctrl Pts',(-50.,-5.35894790191298,7.23065348642503));
#45396=CARTESIAN_POINT('Ctrl Pts',(-66.,-5.40780718177897,7.34132172472021));
#45397=CARTESIAN_POINT('Ctrl Pts',(-50.,-5.40780718177897,7.34132172472021));
#45398=CARTESIAN_POINT('Ctrl Pts',(-66.,-5.44911325868757,7.45738867431159));
#45399=CARTESIAN_POINT('Ctrl Pts',(-50.,-5.44911325868757,7.45738867431159));
#45400=CARTESIAN_POINT('Ctrl Pts',(-66.,-5.48355669348136,7.57814301204284));
#45401=CARTESIAN_POINT('Ctrl Pts',(-50.,-5.48355669348136,7.57814301204284));
#45402=CARTESIAN_POINT('Ctrl Pts',(-66.,-5.51305921086426,7.70161357993859));
#45403=CARTESIAN_POINT('Ctrl Pts',(-50.,-5.51305921086426,7.70161357993859));
#45404=CARTESIAN_POINT('Ctrl Pts',(-66.,-5.54016188969533,7.82519591791858));
#45405=CARTESIAN_POINT('Ctrl Pts',(-50.,-5.54016188969533,7.82519591791858));
#45406=CARTESIAN_POINT('Ctrl Pts',(-66.,-5.56683712169066,7.94689743821095));
#45407=CARTESIAN_POINT('Ctrl Pts',(-50.,-5.56683712169066,7.94689743821095));
#45408=CARTESIAN_POINT('Ctrl Pts',(-66.,-5.593664068609,8.06619581758504));
#45409=CARTESIAN_POINT('Ctrl Pts',(-50.,-5.593664068609,8.06619581758504));
#45410=CARTESIAN_POINT('Ctrl Pts',(-66.,-5.61841888633553,8.18551726755207));
#45411=CARTESIAN_POINT('Ctrl Pts',(-50.,-5.61841888633553,8.18551726755207));
#45412=CARTESIAN_POINT('Ctrl Pts',(-66.,-5.63653659580406,8.30973623150492));
#45413=CARTESIAN_POINT('Ctrl Pts',(-50.,-5.63653659580406,8.30973623150492));
#45414=CARTESIAN_POINT('Ctrl Pts',(-66.,-5.64374652834153,8.44337720169133));
#45415=CARTESIAN_POINT('Ctrl Pts',(-50.,-5.64374652834153,8.44337720169133));
#45416=CARTESIAN_POINT('Ctrl Pts',(-66.,-5.63801473825513,8.58855037100336));
#45417=CARTESIAN_POINT('Ctrl Pts',(-50.,-5.63801473825513,8.58855037100336));
#45418=CARTESIAN_POINT('Ctrl Pts',(-66.,-5.62205967606046,8.74227816633361));
#45419=CARTESIAN_POINT('Ctrl Pts',(-50.,-5.62205967606046,8.74227816633361));
#45420=CARTESIAN_POINT('Ctrl Pts',(-66.,-5.60480171912049,8.89495790780604));
#45421=CARTESIAN_POINT('Ctrl Pts',(-50.,-5.60480171912049,8.89495790780604));
#45422=CARTESIAN_POINT('Ctrl Pts',(-66.,-5.59881093895816,9.0330922053215));
#45423=CARTESIAN_POINT('Ctrl Pts',(-50.,-5.59881093895816,9.0330922053215));
#45424=CARTESIAN_POINT('Ctrl Pts',(-66.,-5.61830723712665,9.14143059178176));
#45425=CARTESIAN_POINT('Ctrl Pts',(-50.,-5.61830723712665,9.14143059178176));
#45426=CARTESIAN_POINT('Ctrl Pts',(-66.,-5.67703542746581,9.20524426521879));
#45427=CARTESIAN_POINT('Ctrl Pts',(-50.,-5.67703542746581,9.20524426521879));
#45428=CARTESIAN_POINT('Ctrl Pts',(-66.,-5.78598690780261,9.21276610214511));
#45429=CARTESIAN_POINT('Ctrl Pts',(-50.,-5.78598690780261,9.21276610214511));
#45430=CARTESIAN_POINT('Ctrl Pts',(-66.,-5.95351398409578,9.1550652704948));
#45431=CARTESIAN_POINT('Ctrl Pts',(-50.,-5.95351398409578,9.1550652704948));
#45432=CARTESIAN_POINT('Ctrl Pts',(-66.,-6.1857832706813,9.0255586111413));
#45433=CARTESIAN_POINT('Ctrl Pts',(-50.,-6.1857832706813,9.0255586111413));
#45434=CARTESIAN_POINT('Ctrl Pts',(-66.,-6.4870891147678,8.81967227800013));
#45435=CARTESIAN_POINT('Ctrl Pts',(-50.,-6.4870891147678,8.81967227800013));
#45436=CARTESIAN_POINT('Ctrl Pts',(-66.,-6.86020750749309,8.5344601927968));
#45437=CARTESIAN_POINT('Ctrl Pts',(-50.,-6.86020750749309,8.5344601927968));
#45438=CARTESIAN_POINT('Ctrl Pts',(-66.,-7.30671529340422,8.16825989491623));
#45439=CARTESIAN_POINT('Ctrl Pts',(-50.,-7.30671529340422,8.16825989491623));
#45440=CARTESIAN_POINT('Ctrl Pts',(-66.,-7.8273085045771,7.72034951863681));
#45441=CARTESIAN_POINT('Ctrl Pts',(-50.,-7.8273085045771,7.72034951863681));
#45442=CARTESIAN_POINT('Ctrl Pts',(-66.,-8.30314715005506,7.2965657688752));
#45443=CARTESIAN_POINT('Ctrl Pts',(-50.,-8.30314715005506,7.2965657688752));
#45444=CARTESIAN_POINT('Ctrl Pts',(-66.,-8.69334695511751,6.9419914678159));
#45445=CARTESIAN_POINT('Ctrl Pts',(-50.,-8.69334695511751,6.9419914678159));
#45446=CARTESIAN_POINT('Ctrl Pts',(-66.,-8.96826972520416,6.68930297706156));
#45447=CARTESIAN_POINT('Ctrl Pts',(-50.,-8.96826972520416,6.68930297706156));
#45448=CARTESIAN_POINT('Ctrl Pts',(-66.,-9.10942850298702,6.55888232467755));
#45449=CARTESIAN_POINT('Ctrl Pts',(-50.,-9.10942850298702,6.55888232467755));
#45450=CARTESIAN_POINT('',(-65.5,-5.60521455261512,9.02619492472613));
#45451=CARTESIAN_POINT('Ctrl Pts',(-66.,-5.63989399158651,8.40875857446665));
#45452=CARTESIAN_POINT('Ctrl Pts',(-65.7982417703062,-5.64698827769721,
8.64693773448211));
#45453=CARTESIAN_POINT('Ctrl Pts',(-65.6331946192802,-5.59528609755734,
8.87557312667991));
#45454=CARTESIAN_POINT('Ctrl Pts',(-65.5,-5.60521455261512,9.02619492472612));
#45455=CARTESIAN_POINT('',(-50.,-4.66907432066881,6.26377691477523));
#45456=CARTESIAN_POINT('',(-66.,-4.66907432066881,6.26377691477523));
#45457=CARTESIAN_POINT('',(-50.,-5.63989399158651,8.40875857446667));
#45458=CARTESIAN_POINT('Ctrl Pts',(-50.,-4.66907432066881,6.26377691477523));
#45459=CARTESIAN_POINT('Ctrl Pts',(-50.,-4.68258736973401,6.28328945005467));
#45460=CARTESIAN_POINT('Ctrl Pts',(-50.,-4.70979548740211,6.32219595087909));
#45461=CARTESIAN_POINT('Ctrl Pts',(-50.,-4.75115374374443,6.3801999799666));
#45462=CARTESIAN_POINT('Ctrl Pts',(-50.,-4.80739151505302,6.45682640629315));
#45463=CARTESIAN_POINT('Ctrl Pts',(-50.,-4.87940339472638,6.55149182098506));
#45464=CARTESIAN_POINT('Ctrl Pts',(-50.,-4.95278821116117,6.645260114762));
#45465=CARTESIAN_POINT('Ctrl Pts',(-50.,-5.02685611555883,6.7385766957876));
#45466=CARTESIAN_POINT('Ctrl Pts',(-50.,-5.10042834492066,6.83220206842988));
#45467=CARTESIAN_POINT('Ctrl Pts',(-50.,-5.17200306149544,6.92712124167231));
#45468=CARTESIAN_POINT('Ctrl Pts',(-50.,-5.23995252537855,7.02443775083668));
#45469=CARTESIAN_POINT('Ctrl Pts',(-50.,-5.3027072062188,7.12526883629655));
#45470=CARTESIAN_POINT('Ctrl Pts',(-50.,-5.35894790191298,7.23065348642503));
#45471=CARTESIAN_POINT('Ctrl Pts',(-50.,-5.40780718177897,7.34132172472021));
#45472=CARTESIAN_POINT('Ctrl Pts',(-50.,-5.44911325868757,7.45738867431159));
#45473=CARTESIAN_POINT('Ctrl Pts',(-50.,-5.48355669348136,7.57814301204284));
#45474=CARTESIAN_POINT('Ctrl Pts',(-50.,-5.51305921086426,7.70161357993859));
#45475=CARTESIAN_POINT('Ctrl Pts',(-50.,-5.54016188969533,7.82519591791858));
#45476=CARTESIAN_POINT('Ctrl Pts',(-50.,-5.56683712169066,7.94689743821095));
#45477=CARTESIAN_POINT('Ctrl Pts',(-50.,-5.593664068609,8.06619581758504));
#45478=CARTESIAN_POINT('Ctrl Pts',(-50.,-5.61707418533788,8.17903563336739));
#45479=CARTESIAN_POINT('Ctrl Pts',(-50.,-5.63092023716983,8.27141516094588));
#45480=CARTESIAN_POINT('Ctrl Pts',(-50.,-5.63713657156084,8.34237187934735));
#45481=CARTESIAN_POINT('Ctrl Pts',(-50.,-5.63930183311986,8.3888778135301));
#45482=CARTESIAN_POINT('Ctrl Pts',(-50.,-5.63989399158651,8.40875857446667));
#45483=CARTESIAN_POINT('',(-50.5,-5.60521455261512,9.02619492472613));
#45484=CARTESIAN_POINT('Ctrl Pts',(-50.5,-5.60521455261512,9.02619492472614));
#45485=CARTESIAN_POINT('Ctrl Pts',(-50.4982567069803,-5.60508460587634,
9.02422353931612));
#45486=CARTESIAN_POINT('Ctrl Pts',(-50.4965113438768,-5.60496484245642,
9.02224324973366));
#45487=CARTESIAN_POINT('Ctrl Pts',(-50.3581212730784,-5.59625809416611,
8.86472332078281));
#45488=CARTESIAN_POINT('Ctrl Pts',(-50.2022201285465,-5.64700451912944,
8.64748301425043));
#45489=CARTESIAN_POINT('Ctrl Pts',(-50.,-5.63989399158651,8.40875857446667));
#45490=CARTESIAN_POINT('Ctrl Pts',(-65.5,-5.60521455261512,9.02619492472613));
#45491=CARTESIAN_POINT('Ctrl Pts',(-60.5,-5.60521455261512,9.02619492472613));
#45492=CARTESIAN_POINT('Ctrl Pts',(-55.5,-5.60521455261512,9.02619492472613));
#45493=CARTESIAN_POINT('Ctrl Pts',(-50.5,-5.60521455261512,9.02619492472613));
#45494=CARTESIAN_POINT('Origin',(-66.,0.,0.));
#45495=CARTESIAN_POINT('',(-50.,-5.74141212582432,5.29823961815974));
#45496=CARTESIAN_POINT('',(-66.,-5.74141212582432,5.29823961815974));
#45497=CARTESIAN_POINT('Origin',(-50.,0.,0.));
#45498=CARTESIAN_POINT('Ctrl Pts',(-66.,-9.10942850298702,6.55888232467755));
#45499=CARTESIAN_POINT('Ctrl Pts',(-50.,-9.10942850298702,6.55888232467755));
#45500=CARTESIAN_POINT('Ctrl Pts',(-66.,-9.08576143793161,6.55992054266089));
#45501=CARTESIAN_POINT('Ctrl Pts',(-50.,-9.08576143793161,6.55992054266089));
#45502=CARTESIAN_POINT('Ctrl Pts',(-66.,-9.03849534181953,6.56179460771868));
#45503=CARTESIAN_POINT('Ctrl Pts',(-50.,-9.03849534181953,6.56179460771868));
#45504=CARTESIAN_POINT('Ctrl Pts',(-66.,-8.96780029988517,6.56399859267612));
#45505=CARTESIAN_POINT('Ctrl Pts',(-50.,-8.96780029988517,6.56399859267612));
#45506=CARTESIAN_POINT('Ctrl Pts',(-66.,-8.87394898919059,6.56572139847731));
#45507=CARTESIAN_POINT('Ctrl Pts',(-50.,-8.87394898919059,6.56572139847731));
#45508=CARTESIAN_POINT('Ctrl Pts',(-66.,-8.75732214056418,6.56583717553711));
#45509=CARTESIAN_POINT('Ctrl Pts',(-50.,-8.75732214056418,6.56583717553711));
#45510=CARTESIAN_POINT('Ctrl Pts',(-66.,-8.64139521040441,6.56389753528232));
#45511=CARTESIAN_POINT('Ctrl Pts',(-50.,-8.64139521040441,6.56389753528232));
#45512=CARTESIAN_POINT('Ctrl Pts',(-66.,-8.5261893930021,6.55987949669048));
#45513=CARTESIAN_POINT('Ctrl Pts',(-50.,-8.5261893930021,6.55987949669048));
#45514=CARTESIAN_POINT('Ctrl Pts',(-66.,-8.41173611627071,6.55375602860952));
#45515=CARTESIAN_POINT('Ctrl Pts',(-50.,-8.41173611627071,6.55375602860952));
#45516=CARTESIAN_POINT('Ctrl Pts',(-66.,-8.29807942911973,6.54549737862328));
#45517=CARTESIAN_POINT('Ctrl Pts',(-50.,-8.29807942911973,6.54549737862328));
#45518=CARTESIAN_POINT('Ctrl Pts',(-66.,-8.18527357628522,6.53507290801895));
#45519=CARTESIAN_POINT('Ctrl Pts',(-50.,-8.18527357628522,6.53507290801895));
#45520=CARTESIAN_POINT('Ctrl Pts',(-66.,-8.07337944645762,6.52245299848617));
#45521=CARTESIAN_POINT('Ctrl Pts',(-50.,-8.07337944645762,6.52245299848617));
#45522=CARTESIAN_POINT('Ctrl Pts',(-66.,-7.96246113297438,6.50761151737996));
#45523=CARTESIAN_POINT('Ctrl Pts',(-50.,-7.96246113297438,6.50761151737996));
#45524=CARTESIAN_POINT('Ctrl Pts',(-66.,-7.85258285330582,6.49052756009744));
#45525=CARTESIAN_POINT('Ctrl Pts',(-50.,-7.85258285330582,6.49052756009744));
#45526=CARTESIAN_POINT('Ctrl Pts',(-66.,-7.74380437584162,6.47118971339301));
#45527=CARTESIAN_POINT('Ctrl Pts',(-50.,-7.74380437584162,6.47118971339301));
#45528=CARTESIAN_POINT('Ctrl Pts',(-66.,-7.63618323735142,6.44958986632227));
#45529=CARTESIAN_POINT('Ctrl Pts',(-50.,-7.63618323735142,6.44958986632227));
#45530=CARTESIAN_POINT('Ctrl Pts',(-66.,-7.52978062910616,6.42571181012752));
#45531=CARTESIAN_POINT('Ctrl Pts',(-50.,-7.52978062910616,6.42571181012752));
#45532=CARTESIAN_POINT('Ctrl Pts',(-66.,-7.42466575500371,6.39952147476842));
#45533=CARTESIAN_POINT('Ctrl Pts',(-50.,-7.42466575500371,6.39952147476842));
#45534=CARTESIAN_POINT('Ctrl Pts',(-66.,-7.3209213165869,6.37095713183339));
#45535=CARTESIAN_POINT('Ctrl Pts',(-50.,-7.3209213165869,6.37095713183339));
#45536=CARTESIAN_POINT('Ctrl Pts',(-66.,-7.21864696410326,6.33991858248025));
#45537=CARTESIAN_POINT('Ctrl Pts',(-50.,-7.21864696410326,6.33991858248025));
#45538=CARTESIAN_POINT('Ctrl Pts',(-66.,-7.11796972459708,6.30626252916358));
#45539=CARTESIAN_POINT('Ctrl Pts',(-50.,-7.11796972459708,6.30626252916358));
#45540=CARTESIAN_POINT('Ctrl Pts',(-66.,-7.01905715111184,6.26980372166142));
#45541=CARTESIAN_POINT('Ctrl Pts',(-50.,-7.01905715111184,6.26980372166142));
#45542=CARTESIAN_POINT('Ctrl Pts',(-66.,-6.92213264398368,6.23031211373657));
#45543=CARTESIAN_POINT('Ctrl Pts',(-50.,-6.92213264398368,6.23031211373657));
#45544=CARTESIAN_POINT('Ctrl Pts',(-66.,-6.82748343979352,6.18751687615083));
#45545=CARTESIAN_POINT('Ctrl Pts',(-50.,-6.82748343979352,6.18751687615083));
#45546=CARTESIAN_POINT('Ctrl Pts',(-66.,-6.73548810524172,6.14109480995689));
#45547=CARTESIAN_POINT('Ctrl Pts',(-50.,-6.73548810524172,6.14109480995689));
#45548=CARTESIAN_POINT('Ctrl Pts',(-66.,-6.64656015751461,6.09072492635055));
#45549=CARTESIAN_POINT('Ctrl Pts',(-50.,-6.64656015751461,6.09072492635055));
#45550=CARTESIAN_POINT('Ctrl Pts',(-66.,-6.56104388578368,6.03618002486629));
#45551=CARTESIAN_POINT('Ctrl Pts',(-50.,-6.56104388578368,6.03618002486629));
#45552=CARTESIAN_POINT('Ctrl Pts',(-66.,-6.47911851546308,5.97741330588777));
#45553=CARTESIAN_POINT('Ctrl Pts',(-50.,-6.47911851546308,5.97741330588777));
#45554=CARTESIAN_POINT('Ctrl Pts',(-66.,-6.4007102042632,5.91463628394544));
#45555=CARTESIAN_POINT('Ctrl Pts',(-50.,-6.4007102042632,5.91463628394544));
#45556=CARTESIAN_POINT('Ctrl Pts',(-66.,-6.32536729565295,5.8484330883917));
#45557=CARTESIAN_POINT('Ctrl Pts',(-50.,-6.32536729565295,5.8484330883917));
#45558=CARTESIAN_POINT('Ctrl Pts',(-66.,-6.25233913230877,5.77967659171849));
#45559=CARTESIAN_POINT('Ctrl Pts',(-50.,-6.25233913230877,5.77967659171849));
#45560=CARTESIAN_POINT('Ctrl Pts',(-66.,-6.18072779481142,5.70937384347389));
#45561=CARTESIAN_POINT('Ctrl Pts',(-50.,-6.18072779481142,5.70937384347389));
#45562=CARTESIAN_POINT('Ctrl Pts',(-66.,-6.10961745579836,5.63853298297221));
#45563=CARTESIAN_POINT('Ctrl Pts',(-50.,-6.10961745579836,5.63853298297221));
#45564=CARTESIAN_POINT('Ctrl Pts',(-66.,-6.03820626716823,5.56802821638893));
#45565=CARTESIAN_POINT('Ctrl Pts',(-50.,-6.03820626716823,5.56802821638893));
#45566=CARTESIAN_POINT('Ctrl Pts',(-66.,-5.96595410170651,5.49844782238954));
#45567=CARTESIAN_POINT('Ctrl Pts',(-50.,-5.96595410170651,5.49844782238954));
#45568=CARTESIAN_POINT('Ctrl Pts',(-66.,-5.89254591434388,5.43013507033993));
#45569=CARTESIAN_POINT('Ctrl Pts',(-50.,-5.89254591434388,5.43013507033993));
#45570=CARTESIAN_POINT('Ctrl Pts',(-66.,-5.8327710073448,5.37663351860743));
#45571=CARTESIAN_POINT('Ctrl Pts',(-50.,-5.8327710073448,5.37663351860743));
#45572=CARTESIAN_POINT('Ctrl Pts',(-66.,-5.78732886917933,5.33717661990139));
#45573=CARTESIAN_POINT('Ctrl Pts',(-50.,-5.78732886917933,5.33717661990139));
#45574=CARTESIAN_POINT('Ctrl Pts',(-66.,-5.75676290651676,5.31116910570307));
#45575=CARTESIAN_POINT('Ctrl Pts',(-50.,-5.75676290651676,5.31116910570307));
#45576=CARTESIAN_POINT('Ctrl Pts',(-66.,-5.74141212582432,5.29823961815974));
#45577=CARTESIAN_POINT('Ctrl Pts',(-50.,-5.74141212582432,5.29823961815974));
#45578=CARTESIAN_POINT('Ctrl Pts',(-50.,-7.78178935653717,6.47760599376692));
#45579=CARTESIAN_POINT('Ctrl Pts',(-50.,-7.77423639474705,6.47623696517724));
#45580=CARTESIAN_POINT('Ctrl Pts',(-50.,-7.74499129323442,6.47087829659421));
#45581=CARTESIAN_POINT('Ctrl Pts',(-50.,-7.69422820821259,6.46118598421581));
#45582=CARTESIAN_POINT('Ctrl Pts',(-50.,-7.62230326232111,6.44647502892099));
#45583=CARTESIAN_POINT('Ctrl Pts',(-50.,-7.52978062910616,6.42571181012752));
#45584=CARTESIAN_POINT('Ctrl Pts',(-50.,-7.42466575500371,6.39952147476842));
#45585=CARTESIAN_POINT('Ctrl Pts',(-50.,-7.3209213165869,6.37095713183339));
#45586=CARTESIAN_POINT('Ctrl Pts',(-50.,-7.21864696410326,6.33991858248025));
#45587=CARTESIAN_POINT('Ctrl Pts',(-50.,-7.11796972459708,6.30626252916358));
#45588=CARTESIAN_POINT('Ctrl Pts',(-50.,-7.01905715111184,6.26980372166142));
#45589=CARTESIAN_POINT('Ctrl Pts',(-50.,-6.92213264398368,6.23031211373657));
#45590=CARTESIAN_POINT('Ctrl Pts',(-50.,-6.82748343979352,6.18751687615083));
#45591=CARTESIAN_POINT('Ctrl Pts',(-50.,-6.73548810524172,6.14109480995689));
#45592=CARTESIAN_POINT('Ctrl Pts',(-50.,-6.64656015751461,6.09072492635055));
#45593=CARTESIAN_POINT('Ctrl Pts',(-50.,-6.56104388578368,6.03618002486629));
#45594=CARTESIAN_POINT('Ctrl Pts',(-50.,-6.47911851546308,5.97741330588777));
#45595=CARTESIAN_POINT('Ctrl Pts',(-50.,-6.4007102042632,5.91463628394544));
#45596=CARTESIAN_POINT('Ctrl Pts',(-50.,-6.32536729565295,5.8484330883917));
#45597=CARTESIAN_POINT('Ctrl Pts',(-50.,-6.25233913230877,5.77967659171849));
#45598=CARTESIAN_POINT('Ctrl Pts',(-50.,-6.18072779481142,5.70937384347389));
#45599=CARTESIAN_POINT('Ctrl Pts',(-50.,-6.10961745579836,5.63853298297221));
#45600=CARTESIAN_POINT('Ctrl Pts',(-50.,-6.03820626716823,5.56802821638893));
#45601=CARTESIAN_POINT('Ctrl Pts',(-50.,-5.96595410170651,5.49844782238954));
#45602=CARTESIAN_POINT('Ctrl Pts',(-50.,-5.89254591434388,5.43013507033993));
#45603=CARTESIAN_POINT('Ctrl Pts',(-50.,-5.8327710073448,5.37663351860743));
#45604=CARTESIAN_POINT('Ctrl Pts',(-50.,-5.78732886917933,5.33717661990139));
#45605=CARTESIAN_POINT('Ctrl Pts',(-50.,-5.75676290651676,5.31116910570307));
#45606=CARTESIAN_POINT('Ctrl Pts',(-50.,-5.74141212582432,5.29823961815974));
#45607=CARTESIAN_POINT('Origin',(-50.,-6.71577615516547,6.72762868007336));
#45608=CARTESIAN_POINT('Origin',(-50.,0.,0.));
#45609=CARTESIAN_POINT('Origin',(-65.75,0.,0.));
#45610=CARTESIAN_POINT('',(-65.5,-4.97834853060433,9.38651537621016));
#45611=CARTESIAN_POINT('Origin',(-65.5,0.,0.));
#45612=CARTESIAN_POINT('',(-66.,-4.47433860192361,9.08272641200517));
#45613=CARTESIAN_POINT('Ctrl Pts',(-65.5,-4.97834853060432,9.38651537621016));
#45614=CARTESIAN_POINT('Ctrl Pts',(-65.664291736,-4.80345165052451,9.29330697735479));
#45615=CARTESIAN_POINT('Ctrl Pts',(-65.831118235484,-4.63468361464914,9.19199866580212));
#45616=CARTESIAN_POINT('Ctrl Pts',(-66.,-4.47433860192361,9.08272641200516));
#45617=CARTESIAN_POINT('Origin',(-66.,0.,0.));
#45618=CARTESIAN_POINT('Origin',(-58.,0.,0.));
#45619=CARTESIAN_POINT('',(-50.5,-4.97834853060433,9.38651537621016));
#45620=CARTESIAN_POINT('Origin',(-50.5,0.,0.));
#45621=CARTESIAN_POINT('Ctrl Pts',(-50.5,-4.97834853060433,9.38651537621016));
#45622=CARTESIAN_POINT('Ctrl Pts',(-55.5,-4.97834853060433,9.38651537621016));
#45623=CARTESIAN_POINT('Ctrl Pts',(-60.5,-4.97834853060433,9.38651537621016));
#45624=CARTESIAN_POINT('Ctrl Pts',(-65.5,-4.97834853060433,9.38651537621016));
#45625=CARTESIAN_POINT('Origin',(-50.25,0.,0.));
#45626=CARTESIAN_POINT('',(-50.,-4.47433860192363,9.08272641200518));
#45627=CARTESIAN_POINT('Origin',(-50.,0.,0.));
#45628=CARTESIAN_POINT('Ctrl Pts',(-50.,-4.47433860192363,9.08272641200517));
#45629=CARTESIAN_POINT('Ctrl Pts',(-50.1688817645162,-4.6346836146493,9.19199866580223));
#45630=CARTESIAN_POINT('Ctrl Pts',(-50.3357082640001,-4.80345165052468,
9.29330697735489));
#45631=CARTESIAN_POINT('Ctrl Pts',(-50.5,-4.97834853060434,9.38651537621016));
#45632=CARTESIAN_POINT('Origin',(-66.,-3.39879369590239,8.87754687038761));
#45633=CARTESIAN_POINT('',(-66.,-1.73214930258623,9.97573474955855));
#45634=CARTESIAN_POINT('Origin',(-66.,0.,0.));
#45635=CARTESIAN_POINT('',(-66.,-3.09005277149945,7.17542543124438));
#45636=CARTESIAN_POINT('Ctrl Pts',(-66.,-3.09005277149946,7.17542543124437));
#45637=CARTESIAN_POINT('Ctrl Pts',(-66.,-3.09881751111224,7.19348083086667));
#45638=CARTESIAN_POINT('Ctrl Pts',(-66.,-3.11616269844133,7.22967217437288));
#45639=CARTESIAN_POINT('Ctrl Pts',(-66.,-3.14162759082209,7.28420082769005));
#45640=CARTESIAN_POINT('Ctrl Pts',(-66.,-3.17447364404108,7.35738957226508));
#45641=CARTESIAN_POINT('Ctrl Pts',(-66.,-3.21375006071206,7.44965417630122));
#45642=CARTESIAN_POINT('Ctrl Pts',(-66.,-3.25145480239525,7.5426066324152));
#45643=CARTESIAN_POINT('Ctrl Pts',(-66.,-3.28801529731225,7.63606148881098));
#45644=CARTESIAN_POINT('Ctrl Pts',(-66.,-3.32416425071599,7.72970101571594));
#45645=CARTESIAN_POINT('Ctrl Pts',(-66.,-3.3609897589824,7.82305272705443));
#45646=CARTESIAN_POINT('Ctrl Pts',(-66.,-3.39973851923894,7.91556814228226));
#45647=CARTESIAN_POINT('Ctrl Pts',(-66.,-3.441640425645,8.00669249258951));
#45648=CARTESIAN_POINT('Ctrl Pts',(-66.,-3.48773626701595,8.09593368911593));
#45649=CARTESIAN_POINT('Ctrl Pts',(-66.,-3.53867623893612,8.18294180840626));
#45650=CARTESIAN_POINT('Ctrl Pts',(-66.,-3.59461383040384,8.26755365668696));
#45651=CARTESIAN_POINT('Ctrl Pts',(-66.,-3.65536627573726,8.34973908999167));
#45652=CARTESIAN_POINT('Ctrl Pts',(-66.,-3.720526640373,8.42956563125176));
#45653=CARTESIAN_POINT('Ctrl Pts',(-66.,-3.78958659965516,8.50715832573905));
#45654=CARTESIAN_POINT('Ctrl Pts',(-66.,-3.86206885883931,8.58265845343488));
#45655=CARTESIAN_POINT('Ctrl Pts',(-66.,-3.93760085807652,8.65619659951692));
#45656=CARTESIAN_POINT('Ctrl Pts',(-66.,-4.01588494277018,8.72789205657743));
#45657=CARTESIAN_POINT('Ctrl Pts',(-66.,-4.09669269754511,8.79784590915275));
#45658=CARTESIAN_POINT('Ctrl Pts',(-66.,-4.17984979305941,8.86613739951103));
#45659=CARTESIAN_POINT('Ctrl Pts',(-66.,-4.26522443974139,8.93281753244224));
#45660=CARTESIAN_POINT('Ctrl Pts',(-66.,-4.34130290913253,8.98941802189943));
#45661=CARTESIAN_POINT('Ctrl Pts',(-66.,-4.40102613216983,9.03211165933191));
#45662=CARTESIAN_POINT('Ctrl Pts',(-66.,-4.443458299307,9.06161323407319));
#45663=CARTESIAN_POINT('Ctrl Pts',(-66.,-4.46799546208135,9.07840367583189));
#45664=CARTESIAN_POINT('Ctrl Pts',(-66.,-4.47433860192361,9.08272641200517));
#45665=CARTESIAN_POINT('',(-66.,-1.71770404175133,7.62132856363975));
#45666=CARTESIAN_POINT('Origin',(-66.,0.,0.));
#45667=CARTESIAN_POINT('Ctrl Pts',(-66.,-1.73214930258623,9.97573474955855));
#45668=CARTESIAN_POINT('Ctrl Pts',(-66.,-1.73969457287395,9.95733191816358));
#45669=CARTESIAN_POINT('Ctrl Pts',(-66.,-1.7566321755647,9.9139659420196));
#45670=CARTESIAN_POINT('Ctrl Pts',(-66.,-1.77981396896489,9.84661534325229));
#45671=CARTESIAN_POINT('Ctrl Pts',(-66.,-1.80473911014373,9.75659074881182));
#45672=CARTESIAN_POINT('Ctrl Pts',(-66.,-1.82924899221979,9.6439846953703));
#45673=CARTESIAN_POINT('Ctrl Pts',(-66.,-1.85326437907112,9.52408870045544));
#45674=CARTESIAN_POINT('Ctrl Pts',(-66.,-1.87839580987116,9.40205903508911));
#45675=CARTESIAN_POINT('Ctrl Pts',(-66.,-1.90390174602853,9.27813729897652));
#45676=CARTESIAN_POINT('Ctrl Pts',(-66.,-1.92716985958894,9.15334156764019));
#45677=CARTESIAN_POINT('Ctrl Pts',(-66.,-1.94481943015312,9.02901758387114));
#45678=CARTESIAN_POINT('Ctrl Pts',(-66.,-1.95429313266907,8.90618445422908));
#45679=CARTESIAN_POINT('Ctrl Pts',(-66.,-1.9546707872231,8.78521112835341));
#45680=CARTESIAN_POINT('Ctrl Pts',(-66.,-1.946156153962,8.66606230815238));
#45681=CARTESIAN_POINT('Ctrl Pts',(-66.,-1.92983859755222,8.54842389981909));
#45682=CARTESIAN_POINT('Ctrl Pts',(-66.,-1.90734586372592,8.43188330807973));
#45683=CARTESIAN_POINT('Ctrl Pts',(-66.,-1.88056621240513,8.31605826857219));
#45684=CARTESIAN_POINT('Ctrl Pts',(-66.,-1.85143550623823,8.20060271308051));
#45685=CARTESIAN_POINT('Ctrl Pts',(-66.,-1.82172638152831,8.08522764356747));
#45686=CARTESIAN_POINT('Ctrl Pts',(-66.,-1.79282501685215,7.96971775082723));
#45687=CARTESIAN_POINT('Ctrl Pts',(-66.,-1.76554278426741,7.85394672103966));
#45688=CARTESIAN_POINT('Ctrl Pts',(-66.,-1.74533379915545,7.76107103501753));
#45689=CARTESIAN_POINT('Ctrl Pts',(-66.,-1.73114351601384,7.69125979937153));
#45690=CARTESIAN_POINT('Ctrl Pts',(-66.,-1.72211236324629,7.64465040382587));
#45691=CARTESIAN_POINT('Ctrl Pts',(-66.,-1.71770404175133,7.62132856363975));
#45692=CARTESIAN_POINT('Ctrl Pts',(-66.,-1.71770404175133,7.62132856363975));
#45693=CARTESIAN_POINT('Ctrl Pts',(-50.,-1.71770404175133,7.62132856363975));
#45694=CARTESIAN_POINT('Ctrl Pts',(-66.,-1.72211236324629,7.64465040382587));
#45695=CARTESIAN_POINT('Ctrl Pts',(-50.,-1.72211236324629,7.64465040382587));
#45696=CARTESIAN_POINT('Ctrl Pts',(-66.,-1.73114351601384,7.69125979937153));
#45697=CARTESIAN_POINT('Ctrl Pts',(-50.,-1.73114351601384,7.69125979937153));
#45698=CARTESIAN_POINT('Ctrl Pts',(-66.,-1.74533379915545,7.76107103501753));
#45699=CARTESIAN_POINT('Ctrl Pts',(-50.,-1.74533379915545,7.76107103501753));
#45700=CARTESIAN_POINT('Ctrl Pts',(-66.,-1.76554278426741,7.85394672103966));
#45701=CARTESIAN_POINT('Ctrl Pts',(-50.,-1.76554278426741,7.85394672103966));
#45702=CARTESIAN_POINT('Ctrl Pts',(-66.,-1.79282501685215,7.96971775082723));
#45703=CARTESIAN_POINT('Ctrl Pts',(-50.,-1.79282501685215,7.96971775082723));
#45704=CARTESIAN_POINT('Ctrl Pts',(-66.,-1.82172638152831,8.08522764356747));
#45705=CARTESIAN_POINT('Ctrl Pts',(-50.,-1.82172638152831,8.08522764356747));
#45706=CARTESIAN_POINT('Ctrl Pts',(-66.,-1.85143550623823,8.20060271308051));
#45707=CARTESIAN_POINT('Ctrl Pts',(-50.,-1.85143550623823,8.20060271308051));
#45708=CARTESIAN_POINT('Ctrl Pts',(-66.,-1.88056621240513,8.31605826857219));
#45709=CARTESIAN_POINT('Ctrl Pts',(-50.,-1.88056621240513,8.31605826857219));
#45710=CARTESIAN_POINT('Ctrl Pts',(-66.,-1.90734586372592,8.43188330807973));
#45711=CARTESIAN_POINT('Ctrl Pts',(-50.,-1.90734586372592,8.43188330807973));
#45712=CARTESIAN_POINT('Ctrl Pts',(-66.,-1.92983859755222,8.54842389981909));
#45713=CARTESIAN_POINT('Ctrl Pts',(-50.,-1.92983859755222,8.54842389981909));
#45714=CARTESIAN_POINT('Ctrl Pts',(-66.,-1.946156153962,8.66606230815238));
#45715=CARTESIAN_POINT('Ctrl Pts',(-50.,-1.946156153962,8.66606230815238));
#45716=CARTESIAN_POINT('Ctrl Pts',(-66.,-1.9546707872231,8.78521112835341));
#45717=CARTESIAN_POINT('Ctrl Pts',(-50.,-1.9546707872231,8.78521112835341));
#45718=CARTESIAN_POINT('Ctrl Pts',(-66.,-1.95429313266907,8.90618445422908));
#45719=CARTESIAN_POINT('Ctrl Pts',(-50.,-1.95429313266907,8.90618445422908));
#45720=CARTESIAN_POINT('Ctrl Pts',(-66.,-1.94481943015312,9.02901758387114));
#45721=CARTESIAN_POINT('Ctrl Pts',(-50.,-1.94481943015312,9.02901758387114));
#45722=CARTESIAN_POINT('Ctrl Pts',(-66.,-1.92716985958894,9.15334156764019));
#45723=CARTESIAN_POINT('Ctrl Pts',(-50.,-1.92716985958894,9.15334156764019));
#45724=CARTESIAN_POINT('Ctrl Pts',(-66.,-1.90390174602853,9.27813729897652));
#45725=CARTESIAN_POINT('Ctrl Pts',(-50.,-1.90390174602853,9.27813729897652));
#45726=CARTESIAN_POINT('Ctrl Pts',(-66.,-1.87839580987116,9.40205903508911));
#45727=CARTESIAN_POINT('Ctrl Pts',(-50.,-1.87839580987116,9.40205903508911));
#45728=CARTESIAN_POINT('Ctrl Pts',(-66.,-1.85326437907112,9.52408870045544));
#45729=CARTESIAN_POINT('Ctrl Pts',(-50.,-1.85326437907112,9.52408870045544));
#45730=CARTESIAN_POINT('Ctrl Pts',(-66.,-1.82924899221979,9.6439846953703));
#45731=CARTESIAN_POINT('Ctrl Pts',(-50.,-1.82924899221979,9.6439846953703));
#45732=CARTESIAN_POINT('Ctrl Pts',(-66.,-1.8033312375021,9.76305895544906));
#45733=CARTESIAN_POINT('Ctrl Pts',(-50.,-1.8033312375021,9.76305895544906));
#45734=CARTESIAN_POINT('Ctrl Pts',(-66.,-1.76935818428543,9.88390776205071));
#45735=CARTESIAN_POINT('Ctrl Pts',(-50.,-1.76935818428543,9.88390776205071));
#45736=CARTESIAN_POINT('Ctrl Pts',(-66.,-1.72158810581393,10.0089274070765));
#45737=CARTESIAN_POINT('Ctrl Pts',(-50.,-1.72158810581393,10.0089274070765));
#45738=CARTESIAN_POINT('Ctrl Pts',(-66.,-1.65730460746568,10.1392183674146));
#45739=CARTESIAN_POINT('Ctrl Pts',(-50.,-1.65730460746568,10.1392183674146));
#45740=CARTESIAN_POINT('Ctrl Pts',(-66.,-1.58020220545128,10.2731661881148));
#45741=CARTESIAN_POINT('Ctrl Pts',(-50.,-1.58020220545128,10.2731661881148));
#45742=CARTESIAN_POINT('Ctrl Pts',(-66.,-1.5023358317684,10.4056266289389));
#45743=CARTESIAN_POINT('Ctrl Pts',(-50.,-1.5023358317684,10.4056266289389));
#45744=CARTESIAN_POINT('Ctrl Pts',(-66.,-1.44067870129829,10.5293819191661));
#45745=CARTESIAN_POINT('Ctrl Pts',(-50.,-1.44067870129829,10.5293819191661));
#45746=CARTESIAN_POINT('Ctrl Pts',(-66.,-1.41442426430587,10.6362838188747));
#45747=CARTESIAN_POINT('Ctrl Pts',(-50.,-1.41442426430587,10.6362838188747));
#45748=CARTESIAN_POINT('Ctrl Pts',(-66.,-1.44211977650966,10.7184674173711));
#45749=CARTESIAN_POINT('Ctrl Pts',(-50.,-1.44211977650966,10.7184674173711));
#45750=CARTESIAN_POINT('Ctrl Pts',(-66.,-1.53859249977361,10.7696535166986));
#45751=CARTESIAN_POINT('Ctrl Pts',(-50.,-1.53859249977361,10.7696535166986));
#45752=CARTESIAN_POINT('Ctrl Pts',(-66.,-1.71510514192151,10.785080584678));
#45753=CARTESIAN_POINT('Ctrl Pts',(-50.,-1.71510514192151,10.785080584678));
#45754=CARTESIAN_POINT('Ctrl Pts',(-66.,-1.979968797513,10.7612427942066));
#45755=CARTESIAN_POINT('Ctrl Pts',(-50.,-1.979968797513,10.7612427942066));
#45756=CARTESIAN_POINT('Ctrl Pts',(-66.,-2.33896689873642,10.6957083973376));
#45757=CARTESIAN_POINT('Ctrl Pts',(-50.,-2.33896689873642,10.6957083973376));
#45758=CARTESIAN_POINT('Ctrl Pts',(-66.,-2.79583371767377,10.5869151149623));
#45759=CARTESIAN_POINT('Ctrl Pts',(-50.,-2.79583371767377,10.5869151149623));
#45760=CARTESIAN_POINT('Ctrl Pts',(-66.,-3.35268595714823,10.4339855741948));
#45761=CARTESIAN_POINT('Ctrl Pts',(-50.,-3.35268595714823,10.4339855741948));
#45762=CARTESIAN_POINT('Ctrl Pts',(-66.,-4.0104530833415,10.2365434196342));
#45763=CARTESIAN_POINT('Ctrl Pts',(-50.,-4.0104530833415,10.2365434196342));
#45764=CARTESIAN_POINT('Ctrl Pts',(-66.,-4.61752169625681,10.0429387133242));
#45765=CARTESIAN_POINT('Ctrl Pts',(-50.,-4.61752169625681,10.0429387133242));
#45766=CARTESIAN_POINT('Ctrl Pts',(-66.,-5.11820531667845,9.87772753003463));
#45767=CARTESIAN_POINT('Ctrl Pts',(-50.,-5.11820531667845,9.87772753003463));
#45768=CARTESIAN_POINT('Ctrl Pts',(-66.,-5.47213743296694,9.75870627171758));
#45769=CARTESIAN_POINT('Ctrl Pts',(-50.,-5.47213743296694,9.75870627171758));
#45770=CARTESIAN_POINT('Ctrl Pts',(-66.,-5.65413925155529,9.69697552456547));
#45771=CARTESIAN_POINT('Ctrl Pts',(-50.,-5.65413925155529,9.69697552456547));
#45772=CARTESIAN_POINT('',(-65.5,-1.44933407022281,10.5256855241305));
#45773=CARTESIAN_POINT('Ctrl Pts',(-66.,-1.73214930258624,9.97573474955854));
#45774=CARTESIAN_POINT('Ctrl Pts',(-65.798241770306,-1.64175406344253,10.1962077454137));
#45775=CARTESIAN_POINT('Ctrl Pts',(-65.6331946192802,-1.50152737971468,
10.3840473982224));
#45776=CARTESIAN_POINT('Ctrl Pts',(-65.5,-1.44933407022282,10.5256855241305));
#45777=CARTESIAN_POINT('',(-50.,-1.71770404175133,7.62132856363975));
#45778=CARTESIAN_POINT('',(-66.,-1.71770404175133,7.62132856363975));
#45779=CARTESIAN_POINT('',(-50.,-1.73214930258623,9.97573474955857));
#45780=CARTESIAN_POINT('Ctrl Pts',(-50.,-1.71770404175133,7.62132856363975));
#45781=CARTESIAN_POINT('Ctrl Pts',(-50.,-1.72211236324629,7.64465040382587));
#45782=CARTESIAN_POINT('Ctrl Pts',(-50.,-1.73114351601384,7.69125979937153));
#45783=CARTESIAN_POINT('Ctrl Pts',(-50.,-1.74533379915545,7.76107103501753));
#45784=CARTESIAN_POINT('Ctrl Pts',(-50.,-1.76554278426741,7.85394672103966));
#45785=CARTESIAN_POINT('Ctrl Pts',(-50.,-1.79282501685215,7.96971775082723));
#45786=CARTESIAN_POINT('Ctrl Pts',(-50.,-1.82172638152831,8.08522764356747));
#45787=CARTESIAN_POINT('Ctrl Pts',(-50.,-1.85143550623823,8.20060271308051));
#45788=CARTESIAN_POINT('Ctrl Pts',(-50.,-1.88056621240513,8.31605826857219));
#45789=CARTESIAN_POINT('Ctrl Pts',(-50.,-1.90734586372592,8.43188330807973));
#45790=CARTESIAN_POINT('Ctrl Pts',(-50.,-1.92983859755222,8.54842389981909));
#45791=CARTESIAN_POINT('Ctrl Pts',(-50.,-1.946156153962,8.66606230815238));
#45792=CARTESIAN_POINT('Ctrl Pts',(-50.,-1.9546707872231,8.78521112835341));
#45793=CARTESIAN_POINT('Ctrl Pts',(-50.,-1.95429313266907,8.90618445422908));
#45794=CARTESIAN_POINT('Ctrl Pts',(-50.,-1.94481943015312,9.02901758387114));
#45795=CARTESIAN_POINT('Ctrl Pts',(-50.,-1.92716985958894,9.15334156764019));
#45796=CARTESIAN_POINT('Ctrl Pts',(-50.,-1.90390174602853,9.27813729897652));
#45797=CARTESIAN_POINT('Ctrl Pts',(-50.,-1.87839580987116,9.40205903508911));
#45798=CARTESIAN_POINT('Ctrl Pts',(-50.,-1.85326437907112,9.52408870045544));
#45799=CARTESIAN_POINT('Ctrl Pts',(-50.,-1.82924899221979,9.6439846953703));
#45800=CARTESIAN_POINT('Ctrl Pts',(-50.,-1.80473911014373,9.75659074881182));
#45801=CARTESIAN_POINT('Ctrl Pts',(-50.,-1.77981396896489,9.84661534325229));
#45802=CARTESIAN_POINT('Ctrl Pts',(-50.,-1.7566321755647,9.91396594201961));
#45803=CARTESIAN_POINT('Ctrl Pts',(-50.,-1.73969457287395,9.95733191816359));
#45804=CARTESIAN_POINT('Ctrl Pts',(-50.,-1.73214930258623,9.97573474955856));
#45805=CARTESIAN_POINT('',(-50.5,-1.44933407022281,10.5256855241305));
#45806=CARTESIAN_POINT('Ctrl Pts',(-50.5,-1.44933407022281,10.5256855241306));
#45807=CARTESIAN_POINT('Ctrl Pts',(-50.4982567069801,-1.45001719265382,
10.5238317198435));
#45808=CARTESIAN_POINT('Ctrl Pts',(-50.4965113438764,-1.45071323966274,
10.521973923119));
#45809=CARTESIAN_POINT('Ctrl Pts',(-50.3581212730779,-1.50682835643054,
10.3745309539659));
#45810=CARTESIAN_POINT('Ctrl Pts',(-50.2022201285462,-1.64154711546685,
10.1967124892543));
#45811=CARTESIAN_POINT('Ctrl Pts',(-50.,-1.73214930258623,9.97573474955857));
#45812=CARTESIAN_POINT('Ctrl Pts',(-65.5,-1.44933407022281,10.5256855241305));
#45813=CARTESIAN_POINT('Ctrl Pts',(-60.5,-1.44933407022281,10.5256855241305));
#45814=CARTESIAN_POINT('Ctrl Pts',(-55.5,-1.44933407022281,10.5256855241305));
#45815=CARTESIAN_POINT('Ctrl Pts',(-50.5,-1.44933407022281,10.5256855241305));
#45816=CARTESIAN_POINT('Origin',(-66.,0.,0.));
#45817=CARTESIAN_POINT('',(-50.,-3.09005277149945,7.17542543124438));
#45818=CARTESIAN_POINT('',(-66.,-3.09005277149945,7.17542543124438));
#45819=CARTESIAN_POINT('Origin',(-50.,0.,0.));
#45820=CARTESIAN_POINT('Ctrl Pts',(-66.,-5.65413925155529,9.69697552456547));
#45821=CARTESIAN_POINT('Ctrl Pts',(-50.,-5.65413925155529,9.69697552456547));
#45822=CARTESIAN_POINT('Ctrl Pts',(-66.,-5.63209603048086,9.68829772129611));
#45823=CARTESIAN_POINT('Ctrl Pts',(-50.,-5.63209603048086,9.68829772129611));
#45824=CARTESIAN_POINT('Ctrl Pts',(-66.,-5.58815405214666,9.67078491165305));
#45825=CARTESIAN_POINT('Ctrl Pts',(-50.,-5.58815405214666,9.67078491165305));
#45826=CARTESIAN_POINT('Ctrl Pts',(-66.,-5.5226744762667,9.64404408806114));
#45827=CARTESIAN_POINT('Ctrl Pts',(-50.,-5.5226744762667,9.64404408806114));
#45828=CARTESIAN_POINT('Ctrl Pts',(-66.,-5.4362363094396,9.60744518241504));
#45829=CARTESIAN_POINT('Ctrl Pts',(-50.,-5.4362363094396,9.60744518241504));
#45830=CARTESIAN_POINT('Ctrl Pts',(-66.,-5.32964529086513,9.56011453711931));
#45831=CARTESIAN_POINT('Ctrl Pts',(-50.,-5.32964529086513,9.56011453711931));
#45832=CARTESIAN_POINT('Ctrl Pts',(-66.,-5.22452969316523,9.51119085715981));
#45833=CARTESIAN_POINT('Ctrl Pts',(-50.,-5.22452969316523,9.51119085715981));
#45834=CARTESIAN_POINT('Ctrl Pts',(-66.,-5.12091822551194,9.46066176882258));
#45835=CARTESIAN_POINT('Ctrl Pts',(-50.,-5.12091822551194,9.46066176882258));
#45836=CARTESIAN_POINT('Ctrl Pts',(-66.,-5.01885059329289,9.40851536080546));
#45837=CARTESIAN_POINT('Ctrl Pts',(-50.,-5.01885059329289,9.40851536080546));
#45838=CARTESIAN_POINT('Ctrl Pts',(-66.,-4.91837913858716,9.35474236922936));
#45839=CARTESIAN_POINT('Ctrl Pts',(-50.,-4.91837913858716,9.35474236922936));
#45840=CARTESIAN_POINT('Ctrl Pts',(-66.,-4.81956587831414,9.29933686755924));
#45841=CARTESIAN_POINT('Ctrl Pts',(-50.,-4.81956587831414,9.29933686755924));
#45842=CARTESIAN_POINT('Ctrl Pts',(-66.,-4.72247848391254,9.24229656378374));
#45843=CARTESIAN_POINT('Ctrl Pts',(-50.,-4.72247848391254,9.24229656378374));
#45844=CARTESIAN_POINT('Ctrl Pts',(-66.,-4.62718613666396,9.18362365365267));
#45845=CARTESIAN_POINT('Ctrl Pts',(-50.,-4.62718613666396,9.18362365365267));
#45846=CARTESIAN_POINT('Ctrl Pts',(-66.,-4.53375600481471,9.12332515945933));
#45847=CARTESIAN_POINT('Ctrl Pts',(-50.,-4.53375600481471,9.12332515945933));
#45848=CARTESIAN_POINT('Ctrl Pts',(-66.,-4.44224733169088,9.06141496467922));
#45849=CARTESIAN_POINT('Ctrl Pts',(-50.,-4.44224733169088,9.06141496467922));
#45850=CARTESIAN_POINT('Ctrl Pts',(-66.,-4.35271597876535,8.99790906190847));
#45851=CARTESIAN_POINT('Ctrl Pts',(-50.,-4.35271597876535,8.99790906190847));
#45852=CARTESIAN_POINT('Ctrl Pts',(-66.,-4.26522443974139,8.93281753244224));
#45853=CARTESIAN_POINT('Ctrl Pts',(-50.,-4.26522443974139,8.93281753244224));
#45854=CARTESIAN_POINT('Ctrl Pts',(-66.,-4.17984979305941,8.86613739951103));
#45855=CARTESIAN_POINT('Ctrl Pts',(-50.,-4.17984979305941,8.86613739951103));
#45856=CARTESIAN_POINT('Ctrl Pts',(-66.,-4.09669269754511,8.79784590915275));
#45857=CARTESIAN_POINT('Ctrl Pts',(-50.,-4.09669269754511,8.79784590915275));
#45858=CARTESIAN_POINT('Ctrl Pts',(-66.,-4.01588494277018,8.72789205657743));
#45859=CARTESIAN_POINT('Ctrl Pts',(-50.,-4.01588494277018,8.72789205657743));
#45860=CARTESIAN_POINT('Ctrl Pts',(-66.,-3.93760085807652,8.65619659951692));
#45861=CARTESIAN_POINT('Ctrl Pts',(-50.,-3.93760085807652,8.65619659951692));
#45862=CARTESIAN_POINT('Ctrl Pts',(-66.,-3.86206885883931,8.58265845343488));
#45863=CARTESIAN_POINT('Ctrl Pts',(-50.,-3.86206885883931,8.58265845343488));
#45864=CARTESIAN_POINT('Ctrl Pts',(-66.,-3.78958659965516,8.50715832573905));
#45865=CARTESIAN_POINT('Ctrl Pts',(-50.,-3.78958659965516,8.50715832573905));
#45866=CARTESIAN_POINT('Ctrl Pts',(-66.,-3.720526640373,8.42956563125176));
#45867=CARTESIAN_POINT('Ctrl Pts',(-50.,-3.720526640373,8.42956563125176));
#45868=CARTESIAN_POINT('Ctrl Pts',(-66.,-3.65536627573726,8.34973908999167));
#45869=CARTESIAN_POINT('Ctrl Pts',(-50.,-3.65536627573726,8.34973908999167));
#45870=CARTESIAN_POINT('Ctrl Pts',(-66.,-3.59461383040384,8.26755365668696));
#45871=CARTESIAN_POINT('Ctrl Pts',(-50.,-3.59461383040384,8.26755365668696));
#45872=CARTESIAN_POINT('Ctrl Pts',(-66.,-3.53867623893612,8.18294180840626));
#45873=CARTESIAN_POINT('Ctrl Pts',(-50.,-3.53867623893612,8.18294180840626));
#45874=CARTESIAN_POINT('Ctrl Pts',(-66.,-3.48773626701595,8.09593368911593));
#45875=CARTESIAN_POINT('Ctrl Pts',(-50.,-3.48773626701595,8.09593368911593));
#45876=CARTESIAN_POINT('Ctrl Pts',(-66.,-3.441640425645,8.00669249258951));
#45877=CARTESIAN_POINT('Ctrl Pts',(-50.,-3.441640425645,8.00669249258951));
#45878=CARTESIAN_POINT('Ctrl Pts',(-66.,-3.39973851923894,7.91556814228226));
#45879=CARTESIAN_POINT('Ctrl Pts',(-50.,-3.39973851923894,7.91556814228226));
#45880=CARTESIAN_POINT('Ctrl Pts',(-66.,-3.3609897589824,7.82305272705443));
#45881=CARTESIAN_POINT('Ctrl Pts',(-50.,-3.3609897589824,7.82305272705443));
#45882=CARTESIAN_POINT('Ctrl Pts',(-66.,-3.32416425071599,7.72970101571594));
#45883=CARTESIAN_POINT('Ctrl Pts',(-50.,-3.32416425071599,7.72970101571594));
#45884=CARTESIAN_POINT('Ctrl Pts',(-66.,-3.28801529731225,7.63606148881098));
#45885=CARTESIAN_POINT('Ctrl Pts',(-50.,-3.28801529731225,7.63606148881098));
#45886=CARTESIAN_POINT('Ctrl Pts',(-66.,-3.25145480239525,7.5426066324152));
#45887=CARTESIAN_POINT('Ctrl Pts',(-50.,-3.25145480239525,7.5426066324152));
#45888=CARTESIAN_POINT('Ctrl Pts',(-66.,-3.21375006071206,7.44965417630122));
#45889=CARTESIAN_POINT('Ctrl Pts',(-50.,-3.21375006071206,7.44965417630122));
#45890=CARTESIAN_POINT('Ctrl Pts',(-66.,-3.17447364404108,7.35738957226508));
#45891=CARTESIAN_POINT('Ctrl Pts',(-50.,-3.17447364404108,7.35738957226508));
#45892=CARTESIAN_POINT('Ctrl Pts',(-66.,-3.14162759082209,7.28420082769005));
#45893=CARTESIAN_POINT('Ctrl Pts',(-50.,-3.14162759082209,7.28420082769005));
#45894=CARTESIAN_POINT('Ctrl Pts',(-66.,-3.11616269844133,7.22967217437288));
#45895=CARTESIAN_POINT('Ctrl Pts',(-50.,-3.11616269844133,7.22967217437288));
#45896=CARTESIAN_POINT('Ctrl Pts',(-66.,-3.09881751111224,7.19348083086667));
#45897=CARTESIAN_POINT('Ctrl Pts',(-50.,-3.09881751111224,7.19348083086667));
#45898=CARTESIAN_POINT('Ctrl Pts',(-66.,-3.09005277149946,7.17542543124437));
#45899=CARTESIAN_POINT('Ctrl Pts',(-50.,-3.09005277149946,7.17542543124437));
#45900=CARTESIAN_POINT('Ctrl Pts',(-50.,-4.47433860192363,9.08272641200518));
#45901=CARTESIAN_POINT('Ctrl Pts',(-50.,-4.46799546208136,9.07840367583189));
#45902=CARTESIAN_POINT('Ctrl Pts',(-50.,-4.44345829930701,9.0616132340732));
#45903=CARTESIAN_POINT('Ctrl Pts',(-50.,-4.40102613216983,9.03211165933191));
#45904=CARTESIAN_POINT('Ctrl Pts',(-50.,-4.34130290913254,8.98941802189944));
#45905=CARTESIAN_POINT('Ctrl Pts',(-50.,-4.26522443974139,8.93281753244224));
#45906=CARTESIAN_POINT('Ctrl Pts',(-50.,-4.17984979305941,8.86613739951103));
#45907=CARTESIAN_POINT('Ctrl Pts',(-50.,-4.09669269754511,8.79784590915275));
#45908=CARTESIAN_POINT('Ctrl Pts',(-50.,-4.01588494277018,8.72789205657743));
#45909=CARTESIAN_POINT('Ctrl Pts',(-50.,-3.93760085807652,8.65619659951692));
#45910=CARTESIAN_POINT('Ctrl Pts',(-50.,-3.86206885883931,8.58265845343488));
#45911=CARTESIAN_POINT('Ctrl Pts',(-50.,-3.78958659965516,8.50715832573905));
#45912=CARTESIAN_POINT('Ctrl Pts',(-50.,-3.720526640373,8.42956563125176));
#45913=CARTESIAN_POINT('Ctrl Pts',(-50.,-3.65536627573726,8.34973908999167));
#45914=CARTESIAN_POINT('Ctrl Pts',(-50.,-3.59461383040384,8.26755365668696));
#45915=CARTESIAN_POINT('Ctrl Pts',(-50.,-3.53867623893612,8.18294180840626));
#45916=CARTESIAN_POINT('Ctrl Pts',(-50.,-3.48773626701595,8.09593368911593));
#45917=CARTESIAN_POINT('Ctrl Pts',(-50.,-3.441640425645,8.00669249258951));
#45918=CARTESIAN_POINT('Ctrl Pts',(-50.,-3.39973851923894,7.91556814228226));
#45919=CARTESIAN_POINT('Ctrl Pts',(-50.,-3.3609897589824,7.82305272705443));
#45920=CARTESIAN_POINT('Ctrl Pts',(-50.,-3.32416425071599,7.72970101571594));
#45921=CARTESIAN_POINT('Ctrl Pts',(-50.,-3.28801529731225,7.63606148881098));
#45922=CARTESIAN_POINT('Ctrl Pts',(-50.,-3.25145480239525,7.5426066324152));
#45923=CARTESIAN_POINT('Ctrl Pts',(-50.,-3.21375006071206,7.44965417630122));
#45924=CARTESIAN_POINT('Ctrl Pts',(-50.,-3.17447364404108,7.35738957226508));
#45925=CARTESIAN_POINT('Ctrl Pts',(-50.,-3.14162759082209,7.28420082769005));
#45926=CARTESIAN_POINT('Ctrl Pts',(-50.,-3.11616269844133,7.22967217437288));
#45927=CARTESIAN_POINT('Ctrl Pts',(-50.,-3.09881751111224,7.19348083086667));
#45928=CARTESIAN_POINT('Ctrl Pts',(-50.,-3.09005277149946,7.17542543124437));
#45929=CARTESIAN_POINT('Origin',(-50.,-3.39879369590239,8.87754687038761));
#45930=CARTESIAN_POINT('Origin',(-50.,0.,0.));
#45931=CARTESIAN_POINT('Origin',(-65.75,0.,0.));
#45932=CARTESIAN_POINT('',(-65.5,-0.730107932396199,10.5998852544286));
#45933=CARTESIAN_POINT('Origin',(-65.5,0.,0.));
#45934=CARTESIAN_POINT('',(-66.,-0.393234054947371,10.1173609196287));
#45935=CARTESIAN_POINT('Ctrl Pts',(-65.5,-0.730107932396319,10.5998852544287));
#45936=CARTESIAN_POINT('Ctrl Pts',(-65.5869131822983,-0.665642665095681,
10.5172110652076));
#45937=CARTESIAN_POINT('Ctrl Pts',(-65.6744370580972,-0.603721341078077,
10.4332627470386));
#45938=CARTESIAN_POINT('Ctrl Pts',(-65.762669377962,-0.544547419148644,
10.3480202685378));
#45939=CARTESIAN_POINT('Ctrl Pts',(-65.8411954666452,-0.491883081995573,
10.2721551157618));
#45940=CARTESIAN_POINT('Ctrl Pts',(-65.9202827042116,-0.441398804290209,
10.1952663740677));
#45941=CARTESIAN_POINT('Ctrl Pts',(-66.,-0.39323405494737,10.1173609196287));
#45942=CARTESIAN_POINT('Origin',(-66.,0.,0.));
#45943=CARTESIAN_POINT('Origin',(-58.,0.,0.));
#45944=CARTESIAN_POINT('',(-50.5,-0.730107932396199,10.5998852544286));
#45945=CARTESIAN_POINT('Origin',(-50.5,0.,0.));
#45946=CARTESIAN_POINT('Ctrl Pts',(-50.5,-0.730107932396198,10.5998852544286));
#45947=CARTESIAN_POINT('Ctrl Pts',(-55.5,-0.730107932396198,10.5998852544286));
#45948=CARTESIAN_POINT('Ctrl Pts',(-60.5,-0.730107932396198,10.5998852544286));
#45949=CARTESIAN_POINT('Ctrl Pts',(-65.5,-0.730107932396198,10.5998852544286));
#45950=CARTESIAN_POINT('Origin',(-50.25,0.,0.));
#45951=CARTESIAN_POINT('',(-50.,-0.393234054947381,10.1173609196287));
#45952=CARTESIAN_POINT('Origin',(-50.,0.,0.));
#45953=CARTESIAN_POINT('Ctrl Pts',(-50.,-0.393234054947385,10.1173609196287));
#45954=CARTESIAN_POINT('Ctrl Pts',(-50.0956594798899,-0.451030983776946,
10.2108462188794));
#45955=CARTESIAN_POINT('Ctrl Pts',(-50.190411700126,-0.512169084664846,
10.3028667171489));
#45956=CARTESIAN_POINT('Ctrl Pts',(-50.2843757312842,-0.576403624495566,
10.3934130596283));
#45957=CARTESIAN_POINT('Ctrl Pts',(-50.3566993358377,-0.625844601006806,
10.4631060877639));
#45958=CARTESIAN_POINT('Ctrl Pts',(-50.4285559937478,-0.677116466219517,
10.5319257673242));
#45959=CARTESIAN_POINT('Ctrl Pts',(-50.5,-0.730107932396319,10.5998852544287));
#45960=CARTESIAN_POINT('Origin',(-66.,0.505871070453596,9.49245655683042));
#45961=CARTESIAN_POINT('',(-66.,2.4750997369136,9.81781575974668));
#45962=CARTESIAN_POINT('Origin',(-66.,0.,0.));
#45963=CARTESIAN_POINT('',(-66.,0.0956047792658118,7.81191500057326));
#45964=CARTESIAN_POINT('Ctrl Pts',(-66.,0.0956047792658046,7.81191500057326));
#45965=CARTESIAN_POINT('Ctrl Pts',(-66.,0.0949415838368861,7.83197436965167));
#45966=CARTESIAN_POINT('Ctrl Pts',(-66.,0.0938163123065552,7.8720917303855));
#45967=CARTESIAN_POINT('Ctrl Pts',(-66.,0.0927317769444286,7.93226363877801));
#45968=CARTESIAN_POINT('Ctrl Pts',(-66.,0.0924939585041115,8.01248457735968));
#45969=CARTESIAN_POINT('Ctrl Pts',(-66.,0.094140561782238,8.11274764514689));
#45970=CARTESIAN_POINT('Ctrl Pts',(-66.,0.0975027362514239,8.2129998392668));
#45971=CARTESIAN_POINT('Ctrl Pts',(-66.,0.102114576760388,8.31324559179353));
#45972=CARTESIAN_POINT('Ctrl Pts',(-66.,0.107177491412388,8.4134926602115));
#45973=CARTESIAN_POINT('Ctrl Pts',(-66.,0.111505277305432,8.51375197567978));
#45974=CARTESIAN_POINT('Ctrl Pts',(-66.,0.113735932806315,8.61402955369318));
#45975=CARTESIAN_POINT('Ctrl Pts',(-66.,0.112520248888933,8.71431883074707));
#45976=CARTESIAN_POINT('Ctrl Pts',(-66.,0.106707267087506,8.81459358824736));
#45977=CARTESIAN_POINT('Ctrl Pts',(-66.,0.095560677487882,8.91479861358025));
#45978=CARTESIAN_POINT('Ctrl Pts',(-66.,0.078873884025214,9.01484725141515));
#45979=CARTESIAN_POINT('Ctrl Pts',(-66.,0.0568015908022762,9.11463762636861));
#45980=CARTESIAN_POINT('Ctrl Pts',(-66.,0.0297430150914363,9.21406590850962));
#45981=CARTESIAN_POINT('Ctrl Pts',(-66.,-0.00178660493279414,9.31303957811411));
#45982=CARTESIAN_POINT('Ctrl Pts',(-66.,-0.0372937750793528,9.41149356760519));
#45983=CARTESIAN_POINT('Ctrl Pts',(-66.,-0.0763850312137404,9.50939563873644));
#45984=CARTESIAN_POINT('Ctrl Pts',(-66.,-0.11873993166277,9.60673370368225));
#45985=CARTESIAN_POINT('Ctrl Pts',(-66.,-0.164108693813002,9.70350720285868));
#45986=CARTESIAN_POINT('Ctrl Pts',(-66.,-0.212299829151872,9.79971762154855));
#45987=CARTESIAN_POINT('Ctrl Pts',(-66.,-0.263172196397742,9.89535795129807));
#45988=CARTESIAN_POINT('Ctrl Pts',(-66.,-0.309651843456158,9.97800897259254));
#45989=CARTESIAN_POINT('Ctrl Pts',(-66.,-0.346846655807676,10.0413031743911));
#45990=CARTESIAN_POINT('Ctrl Pts',(-66.,-0.373610997878055,10.0855129212091));
#45991=CARTESIAN_POINT('Ctrl Pts',(-66.,-0.389197523557302,10.110831916227));
#45992=CARTESIAN_POINT('Ctrl Pts',(-66.,-0.393234054947371,10.1173609196287));
#45993=CARTESIAN_POINT('',(-66.,1.53067287083627,7.66108326625457));
#45994=CARTESIAN_POINT('Origin',(-66.,0.,0.));
#45995=CARTESIAN_POINT('Ctrl Pts',(-66.,2.4750997369136,9.81781575974667));
#45996=CARTESIAN_POINT('Ctrl Pts',(-66.,2.46072168365089,9.80407287462596));
#45997=CARTESIAN_POINT('Ctrl Pts',(-66.,2.42760988208889,9.77134522776358));
#45998=CARTESIAN_POINT('Ctrl Pts',(-66.,2.37903830357638,9.71924627901826));
#45999=CARTESIAN_POINT('Ctrl Pts',(-66.,2.31965175273437,9.64714268794233));
#46000=CARTESIAN_POINT('Ctrl Pts',(-66.,2.25145985312962,9.55424100647557));
#46001=CARTESIAN_POINT('Ctrl Pts',(-66.,2.18075461106815,9.45447850276164));
#46002=CARTESIAN_POINT('Ctrl Pts',(-66.,2.10816197016995,9.35322073006787));
#46003=CARTESIAN_POINT('Ctrl Pts',(-66.,2.0344576270999,9.25038678979018));
#46004=CARTESIAN_POINT('Ctrl Pts',(-66.,1.96244215081495,9.14584421069497));
#46005=CARTESIAN_POINT('Ctrl Pts',(-66.,1.89575134598467,9.03944732712972));
#46006=CARTESIAN_POINT('Ctrl Pts',(-66.,1.83713595327505,8.93108698145603));
#46007=CARTESIAN_POINT('Ctrl Pts',(-66.,1.78758666420428,8.82072595505194));
#46008=CARTESIAN_POINT('Ctrl Pts',(-66.,1.74690297758844,8.70841487822418));
#46009=CARTESIAN_POINT('Ctrl Pts',(-66.,1.71396195582416,8.59430989652968));
#46010=CARTESIAN_POINT('Ctrl Pts',(-66.,1.687108761575,8.4786961492651));
#46011=CARTESIAN_POINT('Ctrl Pts',(-66.,1.66446290264294,8.36199244506075));
#46012=CARTESIAN_POINT('Ctrl Pts',(-66.,1.6441151218745,8.24467002114497));
#46013=CARTESIAN_POINT('Ctrl Pts',(-66.,1.62432848933541,8.1271858608129));
#46014=CARTESIAN_POINT('Ctrl Pts',(-66.,1.60374909373978,8.00990707893858));
#46015=CARTESIAN_POINT('Ctrl Pts',(-66.,1.5815843333707,7.89304829685241));
#46016=CARTESIAN_POINT('Ctrl Pts',(-66.,1.56227021516729,7.79998240099705));
#46017=CARTESIAN_POINT('Ctrl Pts',(-66.,1.54683889623834,7.73043495565091));
#46018=CARTESIAN_POINT('Ctrl Pts',(-66.,1.53613151574638,7.68418185330693));
#46019=CARTESIAN_POINT('Ctrl Pts',(-66.,1.53067287083627,7.66108326625457));
#46020=CARTESIAN_POINT('Ctrl Pts',(-66.,1.53067287083627,7.66108326625457));
#46021=CARTESIAN_POINT('Ctrl Pts',(-50.,1.53067287083627,7.66108326625457));
#46022=CARTESIAN_POINT('Ctrl Pts',(-66.,1.53613151574638,7.68418185330693));
#46023=CARTESIAN_POINT('Ctrl Pts',(-50.,1.53613151574638,7.68418185330693));
#46024=CARTESIAN_POINT('Ctrl Pts',(-66.,1.54683889623834,7.73043495565091));
#46025=CARTESIAN_POINT('Ctrl Pts',(-50.,1.54683889623834,7.73043495565091));
#46026=CARTESIAN_POINT('Ctrl Pts',(-66.,1.56227021516729,7.79998240099705));
#46027=CARTESIAN_POINT('Ctrl Pts',(-50.,1.56227021516729,7.79998240099705));
#46028=CARTESIAN_POINT('Ctrl Pts',(-66.,1.5815843333707,7.89304829685241));
#46029=CARTESIAN_POINT('Ctrl Pts',(-50.,1.5815843333707,7.89304829685241));
#46030=CARTESIAN_POINT('Ctrl Pts',(-66.,1.60374909373978,8.00990707893858));
#46031=CARTESIAN_POINT('Ctrl Pts',(-50.,1.60374909373978,8.00990707893858));
#46032=CARTESIAN_POINT('Ctrl Pts',(-66.,1.62432848933541,8.1271858608129));
#46033=CARTESIAN_POINT('Ctrl Pts',(-50.,1.62432848933541,8.1271858608129));
#46034=CARTESIAN_POINT('Ctrl Pts',(-66.,1.6441151218745,8.24467002114497));
#46035=CARTESIAN_POINT('Ctrl Pts',(-50.,1.6441151218745,8.24467002114497));
#46036=CARTESIAN_POINT('Ctrl Pts',(-66.,1.66446290264294,8.36199244506075));
#46037=CARTESIAN_POINT('Ctrl Pts',(-50.,1.66446290264294,8.36199244506075));
#46038=CARTESIAN_POINT('Ctrl Pts',(-66.,1.687108761575,8.4786961492651));
#46039=CARTESIAN_POINT('Ctrl Pts',(-50.,1.687108761575,8.4786961492651));
#46040=CARTESIAN_POINT('Ctrl Pts',(-66.,1.71396195582416,8.59430989652968));
#46041=CARTESIAN_POINT('Ctrl Pts',(-50.,1.71396195582416,8.59430989652968));
#46042=CARTESIAN_POINT('Ctrl Pts',(-66.,1.74690297758844,8.70841487822418));
#46043=CARTESIAN_POINT('Ctrl Pts',(-50.,1.74690297758844,8.70841487822418));
#46044=CARTESIAN_POINT('Ctrl Pts',(-66.,1.78758666420428,8.82072595505194));
#46045=CARTESIAN_POINT('Ctrl Pts',(-50.,1.78758666420428,8.82072595505194));
#46046=CARTESIAN_POINT('Ctrl Pts',(-66.,1.83713595327505,8.93108698145603));
#46047=CARTESIAN_POINT('Ctrl Pts',(-50.,1.83713595327505,8.93108698145603));
#46048=CARTESIAN_POINT('Ctrl Pts',(-66.,1.89575134598467,9.03944732712972));
#46049=CARTESIAN_POINT('Ctrl Pts',(-50.,1.89575134598467,9.03944732712972));
#46050=CARTESIAN_POINT('Ctrl Pts',(-66.,1.96244215081495,9.14584421069497));
#46051=CARTESIAN_POINT('Ctrl Pts',(-50.,1.96244215081495,9.14584421069497));
#46052=CARTESIAN_POINT('Ctrl Pts',(-66.,2.0344576270999,9.25038678979018));
#46053=CARTESIAN_POINT('Ctrl Pts',(-50.,2.0344576270999,9.25038678979018));
#46054=CARTESIAN_POINT('Ctrl Pts',(-66.,2.10816197016995,9.35322073006787));
#46055=CARTESIAN_POINT('Ctrl Pts',(-50.,2.10816197016995,9.35322073006787));
#46056=CARTESIAN_POINT('Ctrl Pts',(-66.,2.18075461106815,9.45447850276164));
#46057=CARTESIAN_POINT('Ctrl Pts',(-50.,2.18075461106815,9.45447850276164));
#46058=CARTESIAN_POINT('Ctrl Pts',(-66.,2.25145985312962,9.55424100647557));
#46059=CARTESIAN_POINT('Ctrl Pts',(-50.,2.25145985312962,9.55424100647557));
#46060=CARTESIAN_POINT('Ctrl Pts',(-66.,2.32356876504542,9.65247905534274));
#46061=CARTESIAN_POINT('Ctrl Pts',(-50.,2.32356876504542,9.65247905534274));
#46062=CARTESIAN_POINT('Ctrl Pts',(-66.,2.40375833141064,9.74906184805482));
#46063=CARTESIAN_POINT('Ctrl Pts',(-50.,2.40375833141064,9.74906184805482));
#46064=CARTESIAN_POINT('Ctrl Pts',(-66.,2.49824854034584,9.8438431355273));
#46065=CARTESIAN_POINT('Ctrl Pts',(-50.,2.49824854034584,9.8438431355273));
#46066=CARTESIAN_POINT('Ctrl Pts',(-66.,2.60996854609427,9.93672339619266));
#46067=CARTESIAN_POINT('Ctrl Pts',(-50.,2.60996854609427,9.93672339619266));
#46068=CARTESIAN_POINT('Ctrl Pts',(-66.,2.7348865821668,10.0277304471861));
#46069=CARTESIAN_POINT('Ctrl Pts',(-50.,2.7348865821668,10.0277304471861));
#46070=CARTESIAN_POINT('Ctrl Pts',(-66.,2.85989756918902,10.117067973778));
#46071=CARTESIAN_POINT('Ctrl Pts',(-50.,2.85989756918902,10.117067973778));
#46072=CARTESIAN_POINT('Ctrl Pts',(-66.,2.96655997197117,10.2050458427552));
#46073=CARTESIAN_POINT('Ctrl Pts',(-50.,2.96655997197117,10.2050458427552));
#46074=CARTESIAN_POINT('Ctrl Pts',(-66.,3.03402551345445,10.2920269460792));
#46075=CARTESIAN_POINT('Ctrl Pts',(-50.,3.03402551345445,10.2920269460792));
#46076=CARTESIAN_POINT('Ctrl Pts',(-66.,3.04215148505188,10.3783701788403));
#46077=CARTESIAN_POINT('Ctrl Pts',(-50.,3.04215148505188,10.3783701788403));
#46078=CARTESIAN_POINT('Ctrl Pts',(-66.,2.9748385291403,10.4643699989842));
#46079=CARTESIAN_POINT('Ctrl Pts',(-50.,2.9748385291403,10.4643699989842));
#46080=CARTESIAN_POINT('Ctrl Pts',(-66.,2.81986096053206,10.5502574863892));
#46081=CARTESIAN_POINT('Ctrl Pts',(-50.,2.81986096053206,10.5502574863892));
#46082=CARTESIAN_POINT('Ctrl Pts',(-66.,2.56820026819713,10.6362103353318));
#46083=CARTESIAN_POINT('Ctrl Pts',(-50.,2.56820026819713,10.6362103353318));
#46084=CARTESIAN_POINT('Ctrl Pts',(-66.,2.21358394293369,10.7223593673151));
#46085=CARTESIAN_POINT('Ctrl Pts',(-50.,2.21358394293369,10.7223593673151));
#46086=CARTESIAN_POINT('Ctrl Pts',(-66.,1.7519651212833,10.8087962346463));
#46087=CARTESIAN_POINT('Ctrl Pts',(-50.,1.7519651212833,10.8087962346463));
#46088=CARTESIAN_POINT('Ctrl Pts',(-66.,1.18105323929441,10.8955803579119));
#46089=CARTESIAN_POINT('Ctrl Pts',(-50.,1.18105323929441,10.8955803579119));
#46090=CARTESIAN_POINT('Ctrl Pts',(-66.,0.499846109826311,10.9827459672994));
#46091=CARTESIAN_POINT('Ctrl Pts',(-50.,0.499846109826311,10.9827459672994));
#46092=CARTESIAN_POINT('Ctrl Pts',(-66.,-0.133484792308076,11.0527963170055));
#46093=CARTESIAN_POINT('Ctrl Pts',(-50.,-0.133484792308076,11.0527963170055));
#46094=CARTESIAN_POINT('Ctrl Pts',(-66.,-0.658079481550103,11.1055147659729));
#46095=CARTESIAN_POINT('Ctrl Pts',(-50.,-0.658079481550103,11.1055147659729));
#46096=CARTESIAN_POINT('Ctrl Pts',(-66.,-1.02982286576183,11.1407405969304));
#46097=CARTESIAN_POINT('Ctrl Pts',(-50.,-1.02982286576183,11.1407405969304));
#46098=CARTESIAN_POINT('Ctrl Pts',(-66.,-1.22119795728711,11.158373561999));
#46099=CARTESIAN_POINT('Ctrl Pts',(-50.,-1.22119795728711,11.158373561999));
#46100=CARTESIAN_POINT('',(-65.5,2.95714943969769,10.2051894735618));
#46101=CARTESIAN_POINT('Ctrl Pts',(-66.,2.47509973691359,9.81781575974667));
#46102=CARTESIAN_POINT('Ctrl Pts',(-65.7982417703062,2.64735434324867,9.98246080752347));
#46103=CARTESIAN_POINT('Ctrl Pts',(-65.6331946192803,2.85185906302854,10.097025538503));
#46104=CARTESIAN_POINT('Ctrl Pts',(-65.5,2.95714943969768,10.2051894735618));
#46105=CARTESIAN_POINT('',(-50.,1.53067287083627,7.66108326625457));
#46106=CARTESIAN_POINT('',(-66.,1.53067287083627,7.66108326625457));
#46107=CARTESIAN_POINT('',(-50.,2.47509973691361,9.81781575974669));
#46108=CARTESIAN_POINT('Ctrl Pts',(-50.,1.53067287083627,7.66108326625457));
#46109=CARTESIAN_POINT('Ctrl Pts',(-50.,1.53613151574638,7.68418185330693));
#46110=CARTESIAN_POINT('Ctrl Pts',(-50.,1.54683889623834,7.73043495565091));
#46111=CARTESIAN_POINT('Ctrl Pts',(-50.,1.56227021516729,7.79998240099705));
#46112=CARTESIAN_POINT('Ctrl Pts',(-50.,1.5815843333707,7.89304829685241));
#46113=CARTESIAN_POINT('Ctrl Pts',(-50.,1.60374909373978,8.00990707893858));
#46114=CARTESIAN_POINT('Ctrl Pts',(-50.,1.62432848933541,8.1271858608129));
#46115=CARTESIAN_POINT('Ctrl Pts',(-50.,1.6441151218745,8.24467002114497));
#46116=CARTESIAN_POINT('Ctrl Pts',(-50.,1.66446290264294,8.36199244506075));
#46117=CARTESIAN_POINT('Ctrl Pts',(-50.,1.687108761575,8.4786961492651));
#46118=CARTESIAN_POINT('Ctrl Pts',(-50.,1.71396195582416,8.59430989652968));
#46119=CARTESIAN_POINT('Ctrl Pts',(-50.,1.74690297758844,8.70841487822418));
#46120=CARTESIAN_POINT('Ctrl Pts',(-50.,1.78758666420428,8.82072595505194));
#46121=CARTESIAN_POINT('Ctrl Pts',(-50.,1.83713595327505,8.93108698145603));
#46122=CARTESIAN_POINT('Ctrl Pts',(-50.,1.89575134598467,9.03944732712972));
#46123=CARTESIAN_POINT('Ctrl Pts',(-50.,1.96244215081495,9.14584421069497));
#46124=CARTESIAN_POINT('Ctrl Pts',(-50.,2.0344576270999,9.25038678979018));
#46125=CARTESIAN_POINT('Ctrl Pts',(-50.,2.10816197016995,9.35322073006787));
#46126=CARTESIAN_POINT('Ctrl Pts',(-50.,2.18075461106815,9.45447850276164));
#46127=CARTESIAN_POINT('Ctrl Pts',(-50.,2.25145985312962,9.55424100647557));
#46128=CARTESIAN_POINT('Ctrl Pts',(-50.,2.31965175273437,9.64714268794233));
#46129=CARTESIAN_POINT('Ctrl Pts',(-50.,2.37903830357638,9.71924627901827));
#46130=CARTESIAN_POINT('Ctrl Pts',(-50.,2.4276098820889,9.77134522776359));
#46131=CARTESIAN_POINT('Ctrl Pts',(-50.,2.4607216836509,9.80407287462597));
#46132=CARTESIAN_POINT('Ctrl Pts',(-50.,2.47509973691361,9.81781575974669));
#46133=CARTESIAN_POINT('',(-50.5,2.95714943969769,10.2051894735618));
#46134=CARTESIAN_POINT('Ctrl Pts',(-50.5,2.9571494396977,10.2051894735618));
#46135=CARTESIAN_POINT('Ctrl Pts',(-50.4466445089803,2.91497191197781,10.161860847399));
#46136=CARTESIAN_POINT('Ctrl Pts',(-50.3887477139858,2.85816646933579,10.1179041696984));
#46137=CARTESIAN_POINT('Ctrl Pts',(-50.2270346138796,2.69292179906152,9.99595555654163));
#46138=CARTESIAN_POINT('Ctrl Pts',(-50.1250229592142,2.58184026816719,9.91984089708192));
#46139=CARTESIAN_POINT('Ctrl Pts',(-50.,2.47509973691361,9.81781575974669));
#46140=CARTESIAN_POINT('Ctrl Pts',(-65.5,2.95714943969769,10.2051894735618));
#46141=CARTESIAN_POINT('Ctrl Pts',(-60.5,2.95714943969769,10.2051894735618));
#46142=CARTESIAN_POINT('Ctrl Pts',(-55.5,2.95714943969769,10.2051894735618));
#46143=CARTESIAN_POINT('Ctrl Pts',(-50.5,2.95714943969769,10.2051894735618));
#46144=CARTESIAN_POINT('Origin',(-66.,0.,0.));
#46145=CARTESIAN_POINT('',(-50.,0.0956047792658118,7.81191500057326));
#46146=CARTESIAN_POINT('',(-66.,0.0956047792658118,7.81191500057326));
#46147=CARTESIAN_POINT('Origin',(-50.,0.,0.));
#46148=CARTESIAN_POINT('Ctrl Pts',(-66.,-1.22119795728711,11.158373561999));
#46149=CARTESIAN_POINT('Ctrl Pts',(-50.,-1.22119795728711,11.158373561999));
#46150=CARTESIAN_POINT('Ctrl Pts',(-66.,-1.20459005337381,11.1414802084975));
#46151=CARTESIAN_POINT('Ctrl Pts',(-50.,-1.20459005337381,11.1414802084975));
#46152=CARTESIAN_POINT('Ctrl Pts',(-66.,-1.17157016007181,11.1076086480398));
#46153=CARTESIAN_POINT('Ctrl Pts',(-50.,-1.17157016007181,11.1076086480398));
#46154=CARTESIAN_POINT('Ctrl Pts',(-66.,-1.12262806377916,11.0565467472304));
#46155=CARTESIAN_POINT('Ctrl Pts',(-50.,-1.12262806377916,11.0565467472304));
#46156=CARTESIAN_POINT('Ctrl Pts',(-66.,-1.05854898513006,10.9879544134138));
#46157=CARTESIAN_POINT('Ctrl Pts',(-50.,-1.05854898513006,10.9879544134138));
#46158=CARTESIAN_POINT('Ctrl Pts',(-66.,-0.98042435206805,10.9013612443196));
#46159=CARTESIAN_POINT('Ctrl Pts',(-50.,-0.98042435206805,10.9013612443196));
#46160=CARTESIAN_POINT('Ctrl Pts',(-66.,-0.904295528615561,10.813912873378));
#46161=CARTESIAN_POINT('Ctrl Pts',(-50.,-0.904295528615561,10.813912873378));
#46162=CARTESIAN_POINT('Ctrl Pts',(-66.,-0.830193774749181,10.7256096737113));
#46163=CARTESIAN_POINT('Ctrl Pts',(-50.,-0.830193774749181,10.7256096737113));
#46164=CARTESIAN_POINT('Ctrl Pts',(-66.,-0.758160207908483,10.6364569134394));
#46165=CARTESIAN_POINT('Ctrl Pts',(-50.,-0.758160207908483,10.6364569134394));
#46166=CARTESIAN_POINT('Ctrl Pts',(-66.,-0.688246412921118,10.5464674190292));
#46167=CARTESIAN_POINT('Ctrl Pts',(-50.,-0.688246412921118,10.5464674190292));
#46168=CARTESIAN_POINT('Ctrl Pts',(-66.,-0.62051145560108,10.4556610008753));
#46169=CARTESIAN_POINT('Ctrl Pts',(-50.,-0.62051145560108,10.4556610008753));
#46170=CARTESIAN_POINT('Ctrl Pts',(-66.,-0.55501808912882,10.3640630895747));
#46171=CARTESIAN_POINT('Ctrl Pts',(-50.,-0.55501808912882,10.3640630895747));
#46172=CARTESIAN_POINT('Ctrl Pts',(-66.,-0.491828620657976,10.2717038296071));
#46173=CARTESIAN_POINT('Ctrl Pts',(-50.,-0.491828620657976,10.2717038296071));
#46174=CARTESIAN_POINT('Ctrl Pts',(-66.,-0.431001555210865,10.1786169559436));
#46175=CARTESIAN_POINT('Ctrl Pts',(-50.,-0.431001555210865,10.1786169559436));
#46176=CARTESIAN_POINT('Ctrl Pts',(-66.,-0.372585367340722,10.0848392482018));
#46177=CARTESIAN_POINT('Ctrl Pts',(-50.,-0.372585367340722,10.0848392482018));
#46178=CARTESIAN_POINT('Ctrl Pts',(-66.,-0.316624584267477,9.99040803725309));
#46179=CARTESIAN_POINT('Ctrl Pts',(-50.,-0.316624584267477,9.99040803725309));
#46180=CARTESIAN_POINT('Ctrl Pts',(-66.,-0.263172196397742,9.89535795129807));
#46181=CARTESIAN_POINT('Ctrl Pts',(-50.,-0.263172196397742,9.89535795129807));
#46182=CARTESIAN_POINT('Ctrl Pts',(-66.,-0.212299829151872,9.79971762154855));
#46183=CARTESIAN_POINT('Ctrl Pts',(-50.,-0.212299829151872,9.79971762154855));
#46184=CARTESIAN_POINT('Ctrl Pts',(-66.,-0.164108693813002,9.70350720285868));
#46185=CARTESIAN_POINT('Ctrl Pts',(-50.,-0.164108693813002,9.70350720285868));
#46186=CARTESIAN_POINT('Ctrl Pts',(-66.,-0.11873993166277,9.60673370368225));
#46187=CARTESIAN_POINT('Ctrl Pts',(-50.,-0.11873993166277,9.60673370368225));
#46188=CARTESIAN_POINT('Ctrl Pts',(-66.,-0.0763850312137404,9.50939563873644));
#46189=CARTESIAN_POINT('Ctrl Pts',(-50.,-0.0763850312137404,9.50939563873644));
#46190=CARTESIAN_POINT('Ctrl Pts',(-66.,-0.0372937750793528,9.41149356760519));
#46191=CARTESIAN_POINT('Ctrl Pts',(-50.,-0.0372937750793528,9.41149356760519));
#46192=CARTESIAN_POINT('Ctrl Pts',(-66.,-0.00178660493279414,9.31303957811411));
#46193=CARTESIAN_POINT('Ctrl Pts',(-50.,-0.00178660493279414,9.31303957811411));
#46194=CARTESIAN_POINT('Ctrl Pts',(-66.,0.0297430150914363,9.21406590850962));
#46195=CARTESIAN_POINT('Ctrl Pts',(-50.,0.0297430150914363,9.21406590850962));
#46196=CARTESIAN_POINT('Ctrl Pts',(-66.,0.0568015908022762,9.11463762636861));
#46197=CARTESIAN_POINT('Ctrl Pts',(-50.,0.0568015908022762,9.11463762636861));
#46198=CARTESIAN_POINT('Ctrl Pts',(-66.,0.078873884025214,9.01484725141515));
#46199=CARTESIAN_POINT('Ctrl Pts',(-50.,0.078873884025214,9.01484725141515));
#46200=CARTESIAN_POINT('Ctrl Pts',(-66.,0.095560677487882,8.91479861358025));
#46201=CARTESIAN_POINT('Ctrl Pts',(-50.,0.095560677487882,8.91479861358025));
#46202=CARTESIAN_POINT('Ctrl Pts',(-66.,0.106707267087506,8.81459358824736));
#46203=CARTESIAN_POINT('Ctrl Pts',(-50.,0.106707267087506,8.81459358824736));
#46204=CARTESIAN_POINT('Ctrl Pts',(-66.,0.112520248888933,8.71431883074707));
#46205=CARTESIAN_POINT('Ctrl Pts',(-50.,0.112520248888933,8.71431883074707));
#46206=CARTESIAN_POINT('Ctrl Pts',(-66.,0.113735932806315,8.61402955369318));
#46207=CARTESIAN_POINT('Ctrl Pts',(-50.,0.113735932806315,8.61402955369318));
#46208=CARTESIAN_POINT('Ctrl Pts',(-66.,0.111505277305432,8.51375197567978));
#46209=CARTESIAN_POINT('Ctrl Pts',(-50.,0.111505277305432,8.51375197567978));
#46210=CARTESIAN_POINT('Ctrl Pts',(-66.,0.107177491412388,8.4134926602115));
#46211=CARTESIAN_POINT('Ctrl Pts',(-50.,0.107177491412388,8.4134926602115));
#46212=CARTESIAN_POINT('Ctrl Pts',(-66.,0.102114576760388,8.31324559179353));
#46213=CARTESIAN_POINT('Ctrl Pts',(-50.,0.102114576760388,8.31324559179353));
#46214=CARTESIAN_POINT('Ctrl Pts',(-66.,0.0975027362514239,8.2129998392668));
#46215=CARTESIAN_POINT('Ctrl Pts',(-50.,0.0975027362514239,8.2129998392668));
#46216=CARTESIAN_POINT('Ctrl Pts',(-66.,0.094140561782238,8.11274764514689));
#46217=CARTESIAN_POINT('Ctrl Pts',(-50.,0.094140561782238,8.11274764514689));
#46218=CARTESIAN_POINT('Ctrl Pts',(-66.,0.0924939585041115,8.01248457735968));
#46219=CARTESIAN_POINT('Ctrl Pts',(-50.,0.0924939585041115,8.01248457735968));
#46220=CARTESIAN_POINT('Ctrl Pts',(-66.,0.0927317769444286,7.93226363877801));
#46221=CARTESIAN_POINT('Ctrl Pts',(-50.,0.0927317769444286,7.93226363877801));
#46222=CARTESIAN_POINT('Ctrl Pts',(-66.,0.0938163123065552,7.8720917303855));
#46223=CARTESIAN_POINT('Ctrl Pts',(-50.,0.0938163123065552,7.8720917303855));
#46224=CARTESIAN_POINT('Ctrl Pts',(-66.,0.0949415838368861,7.83197436965167));
#46225=CARTESIAN_POINT('Ctrl Pts',(-50.,0.0949415838368861,7.83197436965167));
#46226=CARTESIAN_POINT('Ctrl Pts',(-66.,0.0956047792658046,7.81191500057326));
#46227=CARTESIAN_POINT('Ctrl Pts',(-50.,0.0956047792658046,7.81191500057326));
#46228=CARTESIAN_POINT('Ctrl Pts',(-50.,-0.393234054947381,10.1173609196287));
#46229=CARTESIAN_POINT('Ctrl Pts',(-50.,-0.389197523557309,10.110831916227));
#46230=CARTESIAN_POINT('Ctrl Pts',(-50.,-0.373610997878061,10.0855129212091));
#46231=CARTESIAN_POINT('Ctrl Pts',(-50.,-0.34684665580768,10.0413031743911));
#46232=CARTESIAN_POINT('Ctrl Pts',(-50.,-0.30965184345616,9.97800897259254));
#46233=CARTESIAN_POINT('Ctrl Pts',(-50.,-0.263172196397742,9.89535795129807));
#46234=CARTESIAN_POINT('Ctrl Pts',(-50.,-0.212299829151872,9.79971762154855));
#46235=CARTESIAN_POINT('Ctrl Pts',(-50.,-0.164108693813002,9.70350720285868));
#46236=CARTESIAN_POINT('Ctrl Pts',(-50.,-0.11873993166277,9.60673370368225));
#46237=CARTESIAN_POINT('Ctrl Pts',(-50.,-0.0763850312137404,9.50939563873644));
#46238=CARTESIAN_POINT('Ctrl Pts',(-50.,-0.0372937750793528,9.41149356760519));
#46239=CARTESIAN_POINT('Ctrl Pts',(-50.,-0.00178660493279414,9.31303957811411));
#46240=CARTESIAN_POINT('Ctrl Pts',(-50.,0.0297430150914363,9.21406590850962));
#46241=CARTESIAN_POINT('Ctrl Pts',(-50.,0.0568015908022762,9.11463762636861));
#46242=CARTESIAN_POINT('Ctrl Pts',(-50.,0.078873884025214,9.01484725141515));
#46243=CARTESIAN_POINT('Ctrl Pts',(-50.,0.095560677487882,8.91479861358025));
#46244=CARTESIAN_POINT('Ctrl Pts',(-50.,0.106707267087506,8.81459358824736));
#46245=CARTESIAN_POINT('Ctrl Pts',(-50.,0.112520248888933,8.71431883074707));
#46246=CARTESIAN_POINT('Ctrl Pts',(-50.,0.113735932806315,8.61402955369318));
#46247=CARTESIAN_POINT('Ctrl Pts',(-50.,0.111505277305432,8.51375197567978));
#46248=CARTESIAN_POINT('Ctrl Pts',(-50.,0.107177491412388,8.4134926602115));
#46249=CARTESIAN_POINT('Ctrl Pts',(-50.,0.102114576760388,8.31324559179353));
#46250=CARTESIAN_POINT('Ctrl Pts',(-50.,0.0975027362514239,8.2129998392668));
#46251=CARTESIAN_POINT('Ctrl Pts',(-50.,0.094140561782238,8.11274764514689));
#46252=CARTESIAN_POINT('Ctrl Pts',(-50.,0.0924939585041115,8.01248457735968));
#46253=CARTESIAN_POINT('Ctrl Pts',(-50.,0.0927317769444286,7.93226363877801));
#46254=CARTESIAN_POINT('Ctrl Pts',(-50.,0.0938163123065552,7.8720917303855));
#46255=CARTESIAN_POINT('Ctrl Pts',(-50.,0.0949415838368861,7.83197436965167));
#46256=CARTESIAN_POINT('Ctrl Pts',(-50.,0.0956047792658046,7.81191500057326));
#46257=CARTESIAN_POINT('Origin',(-50.,0.505871070453596,9.49245655683042));
#46258=CARTESIAN_POINT('Origin',(-50.,0.,0.));
#46259=CARTESIAN_POINT('Origin',(-65.75,0.,0.));
#46260=CARTESIAN_POINT('',(-65.5,3.64437496014557,9.98043867522185));
#46261=CARTESIAN_POINT('Origin',(-65.5,0.,0.));
#46262=CARTESIAN_POINT('',(-66.,3.7558642325485,9.40261181090992));
#46263=CARTESIAN_POINT('Ctrl Pts',(-65.5,3.64437496014557,9.98043867522184));
#46264=CARTESIAN_POINT('Ctrl Pts',(-65.6642917360006,3.69213647626342,9.78809637135388));
#46265=CARTESIAN_POINT('Ctrl Pts',(-65.8311182354843,3.72977758693438,9.59488878684897));
#46266=CARTESIAN_POINT('Ctrl Pts',(-66.,3.7558642325485,9.40261181090993));
#46267=CARTESIAN_POINT('Origin',(-66.,0.,0.));
#46268=CARTESIAN_POINT('Origin',(-58.,0.,0.));
#46269=CARTESIAN_POINT('',(-50.5,3.64437496014557,9.98043867522185));
#46270=CARTESIAN_POINT('Origin',(-50.5,0.,0.));
#46271=CARTESIAN_POINT('Ctrl Pts',(-50.5,3.64437496014557,9.98043867522185));
#46272=CARTESIAN_POINT('Ctrl Pts',(-55.5,3.64437496014557,9.98043867522185));
#46273=CARTESIAN_POINT('Ctrl Pts',(-60.5,3.64437496014557,9.98043867522185));
#46274=CARTESIAN_POINT('Ctrl Pts',(-65.5,3.64437496014557,9.98043867522185));
#46275=CARTESIAN_POINT('Origin',(-50.25,0.,0.));
#46276=CARTESIAN_POINT('',(-50.,3.7558642325485,9.40261181090994));
#46277=CARTESIAN_POINT('Origin',(-50.,0.,0.));
#46278=CARTESIAN_POINT('Ctrl Pts',(-50.,3.7558642325485,9.40261181090995));
#46279=CARTESIAN_POINT('Ctrl Pts',(-50.1688817645159,3.72977758693434,9.59488878684923));
#46280=CARTESIAN_POINT('Ctrl Pts',(-50.3357082639996,3.69213647626336,9.78809637135414));
#46281=CARTESIAN_POINT('Ctrl Pts',(-50.5,3.64437496014557,9.98043867522185));
#46282=CARTESIAN_POINT('Origin',(-66.,4.32306613303376,8.4660342683367));
#46283=CARTESIAN_POINT('',(-66.,6.25438154632586,7.96230723301848));
#46284=CARTESIAN_POINT('Origin',(-66.,0.,0.));
#46285=CARTESIAN_POINT('',(-66.,3.26473139515386,7.09765349728322));
#46286=CARTESIAN_POINT('Ctrl Pts',(-66.,3.26473139515386,7.09765349728322));
#46287=CARTESIAN_POINT('Ctrl Pts',(-66.,3.27228441642341,7.11624838867044));
#46288=CARTESIAN_POINT('Ctrl Pts',(-66.,3.2875736303622,7.15335511050624));
#46289=CARTESIAN_POINT('Ctrl Pts',(-66.,3.31105697803551,7.20876600436839));
#46290=CARTESIAN_POINT('Ctrl Pts',(-66.,3.34346851534271,7.28214820789157));
#46291=CARTESIAN_POINT('Ctrl Pts',(-66.,3.38575342590423,7.37307334414807));
#46292=CARTESIAN_POINT('Ctrl Pts',(-66.,3.42960116601568,7.46329076114798));
#46293=CARTESIAN_POINT('Ctrl Pts',(-66.,3.47458791282935,7.55299400848973));
#46294=CARTESIAN_POINT('Ctrl Pts',(-66.,3.51998727159863,7.64251498957522));
#46295=CARTESIAN_POINT('Ctrl Pts',(-66.,3.56472003815351,7.73234616270153));
#46296=CARTESIAN_POINT('Ctrl Pts',(-66.,3.60754440881085,7.82304699926879));
#46297=CARTESIAN_POINT('Ctrl Pts',(-66.,3.6472251501756,7.91516027596723));
#46298=CARTESIAN_POINT('Ctrl Pts',(-66.,3.68270014530645,8.009130177902));
#46299=CARTESIAN_POINT('Ctrl Pts',(-66.,3.71327428463273,8.10520575006332));
#46300=CARTESIAN_POINT('Ctrl Pts',(-66.,3.73872358735957,8.20339185905743));
#46301=CARTESIAN_POINT('Ctrl Pts',(-66.,3.75914794626584,8.3035325132631));
#46302=CARTESIAN_POINT('Ctrl Pts',(-66.,3.77486983303976,8.40537048302527));
#46303=CARTESIAN_POINT('Ctrl Pts',(-66.,3.78632231001325,8.50861168112478));
#46304=CARTESIAN_POINT('Ctrl Pts',(-66.,3.79392974119514,8.61299594320168));
#46305=CARTESIAN_POINT('Ctrl Pts',(-66.,3.79803846148212,8.71833378187116));
#46306=CARTESIAN_POINT('Ctrl Pts',(-66.,3.79893629234755,8.82448381898456));
#46307=CARTESIAN_POINT('Ctrl Pts',(-66.,3.79685119396006,8.93134394759486));
#46308=CARTESIAN_POINT('Ctrl Pts',(-66.,3.79195870389943,9.03883763918063));
#46309=CARTESIAN_POINT('Ctrl Pts',(-66.,3.78438491054742,9.14690108386965));
#46310=CARTESIAN_POINT('Ctrl Pts',(-66.,3.77554083905247,9.24131152455862));
#46311=CARTESIAN_POINT('Ctrl Pts',(-66.,3.76730575834657,9.31426214822247));
#46312=CARTESIAN_POINT('Ctrl Pts',(-66.,3.76083703923337,9.36553580025943));
#46313=CARTESIAN_POINT('Ctrl Pts',(-66.,3.7568962025383,9.39500546428211));
#46314=CARTESIAN_POINT('Ctrl Pts',(-66.,3.7558642325485,9.40261181090992));
#46315=CARTESIAN_POINT('',(-66.,4.51438253832981,6.37616707337746));
#46316=CARTESIAN_POINT('Origin',(-66.,0.,0.));
#46317=CARTESIAN_POINT('Ctrl Pts',(-66.,6.25438154632586,7.96230723301848));
#46318=CARTESIAN_POINT('Ctrl Pts',(-66.,6.2356568061178,7.95560056385959));
#46319=CARTESIAN_POINT('Ctrl Pts',(-66.,6.1920961369859,7.93917015374265));
#46320=CARTESIAN_POINT('Ctrl Pts',(-66.,6.12653324054481,7.91133123656148));
#46321=CARTESIAN_POINT('Ctrl Pts',(-66.,6.04295375419009,7.86961601478767));
#46322=CARTESIAN_POINT('Ctrl Pts',(-66.,5.94287083600227,7.81248225000655));
#46323=CARTESIAN_POINT('Ctrl Pts',(-66.,5.83770131742005,7.75010308069958));
#46324=CARTESIAN_POINT('Ctrl Pts',(-66.,5.73019939351842,7.68712558947513));
#46325=CARTESIAN_POINT('Ctrl Pts',(-66.,5.62104079403545,7.62316036752337));
#46326=CARTESIAN_POINT('Ctrl Pts',(-66.,5.51273008511568,7.55694730233435));
#46327=CARTESIAN_POINT('Ctrl Pts',(-66.,5.4085294920414,7.48687450672668));
#46328=CARTESIAN_POINT('Ctrl Pts',(-66.,5.31090754304174,7.41172343321117));
#46329=CARTESIAN_POINT('Ctrl Pts',(-66.,5.22075414167572,7.33105713034238));
#46330=CARTESIAN_POINT('Ctrl Pts',(-66.,5.13790671419851,7.2450034023855));
#46331=CARTESIAN_POINT('Ctrl Pts',(-66.,5.061402916183,7.15416163527599));
#46332=CARTESIAN_POINT('Ctrl Pts',(-66.,4.98984695509768,7.05946539970615));
#46333=CARTESIAN_POINT('Ctrl Pts',(-66.,4.9216912606533,6.9620621614818));
#46334=CARTESIAN_POINT('Ctrl Pts',(-66.,4.85538330909815,6.86315898207772));
#46335=CARTESIAN_POINT('Ctrl Pts',(-66.,4.78952220783198,6.76387980955812));
#46336=CARTESIAN_POINT('Ctrl Pts',(-66.,4.72302041642098,6.66511070538007));
#46337=CARTESIAN_POINT('Ctrl Pts',(-66.,4.65524115152641,6.56737011604671));
#46338=CARTESIAN_POINT('Ctrl Pts',(-66.,4.59974351650827,6.49020594922863));
#46339=CARTESIAN_POINT('Ctrl Pts',(-66.,4.5573588107407,6.43294767930141));
#46340=CARTESIAN_POINT('Ctrl Pts',(-66.,4.52876430034979,6.39504845175062));
#46341=CARTESIAN_POINT('Ctrl Pts',(-66.,4.51438253832981,6.37616707337746));
#46342=CARTESIAN_POINT('Ctrl Pts',(-66.,4.51438253832981,6.37616707337746));
#46343=CARTESIAN_POINT('Ctrl Pts',(-50.,4.51438253832981,6.37616707337746));
#46344=CARTESIAN_POINT('Ctrl Pts',(-66.,4.52876430034979,6.39504845175062));
#46345=CARTESIAN_POINT('Ctrl Pts',(-50.,4.52876430034979,6.39504845175062));
#46346=CARTESIAN_POINT('Ctrl Pts',(-66.,4.5573588107407,6.43294767930141));
#46347=CARTESIAN_POINT('Ctrl Pts',(-50.,4.5573588107407,6.43294767930141));
#46348=CARTESIAN_POINT('Ctrl Pts',(-66.,4.59974351650827,6.49020594922863));
#46349=CARTESIAN_POINT('Ctrl Pts',(-50.,4.59974351650827,6.49020594922863));
#46350=CARTESIAN_POINT('Ctrl Pts',(-66.,4.65524115152641,6.56737011604671));
#46351=CARTESIAN_POINT('Ctrl Pts',(-50.,4.65524115152641,6.56737011604671));
#46352=CARTESIAN_POINT('Ctrl Pts',(-66.,4.72302041642098,6.66511070538007));
#46353=CARTESIAN_POINT('Ctrl Pts',(-50.,4.72302041642098,6.66511070538007));
#46354=CARTESIAN_POINT('Ctrl Pts',(-66.,4.78952220783198,6.76387980955812));
#46355=CARTESIAN_POINT('Ctrl Pts',(-50.,4.78952220783198,6.76387980955812));
#46356=CARTESIAN_POINT('Ctrl Pts',(-66.,4.85538330909815,6.86315898207772));
#46357=CARTESIAN_POINT('Ctrl Pts',(-50.,4.85538330909815,6.86315898207772));
#46358=CARTESIAN_POINT('Ctrl Pts',(-66.,4.9216912606533,6.9620621614818));
#46359=CARTESIAN_POINT('Ctrl Pts',(-50.,4.9216912606533,6.9620621614818));
#46360=CARTESIAN_POINT('Ctrl Pts',(-66.,4.98984695509768,7.05946539970615));
#46361=CARTESIAN_POINT('Ctrl Pts',(-50.,4.98984695509768,7.05946539970615));
#46362=CARTESIAN_POINT('Ctrl Pts',(-66.,5.061402916183,7.15416163527599));
#46363=CARTESIAN_POINT('Ctrl Pts',(-50.,5.061402916183,7.15416163527599));
#46364=CARTESIAN_POINT('Ctrl Pts',(-66.,5.13790671419851,7.2450034023855));
#46365=CARTESIAN_POINT('Ctrl Pts',(-50.,5.13790671419851,7.2450034023855));
#46366=CARTESIAN_POINT('Ctrl Pts',(-66.,5.22075414167572,7.33105713034238));
#46367=CARTESIAN_POINT('Ctrl Pts',(-50.,5.22075414167572,7.33105713034238));
#46368=CARTESIAN_POINT('Ctrl Pts',(-66.,5.31090754304174,7.41172343321117));
#46369=CARTESIAN_POINT('Ctrl Pts',(-50.,5.31090754304174,7.41172343321117));
#46370=CARTESIAN_POINT('Ctrl Pts',(-66.,5.4085294920414,7.48687450672668));
#46371=CARTESIAN_POINT('Ctrl Pts',(-50.,5.4085294920414,7.48687450672668));
#46372=CARTESIAN_POINT('Ctrl Pts',(-66.,5.51273008511568,7.55694730233435));
#46373=CARTESIAN_POINT('Ctrl Pts',(-50.,5.51273008511568,7.55694730233435));
#46374=CARTESIAN_POINT('Ctrl Pts',(-66.,5.62104079403545,7.62316036752337));
#46375=CARTESIAN_POINT('Ctrl Pts',(-50.,5.62104079403545,7.62316036752337));
#46376=CARTESIAN_POINT('Ctrl Pts',(-66.,5.73019939351842,7.68712558947513));
#46377=CARTESIAN_POINT('Ctrl Pts',(-50.,5.73019939351842,7.68712558947513));
#46378=CARTESIAN_POINT('Ctrl Pts',(-66.,5.83770131742005,7.75010308069958));
#46379=CARTESIAN_POINT('Ctrl Pts',(-50.,5.83770131742005,7.75010308069958));
#46380=CARTESIAN_POINT('Ctrl Pts',(-66.,5.94287083600227,7.81248225000655));
#46381=CARTESIAN_POINT('Ctrl Pts',(-50.,5.94287083600227,7.81248225000655));
#46382=CARTESIAN_POINT('Ctrl Pts',(-66.,6.04870261915705,7.87289783654834));
#46383=CARTESIAN_POINT('Ctrl Pts',(-50.,6.04870261915705,7.87289783654834));
#46384=CARTESIAN_POINT('Ctrl Pts',(-66.,6.16124319414692,7.92851457308381));
#46385=CARTESIAN_POINT('Ctrl Pts',(-50.,6.16124319414692,7.92851457308381));
#46386=CARTESIAN_POINT('Ctrl Pts',(-66.,6.28611531800434,7.97666895733798));
#46387=CARTESIAN_POINT('Ctrl Pts',(-50.,6.28611531800434,7.97666895733798));
#46388=CARTESIAN_POINT('Ctrl Pts',(-66.,6.42595442721465,8.01607867747095));
#46389=CARTESIAN_POINT('Ctrl Pts',(-50.,6.42595442721465,8.01607867747095));
#46390=CARTESIAN_POINT('Ctrl Pts',(-66.,6.57708863406363,8.04840901286766));
#46391=CARTESIAN_POINT('Ctrl Pts',(-50.,6.57708863406363,8.04840901286766));
#46392=CARTESIAN_POINT('Ctrl Pts',(-66.,6.72762869907988,8.07917635527372));
#46393=CARTESIAN_POINT('Ctrl Pts',(-50.,6.72762869907988,8.07917635527372));
#46394=CARTESIAN_POINT('Ctrl Pts',(-66.,6.86085347573554,8.11616463020096));
#46395=CARTESIAN_POINT('Ctrl Pts',(-50.,6.86085347573554,8.11616463020096));
#46396=CARTESIAN_POINT('Ctrl Pts',(-66.,6.95786471668201,8.16818511417712));
#46397=CARTESIAN_POINT('Ctrl Pts',(-50.,6.95786471668201,8.16818511417712));
#46398=CARTESIAN_POINT('Ctrl Pts',(-66.,7.00040711776935,8.24375845185494));
#46399=CARTESIAN_POINT('Ctrl Pts',(-50.,7.00040711776935,8.24375845185494));
#46400=CARTESIAN_POINT('Ctrl Pts',(-66.,6.97389295080625,8.3497018426284));
#46401=CARTESIAN_POINT('Ctrl Pts',(-50.,6.97389295080625,8.3497018426284));
#46402=CARTESIAN_POINT('Ctrl Pts',(-66.,6.86724748527703,8.49119902262338));
#46403=CARTESIAN_POINT('Ctrl Pts',(-50.,6.86724748527703,8.49119902262338));
#46404=CARTESIAN_POINT('Ctrl Pts',(-66.,6.672304176169,8.67208048254081));
#46405=CARTESIAN_POINT('Ctrl Pts',(-50.,6.672304176169,8.67208048254081));
#46406=CARTESIAN_POINT('Ctrl Pts',(-66.,6.38338601109175,8.89501699310692));
#46407=CARTESIAN_POINT('Ctrl Pts',(-50.,6.38338601109175,8.89501699310692));
#46408=CARTESIAN_POINT('Ctrl Pts',(-66.,5.99683327466702,9.16173829052894));
#46409=CARTESIAN_POINT('Ctrl Pts',(-50.,5.99683327466702,9.16173829052894));
#46410=CARTESIAN_POINT('Ctrl Pts',(-66.,5.51057760113121,9.47323031450598));
#46411=CARTESIAN_POINT('Ctrl Pts',(-50.,5.51057760113121,9.47323031450598));
#46412=CARTESIAN_POINT('Ctrl Pts',(-66.,4.92371736964581,9.82993196210374));
#46413=CARTESIAN_POINT('Ctrl Pts',(-50.,4.92371736964581,9.82993196210374));
#46414=CARTESIAN_POINT('Ctrl Pts',(-66.,4.37363284490199,10.1515250259743));
#46415=CARTESIAN_POINT('Ctrl Pts',(-50.,4.37363284490199,10.1515250259743));
#46416=CARTESIAN_POINT('Ctrl Pts',(-66.,3.91583427440266,10.4130576084401));
#46417=CARTESIAN_POINT('Ctrl Pts',(-50.,3.91583427440266,10.4130576084401));
#46418=CARTESIAN_POINT('Ctrl Pts',(-66.,3.59055743058054,10.5964396624829));
#46419=CARTESIAN_POINT('Ctrl Pts',(-50.,3.59055743058054,10.5964396624829));
#46420=CARTESIAN_POINT('Ctrl Pts',(-66.,3.42289955803116,10.6903874399214));
#46421=CARTESIAN_POINT('Ctrl Pts',(-50.,3.42289955803116,10.6903874399214));
#46422=CARTESIAN_POINT('',(-65.5,6.85231494663519,8.12012345177831));
#46423=CARTESIAN_POINT('Ctrl Pts',(-66.,6.25438154632586,7.96230723301848));
#46424=CARTESIAN_POINT('Ctrl Pts',(-65.7982417703063,6.478711133533,8.04265570820322));
#46425=CARTESIAN_POINT('Ctrl Pts',(-65.6331946192803,6.71213316544796,8.06413623457925));
#46426=CARTESIAN_POINT('Ctrl Pts',(-65.5,6.85231494663518,8.1201234517783));
#46427=CARTESIAN_POINT('',(-50.,4.51438253832981,6.37616707337746));
#46428=CARTESIAN_POINT('',(-66.,4.51438253832981,6.37616707337746));
#46429=CARTESIAN_POINT('',(-50.,6.25438154632588,7.96230723301849));
#46430=CARTESIAN_POINT('Ctrl Pts',(-50.,4.51438253832981,6.37616707337746));
#46431=CARTESIAN_POINT('Ctrl Pts',(-50.,4.52876430034979,6.39504845175062));
#46432=CARTESIAN_POINT('Ctrl Pts',(-50.,4.5573588107407,6.43294767930141));
#46433=CARTESIAN_POINT('Ctrl Pts',(-50.,4.59974351650827,6.49020594922863));
#46434=CARTESIAN_POINT('Ctrl Pts',(-50.,4.65524115152641,6.56737011604671));
#46435=CARTESIAN_POINT('Ctrl Pts',(-50.,4.72302041642098,6.66511070538007));
#46436=CARTESIAN_POINT('Ctrl Pts',(-50.,4.78952220783198,6.76387980955812));
#46437=CARTESIAN_POINT('Ctrl Pts',(-50.,4.85538330909815,6.86315898207772));
#46438=CARTESIAN_POINT('Ctrl Pts',(-50.,4.9216912606533,6.9620621614818));
#46439=CARTESIAN_POINT('Ctrl Pts',(-50.,4.98984695509768,7.05946539970615));
#46440=CARTESIAN_POINT('Ctrl Pts',(-50.,5.061402916183,7.15416163527599));
#46441=CARTESIAN_POINT('Ctrl Pts',(-50.,5.13790671419851,7.2450034023855));
#46442=CARTESIAN_POINT('Ctrl Pts',(-50.,5.22075414167572,7.33105713034238));
#46443=CARTESIAN_POINT('Ctrl Pts',(-50.,5.31090754304174,7.41172343321117));
#46444=CARTESIAN_POINT('Ctrl Pts',(-50.,5.4085294920414,7.48687450672668));
#46445=CARTESIAN_POINT('Ctrl Pts',(-50.,5.51273008511568,7.55694730233435));
#46446=CARTESIAN_POINT('Ctrl Pts',(-50.,5.62104079403545,7.62316036752337));
#46447=CARTESIAN_POINT('Ctrl Pts',(-50.,5.73019939351842,7.68712558947513));
#46448=CARTESIAN_POINT('Ctrl Pts',(-50.,5.83770131742005,7.75010308069958));
#46449=CARTESIAN_POINT('Ctrl Pts',(-50.,5.94287083600227,7.81248225000655));
#46450=CARTESIAN_POINT('Ctrl Pts',(-50.,6.04295375419009,7.86961601478767));
#46451=CARTESIAN_POINT('Ctrl Pts',(-50.,6.12653324054482,7.91133123656149));
#46452=CARTESIAN_POINT('Ctrl Pts',(-50.,6.19209613698591,7.93917015374266));
#46453=CARTESIAN_POINT('Ctrl Pts',(-50.,6.23565680611781,7.9556005638596));
#46454=CARTESIAN_POINT('Ctrl Pts',(-50.,6.25438154632588,7.96230723301849));
#46455=CARTESIAN_POINT('',(-50.5,6.85231494663519,8.12012345177831));
#46456=CARTESIAN_POINT('Ctrl Pts',(-50.5,6.8523149466352,8.12012345177831));
#46457=CARTESIAN_POINT('Ctrl Pts',(-50.493830180584,6.8458214690457,8.11753002104072));
#46458=CARTESIAN_POINT('Ctrl Pts',(-50.4876312970856,6.83917923121437,8.1150220909353));
#46459=CARTESIAN_POINT('Ctrl Pts',(-50.3468664668717,6.68598458219145,8.06000624664622));
#46460=CARTESIAN_POINT('Ctrl Pts',(-50.1957285018887,6.47200684022351,8.04025442110009));
#46461=CARTESIAN_POINT('Ctrl Pts',(-50.,6.25438154632588,7.96230723301849));
#46462=CARTESIAN_POINT('Ctrl Pts',(-65.5,6.85231494663519,8.1201234517783));
#46463=CARTESIAN_POINT('Ctrl Pts',(-60.5,6.85231494663519,8.1201234517783));
#46464=CARTESIAN_POINT('Ctrl Pts',(-55.5,6.85231494663519,8.12012345177831));
#46465=CARTESIAN_POINT('Ctrl Pts',(-50.5,6.85231494663519,8.12012345177831));
#46466=CARTESIAN_POINT('Origin',(-66.,0.,0.));
#46467=CARTESIAN_POINT('',(-50.,3.26473139515386,7.09765349728322));
#46468=CARTESIAN_POINT('',(-66.,3.26473139515386,7.09765349728322));
#46469=CARTESIAN_POINT('Origin',(-50.,0.,0.));
#46470=CARTESIAN_POINT('Ctrl Pts',(-66.,3.42289955803116,10.6903874399214));
#46471=CARTESIAN_POINT('Ctrl Pts',(-50.,3.42289955803116,10.6903874399214));
#46472=CARTESIAN_POINT('Ctrl Pts',(-66.,3.43120048731865,10.6681995504796));
#46473=CARTESIAN_POINT('Ctrl Pts',(-50.,3.43120048731865,10.6681995504796));
#46474=CARTESIAN_POINT('Ctrl Pts',(-66.,3.44758885606022,10.6238259397238));
#46475=CARTESIAN_POINT('Ctrl Pts',(-50.,3.44758885606022,10.6238259397238));
#46476=CARTESIAN_POINT('Ctrl Pts',(-66.,3.47153093969157,10.5572720282296));
#46477=CARTESIAN_POINT('Ctrl Pts',(-50.,3.47153093969157,10.5572720282296));
#46478=CARTESIAN_POINT('Ctrl Pts',(-66.,3.50217107532409,10.4685465039012));
#46479=CARTESIAN_POINT('Ctrl Pts',(-50.,3.50217107532409,10.4685465039012));
#46480=CARTESIAN_POINT('Ctrl Pts',(-66.,3.53832086407721,10.3576635566192));
#46481=CARTESIAN_POINT('Ctrl Pts',(-50.,3.53832086407721,10.3576635566192));
#46482=CARTESIAN_POINT('Ctrl Pts',(-66.,3.57229954809871,10.2468111124749));
#46483=CARTESIAN_POINT('Ctrl Pts',(-50.,3.57229954809871,10.2468111124749));
#46484=CARTESIAN_POINT('Ctrl Pts',(-66.,3.60407872174138,10.1360022269104));
#46485=CARTESIAN_POINT('Ctrl Pts',(-50.,3.60407872174138,10.1360022269104));
#46486=CARTESIAN_POINT('Ctrl Pts',(-66.,3.63362296509257,10.0252584365622));
#46487=CARTESIAN_POINT('Ctrl Pts',(-50.,3.63362296509257,10.0252584365622));
#46488=CARTESIAN_POINT('Ctrl Pts',(-66.,3.66089037006135,9.91461244043035));
#46489=CARTESIAN_POINT('Ctrl Pts',(-50.,3.66089037006135,9.91461244043035));
#46490=CARTESIAN_POINT('Ctrl Pts',(-66.,3.68583503495501,9.80410636044176));
#46491=CARTESIAN_POINT('Ctrl Pts',(-50.,3.68583503495501,9.80410636044176));
#46492=CARTESIAN_POINT('Ctrl Pts',(-66.,3.70840997544632,9.69378895262094));
#46493=CARTESIAN_POINT('Ctrl Pts',(-50.,3.70840997544632,9.69378895262094));
#46494=CARTESIAN_POINT('Ctrl Pts',(-66.,3.72857053198252,9.58371309792272));
#46495=CARTESIAN_POINT('Ctrl Pts',(-50.,3.72857053198252,9.58371309792272));
#46496=CARTESIAN_POINT('Ctrl Pts',(-66.,3.74627697881514,9.47393341091317));
#46497=CARTESIAN_POINT('Ctrl Pts',(-50.,3.74627697881514,9.47393341091317));
#46498=CARTESIAN_POINT('Ctrl Pts',(-66.,3.76149999185445,9.36450320782188));
#46499=CARTESIAN_POINT('Ctrl Pts',(-50.,3.76149999185445,9.36450320782188));
#46500=CARTESIAN_POINT('Ctrl Pts',(-66.,3.77421407729429,9.25547470294892));
#46501=CARTESIAN_POINT('Ctrl Pts',(-50.,3.77421407729429,9.25547470294892));
#46502=CARTESIAN_POINT('Ctrl Pts',(-66.,3.78438491054742,9.14690108386965));
#46503=CARTESIAN_POINT('Ctrl Pts',(-50.,3.78438491054742,9.14690108386965));
#46504=CARTESIAN_POINT('Ctrl Pts',(-66.,3.79195870389943,9.03883763918063));
#46505=CARTESIAN_POINT('Ctrl Pts',(-50.,3.79195870389943,9.03883763918063));
#46506=CARTESIAN_POINT('Ctrl Pts',(-66.,3.79685119396006,8.93134394759486));
#46507=CARTESIAN_POINT('Ctrl Pts',(-50.,3.79685119396006,8.93134394759486));
#46508=CARTESIAN_POINT('Ctrl Pts',(-66.,3.79893629234755,8.82448381898456));
#46509=CARTESIAN_POINT('Ctrl Pts',(-50.,3.79893629234755,8.82448381898456));
#46510=CARTESIAN_POINT('Ctrl Pts',(-66.,3.79803846148212,8.71833378187116));
#46511=CARTESIAN_POINT('Ctrl Pts',(-50.,3.79803846148212,8.71833378187116));
#46512=CARTESIAN_POINT('Ctrl Pts',(-66.,3.79392974119514,8.61299594320168));
#46513=CARTESIAN_POINT('Ctrl Pts',(-50.,3.79392974119514,8.61299594320168));
#46514=CARTESIAN_POINT('Ctrl Pts',(-66.,3.78632231001325,8.50861168112478));
#46515=CARTESIAN_POINT('Ctrl Pts',(-50.,3.78632231001325,8.50861168112478));
#46516=CARTESIAN_POINT('Ctrl Pts',(-66.,3.77486983303976,8.40537048302527));
#46517=CARTESIAN_POINT('Ctrl Pts',(-50.,3.77486983303976,8.40537048302527));
#46518=CARTESIAN_POINT('Ctrl Pts',(-66.,3.75914794626584,8.3035325132631));
#46519=CARTESIAN_POINT('Ctrl Pts',(-50.,3.75914794626584,8.3035325132631));
#46520=CARTESIAN_POINT('Ctrl Pts',(-66.,3.73872358735957,8.20339185905743));
#46521=CARTESIAN_POINT('Ctrl Pts',(-50.,3.73872358735957,8.20339185905743));
#46522=CARTESIAN_POINT('Ctrl Pts',(-66.,3.71327428463273,8.10520575006332));
#46523=CARTESIAN_POINT('Ctrl Pts',(-50.,3.71327428463273,8.10520575006332));
#46524=CARTESIAN_POINT('Ctrl Pts',(-66.,3.68270014530645,8.009130177902));
#46525=CARTESIAN_POINT('Ctrl Pts',(-50.,3.68270014530645,8.009130177902));
#46526=CARTESIAN_POINT('Ctrl Pts',(-66.,3.6472251501756,7.91516027596723));
#46527=CARTESIAN_POINT('Ctrl Pts',(-50.,3.6472251501756,7.91516027596723));
#46528=CARTESIAN_POINT('Ctrl Pts',(-66.,3.60754440881085,7.82304699926879));
#46529=CARTESIAN_POINT('Ctrl Pts',(-50.,3.60754440881085,7.82304699926879));
#46530=CARTESIAN_POINT('Ctrl Pts',(-66.,3.56472003815351,7.73234616270153));
#46531=CARTESIAN_POINT('Ctrl Pts',(-50.,3.56472003815351,7.73234616270153));
#46532=CARTESIAN_POINT('Ctrl Pts',(-66.,3.51998727159863,7.64251498957522));
#46533=CARTESIAN_POINT('Ctrl Pts',(-50.,3.51998727159863,7.64251498957522));
#46534=CARTESIAN_POINT('Ctrl Pts',(-66.,3.47458791282935,7.55299400848973));
#46535=CARTESIAN_POINT('Ctrl Pts',(-50.,3.47458791282935,7.55299400848973));
#46536=CARTESIAN_POINT('Ctrl Pts',(-66.,3.42960116601568,7.46329076114798));
#46537=CARTESIAN_POINT('Ctrl Pts',(-50.,3.42960116601568,7.46329076114798));
#46538=CARTESIAN_POINT('Ctrl Pts',(-66.,3.38575342590423,7.37307334414807));
#46539=CARTESIAN_POINT('Ctrl Pts',(-50.,3.38575342590423,7.37307334414807));
#46540=CARTESIAN_POINT('Ctrl Pts',(-66.,3.34346851534271,7.28214820789157));
#46541=CARTESIAN_POINT('Ctrl Pts',(-50.,3.34346851534271,7.28214820789157));
#46542=CARTESIAN_POINT('Ctrl Pts',(-66.,3.31105697803551,7.20876600436839));
#46543=CARTESIAN_POINT('Ctrl Pts',(-50.,3.31105697803551,7.20876600436839));
#46544=CARTESIAN_POINT('Ctrl Pts',(-66.,3.2875736303622,7.15335511050624));
#46545=CARTESIAN_POINT('Ctrl Pts',(-50.,3.2875736303622,7.15335511050624));
#46546=CARTESIAN_POINT('Ctrl Pts',(-66.,3.27228441642341,7.11624838867044));
#46547=CARTESIAN_POINT('Ctrl Pts',(-50.,3.27228441642341,7.11624838867044));
#46548=CARTESIAN_POINT('Ctrl Pts',(-66.,3.26473139515386,7.09765349728322));
#46549=CARTESIAN_POINT('Ctrl Pts',(-50.,3.26473139515386,7.09765349728322));
#46550=CARTESIAN_POINT('Ctrl Pts',(-50.,3.7558642325485,9.40261181090994));
#46551=CARTESIAN_POINT('Ctrl Pts',(-50.,3.7568962025383,9.39500546428213));
#46552=CARTESIAN_POINT('Ctrl Pts',(-50.,3.76083703923337,9.36553580025944));
#46553=CARTESIAN_POINT('Ctrl Pts',(-50.,3.76730575834657,9.31426214822248));
#46554=CARTESIAN_POINT('Ctrl Pts',(-50.,3.77554083905247,9.24131152455862));
#46555=CARTESIAN_POINT('Ctrl Pts',(-50.,3.78438491054742,9.14690108386965));
#46556=CARTESIAN_POINT('Ctrl Pts',(-50.,3.79195870389943,9.03883763918063));
#46557=CARTESIAN_POINT('Ctrl Pts',(-50.,3.79685119396006,8.93134394759486));
#46558=CARTESIAN_POINT('Ctrl Pts',(-50.,3.79893629234755,8.82448381898456));
#46559=CARTESIAN_POINT('Ctrl Pts',(-50.,3.79803846148212,8.71833378187116));
#46560=CARTESIAN_POINT('Ctrl Pts',(-50.,3.79392974119514,8.61299594320168));
#46561=CARTESIAN_POINT('Ctrl Pts',(-50.,3.78632231001325,8.50861168112478));
#46562=CARTESIAN_POINT('Ctrl Pts',(-50.,3.77486983303976,8.40537048302527));
#46563=CARTESIAN_POINT('Ctrl Pts',(-50.,3.75914794626584,8.3035325132631));
#46564=CARTESIAN_POINT('Ctrl Pts',(-50.,3.73872358735957,8.20339185905743));
#46565=CARTESIAN_POINT('Ctrl Pts',(-50.,3.71327428463273,8.10520575006332));
#46566=CARTESIAN_POINT('Ctrl Pts',(-50.,3.68270014530645,8.009130177902));
#46567=CARTESIAN_POINT('Ctrl Pts',(-50.,3.6472251501756,7.91516027596723));
#46568=CARTESIAN_POINT('Ctrl Pts',(-50.,3.60754440881085,7.82304699926879));
#46569=CARTESIAN_POINT('Ctrl Pts',(-50.,3.56472003815351,7.73234616270153));
#46570=CARTESIAN_POINT('Ctrl Pts',(-50.,3.51998727159863,7.64251498957522));
#46571=CARTESIAN_POINT('Ctrl Pts',(-50.,3.47458791282935,7.55299400848973));
#46572=CARTESIAN_POINT('Ctrl Pts',(-50.,3.42960116601568,7.46329076114798));
#46573=CARTESIAN_POINT('Ctrl Pts',(-50.,3.38575342590423,7.37307334414807));
#46574=CARTESIAN_POINT('Ctrl Pts',(-50.,3.34346851534271,7.28214820789157));
#46575=CARTESIAN_POINT('Ctrl Pts',(-50.,3.31105697803551,7.20876600436839));
#46576=CARTESIAN_POINT('Ctrl Pts',(-50.,3.2875736303622,7.15335511050624));
#46577=CARTESIAN_POINT('Ctrl Pts',(-50.,3.27228441642341,7.11624838867044));
#46578=CARTESIAN_POINT('Ctrl Pts',(-50.,3.26473139515386,7.09765349728322));
#46579=CARTESIAN_POINT('Origin',(-50.,4.32306613303376,8.4660342683367));
#46580=CARTESIAN_POINT('Origin',(-50.,0.,0.));
#46581=CARTESIAN_POINT('Origin',(-65.75,0.,0.));
#46582=CARTESIAN_POINT('',(-65.5,7.38871231397104,7.63528357963034));
#46583=CARTESIAN_POINT('Origin',(-65.5,0.,0.));
#46584=CARTESIAN_POINT('',(-66.,7.25553947328137,7.06206570003818));
#46585=CARTESIAN_POINT('Ctrl Pts',(-65.5,7.38871231397104,7.63528357963033));
#46586=CARTESIAN_POINT('Ctrl Pts',(-65.6642917360006,7.35411196707391,7.44014378288531));
#46587=CARTESIAN_POINT('Ctrl Pts',(-65.8311182354837,7.30991422840986,7.24832985268342));
#46588=CARTESIAN_POINT('Ctrl Pts',(-66.,7.25553947328137,7.06206570003818));
#46589=CARTESIAN_POINT('Origin',(-66.,0.,0.));
#46590=CARTESIAN_POINT('Origin',(-58.,0.,0.));
#46591=CARTESIAN_POINT('',(-50.5,7.38871231397104,7.63528357963034));
#46592=CARTESIAN_POINT('Origin',(-50.5,0.,0.));
#46593=CARTESIAN_POINT('Ctrl Pts',(-50.5,7.38871231397104,7.63528357963034));
#46594=CARTESIAN_POINT('Ctrl Pts',(-55.5,7.38871231397104,7.63528357963034));
#46595=CARTESIAN_POINT('Ctrl Pts',(-60.5,7.38871231397104,7.63528357963034));
#46596=CARTESIAN_POINT('Ctrl Pts',(-65.5,7.38871231397104,7.63528357963034));
#46597=CARTESIAN_POINT('Origin',(-50.25,0.,0.));
#46598=CARTESIAN_POINT('',(-50.,7.25553947328138,7.0620657000382));
#46599=CARTESIAN_POINT('Origin',(-50.,0.,0.));
#46600=CARTESIAN_POINT('Ctrl Pts',(-50.,7.25553947328138,7.0620657000382));
#46601=CARTESIAN_POINT('Ctrl Pts',(-50.1688817645172,7.30991422841014,7.24832985268443));
#46602=CARTESIAN_POINT('Ctrl Pts',(-50.3357082640003,7.35411196707409,7.4401437828864));
#46603=CARTESIAN_POINT('Ctrl Pts',(-50.5,7.38871231397104,7.63528357963035));
#46604=CARTESIAN_POINT('Origin',(-66.,7.39276378738951,5.97575774334076));
#46605=CARTESIAN_POINT('',(-66.,8.9522239671058,4.73004345041105));
#46606=CARTESIAN_POINT('Origin',(-66.,0.,0.));
#46607=CARTESIAN_POINT('',(-66.,5.86935629366619,5.15614322415515));
#46608=CARTESIAN_POINT('Ctrl Pts',(-66.,5.86935629366619,5.15614322415516));
#46609=CARTESIAN_POINT('Ctrl Pts',(-66.,5.88381954563966,5.17005841220104));
#46610=CARTESIAN_POINT('Ctrl Pts',(-66.,5.91287960105941,5.19773840582942));
#46611=CARTESIAN_POINT('Ctrl Pts',(-66.,5.95687034761592,5.23880723822028));
#46612=CARTESIAN_POINT('Ctrl Pts',(-66.,6.01632699142066,5.29266225703943));
#46613=CARTESIAN_POINT('Ctrl Pts',(-66.,6.09193876408314,5.35852767967753));
#46614=CARTESIAN_POINT('Ctrl Pts',(-66.,6.16869039722735,5.42311090855867));
#46615=CARTESIAN_POINT('Ctrl Pts',(-66.,6.24627343312988,5.48676114432161));
#46616=CARTESIAN_POINT('Ctrl Pts',(-66.,6.32415927444501,5.55007704717236));
#46617=CARTESIAN_POINT('Ctrl Pts',(-66.,6.40156231993997,5.61394745203258));
#46618=CARTESIAN_POINT('Ctrl Pts',(-66.,6.47757568301991,5.67938854851998));
#46619=CARTESIAN_POINT('Ctrl Pts',(-66.,6.5512916889966,5.74739860249896));
#46620=CARTESIAN_POINT('Ctrl Pts',(-66.,6.6219207121214,5.81881539913394));
#46621=CARTESIAN_POINT('Ctrl Pts',(-66.,6.68892903392674,5.89414917887782));
#46622=CARTESIAN_POINT('Ctrl Pts',(-66.,6.75211401720195,5.97349548879327));
#46623=CARTESIAN_POINT('Ctrl Pts',(-66.,6.81150347103307,6.0566711933897));
#46624=CARTESIAN_POINT('Ctrl Pts',(-66.,6.86728736323967,6.14331014063223));
#46625=CARTESIAN_POINT('Ctrl Pts',(-66.,6.91974169989968,6.23296752615852));
#46626=CARTESIAN_POINT('Ctrl Pts',(-66.,6.96914833844732,6.3252330736069));
#46627=CARTESIAN_POINT('Ctrl Pts',(-66.,7.0157466000915,6.41979281054442));
#46628=CARTESIAN_POINT('Ctrl Pts',(-66.,7.05974191915822,6.51640051406571));
#46629=CARTESIAN_POINT('Ctrl Pts',(-66.,7.10130101698719,6.61487018507936));
#46630=CARTESIAN_POINT('Ctrl Pts',(-66.,7.14055312818317,6.71506051373632));
#46631=CARTESIAN_POINT('Ctrl Pts',(-66.,7.17758748640133,6.81686192205253));
#46632=CARTESIAN_POINT('Ctrl Pts',(-66.,7.2079082107772,6.90670735924895));
#46633=CARTESIAN_POINT('Ctrl Pts',(-66.,7.23005678198432,6.97670057921104));
#46634=CARTESIAN_POINT('Ctrl Pts',(-66.,7.24500218612944,7.02617245622325));
#46635=CARTESIAN_POINT('Ctrl Pts',(-66.,7.25338844488451,7.05469721661769));
#46636=CARTESIAN_POINT('Ctrl Pts',(-66.,7.25553947328137,7.06206570003819));
#46637=CARTESIAN_POINT('',(-66.,6.71751445306827,3.98875366785402));
#46638=CARTESIAN_POINT('Origin',(-66.,0.,0.));
#46639=CARTESIAN_POINT('Ctrl Pts',(-66.,8.9522239671058,4.73004345041105));
#46640=CARTESIAN_POINT('Ctrl Pts',(-66.,8.93239021764327,4.73153264123973));
#46641=CARTESIAN_POINT('Ctrl Pts',(-66.,8.88591271637064,4.73424043504303));
#46642=CARTESIAN_POINT('Ctrl Pts',(-66.,8.81469492241586,4.73547515111526));
#46643=CARTESIAN_POINT('Ctrl Pts',(-66.,8.72137415303495,4.73136123945916));
#46644=CARTESIAN_POINT('Ctrl Pts',(-66.,8.6067054620435,4.7198743383383));
#46645=CARTESIAN_POINT('Ctrl Pts',(-66.,8.48525643213848,4.70566442850842));
#46646=CARTESIAN_POINT('Ctrl Pts',(-66.,8.36143328450034,4.69185659911854));
#46647=CARTESIAN_POINT('Ctrl Pts',(-66.,8.23569494212978,4.67782026347397));
#46648=CARTESIAN_POINT('Ctrl Pts',(-66.,8.10981690611934,4.66138555268912));
#46649=CARTESIAN_POINT('Ctrl Pts',(-66.,7.98612375397626,4.63975306799096));
#46650=CARTESIAN_POINT('Ctrl Pts',(-66.,7.86637497053616,4.61080556997054));
#46651=CARTESIAN_POINT('Ctrl Pts',(-66.,7.75120579898901,4.57378192723342));
#46652=CARTESIAN_POINT('Ctrl Pts',(-66.,7.6405197035065,4.52886501948474));
#46653=CARTESIAN_POINT('Ctrl Pts',(-66.,7.53368133093183,4.476993833765));
#46654=CARTESIAN_POINT('Ctrl Pts',(-66.,7.42979527874749,4.41958894930823));
#46655=CARTESIAN_POINT('Ctrl Pts',(-66.,7.32791448753526,4.35832808183351));
#46656=CARTESIAN_POINT('Ctrl Pts',(-66.,7.22711161240614,4.29494540516727));
#46657=CARTESIAN_POINT('Ctrl Pts',(-66.,7.12656402515112,4.23103749131175));
#46658=CARTESIAN_POINT('Ctrl Pts',(-66.,7.02563860180952,4.1678561402315));
#46659=CARTESIAN_POINT('Ctrl Pts',(-66.,6.92396448304503,4.10613397949206));
#46660=CARTESIAN_POINT('Ctrl Pts',(-66.,6.84187937648697,4.05821392716855));
#46661=CARTESIAN_POINT('Ctrl Pts',(-66.,6.77986998456097,4.02314530770572));
#46662=CARTESIAN_POINT('Ctrl Pts',(-66.,6.73833259489066,4.00015307569533));
#46663=CARTESIAN_POINT('Ctrl Pts',(-66.,6.71751445306827,3.98875366785402));
#46664=CARTESIAN_POINT('Ctrl Pts',(-66.,6.71751445306827,3.98875366785402));
#46665=CARTESIAN_POINT('Ctrl Pts',(-50.,6.71751445306827,3.98875366785402));
#46666=CARTESIAN_POINT('Ctrl Pts',(-66.,6.73833259489066,4.00015307569533));
#46667=CARTESIAN_POINT('Ctrl Pts',(-50.,6.73833259489066,4.00015307569533));
#46668=CARTESIAN_POINT('Ctrl Pts',(-66.,6.77986998456097,4.02314530770572));
#46669=CARTESIAN_POINT('Ctrl Pts',(-50.,6.77986998456097,4.02314530770572));
#46670=CARTESIAN_POINT('Ctrl Pts',(-66.,6.84187937648697,4.05821392716855));
#46671=CARTESIAN_POINT('Ctrl Pts',(-50.,6.84187937648697,4.05821392716855));
#46672=CARTESIAN_POINT('Ctrl Pts',(-66.,6.92396448304503,4.10613397949206));
#46673=CARTESIAN_POINT('Ctrl Pts',(-50.,6.92396448304503,4.10613397949206));
#46674=CARTESIAN_POINT('Ctrl Pts',(-66.,7.02563860180952,4.1678561402315));
#46675=CARTESIAN_POINT('Ctrl Pts',(-50.,7.02563860180952,4.1678561402315));
#46676=CARTESIAN_POINT('Ctrl Pts',(-66.,7.12656402515112,4.23103749131175));
#46677=CARTESIAN_POINT('Ctrl Pts',(-50.,7.12656402515112,4.23103749131175));
#46678=CARTESIAN_POINT('Ctrl Pts',(-66.,7.22711161240614,4.29494540516727));
#46679=CARTESIAN_POINT('Ctrl Pts',(-50.,7.22711161240614,4.29494540516727));
#46680=CARTESIAN_POINT('Ctrl Pts',(-66.,7.32791448753526,4.35832808183351));
#46681=CARTESIAN_POINT('Ctrl Pts',(-50.,7.32791448753526,4.35832808183351));
#46682=CARTESIAN_POINT('Ctrl Pts',(-66.,7.42979527874749,4.41958894930823));
#46683=CARTESIAN_POINT('Ctrl Pts',(-50.,7.42979527874749,4.41958894930823));
#46684=CARTESIAN_POINT('Ctrl Pts',(-66.,7.53368133093183,4.476993833765));
#46685=CARTESIAN_POINT('Ctrl Pts',(-50.,7.53368133093183,4.476993833765));
#46686=CARTESIAN_POINT('Ctrl Pts',(-66.,7.6405197035065,4.52886501948474));
#46687=CARTESIAN_POINT('Ctrl Pts',(-50.,7.6405197035065,4.52886501948474));
#46688=CARTESIAN_POINT('Ctrl Pts',(-66.,7.75120579898901,4.57378192723342));
#46689=CARTESIAN_POINT('Ctrl Pts',(-50.,7.75120579898901,4.57378192723342));
#46690=CARTESIAN_POINT('Ctrl Pts',(-66.,7.86637497053616,4.61080556997054));
#46691=CARTESIAN_POINT('Ctrl Pts',(-50.,7.86637497053616,4.61080556997054));
#46692=CARTESIAN_POINT('Ctrl Pts',(-66.,7.98612375397626,4.63975306799096));
#46693=CARTESIAN_POINT('Ctrl Pts',(-50.,7.98612375397626,4.63975306799096));
#46694=CARTESIAN_POINT('Ctrl Pts',(-66.,8.10981690611934,4.66138555268912));
#46695=CARTESIAN_POINT('Ctrl Pts',(-50.,8.10981690611934,4.66138555268912));
#46696=CARTESIAN_POINT('Ctrl Pts',(-66.,8.23569494212978,4.67782026347397));
#46697=CARTESIAN_POINT('Ctrl Pts',(-50.,8.23569494212978,4.67782026347397));
#46698=CARTESIAN_POINT('Ctrl Pts',(-66.,8.36143328450034,4.69185659911854));
#46699=CARTESIAN_POINT('Ctrl Pts',(-50.,8.36143328450034,4.69185659911854));
#46700=CARTESIAN_POINT('Ctrl Pts',(-66.,8.48525643213848,4.70566442850842));
#46701=CARTESIAN_POINT('Ctrl Pts',(-50.,8.48525643213848,4.70566442850842));
#46702=CARTESIAN_POINT('Ctrl Pts',(-66.,8.6067054620435,4.7198743383383));
#46703=CARTESIAN_POINT('Ctrl Pts',(-50.,8.6067054620435,4.7198743383383));
#46704=CARTESIAN_POINT('Ctrl Pts',(-66.,8.72796083967823,4.73202105878326));
#46705=CARTESIAN_POINT('Ctrl Pts',(-50.,8.72796083967823,4.73202105878326));
#46706=CARTESIAN_POINT('Ctrl Pts',(-66.,8.85339313547798,4.73705510013294));
#46707=CARTESIAN_POINT('Ctrl Pts',(-50.,8.85339313547798,4.73705510013294));
#46708=CARTESIAN_POINT('Ctrl Pts',(-66.,8.98705564961503,4.7302562506624));
#46709=CARTESIAN_POINT('Ctrl Pts',(-50.,8.98705564961503,4.7302562506624));
#46710=CARTESIAN_POINT('Ctrl Pts',(-66.,9.13083440990634,4.70938113162593));
#46711=CARTESIAN_POINT('Ctrl Pts',(-50.,9.13083440990634,4.70938113162593));
#46712=CARTESIAN_POINT('Ctrl Pts',(-66.,9.28205231015641,4.67744454272398));
#46713=CARTESIAN_POINT('Ctrl Pts',(-50.,9.28205231015641,4.67744454272398));
#46714=CARTESIAN_POINT('Ctrl Pts',(-66.,9.43209170831184,4.64432174792964));
#46715=CARTESIAN_POINT('Ctrl Pts',(-50.,9.43209170831184,4.64432174792964));
#46716=CARTESIAN_POINT('Ctrl Pts',(-66.,9.56884308464813,4.62392482004402));
#46717=CARTESIAN_POINT('Ctrl Pts',(-50.,9.56884308464813,4.62392482004402));
#46718=CARTESIAN_POINT('Ctrl Pts',(-66.,9.6786259001787,4.63198987040163));
#46719=CARTESIAN_POINT('Ctrl Pts',(-50.,9.6786259001787,4.63198987040163));
#46720=CARTESIAN_POINT('Ctrl Pts',(-66.,9.74822876312235,4.68372599634944));
#46721=CARTESIAN_POINT('Ctrl Pts',(-50.,9.74822876312235,4.68372599634944));
#46722=CARTESIAN_POINT('Ctrl Pts',(-66.,9.7670979254493,4.79129438302231));
#46723=CARTESIAN_POINT('Ctrl Pts',(-50.,9.7670979254493,4.79129438302231));
#46724=CARTESIAN_POINT('Ctrl Pts',(-66.,9.72722453283275,4.96393510772457));
#46725=CARTESIAN_POINT('Ctrl Pts',(-50.,9.72722453283275,4.96393510772457));
#46726=CARTESIAN_POINT('Ctrl Pts',(-66.,9.62270607610076,5.20846913094059));
#46727=CARTESIAN_POINT('Ctrl Pts',(-50.,9.62270607610076,5.20846913094059));
#46728=CARTESIAN_POINT('Ctrl Pts',(-66.,9.4494426466907,5.52964537209809));
#46729=CARTESIAN_POINT('Ctrl Pts',(-50.,9.4494426466907,5.52964537209809));
#46730=CARTESIAN_POINT('Ctrl Pts',(-66.,9.20479447534083,5.93053256419968));
#46731=CARTESIAN_POINT('Ctrl Pts',(-50.,9.20479447534083,5.93053256419968));
#46732=CARTESIAN_POINT('Ctrl Pts',(-66.,8.88727303370654,6.41287268812632));
#46733=CARTESIAN_POINT('Ctrl Pts',(-50.,8.88727303370654,6.41287268812632));
#46734=CARTESIAN_POINT('Ctrl Pts',(-66.,8.49623316568549,6.97743341853195));
#46735=CARTESIAN_POINT('Ctrl Pts',(-50.,8.49623316568549,6.97743341853195));
#46736=CARTESIAN_POINT('Ctrl Pts',(-66.,8.12450963002148,7.49496283424254));
#46737=CARTESIAN_POINT('Ctrl Pts',(-50.,8.12450963002148,7.49496283424254));
#46738=CARTESIAN_POINT('Ctrl Pts',(-66.,7.81266471007362,7.92008819074951));
#46739=CARTESIAN_POINT('Ctrl Pts',(-50.,7.81266471007362,7.92008819074951));
#46740=CARTESIAN_POINT('Ctrl Pts',(-66.,7.59009772798531,8.21991804475996));
#46741=CARTESIAN_POINT('Ctrl Pts',(-50.,7.59009772798531,8.21991804475996));
#46742=CARTESIAN_POINT('Ctrl Pts',(-66.,7.47514664369958,8.37393621036051));
#46743=CARTESIAN_POINT('Ctrl Pts',(-50.,7.47514664369958,8.37393621036051));
#46744=CARTESIAN_POINT('',(-65.5,9.56265294797246,4.6310143161767));
#46745=CARTESIAN_POINT('Ctrl Pts',(-66.,8.9522239671058,4.73004345041105));
#46746=CARTESIAN_POINT('Ctrl Pts',(-65.7982417703063,9.18983991158661,4.71220237170136));
#46747=CARTESIAN_POINT('Ctrl Pts',(-65.6331946192803,9.4118184657459,4.63688451531894));
#46748=CARTESIAN_POINT('Ctrl Pts',(-65.5,9.56265294797246,4.6310143161767));
#46749=CARTESIAN_POINT('',(-50.,6.71751445306827,3.98875366785402));
#46750=CARTESIAN_POINT('',(-66.,6.71751445306827,3.98875366785402));
#46751=CARTESIAN_POINT('',(-50.,8.95222396710582,4.73004345041105));
#46752=CARTESIAN_POINT('Ctrl Pts',(-50.,6.71751445306827,3.98875366785402));
#46753=CARTESIAN_POINT('Ctrl Pts',(-50.,6.73833259489066,4.00015307569533));
#46754=CARTESIAN_POINT('Ctrl Pts',(-50.,6.77986998456097,4.02314530770572));
#46755=CARTESIAN_POINT('Ctrl Pts',(-50.,6.84187937648697,4.05821392716855));
#46756=CARTESIAN_POINT('Ctrl Pts',(-50.,6.92396448304503,4.10613397949206));
#46757=CARTESIAN_POINT('Ctrl Pts',(-50.,7.02563860180952,4.1678561402315));
#46758=CARTESIAN_POINT('Ctrl Pts',(-50.,7.12656402515112,4.23103749131175));
#46759=CARTESIAN_POINT('Ctrl Pts',(-50.,7.22711161240614,4.29494540516727));
#46760=CARTESIAN_POINT('Ctrl Pts',(-50.,7.32791448753526,4.35832808183351));
#46761=CARTESIAN_POINT('Ctrl Pts',(-50.,7.42979527874749,4.41958894930823));
#46762=CARTESIAN_POINT('Ctrl Pts',(-50.,7.53368133093183,4.476993833765));
#46763=CARTESIAN_POINT('Ctrl Pts',(-50.,7.6405197035065,4.52886501948474));
#46764=CARTESIAN_POINT('Ctrl Pts',(-50.,7.75120579898901,4.57378192723342));
#46765=CARTESIAN_POINT('Ctrl Pts',(-50.,7.86637497053616,4.61080556997054));
#46766=CARTESIAN_POINT('Ctrl Pts',(-50.,7.98612375397626,4.63975306799096));
#46767=CARTESIAN_POINT('Ctrl Pts',(-50.,8.10981690611934,4.66138555268912));
#46768=CARTESIAN_POINT('Ctrl Pts',(-50.,8.23569494212978,4.67782026347397));
#46769=CARTESIAN_POINT('Ctrl Pts',(-50.,8.36143328450034,4.69185659911854));
#46770=CARTESIAN_POINT('Ctrl Pts',(-50.,8.48525643213848,4.70566442850842));
#46771=CARTESIAN_POINT('Ctrl Pts',(-50.,8.6067054620435,4.7198743383383));
#46772=CARTESIAN_POINT('Ctrl Pts',(-50.,8.72137415303496,4.73136123945916));
#46773=CARTESIAN_POINT('Ctrl Pts',(-50.,8.81469492241586,4.73547515111526));
#46774=CARTESIAN_POINT('Ctrl Pts',(-50.,8.88591271637065,4.73424043504303));
#46775=CARTESIAN_POINT('Ctrl Pts',(-50.,8.93239021764329,4.73153264123973));
#46776=CARTESIAN_POINT('Ctrl Pts',(-50.,8.95222396710582,4.73004345041105));
#46777=CARTESIAN_POINT('',(-50.5,9.56265294797246,4.6310143161767));
#46778=CARTESIAN_POINT('Ctrl Pts',(-50.5,9.56265294797247,4.6310143161767));
#46779=CARTESIAN_POINT('Ctrl Pts',(-50.4982567069791,9.56067877888363,4.63109114718723));
#46780=CARTESIAN_POINT('Ctrl Pts',(-50.4965113438742,9.55869681884698,4.63117903647081));
#46781=CARTESIAN_POINT('Ctrl Pts',(-50.3581212730752,9.40112969752826,4.63898530076718));
#46782=CARTESIAN_POINT('Ctrl Pts',(-50.2022201285446,9.19038390194521,4.71216152690525));
#46783=CARTESIAN_POINT('Ctrl Pts',(-50.,8.95222396710582,4.73004345041105));
#46784=CARTESIAN_POINT('Ctrl Pts',(-65.5,9.56265294797246,4.6310143161767));
#46785=CARTESIAN_POINT('Ctrl Pts',(-60.5,9.56265294797246,4.6310143161767));
#46786=CARTESIAN_POINT('Ctrl Pts',(-55.5,9.56265294797246,4.6310143161767));
#46787=CARTESIAN_POINT('Ctrl Pts',(-50.5,9.56265294797246,4.6310143161767));
#46788=CARTESIAN_POINT('Origin',(-66.,0.,0.));
#46789=CARTESIAN_POINT('',(-50.,5.86935629366619,5.15614322415515));
#46790=CARTESIAN_POINT('',(-66.,5.86935629366619,5.15614322415515));
#46791=CARTESIAN_POINT('Origin',(-50.,0.,0.));
#46792=CARTESIAN_POINT('Ctrl Pts',(-66.,7.47514664369958,8.37393621036051));
#46793=CARTESIAN_POINT('Ctrl Pts',(-50.,7.47514664369958,8.37393621036051));
#46794=CARTESIAN_POINT('Ctrl Pts',(-66.,7.47370529227588,8.35029027263347));
#46795=CARTESIAN_POINT('Ctrl Pts',(-50.,7.47370529227588,8.35029027263347));
#46796=CARTESIAN_POINT('Ctrl Pts',(-66.,7.47062843861794,8.30308721200087));
#46797=CARTESIAN_POINT('Ctrl Pts',(-50.,7.47062843861794,8.30308721200087));
#46798=CARTESIAN_POINT('Ctrl Pts',(-66.,7.46543070582113,8.2325490657425));
#46799=CARTESIAN_POINT('Ctrl Pts',(-50.,7.46543070582113,8.2325490657425));
#46800=CARTESIAN_POINT('Ctrl Pts',(-66.,7.45733394062932,8.13903180010481));
#46801=CARTESIAN_POINT('Ctrl Pts',(-50.,7.45733394062932,8.13903180010481));
#46802=CARTESIAN_POINT('Ctrl Pts',(-66.,7.44525825818761,8.02303174355991));
#46803=CARTESIAN_POINT('Ctrl Pts',(-50.,7.44525825818761,8.02303174355991));
#46804=CARTESIAN_POINT('Ctrl Pts',(-66.,7.43121157962414,7.90794262086832));
#46805=CARTESIAN_POINT('Ctrl Pts',(-50.,7.43121157962414,7.90794262086832));
#46806=CARTESIAN_POINT('Ctrl Pts',(-66.,7.41517326521556,7.79378791238727));
#46807=CARTESIAN_POINT('Ctrl Pts',(-50.,7.41517326521556,7.79378791238727));
#46808=CARTESIAN_POINT('Ctrl Pts',(-66.,7.39711971700079,7.68060169938963));
#46809=CARTESIAN_POINT('Ctrl Pts',(-50.,7.39711971700079,7.68060169938963));
#46810=CARTESIAN_POINT('Ctrl Pts',(-66.,7.3770259499153,7.56843089945469));
#46811=CARTESIAN_POINT('Ctrl Pts',(-50.,7.3770259499153,7.56843089945469));
#46812=CARTESIAN_POINT('Ctrl Pts',(-66.,7.35486716320729,7.45733266277773));
#46813=CARTESIAN_POINT('Ctrl Pts',(-50.,7.35486716320729,7.45733266277773));
#46814=CARTESIAN_POINT('Ctrl Pts',(-66.,7.33062026541981,7.34737064045104));
#46815=CARTESIAN_POINT('Ctrl Pts',(-50.,7.33062026541981,7.34737064045104));
#46816=CARTESIAN_POINT('Ctrl Pts',(-66.,7.30426596664335,7.23861130630728));
#46817=CARTESIAN_POINT('Ctrl Pts',(-50.,7.30426596664335,7.23861130630728));
#46818=CARTESIAN_POINT('Ctrl Pts',(-66.,7.27579018934611,7.13112071115277));
#46819=CARTESIAN_POINT('Ctrl Pts',(-50.,7.27579018934611,7.13112071115277));
#46820=CARTESIAN_POINT('Ctrl Pts',(-66.,7.24518783030335,7.02495948896872));
#46821=CARTESIAN_POINT('Ctrl Pts',(-50.,7.24518783030335,7.02495948896872));
#46822=CARTESIAN_POINT('Ctrl Pts',(-66.,7.21245683723339,6.92018570915688));
#46823=CARTESIAN_POINT('Ctrl Pts',(-50.,7.21245683723339,6.92018570915688));
#46824=CARTESIAN_POINT('Ctrl Pts',(-66.,7.17758748640133,6.81686192205253));
#46825=CARTESIAN_POINT('Ctrl Pts',(-50.,7.17758748640133,6.81686192205253));
#46826=CARTESIAN_POINT('Ctrl Pts',(-66.,7.14055312818317,6.71506051373632));
#46827=CARTESIAN_POINT('Ctrl Pts',(-50.,7.14055312818317,6.71506051373632));
#46828=CARTESIAN_POINT('Ctrl Pts',(-66.,7.10130101698719,6.61487018507936));
#46829=CARTESIAN_POINT('Ctrl Pts',(-50.,7.10130101698719,6.61487018507936));
#46830=CARTESIAN_POINT('Ctrl Pts',(-66.,7.05974191915822,6.51640051406571));
#46831=CARTESIAN_POINT('Ctrl Pts',(-50.,7.05974191915822,6.51640051406571));
#46832=CARTESIAN_POINT('Ctrl Pts',(-66.,7.0157466000915,6.41979281054442));
#46833=CARTESIAN_POINT('Ctrl Pts',(-50.,7.0157466000915,6.41979281054442));
#46834=CARTESIAN_POINT('Ctrl Pts',(-66.,6.96914833844732,6.3252330736069));
#46835=CARTESIAN_POINT('Ctrl Pts',(-50.,6.96914833844732,6.3252330736069));
#46836=CARTESIAN_POINT('Ctrl Pts',(-66.,6.91974169989968,6.23296752615852));
#46837=CARTESIAN_POINT('Ctrl Pts',(-50.,6.91974169989968,6.23296752615852));
#46838=CARTESIAN_POINT('Ctrl Pts',(-66.,6.86728736323967,6.14331014063223));
#46839=CARTESIAN_POINT('Ctrl Pts',(-50.,6.86728736323967,6.14331014063223));
#46840=CARTESIAN_POINT('Ctrl Pts',(-66.,6.81150347103307,6.0566711933897));
#46841=CARTESIAN_POINT('Ctrl Pts',(-50.,6.81150347103307,6.0566711933897));
#46842=CARTESIAN_POINT('Ctrl Pts',(-66.,6.75211401720195,5.97349548879327));
#46843=CARTESIAN_POINT('Ctrl Pts',(-50.,6.75211401720195,5.97349548879327));
#46844=CARTESIAN_POINT('Ctrl Pts',(-66.,6.68892903392674,5.89414917887782));
#46845=CARTESIAN_POINT('Ctrl Pts',(-50.,6.68892903392674,5.89414917887782));
#46846=CARTESIAN_POINT('Ctrl Pts',(-66.,6.6219207121214,5.81881539913394));
#46847=CARTESIAN_POINT('Ctrl Pts',(-50.,6.6219207121214,5.81881539913394));
#46848=CARTESIAN_POINT('Ctrl Pts',(-66.,6.5512916889966,5.74739860249896));
#46849=CARTESIAN_POINT('Ctrl Pts',(-50.,6.5512916889966,5.74739860249896));
#46850=CARTESIAN_POINT('Ctrl Pts',(-66.,6.47757568301991,5.67938854851998));
#46851=CARTESIAN_POINT('Ctrl Pts',(-50.,6.47757568301991,5.67938854851998));
#46852=CARTESIAN_POINT('Ctrl Pts',(-66.,6.40156231993997,5.61394745203258));
#46853=CARTESIAN_POINT('Ctrl Pts',(-50.,6.40156231993997,5.61394745203258));
#46854=CARTESIAN_POINT('Ctrl Pts',(-66.,6.32415927444501,5.55007704717236));
#46855=CARTESIAN_POINT('Ctrl Pts',(-50.,6.32415927444501,5.55007704717236));
#46856=CARTESIAN_POINT('Ctrl Pts',(-66.,6.24627343312988,5.48676114432161));
#46857=CARTESIAN_POINT('Ctrl Pts',(-50.,6.24627343312988,5.48676114432161));
#46858=CARTESIAN_POINT('Ctrl Pts',(-66.,6.16869039722735,5.42311090855867));
#46859=CARTESIAN_POINT('Ctrl Pts',(-50.,6.16869039722735,5.42311090855867));
#46860=CARTESIAN_POINT('Ctrl Pts',(-66.,6.09193876408314,5.35852767967753));
#46861=CARTESIAN_POINT('Ctrl Pts',(-50.,6.09193876408314,5.35852767967753));
#46862=CARTESIAN_POINT('Ctrl Pts',(-66.,6.01632699142066,5.29266225703943));
#46863=CARTESIAN_POINT('Ctrl Pts',(-50.,6.01632699142066,5.29266225703943));
#46864=CARTESIAN_POINT('Ctrl Pts',(-66.,5.95687034761592,5.23880723822028));
#46865=CARTESIAN_POINT('Ctrl Pts',(-50.,5.95687034761592,5.23880723822028));
#46866=CARTESIAN_POINT('Ctrl Pts',(-66.,5.91287960105941,5.19773840582942));
#46867=CARTESIAN_POINT('Ctrl Pts',(-50.,5.91287960105941,5.19773840582942));
#46868=CARTESIAN_POINT('Ctrl Pts',(-66.,5.88381954563966,5.17005841220104));
#46869=CARTESIAN_POINT('Ctrl Pts',(-50.,5.88381954563966,5.17005841220104));
#46870=CARTESIAN_POINT('Ctrl Pts',(-66.,5.86935629366619,5.15614322415516));
#46871=CARTESIAN_POINT('Ctrl Pts',(-50.,5.86935629366619,5.15614322415516));
#46872=CARTESIAN_POINT('Ctrl Pts',(-50.,7.25553947328138,7.0620657000382));
#46873=CARTESIAN_POINT('Ctrl Pts',(-50.,7.25338844488451,7.0546972166177));
#46874=CARTESIAN_POINT('Ctrl Pts',(-50.,7.24500218612945,7.02617245622326));
#46875=CARTESIAN_POINT('Ctrl Pts',(-50.,7.23005678198432,6.97670057921104));
#46876=CARTESIAN_POINT('Ctrl Pts',(-50.,7.2079082107772,6.90670735924896));
#46877=CARTESIAN_POINT('Ctrl Pts',(-50.,7.17758748640133,6.81686192205253));
#46878=CARTESIAN_POINT('Ctrl Pts',(-50.,7.14055312818317,6.71506051373632));
#46879=CARTESIAN_POINT('Ctrl Pts',(-50.,7.10130101698719,6.61487018507936));
#46880=CARTESIAN_POINT('Ctrl Pts',(-50.,7.05974191915822,6.51640051406571));
#46881=CARTESIAN_POINT('Ctrl Pts',(-50.,7.0157466000915,6.41979281054442));
#46882=CARTESIAN_POINT('Ctrl Pts',(-50.,6.96914833844732,6.3252330736069));
#46883=CARTESIAN_POINT('Ctrl Pts',(-50.,6.91974169989968,6.23296752615852));
#46884=CARTESIAN_POINT('Ctrl Pts',(-50.,6.86728736323967,6.14331014063223));
#46885=CARTESIAN_POINT('Ctrl Pts',(-50.,6.81150347103307,6.0566711933897));
#46886=CARTESIAN_POINT('Ctrl Pts',(-50.,6.75211401720195,5.97349548879327));
#46887=CARTESIAN_POINT('Ctrl Pts',(-50.,6.68892903392674,5.89414917887782));
#46888=CARTESIAN_POINT('Ctrl Pts',(-50.,6.6219207121214,5.81881539913394));
#46889=CARTESIAN_POINT('Ctrl Pts',(-50.,6.5512916889966,5.74739860249896));
#46890=CARTESIAN_POINT('Ctrl Pts',(-50.,6.47757568301991,5.67938854851998));
#46891=CARTESIAN_POINT('Ctrl Pts',(-50.,6.40156231993997,5.61394745203258));
#46892=CARTESIAN_POINT('Ctrl Pts',(-50.,6.32415927444501,5.55007704717236));
#46893=CARTESIAN_POINT('Ctrl Pts',(-50.,6.24627343312988,5.48676114432161));
#46894=CARTESIAN_POINT('Ctrl Pts',(-50.,6.16869039722735,5.42311090855867));
#46895=CARTESIAN_POINT('Ctrl Pts',(-50.,6.09193876408314,5.35852767967753));
#46896=CARTESIAN_POINT('Ctrl Pts',(-50.,6.01632699142066,5.29266225703943));
#46897=CARTESIAN_POINT('Ctrl Pts',(-50.,5.95687034761592,5.23880723822028));
#46898=CARTESIAN_POINT('Ctrl Pts',(-50.,5.91287960105941,5.19773840582942));
#46899=CARTESIAN_POINT('Ctrl Pts',(-50.,5.88381954563966,5.17005841220104));
#46900=CARTESIAN_POINT('Ctrl Pts',(-50.,5.86935629366619,5.15614322415516));
#46901=CARTESIAN_POINT('Origin',(-50.,7.39276378738951,5.97575774334076));
#46902=CARTESIAN_POINT('Origin',(-50.,0.,0.));
#46903=CARTESIAN_POINT('Origin',(-65.75,0.,0.));
#46904=CARTESIAN_POINT('',(-65.5,9.85547418436682,3.96991858874703));
#46905=CARTESIAN_POINT('Origin',(-65.5,0.,0.));
#46906=CARTESIAN_POINT('',(-66.,9.50066602457707,3.50042427277708));
#46907=CARTESIAN_POINT('Ctrl Pts',(-65.5,9.85547418436681,3.96991858874702));
#46908=CARTESIAN_POINT('Ctrl Pts',(-65.6642917360003,9.74449468876773,3.80572274277181));
#46909=CARTESIAN_POINT('Ctrl Pts',(-65.8311182354839,9.62610029130724,3.64846883797855));
#46910=CARTESIAN_POINT('Ctrl Pts',(-66.,9.50066602457707,3.50042427277707));
#46911=CARTESIAN_POINT('Origin',(-66.,0.,0.));
#46912=CARTESIAN_POINT('Origin',(-58.,0.,0.));
#46913=CARTESIAN_POINT('',(-50.5,9.85547418436682,3.96991858874703));
#46914=CARTESIAN_POINT('Origin',(-50.5,0.,0.));
#46915=CARTESIAN_POINT('Ctrl Pts',(-50.5,9.85547418436682,3.96991858874703));
#46916=CARTESIAN_POINT('Ctrl Pts',(-55.5,9.85547418436682,3.96991858874703));
#46917=CARTESIAN_POINT('Ctrl Pts',(-60.5,9.85547418436682,3.96991858874703));
#46918=CARTESIAN_POINT('Ctrl Pts',(-65.5,9.85547418436682,3.96991858874703));
#46919=CARTESIAN_POINT('Origin',(-50.25,0.,0.));
#46920=CARTESIAN_POINT('',(-50.,9.50066602457708,3.50042427277709));
#46921=CARTESIAN_POINT('Origin',(-50.,0.,0.));
#46922=CARTESIAN_POINT('Ctrl Pts',(-50.,9.50066602457708,3.50042427277709));
#46923=CARTESIAN_POINT('Ctrl Pts',(-50.1688817645154,9.62610029130675,3.64846883797794));
#46924=CARTESIAN_POINT('Ctrl Pts',(-50.335708263999,9.74449468876727,3.80572274277114));
#46925=CARTESIAN_POINT('Ctrl Pts',(-50.5,9.85547418436682,3.96991858874704));
#46926=CARTESIAN_POINT('Ctrl Pts',(-66.,10.234872965097,4.60955533520604));
#46927=CARTESIAN_POINT('Ctrl Pts',(-50.,10.234872965097,4.60955533520604));
#46928=CARTESIAN_POINT('Ctrl Pts',(-66.,10.2239385557175,4.58853994664336));
#46929=CARTESIAN_POINT('Ctrl Pts',(-50.,10.2239385557175,4.58853994664336));
#46930=CARTESIAN_POINT('Ctrl Pts',(-66.,10.2019284956099,4.54666927414369));
#46931=CARTESIAN_POINT('Ctrl Pts',(-50.,10.2019284956099,4.54666927414369));
#46932=CARTESIAN_POINT('Ctrl Pts',(-66.,10.1684896816054,4.48434357942821));
#46933=CARTESIAN_POINT('Ctrl Pts',(-50.,10.1684896816054,4.48434357942821));
#46934=CARTESIAN_POINT('Ctrl Pts',(-66.,10.1230560198477,4.40220455728764));
#46935=CARTESIAN_POINT('Ctrl Pts',(-50.,10.1230560198477,4.40220455728764));
#46936=CARTESIAN_POINT('Ctrl Pts',(-66.,10.0648428614095,4.30114485508394));
#46937=CARTESIAN_POINT('Ctrl Pts',(-50.,10.0648428614095,4.30114485508394));
#46938=CARTESIAN_POINT('Ctrl Pts',(-66.,10.0051996185948,4.20171900871024));
#46939=CARTESIAN_POINT('Ctrl Pts',(-50.,10.0051996185948,4.20171900871024));
#46940=CARTESIAN_POINT('Ctrl Pts',(-66.,9.94411698639968,4.103956863472));
#46941=CARTESIAN_POINT('Ctrl Pts',(-50.,9.94411698639968,4.103956863472));
#46942=CARTESIAN_POINT('Ctrl Pts',(-66.,9.88158726911661,4.00789915231672));
#46943=CARTESIAN_POINT('Ctrl Pts',(-50.,9.88158726911661,4.00789915231672));
#46944=CARTESIAN_POINT('Ctrl Pts',(-66.,9.81760672485207,3.91359889892712));
#46945=CARTESIAN_POINT('Ctrl Pts',(-50.,9.81760672485207,3.91359889892712));
#46946=CARTESIAN_POINT('Ctrl Pts',(-66.,9.75217594207047,3.82111839997903));
#46947=CARTESIAN_POINT('Ctrl Pts',(-50.,9.75217594207047,3.82111839997903));
#46948=CARTESIAN_POINT('Ctrl Pts',(-66.,9.68529971490782,3.73052519578036));
#46949=CARTESIAN_POINT('Ctrl Pts',(-50.,9.68529971490782,3.73052519578036));
#46950=CARTESIAN_POINT('Ctrl Pts',(-66.,9.61698745849843,3.64188785911205));
#46951=CARTESIAN_POINT('Ctrl Pts',(-50.,9.61698745849843,3.64188785911205));
#46952=CARTESIAN_POINT('Ctrl Pts',(-66.,9.54725317766033,3.55527245623621));
#46953=CARTESIAN_POINT('Ctrl Pts',(-50.,9.54725317766033,3.55527245623621));
#46954=CARTESIAN_POINT('Ctrl Pts',(-66.,9.4761168724277,3.47073645471943));
#46955=CARTESIAN_POINT('Ctrl Pts',(-50.,9.4761168724277,3.47073645471943));
#46956=CARTESIAN_POINT('Ctrl Pts',(-66.,9.40360028690147,3.3883337383381));
#46957=CARTESIAN_POINT('Ctrl Pts',(-50.,9.40360028690147,3.3883337383381));
#46958=CARTESIAN_POINT('Ctrl Pts',(-66.,9.3297199795212,3.30812540466615));
#46959=CARTESIAN_POINT('Ctrl Pts',(-50.,9.3297199795212,3.30812540466615));
#46960=CARTESIAN_POINT('Ctrl Pts',(-66.,9.25448104671536,3.23018842105738));
#46961=CARTESIAN_POINT('Ctrl Pts',(-50.,9.25448104671536,3.23018842105738));
#46962=CARTESIAN_POINT('Ctrl Pts',(-66.,9.17787138088281,3.15462527335458));
#46963=CARTESIAN_POINT('Ctrl Pts',(-50.,9.17787138088281,3.15462527335458));
#46964=CARTESIAN_POINT('Ctrl Pts',(-66.,9.09985403240456,3.08157236062471));
#46965=CARTESIAN_POINT('Ctrl Pts',(-50.,9.09985403240456,3.08157236062471));
#46966=CARTESIAN_POINT('Ctrl Pts',(-66.,9.0203684154881,3.01121134028781));
#46967=CARTESIAN_POINT('Ctrl Pts',(-50.,9.0203684154881,3.01121134028781));
#46968=CARTESIAN_POINT('Ctrl Pts',(-66.,8.93933787525693,2.94377994264697));
#46969=CARTESIAN_POINT('Ctrl Pts',(-50.,8.93933787525693,2.94377994264697));
#46970=CARTESIAN_POINT('Ctrl Pts',(-66.,8.85667488599363,2.87958666118713));
#46971=CARTESIAN_POINT('Ctrl Pts',(-50.,8.85667488599363,2.87958666118713));
#46972=CARTESIAN_POINT('Ctrl Pts',(-66.,8.7722885209883,2.81901566470334));
#46973=CARTESIAN_POINT('Ctrl Pts',(-50.,8.7722885209883,2.81901566470334));
#46974=CARTESIAN_POINT('Ctrl Pts',(-66.,8.68608816509229,2.7625564010488));
#46975=CARTESIAN_POINT('Ctrl Pts',(-50.,8.68608816509229,2.7625564010488));
#46976=CARTESIAN_POINT('Ctrl Pts',(-66.,8.59800259243998,2.71072748101388));
#46977=CARTESIAN_POINT('Ctrl Pts',(-50.,8.59800259243998,2.71072748101388));
#46978=CARTESIAN_POINT('Ctrl Pts',(-66.,8.50800718624223,2.66394066800009));
#46979=CARTESIAN_POINT('Ctrl Pts',(-50.,8.50800718624223,2.66394066800009));
#46980=CARTESIAN_POINT('Ctrl Pts',(-66.,8.41615102954947,2.62237457557726));
#46981=CARTESIAN_POINT('Ctrl Pts',(-50.,8.41615102954947,2.62237457557726));
#46982=CARTESIAN_POINT('Ctrl Pts',(-66.,8.32258037817354,2.58585949718149));
#46983=CARTESIAN_POINT('Ctrl Pts',(-50.,8.32258037817354,2.58585949718149));
#46984=CARTESIAN_POINT('Ctrl Pts',(-66.,8.22757527470717,2.55371222210688));
#46985=CARTESIAN_POINT('Ctrl Pts',(-50.,8.22757527470717,2.55371222210688));
#46986=CARTESIAN_POINT('Ctrl Pts',(-66.,8.13151632024086,2.52484622579571));
#46987=CARTESIAN_POINT('Ctrl Pts',(-50.,8.13151632024086,2.52484622579571));
#46988=CARTESIAN_POINT('Ctrl Pts',(-66.,8.0348266855565,2.49798036244632));
#46989=CARTESIAN_POINT('Ctrl Pts',(-50.,8.0348266855565,2.49798036244632));
#46990=CARTESIAN_POINT('Ctrl Pts',(-66.,7.93792153122956,2.47181743264013));
#46991=CARTESIAN_POINT('Ctrl Pts',(-50.,7.93792153122956,2.47181743264013));
#46992=CARTESIAN_POINT('Ctrl Pts',(-66.,7.84115701796548,2.44522591246363));
#46993=CARTESIAN_POINT('Ctrl Pts',(-50.,7.84115701796548,2.44522591246363));
#46994=CARTESIAN_POINT('Ctrl Pts',(-66.,7.74477254642582,2.41744389869504));
#46995=CARTESIAN_POINT('Ctrl Pts',(-50.,7.74477254642582,2.41744389869504));
#46996=CARTESIAN_POINT('Ctrl Pts',(-66.,7.64890787406712,2.38802691961804));
#46997=CARTESIAN_POINT('Ctrl Pts',(-50.,7.64890787406712,2.38802691961804));
#46998=CARTESIAN_POINT('Ctrl Pts',(-66.,7.57268671762535,2.36301110751424));
#46999=CARTESIAN_POINT('Ctrl Pts',(-50.,7.57268671762535,2.36301110751424));
#47000=CARTESIAN_POINT('Ctrl Pts',(-66.,7.51579497190863,2.34338551081368));
#47001=CARTESIAN_POINT('Ctrl Pts',(-50.,7.51579497190863,2.34338551081368));
#47002=CARTESIAN_POINT('Ctrl Pts',(-66.,7.47798882259232,2.32991836775593));
#47003=CARTESIAN_POINT('Ctrl Pts',(-50.,7.47798882259232,2.32991836775593));
#47004=CARTESIAN_POINT('Ctrl Pts',(-66.,7.45911616757566,2.32308894548001));
#47005=CARTESIAN_POINT('Ctrl Pts',(-50.,7.45911616757566,2.32308894548001));
#47006=CARTESIAN_POINT('',(-50.,7.45911616757566,2.32308894548));
#47007=CARTESIAN_POINT('Ctrl Pts',(-50.,9.50066602457708,3.50042427277709));
#47008=CARTESIAN_POINT('Ctrl Pts',(-50.,9.49570393014485,3.49456773028788));
#47009=CARTESIAN_POINT('Ctrl Pts',(-50.,9.47644063626517,3.47192006373319));
#47010=CARTESIAN_POINT('Ctrl Pts',(-50.,9.44266530501315,3.43280409871903));
#47011=CARTESIAN_POINT('Ctrl Pts',(-50.,9.39396277106816,3.37787074605859));
#47012=CARTESIAN_POINT('Ctrl Pts',(-50.,9.3297199795212,3.30812540466615));
#47013=CARTESIAN_POINT('Ctrl Pts',(-50.,9.25448104671536,3.23018842105738));
#47014=CARTESIAN_POINT('Ctrl Pts',(-50.,9.17787138088281,3.15462527335458));
#47015=CARTESIAN_POINT('Ctrl Pts',(-50.,9.09985403240456,3.08157236062471));
#47016=CARTESIAN_POINT('Ctrl Pts',(-50.,9.0203684154881,3.01121134028781));
#47017=CARTESIAN_POINT('Ctrl Pts',(-50.,8.93933787525693,2.94377994264697));
#47018=CARTESIAN_POINT('Ctrl Pts',(-50.,8.85667488599363,2.87958666118713));
#47019=CARTESIAN_POINT('Ctrl Pts',(-50.,8.7722885209883,2.81901566470334));
#47020=CARTESIAN_POINT('Ctrl Pts',(-50.,8.68608816509229,2.7625564010488));
#47021=CARTESIAN_POINT('Ctrl Pts',(-50.,8.59800259243998,2.71072748101388));
#47022=CARTESIAN_POINT('Ctrl Pts',(-50.,8.50800718624223,2.66394066800009));
#47023=CARTESIAN_POINT('Ctrl Pts',(-50.,8.41615102954947,2.62237457557726));
#47024=CARTESIAN_POINT('Ctrl Pts',(-50.,8.32258037817354,2.58585949718149));
#47025=CARTESIAN_POINT('Ctrl Pts',(-50.,8.22757527470717,2.55371222210688));
#47026=CARTESIAN_POINT('Ctrl Pts',(-50.,8.13151632024086,2.52484622579571));
#47027=CARTESIAN_POINT('Ctrl Pts',(-50.,8.0348266855565,2.49798036244632));
#47028=CARTESIAN_POINT('Ctrl Pts',(-50.,7.93792153122956,2.47181743264013));
#47029=CARTESIAN_POINT('Ctrl Pts',(-50.,7.84115701796548,2.44522591246363));
#47030=CARTESIAN_POINT('Ctrl Pts',(-50.,7.74477254642582,2.41744389869504));
#47031=CARTESIAN_POINT('Ctrl Pts',(-50.,7.64890787406712,2.38802691961804));
#47032=CARTESIAN_POINT('Ctrl Pts',(-50.,7.57268671762535,2.36301110751424));
#47033=CARTESIAN_POINT('Ctrl Pts',(-50.,7.51579497190863,2.34338551081368));
#47034=CARTESIAN_POINT('Ctrl Pts',(-50.,7.47798882259232,2.32991836775593));
#47035=CARTESIAN_POINT('Ctrl Pts',(-50.,7.45911616757566,2.32308894548001));
#47036=CARTESIAN_POINT('',(-66.,7.45911616757566,2.32308894548));
#47037=CARTESIAN_POINT('',(-66.,7.45911616757566,2.32308894548));
#47038=CARTESIAN_POINT('Ctrl Pts',(-66.,7.45911616757566,2.32308894548001));
#47039=CARTESIAN_POINT('Ctrl Pts',(-66.,7.47798882259232,2.32991836775593));
#47040=CARTESIAN_POINT('Ctrl Pts',(-66.,7.51579497190863,2.34338551081368));
#47041=CARTESIAN_POINT('Ctrl Pts',(-66.,7.57268671762535,2.36301110751424));
#47042=CARTESIAN_POINT('Ctrl Pts',(-66.,7.64890787406712,2.38802691961804));
#47043=CARTESIAN_POINT('Ctrl Pts',(-66.,7.74477254642582,2.41744389869504));
#47044=CARTESIAN_POINT('Ctrl Pts',(-66.,7.84115701796548,2.44522591246363));
#47045=CARTESIAN_POINT('Ctrl Pts',(-66.,7.93792153122956,2.47181743264013));
#47046=CARTESIAN_POINT('Ctrl Pts',(-66.,8.0348266855565,2.49798036244632));
#47047=CARTESIAN_POINT('Ctrl Pts',(-66.,8.13151632024086,2.52484622579571));
#47048=CARTESIAN_POINT('Ctrl Pts',(-66.,8.22757527470717,2.55371222210688));
#47049=CARTESIAN_POINT('Ctrl Pts',(-66.,8.32258037817354,2.58585949718149));
#47050=CARTESIAN_POINT('Ctrl Pts',(-66.,8.41615102954947,2.62237457557726));
#47051=CARTESIAN_POINT('Ctrl Pts',(-66.,8.50800718624223,2.66394066800009));
#47052=CARTESIAN_POINT('Ctrl Pts',(-66.,8.59800259243998,2.71072748101388));
#47053=CARTESIAN_POINT('Ctrl Pts',(-66.,8.68608816509229,2.7625564010488));
#47054=CARTESIAN_POINT('Ctrl Pts',(-66.,8.7722885209883,2.81901566470334));
#47055=CARTESIAN_POINT('Ctrl Pts',(-66.,8.85667488599363,2.87958666118713));
#47056=CARTESIAN_POINT('Ctrl Pts',(-66.,8.93933787525693,2.94377994264697));
#47057=CARTESIAN_POINT('Ctrl Pts',(-66.,9.0203684154881,3.01121134028781));
#47058=CARTESIAN_POINT('Ctrl Pts',(-66.,9.09985403240456,3.08157236062471));
#47059=CARTESIAN_POINT('Ctrl Pts',(-66.,9.17787138088281,3.15462527335458));
#47060=CARTESIAN_POINT('Ctrl Pts',(-66.,9.25448104671536,3.23018842105738));
#47061=CARTESIAN_POINT('Ctrl Pts',(-66.,9.3297199795212,3.30812540466615));
#47062=CARTESIAN_POINT('Ctrl Pts',(-66.,9.39396277106816,3.37787074605859));
#47063=CARTESIAN_POINT('Ctrl Pts',(-66.,9.44266530501315,3.43280409871902));
#47064=CARTESIAN_POINT('Ctrl Pts',(-66.,9.47644063626516,3.47192006373319));
#47065=CARTESIAN_POINT('Ctrl Pts',(-66.,9.49570393014484,3.49456773028787));
#47066=CARTESIAN_POINT('Ctrl Pts',(-66.,9.50066602457707,3.50042427277708));
#47067=CARTESIAN_POINT('Origin',(-66.,9.18418542175504,2.4522184164664));
#47068=CARTESIAN_POINT('Origin',(-66.,0.,0.));
#47069=CARTESIAN_POINT('',(-66.,7.75912709216827,0.911648516469146));
#47070=CARTESIAN_POINT('Origin',(-66.,0.,0.));
#47071=CARTESIAN_POINT('Ctrl Pts',(-66.,10.1021455355716,0.67991218413181));
#47072=CARTESIAN_POINT('Ctrl Pts',(-66.,10.0846322123206,0.689339740324907));
#47073=CARTESIAN_POINT('Ctrl Pts',(-66.,10.0432742611121,0.710717535900336));
#47074=CARTESIAN_POINT('Ctrl Pts',(-66.,9.97871577321179,0.740812391600032));
#47075=CARTESIAN_POINT('Ctrl Pts',(-66.,9.89178972962324,0.775011122760695));
#47076=CARTESIAN_POINT('Ctrl Pts',(-66.,9.78236252423293,0.811157274859099));
#47077=CARTESIAN_POINT('Ctrl Pts',(-66.,9.66563362360549,0.847573647008884));
#47078=CARTESIAN_POINT('Ctrl Pts',(-66.,9.54689939935545,0.885322978595271));
#47079=CARTESIAN_POINT('Ctrl Pts',(-66.,9.42632261579016,0.923642539206944));
#47080=CARTESIAN_POINT('Ctrl Pts',(-66.,9.3046427086813,0.959827893625642));
#47081=CARTESIAN_POINT('Ctrl Pts',(-66.,9.18284466719198,0.990376172966252));
#47082=CARTESIAN_POINT('Ctrl Pts',(-66.,9.06167470185178,1.01263753582842));
#47083=CARTESIAN_POINT('Ctrl Pts',(-66.,8.94140355616308,1.02565827740144));
#47084=CARTESIAN_POINT('Ctrl Pts',(-66.,8.8220174241358,1.02964473126801));
#47085=CARTESIAN_POINT('Ctrl Pts',(-66.,8.70331780221627,1.02571312618391));
#47086=CARTESIAN_POINT('Ctrl Pts',(-66.,8.58506450113074,1.01552541886979));
#47087=CARTESIAN_POINT('Ctrl Pts',(-66.,8.4670747275092,1.00099948266857));
#47088=CARTESIAN_POINT('Ctrl Pts',(-66.,8.34920666168128,0.984096749349312));
#47089=CARTESIAN_POINT('Ctrl Pts',(-66.,8.23135817971997,0.966610353048665));
#47090=CARTESIAN_POINT('Ctrl Pts',(-66.,8.11346004702223,0.949941384652545));
#47091=CARTESIAN_POINT('Ctrl Pts',(-66.,7.99547145320256,0.934909974827099));
#47092=CARTESIAN_POINT('Ctrl Pts',(-66.,7.90099213574826,0.924519849384913));
#47093=CARTESIAN_POINT('Ctrl Pts',(-66.,7.83008004486546,0.917704563279999));
#47094=CARTESIAN_POINT('Ctrl Pts',(-66.,7.7827819679451,0.913594892602471));
#47095=CARTESIAN_POINT('Ctrl Pts',(-66.,7.75912709216827,0.911648516469146));
#47096=CARTESIAN_POINT('Origin',(-66.,0.,0.));
#47097=CARTESIAN_POINT('',(-50.,7.75912709216827,0.911648516469146));
#47098=CARTESIAN_POINT('Origin',(-50.,0.,0.));
#47099=CARTESIAN_POINT('',(-66.,7.75912709216827,0.911648516469146));
#47100=CARTESIAN_POINT('Ctrl Pts',(-66.,7.75912709216827,0.911648516469146));
#47101=CARTESIAN_POINT('Ctrl Pts',(-50.,7.75912709216827,0.911648516469146));
#47102=CARTESIAN_POINT('Ctrl Pts',(-66.,7.7827819679451,0.913594892602471));
#47103=CARTESIAN_POINT('Ctrl Pts',(-50.,7.7827819679451,0.913594892602471));
#47104=CARTESIAN_POINT('Ctrl Pts',(-66.,7.83008004486546,0.917704563279999));
#47105=CARTESIAN_POINT('Ctrl Pts',(-50.,7.83008004486546,0.917704563279999));
#47106=CARTESIAN_POINT('Ctrl Pts',(-66.,7.90099213574826,0.924519849384913));
#47107=CARTESIAN_POINT('Ctrl Pts',(-50.,7.90099213574826,0.924519849384913));
#47108=CARTESIAN_POINT('Ctrl Pts',(-66.,7.99547145320256,0.934909974827099));
#47109=CARTESIAN_POINT('Ctrl Pts',(-50.,7.99547145320256,0.934909974827099));
#47110=CARTESIAN_POINT('Ctrl Pts',(-66.,8.11346004702223,0.949941384652545));
#47111=CARTESIAN_POINT('Ctrl Pts',(-50.,8.11346004702223,0.949941384652545));
#47112=CARTESIAN_POINT('Ctrl Pts',(-66.,8.23135817971997,0.966610353048665));
#47113=CARTESIAN_POINT('Ctrl Pts',(-50.,8.23135817971997,0.966610353048665));
#47114=CARTESIAN_POINT('Ctrl Pts',(-66.,8.34920666168128,0.984096749349312));
#47115=CARTESIAN_POINT('Ctrl Pts',(-50.,8.34920666168128,0.984096749349312));
#47116=CARTESIAN_POINT('Ctrl Pts',(-66.,8.4670747275092,1.00099948266857));
#47117=CARTESIAN_POINT('Ctrl Pts',(-50.,8.4670747275092,1.00099948266857));
#47118=CARTESIAN_POINT('Ctrl Pts',(-66.,8.58506450113074,1.01552541886979));
#47119=CARTESIAN_POINT('Ctrl Pts',(-50.,8.58506450113074,1.01552541886979));
#47120=CARTESIAN_POINT('Ctrl Pts',(-66.,8.70331780221627,1.02571312618391));
#47121=CARTESIAN_POINT('Ctrl Pts',(-50.,8.70331780221627,1.02571312618391));
#47122=CARTESIAN_POINT('Ctrl Pts',(-66.,8.8220174241358,1.02964473126801));
#47123=CARTESIAN_POINT('Ctrl Pts',(-50.,8.8220174241358,1.02964473126801));
#47124=CARTESIAN_POINT('Ctrl Pts',(-66.,8.94140355616308,1.02565827740144));
#47125=CARTESIAN_POINT('Ctrl Pts',(-50.,8.94140355616308,1.02565827740144));
#47126=CARTESIAN_POINT('Ctrl Pts',(-66.,9.06167470185178,1.01263753582842));
#47127=CARTESIAN_POINT('Ctrl Pts',(-50.,9.06167470185178,1.01263753582842));
#47128=CARTESIAN_POINT('Ctrl Pts',(-66.,9.18284466719198,0.990376172966252));
#47129=CARTESIAN_POINT('Ctrl Pts',(-50.,9.18284466719198,0.990376172966252));
#47130=CARTESIAN_POINT('Ctrl Pts',(-66.,9.3046427086813,0.959827893625642));
#47131=CARTESIAN_POINT('Ctrl Pts',(-50.,9.3046427086813,0.959827893625642));
#47132=CARTESIAN_POINT('Ctrl Pts',(-66.,9.42632261579016,0.923642539206944));
#47133=CARTESIAN_POINT('Ctrl Pts',(-50.,9.42632261579016,0.923642539206944));
#47134=CARTESIAN_POINT('Ctrl Pts',(-66.,9.54689939935545,0.885322978595271));
#47135=CARTESIAN_POINT('Ctrl Pts',(-50.,9.54689939935545,0.885322978595271));
#47136=CARTESIAN_POINT('Ctrl Pts',(-66.,9.66563362360549,0.847573647008884));
#47137=CARTESIAN_POINT('Ctrl Pts',(-50.,9.66563362360549,0.847573647008884));
#47138=CARTESIAN_POINT('Ctrl Pts',(-66.,9.78236252423293,0.811157274859099));
#47139=CARTESIAN_POINT('Ctrl Pts',(-50.,9.78236252423293,0.811157274859099));
#47140=CARTESIAN_POINT('Ctrl Pts',(-66.,9.89807533998404,0.772934850892815));
#47141=CARTESIAN_POINT('Ctrl Pts',(-50.,9.89807533998404,0.772934850892815));
#47142=CARTESIAN_POINT('Ctrl Pts',(-66.,10.0147109731333,0.726515765574518));
#47143=CARTESIAN_POINT('Ctrl Pts',(-50.,10.0147109731333,0.726515765574518));
#47144=CARTESIAN_POINT('Ctrl Pts',(-66.,10.1340524145698,0.665939265218336));
#47145=CARTESIAN_POINT('Ctrl Pts',(-50.,10.1340524145698,0.665939265218336));
#47146=CARTESIAN_POINT('Ctrl Pts',(-66.,10.2569101720987,0.588388804738333));
#47147=CARTESIAN_POINT('Ctrl Pts',(-50.,10.2569101720987,0.588388804738333));
#47148=CARTESIAN_POINT('Ctrl Pts',(-66.,10.3820648170252,0.497707417893672));
#47149=CARTESIAN_POINT('Ctrl Pts',(-50.,10.3820648170252,0.497707417893672));
#47150=CARTESIAN_POINT('Ctrl Pts',(-66.,10.5056603733136,0.406421718030022));
#47151=CARTESIAN_POINT('Ctrl Pts',(-50.,10.5056603733136,0.406421718030022));
#47152=CARTESIAN_POINT('Ctrl Pts',(-66.,10.6222927940147,0.332166401463227));
#47153=CARTESIAN_POINT('Ctrl Pts',(-50.,10.6222927940147,0.332166401463227));
#47154=CARTESIAN_POINT('Ctrl Pts',(-66.,10.7258647379785,0.294881497726767));
#47155=CARTESIAN_POINT('Ctrl Pts',(-50.,10.7258647379785,0.294881497726767));
#47156=CARTESIAN_POINT('Ctrl Pts',(-66.,10.8104930954534,0.313834765760248));
#47157=CARTESIAN_POINT('Ctrl Pts',(-50.,10.8104930954534,0.313834765760248));
#47158=CARTESIAN_POINT('Ctrl Pts',(-66.,10.8714829374831,0.404428597048679));
#47159=CARTESIAN_POINT('Ctrl Pts',(-50.,10.8714829374831,0.404428597048679));
#47160=CARTESIAN_POINT('Ctrl Pts',(-66.,10.905276089601,0.578361716765453));
#47161=CARTESIAN_POINT('Ctrl Pts',(-50.,10.905276089601,0.578361716765453));
#47162=CARTESIAN_POINT('Ctrl Pts',(-66.,10.9092546759344,0.844266149144153));
#47163=CARTESIAN_POINT('Ctrl Pts',(-50.,10.9092546759344,0.844266149144153));
#47164=CARTESIAN_POINT('Ctrl Pts',(-66.,10.8816048031854,1.20814783100236));
#47165=CARTESIAN_POINT('Ctrl Pts',(-50.,10.8816048031854,1.20814783100236));
#47166=CARTESIAN_POINT('Ctrl Pts',(-66.,10.8211630882956,1.67388388032334));
#47167=CARTESIAN_POINT('Ctrl Pts',(-50.,10.8211630882956,1.67388388032334));
#47168=CARTESIAN_POINT('Ctrl Pts',(-66.,10.7272782204132,2.24367111485021));
#47169=CARTESIAN_POINT('Ctrl Pts',(-50.,10.7272782204132,2.24367111485021));
#47170=CARTESIAN_POINT('Ctrl Pts',(-66.,10.599673061523,2.91847324890335));
#47171=CARTESIAN_POINT('Ctrl Pts',(-50.,10.599673061523,2.91847324890335));
#47172=CARTESIAN_POINT('Ctrl Pts',(-66.,10.4705848912574,3.54245347887044));
#47173=CARTESIAN_POINT('Ctrl Pts',(-50.,10.4705848912574,3.54245347887044));
#47174=CARTESIAN_POINT('Ctrl Pts',(-66.,10.3586144415421,4.05766357313591));
#47175=CARTESIAN_POINT('Ctrl Pts',(-50.,10.3586144415421,4.05766357313591));
#47176=CARTESIAN_POINT('Ctrl Pts',(-66.,10.2772411743483,4.42209792148691));
#47177=CARTESIAN_POINT('Ctrl Pts',(-50.,10.2772411743483,4.42209792148691));
#47178=CARTESIAN_POINT('Ctrl Pts',(-66.,10.234872965097,4.60955533520604));
#47179=CARTESIAN_POINT('Ctrl Pts',(-50.,10.234872965097,4.60955533520604));
#47180=CARTESIAN_POINT('',(-50.5,10.6195213806306,0.341160733863857));
#47181=CARTESIAN_POINT('',(-50.,10.1021455355716,0.679912184131802));
#47182=CARTESIAN_POINT('Ctrl Pts',(-50.5,10.6195213806306,0.34116073386385));
#47183=CARTESIAN_POINT('Ctrl Pts',(-50.4982567069816,10.6177491374168,0.342033889391285));
#47184=CARTESIAN_POINT('Ctrl Pts',(-50.4965113438794,10.6159742746229,0.342920316017751));
#47185=CARTESIAN_POINT('Ctrl Pts',(-50.3581212730818,10.4752046404048,0.414140015287625));
#47186=CARTESIAN_POINT('Ctrl Pts',(-50.2022201285479,10.3124422287015,0.566707861725606));
#47187=CARTESIAN_POINT('Ctrl Pts',(-50.,10.1021455355716,0.679912184131803));
#47188=CARTESIAN_POINT('Ctrl Pts',(-65.5,10.6195213806306,0.341160733863858));
#47189=CARTESIAN_POINT('Ctrl Pts',(-60.5,10.6195213806306,0.341160733863858));
#47190=CARTESIAN_POINT('Ctrl Pts',(-55.5,10.6195213806306,0.341160733863856));
#47191=CARTESIAN_POINT('Ctrl Pts',(-50.5,10.6195213806306,0.341160733863856));
#47192=CARTESIAN_POINT('Ctrl Pts',(-50.,7.75912709216827,0.911648516469146));
#47193=CARTESIAN_POINT('Ctrl Pts',(-50.,7.7827819679451,0.913594892602471));
#47194=CARTESIAN_POINT('Ctrl Pts',(-50.,7.83008004486546,0.917704563279999));
#47195=CARTESIAN_POINT('Ctrl Pts',(-50.,7.90099213574826,0.924519849384913));
#47196=CARTESIAN_POINT('Ctrl Pts',(-50.,7.99547145320256,0.934909974827099));
#47197=CARTESIAN_POINT('Ctrl Pts',(-50.,8.11346004702223,0.949941384652545));
#47198=CARTESIAN_POINT('Ctrl Pts',(-50.,8.23135817971997,0.966610353048665));
#47199=CARTESIAN_POINT('Ctrl Pts',(-50.,8.34920666168128,0.984096749349312));
#47200=CARTESIAN_POINT('Ctrl Pts',(-50.,8.4670747275092,1.00099948266857));
#47201=CARTESIAN_POINT('Ctrl Pts',(-50.,8.58506450113074,1.01552541886979));
#47202=CARTESIAN_POINT('Ctrl Pts',(-50.,8.70331780221627,1.02571312618391));
#47203=CARTESIAN_POINT('Ctrl Pts',(-50.,8.8220174241358,1.02964473126801));
#47204=CARTESIAN_POINT('Ctrl Pts',(-50.,8.94140355616308,1.02565827740144));
#47205=CARTESIAN_POINT('Ctrl Pts',(-50.,9.06167470185178,1.01263753582842));
#47206=CARTESIAN_POINT('Ctrl Pts',(-50.,9.18284466719198,0.990376172966252));
#47207=CARTESIAN_POINT('Ctrl Pts',(-50.,9.3046427086813,0.959827893625642));
#47208=CARTESIAN_POINT('Ctrl Pts',(-50.,9.42632261579016,0.923642539206944));
#47209=CARTESIAN_POINT('Ctrl Pts',(-50.,9.54689939935545,0.885322978595271));
#47210=CARTESIAN_POINT('Ctrl Pts',(-50.,9.66563362360549,0.847573647008884));
#47211=CARTESIAN_POINT('Ctrl Pts',(-50.,9.78236252423293,0.811157274859099));
#47212=CARTESIAN_POINT('Ctrl Pts',(-50.,9.89178972962325,0.775011122760694));
#47213=CARTESIAN_POINT('Ctrl Pts',(-50.,9.9787157732118,0.74081239160003));
#47214=CARTESIAN_POINT('Ctrl Pts',(-50.,10.0432742611121,0.710717535900332));
#47215=CARTESIAN_POINT('Ctrl Pts',(-50.,10.0846322123207,0.689339740324902));
#47216=CARTESIAN_POINT('Ctrl Pts',(-50.,10.1021455355716,0.679912184131802));
#47217=CARTESIAN_POINT('Origin',(-50.,9.18418542175504,2.4522184164664));
#47218=CARTESIAN_POINT('Origin',(-50.,0.,0.));
#47219=CARTESIAN_POINT('Origin',(-50.25,0.,0.));
#47220=CARTESIAN_POINT('Origin',(-50.5,0.,0.));
#47221=CARTESIAN_POINT('Origin',(-50.,0.,0.));
#47222=CARTESIAN_POINT('Origin',(-58.,0.,0.));
#47223=CARTESIAN_POINT('Origin',(-110.,6.,0.));
#47224=CARTESIAN_POINT('',(-110.,-6.,-7.34788079488411E-16));
#47225=CARTESIAN_POINT('Origin',(-110.,0.,0.));
#47226=CARTESIAN_POINT('Origin',(-109.5,0.,0.));
#47227=CARTESIAN_POINT('',(-109.5,-6.5,-7.96020419445779E-16));
#47228=CARTESIAN_POINT('Origin',(-66.25,0.,0.));
#47229=CARTESIAN_POINT('',(-66.25,-8.5625,-1.04860382176992E-15));
#47230=CARTESIAN_POINT('Origin',(-49.75,0.,0.));
#47231=CARTESIAN_POINT('',(-49.75,-8.5625,-1.04860382176992E-15));
#47232=CARTESIAN_POINT('Origin',(29.75,0.,0.));
#47233=CARTESIAN_POINT('Origin',(109.067,0.,0.));
#47234=CARTESIAN_POINT('Origin',(109.5,0.,0.));
#47235=CARTESIAN_POINT('',(110.,-6.,-7.34788079488411E-16));
#47236=CARTESIAN_POINT('Origin',(110.,0.,0.));
#47237=CARTESIAN_POINT('',(109.5,-6.5,-7.96020419445779E-16));
#47238=CARTESIAN_POINT('Origin',(110.,0.,0.));
#65539=UNCERTAINTY_MEASURE_WITH_UNIT(LENGTH_MEASURE(0.01),#65564,
'DISTANCE_ACCURACY_VALUE',
'Maximum model space distance between geometric entities at asserted c
onnectivities');
#65550=UNCERTAINTY_MEASURE_WITH_UNIT(LENGTH_MEASURE(0.01),#65564,
'DISTANCE_ACCURACY_VALUE',
'Maximum model space distance between geometric entities at asserted c
onnectivities');
#65552=(
GEOMETRIC_REPRESENTATION_CONTEXT(3)
GLOBAL_UNCERTAINTY_ASSIGNED_CONTEXT((#65539))
GLOBAL_UNIT_ASSIGNED_CONTEXT((#65564,#65566,#65567))
REPRESENTATION_CONTEXT('','3D')
);
#65563=(
GEOMETRIC_REPRESENTATION_CONTEXT(3)
GLOBAL_UNCERTAINTY_ASSIGNED_CONTEXT((#65550))
GLOBAL_UNIT_ASSIGNED_CONTEXT((#65564,#65566,#65567))
REPRESENTATION_CONTEXT('','3D')
);
#65564=(
LENGTH_UNIT()
NAMED_UNIT(*)
SI_UNIT(.MILLI.,.METRE.)
);
#65566=(
NAMED_UNIT(*)
PLANE_ANGLE_UNIT()
SI_UNIT($,.RADIAN.)
);
#65567=(
NAMED_UNIT(*)
SI_UNIT($,.STERADIAN.)
SOLID_ANGLE_UNIT()
);
#65569=SHAPE_DEFINITION_REPRESENTATION(#65581,#65614);
#65581=PRODUCT_DEFINITION_SHAPE('',$,#65627);
#65614=SHAPE_REPRESENTATION('',(#20142),#65552);
#65625=PRODUCT_DEFINITION_CONTEXT('part definition',#65663,'design');
#65627=PRODUCT_DEFINITION('2026-10-10-05-45-21-337',
'01_Axle_with_Machined_Sun_Pinion_Z15_M1.25',#65639,#65625);
#65639=PRODUCT_DEFINITION_FORMATION('',$,#65666);
#65663=APPLICATION_CONTEXT(
'Core Data for Automotive Mechanical Design Process');
#65664=PRODUCT_CONTEXT('part definition',#65663,'mechanical');
#65666=PRODUCT('2026-10-10-05-45-21-337',
'01_Axle_with_Machined_Sun_Pinion_Z15_M1.25',$,(#65664));
#65782=COLOUR_RGB('Grey',0.48,0.52,0.57);
#65783=FILL_AREA_STYLE_COLOUR('',#65782);
#65784=FILL_AREA_STYLE('',(#65783));
#65785=SURFACE_STYLE_FILL_AREA(#65784);
#65786=SURFACE_SIDE_STYLE('',(#65785));
#65787=SURFACE_STYLE_USAGE(.BOTH.,#65786);
#65788=PRESENTATION_STYLE_ASSIGNMENT((#65787));
ENDSEC;
END-ISO-10303-21;
